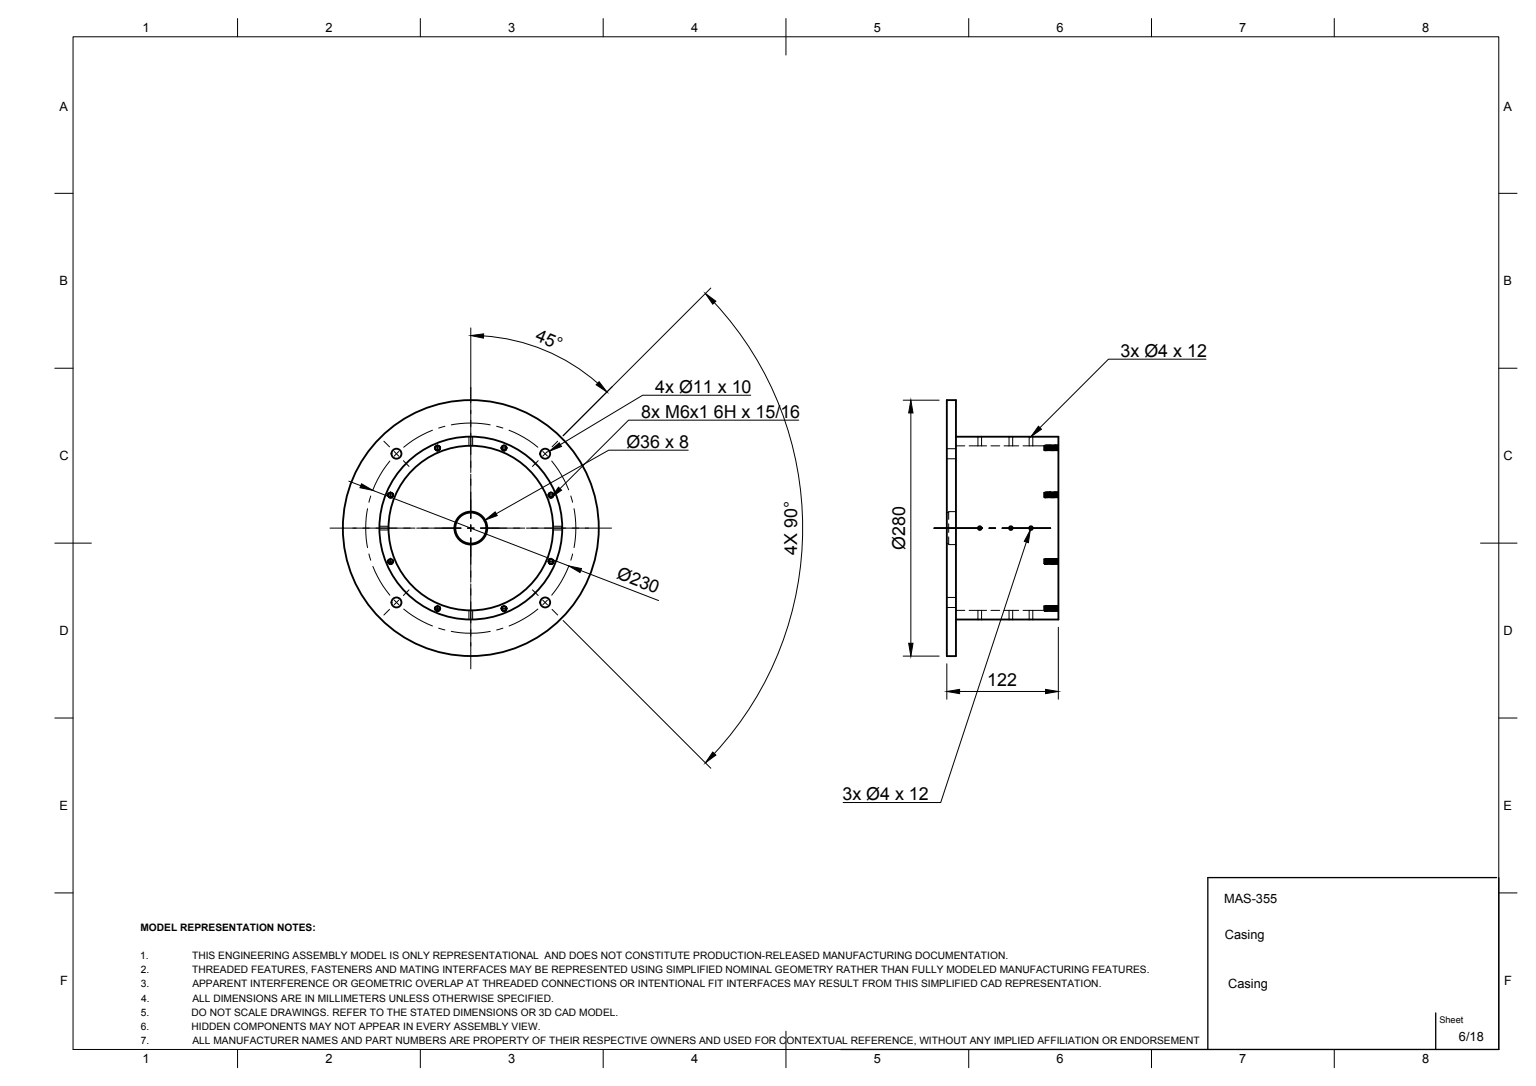
ISO-10303-21;
HEADER;
/* Generated by software containing ST-Developer
 * from STEP Tools, Inc. (www.steptools.com) 
 */

FILE_DESCRIPTION(
/* description */ ('Independent two-stage fixed-ring planetary gearbox,24/24/72 teeth,mod
ule2,20deg involutes,three planets per stage,4:1 x4:1=16:1. Native cut
-space/fillet/pattern tooth profiles derived from reusable gear blanks
; shared sun/planet/ring/carrier parts across both stages. Captured br
onze-journal input/carriers, headed retained planet pins, keyed inters
tage drive and modular keyed output interface. Native ideal gear links
; no torque, precision grade, production backlash/fits, lubrication, s
peed or life rating.'),
/* implementation_level */ '2;1');

FILE_NAME(
/* name */ 'Casing.step',
/* time_stamp */ '2026-11-08T19:10:00-08:00',
/* author */ (''),
/* organization */ (''),
/* preprocessor_version */ 'ST-DEVELOPER v20.2',
/* originating_system */ 'Autodesk Translation Framework v15.17.0.0',
/* authorisation */ '');

FILE_SCHEMA (('AUTOMOTIVE_DESIGN { 1 0 10303 214 3 1 1 }'));
ENDSEC;

DATA;
#10=MECHANICAL_DESIGN_GEOMETRIC_PRESENTATION_REPRESENTATION('',(#1163),#259224);
#1123=SHAPE_REPRESENTATION_RELATIONSHIP('SRR','None',#259370,#1143);
#1143=ADVANCED_BREP_SHAPE_REPRESENTATION('',(#1183),#259204);
#1163=STYLED_ITEM('',(#259479),#1183);
#1183=MANIFOLD_SOLID_BREP('Body1',#25150);
#1203=FACE_BOUND('',#3350,.T.);
#1204=FACE_BOUND('',#3352,.T.);
#1205=FACE_BOUND('',#3353,.T.);
#1206=FACE_BOUND('',#3354,.T.);
#1207=FACE_BOUND('',#3355,.T.);
#1208=FACE_BOUND('',#3356,.T.);
#1209=FACE_BOUND('',#3357,.T.);
#1210=FACE_BOUND('',#3358,.T.);
#1211=FACE_BOUND('',#3359,.T.);
#1212=FACE_BOUND('',#3360,.T.);
#1213=FACE_BOUND('',#3362,.T.);
#1214=FACE_BOUND('',#3363,.T.);
#1215=FACE_BOUND('',#3364,.T.);
#1216=FACE_BOUND('',#3365,.T.);
#1217=FACE_BOUND('',#3366,.T.);
#1218=FACE_BOUND('',#3367,.T.);
#1219=FACE_BOUND('',#3368,.T.);
#1220=FACE_BOUND('',#3369,.T.);
#1221=FACE_BOUND('',#3370,.T.);
#1222=FACE_BOUND('',#3372,.T.);
#1223=FACE_BOUND('',#3373,.T.);
#1224=FACE_BOUND('',#3374,.T.);
#1225=FACE_BOUND('',#3375,.T.);
#1226=FACE_BOUND('',#3376,.T.);
#1227=FACE_BOUND('',#3377,.T.);
#1228=FACE_BOUND('',#3378,.T.);
#1229=FACE_BOUND('',#3379,.T.);
#1230=FACE_BOUND('',#3380,.T.);
#1231=FACE_BOUND('',#3382,.T.);
#1232=FACE_BOUND('',#3383,.T.);
#1233=FACE_BOUND('',#3384,.T.);
#1234=FACE_BOUND('',#3385,.T.);
#1235=FACE_BOUND('',#3386,.T.);
#1236=FACE_BOUND('',#3390,.T.);
#1237=FACE_BOUND('',#3392,.T.);
#1238=FACE_BOUND('',#3393,.T.);
#1239=FACE_BOUND('',#3394,.T.);
#1240=FACE_BOUND('',#3395,.T.);
#1241=FACE_BOUND('',#3396,.T.);
#1318=B_SPLINE_SURFACE_WITH_KNOTS('',3,3,((#42197,#42198,#42199,#42200,
#42201,#42202,#42203,#42204,#42205,#42206,#42207,#42208,#42209,#42210,#42211,
#42212,#42213,#42214,#42215,#42216,#42217,#42218,#42219,#42220,#42221,#42222,
#42223,#42224,#42225,#42226,#42227,#42228,#42229,#42230,#42231,#42232,#42233,
#42234,#42235,#42236,#42237,#42238,#42239,#42240,#42241,#42242,#42243,#42244,
#42245,#42246,#42247,#42248,#42249,#42250,#42251,#42252,#42253,#42254,#42255,
#42256,#42257,#42258,#42259,#42260,#42261,#42262,#42263,#42264,#42265,#42266,
#42267,#42268,#42269,#42270,#42271,#42272,#42273,#42274,#42275,#42276,#42277,
#42278,#42279,#42280,#42281,#42282,#42283,#42284,#42285,#42286,#42287,#42288,
#42289,#42290,#42291,#42292,#42293,#42294,#42295,#42296),(#42297,#42298,
#42299,#42300,#42301,#42302,#42303,#42304,#42305,#42306,#42307,#42308,#42309,
#42310,#42311,#42312,#42313,#42314,#42315,#42316,#42317,#42318,#42319,#42320,
#42321,#42322,#42323,#42324,#42325,#42326,#42327,#42328,#42329,#42330,#42331,
#42332,#42333,#42334,#42335,#42336,#42337,#42338,#42339,#42340,#42341,#42342,
#42343,#42344,#42345,#42346,#42347,#42348,#42349,#42350,#42351,#42352,#42353,
#42354,#42355,#42356,#42357,#42358,#42359,#42360,#42361,#42362,#42363,#42364,
#42365,#42366,#42367,#42368,#42369,#42370,#42371,#42372,#42373,#42374,#42375,
#42376,#42377,#42378,#42379,#42380,#42381,#42382,#42383,#42384,#42385,#42386,
#42387,#42388,#42389,#42390,#42391,#42392,#42393,#42394,#42395,#42396),
(#42397,#42398,#42399,#42400,#42401,#42402,#42403,#42404,#42405,#42406,
#42407,#42408,#42409,#42410,#42411,#42412,#42413,#42414,#42415,#42416,#42417,
#42418,#42419,#42420,#42421,#42422,#42423,#42424,#42425,#42426,#42427,#42428,
#42429,#42430,#42431,#42432,#42433,#42434,#42435,#42436,#42437,#42438,#42439,
#42440,#42441,#42442,#42443,#42444,#42445,#42446,#42447,#42448,#42449,#42450,
#42451,#42452,#42453,#42454,#42455,#42456,#42457,#42458,#42459,#42460,#42461,
#42462,#42463,#42464,#42465,#42466,#42467,#42468,#42469,#42470,#42471,#42472,
#42473,#42474,#42475,#42476,#42477,#42478,#42479,#42480,#42481,#42482,#42483,
#42484,#42485,#42486,#42487,#42488,#42489,#42490,#42491,#42492,#42493,#42494,
#42495,#42496),(#42497,#42498,#42499,#42500,#42501,#42502,#42503,#42504,
#42505,#42506,#42507,#42508,#42509,#42510,#42511,#42512,#42513,#42514,#42515,
#42516,#42517,#42518,#42519,#42520,#42521,#42522,#42523,#42524,#42525,#42526,
#42527,#42528,#42529,#42530,#42531,#42532,#42533,#42534,#42535,#42536,#42537,
#42538,#42539,#42540,#42541,#42542,#42543,#42544,#42545,#42546,#42547,#42548,
#42549,#42550,#42551,#42552,#42553,#42554,#42555,#42556,#42557,#42558,#42559,
#42560,#42561,#42562,#42563,#42564,#42565,#42566,#42567,#42568,#42569,#42570,
#42571,#42572,#42573,#42574,#42575,#42576,#42577,#42578,#42579,#42580,#42581,
#42582,#42583,#42584,#42585,#42586,#42587,#42588,#42589,#42590,#42591,#42592,
#42593,#42594,#42595,#42596)),.UNSPECIFIED.,.F.,.F.,.F.,(4,4),(4,1,1,1,
1,1,1,1,1,1,1,1,1,1,1,1,1,1,1,1,1,1,1,1,1,1,1,1,1,1,1,1,1,1,1,1,1,1,1,1,
1,1,1,1,1,1,1,1,1,1,1,1,1,1,1,1,1,1,1,1,1,1,1,1,1,1,1,1,1,1,1,1,1,1,1,1,
1,1,1,1,1,1,1,1,1,1,1,1,1,1,1,1,1,1,1,1,1,4),(0.,0.064201349933887),(11.8589888623077,
12.8514087025213,13.843828542735,14.8362483829486,15.8286682231622,16.8210880633759,
17.8135079035895,18.8059277438031,19.7983475840168,20.7907674242304,21.783187264444,
22.7756071046577,23.7680269448713,24.7604467850849,25.7528666252985,26.7452864655122,
27.7377063057258,28.7301261459394,29.7225459861531,30.7149658263667,31.7073856665803,
32.699805506794,33.6922253470076,34.6846451872212,35.6770650274349,36.6694848676485,
37.6619047078621,38.6543245480758,39.6467443882894,40.639164228503,41.6315840687166,
42.6240039089303,43.6164237491439,44.6088435893575,45.6012634295712,46.5936832697848,
47.5861031099984,48.5785229502121,49.5709427904257,50.5633626306393,51.555782470853,
52.5482023110666,53.5406221512802,54.5330419914939,55.5254618317075,56.5178816719211,
57.5103015121348,58.5027213523484,59.495141192562,60.4875610327756,61.4799808729893,
62.4724007132029,63.4648205534165,64.4572403936302,65.4496602338438,66.4420800740574,
67.4344999142711,68.4269197544847,69.4193395946983,70.411759434912,71.4041792751256,
72.3965991153392,73.3890189555529,74.3814387957665,75.3738586359801,76.3662784761938,
77.3586983164074,78.351118156621,79.3435379968347,80.3359578370483,81.3283776772619,
82.3207975174756,83.3132173576892,84.3056371979028,85.2980570381164,86.2904768783301,
87.2828967185437,88.2753165587573,89.267736398971,90.2601562391846,91.2525760793982,
92.2449959196119,93.2374157598255,94.2298356000391,95.2222554402528,96.2146752804664,
97.20709512068,98.1995149608937,99.1919348011073,100.184354641321,101.176774481535,
102.169194321748,103.161614161962,104.154034002175,105.146453842389,106.138873682603,
107.131293522816,108.12371336303),.UNSPECIFIED.);
#1319=B_SPLINE_SURFACE_WITH_KNOTS('',3,3,((#42716,#42717,#42718,#42719,
#42720,#42721,#42722,#42723,#42724,#42725,#42726,#42727,#42728,#42729,#42730,
#42731,#42732,#42733,#42734,#42735,#42736,#42737,#42738,#42739,#42740,#42741,
#42742,#42743,#42744,#42745,#42746,#42747,#42748,#42749,#42750,#42751,#42752,
#42753,#42754,#42755,#42756,#42757,#42758,#42759,#42760,#42761,#42762,#42763,
#42764,#42765,#42766,#42767,#42768,#42769,#42770,#42771,#42772,#42773,#42774,
#42775,#42776,#42777,#42778,#42779,#42780,#42781,#42782,#42783,#42784,#42785,
#42786,#42787,#42788,#42789,#42790,#42791,#42792,#42793,#42794,#42795,#42796,
#42797,#42798,#42799,#42800,#42801,#42802,#42803,#42804,#42805,#42806,#42807,
#42808,#42809,#42810,#42811,#42812,#42813,#42814,#42815),(#42816,#42817,
#42818,#42819,#42820,#42821,#42822,#42823,#42824,#42825,#42826,#42827,#42828,
#42829,#42830,#42831,#42832,#42833,#42834,#42835,#42836,#42837,#42838,#42839,
#42840,#42841,#42842,#42843,#42844,#42845,#42846,#42847,#42848,#42849,#42850,
#42851,#42852,#42853,#42854,#42855,#42856,#42857,#42858,#42859,#42860,#42861,
#42862,#42863,#42864,#42865,#42866,#42867,#42868,#42869,#42870,#42871,#42872,
#42873,#42874,#42875,#42876,#42877,#42878,#42879,#42880,#42881,#42882,#42883,
#42884,#42885,#42886,#42887,#42888,#42889,#42890,#42891,#42892,#42893,#42894,
#42895,#42896,#42897,#42898,#42899,#42900,#42901,#42902,#42903,#42904,#42905,
#42906,#42907,#42908,#42909,#42910,#42911,#42912,#42913,#42914,#42915),
(#42916,#42917,#42918,#42919,#42920,#42921,#42922,#42923,#42924,#42925,
#42926,#42927,#42928,#42929,#42930,#42931,#42932,#42933,#42934,#42935,#42936,
#42937,#42938,#42939,#42940,#42941,#42942,#42943,#42944,#42945,#42946,#42947,
#42948,#42949,#42950,#42951,#42952,#42953,#42954,#42955,#42956,#42957,#42958,
#42959,#42960,#42961,#42962,#42963,#42964,#42965,#42966,#42967,#42968,#42969,
#42970,#42971,#42972,#42973,#42974,#42975,#42976,#42977,#42978,#42979,#42980,
#42981,#42982,#42983,#42984,#42985,#42986,#42987,#42988,#42989,#42990,#42991,
#42992,#42993,#42994,#42995,#42996,#42997,#42998,#42999,#43000,#43001,#43002,
#43003,#43004,#43005,#43006,#43007,#43008,#43009,#43010,#43011,#43012,#43013,
#43014,#43015),(#43016,#43017,#43018,#43019,#43020,#43021,#43022,#43023,
#43024,#43025,#43026,#43027,#43028,#43029,#43030,#43031,#43032,#43033,#43034,
#43035,#43036,#43037,#43038,#43039,#43040,#43041,#43042,#43043,#43044,#43045,
#43046,#43047,#43048,#43049,#43050,#43051,#43052,#43053,#43054,#43055,#43056,
#43057,#43058,#43059,#43060,#43061,#43062,#43063,#43064,#43065,#43066,#43067,
#43068,#43069,#43070,#43071,#43072,#43073,#43074,#43075,#43076,#43077,#43078,
#43079,#43080,#43081,#43082,#43083,#43084,#43085,#43086,#43087,#43088,#43089,
#43090,#43091,#43092,#43093,#43094,#43095,#43096,#43097,#43098,#43099,#43100,
#43101,#43102,#43103,#43104,#43105,#43106,#43107,#43108,#43109,#43110,#43111,
#43112,#43113,#43114,#43115)),.UNSPECIFIED.,.F.,.F.,.F.,(4,4),(4,1,1,1,
1,1,1,1,1,1,1,1,1,1,1,1,1,1,1,1,1,1,1,1,1,1,1,1,1,1,1,1,1,1,1,1,1,1,1,1,
1,1,1,1,1,1,1,1,1,1,1,1,1,1,1,1,1,1,1,1,1,1,1,1,1,1,1,1,1,1,1,1,1,1,1,1,
1,1,1,1,1,1,1,1,1,1,1,1,1,1,1,1,1,1,1,1,1,4),(0.,0.064201349933887),(14.3984001269718,
15.3908199671854,16.3832398073991,17.3756596476127,18.3680794878263,19.36049932804,
20.3529191682536,21.3453390084672,22.3377588486809,23.3301786888945,24.3225985291081,
25.3150183693218,26.3074382095354,27.299858049749,28.2922778899627,29.2846977301763,
30.2771175703899,31.2695374106036,32.2619572508172,33.2543770910308,34.2467969312444,
35.2392167714581,36.2316366116717,37.2240564518853,38.216476292099,39.2088961323126,
40.2013159725262,41.1937358127399,42.1861556529535,43.1785754931671,44.1709953333808,
45.1634151735944,46.155835013808,47.1482548540217,48.1406746942353,49.1330945344489,
50.1255143746626,51.1179342148762,52.1103540550898,53.1027738953035,54.0951937355171,
55.0876135757307,56.0800334159443,57.072453256158,58.0648730963716,59.0572929365852,
60.0497127767989,61.0421326170125,62.0345524572261,63.0269722974398,64.0193921376534,
65.011811977867,66.0042318180807,66.9966516582943,67.9890714985079,68.9814913387216,
69.9739111789352,70.9663310191488,71.9587508593625,72.9511706995761,73.9435905397897,
74.9360103800034,75.928430220217,76.9208500604306,77.9132699006443,78.9056897408579,
79.8981095810715,80.8905294212852,81.8829492614988,82.8753691017124,83.867788941926,
84.8602087821397,85.8526286223533,86.8450484625669,87.8374683027806,88.8298881429942,
89.8223079832078,90.8147278234215,91.8071476636351,92.7995675038487,93.7919873440624,
94.784407184276,95.7768270244896,96.7692468647032,97.7616667049169,98.7540865451305,
99.7465063853441,100.738926225558,101.731346065771,102.723765905985,103.716185746199,
104.708605586412,105.701025426626,106.69344526684,107.685865107053,108.678284947267,
109.67070478748,110.663124627694),.UNSPECIFIED.);
#1320=B_SPLINE_SURFACE_WITH_KNOTS('',3,3,((#43444,#43445,#43446,#43447,
#43448,#43449,#43450,#43451,#43452,#43453,#43454,#43455,#43456,#43457,#43458,
#43459,#43460,#43461,#43462,#43463,#43464,#43465,#43466,#43467,#43468,#43469,
#43470,#43471,#43472,#43473,#43474,#43475,#43476,#43477,#43478,#43479,#43480,
#43481,#43482,#43483,#43484,#43485,#43486,#43487,#43488,#43489,#43490,#43491,
#43492,#43493,#43494,#43495,#43496,#43497,#43498,#43499,#43500,#43501,#43502,
#43503,#43504,#43505,#43506,#43507,#43508,#43509,#43510,#43511,#43512,#43513,
#43514,#43515,#43516,#43517,#43518,#43519,#43520,#43521,#43522,#43523,#43524,
#43525,#43526,#43527,#43528,#43529,#43530,#43531,#43532,#43533,#43534,#43535,
#43536,#43537,#43538,#43539,#43540,#43541,#43542,#43543),(#43544,#43545,
#43546,#43547,#43548,#43549,#43550,#43551,#43552,#43553,#43554,#43555,#43556,
#43557,#43558,#43559,#43560,#43561,#43562,#43563,#43564,#43565,#43566,#43567,
#43568,#43569,#43570,#43571,#43572,#43573,#43574,#43575,#43576,#43577,#43578,
#43579,#43580,#43581,#43582,#43583,#43584,#43585,#43586,#43587,#43588,#43589,
#43590,#43591,#43592,#43593,#43594,#43595,#43596,#43597,#43598,#43599,#43600,
#43601,#43602,#43603,#43604,#43605,#43606,#43607,#43608,#43609,#43610,#43611,
#43612,#43613,#43614,#43615,#43616,#43617,#43618,#43619,#43620,#43621,#43622,
#43623,#43624,#43625,#43626,#43627,#43628,#43629,#43630,#43631,#43632,#43633,
#43634,#43635,#43636,#43637,#43638,#43639,#43640,#43641,#43642,#43643),
(#43644,#43645,#43646,#43647,#43648,#43649,#43650,#43651,#43652,#43653,
#43654,#43655,#43656,#43657,#43658,#43659,#43660,#43661,#43662,#43663,#43664,
#43665,#43666,#43667,#43668,#43669,#43670,#43671,#43672,#43673,#43674,#43675,
#43676,#43677,#43678,#43679,#43680,#43681,#43682,#43683,#43684,#43685,#43686,
#43687,#43688,#43689,#43690,#43691,#43692,#43693,#43694,#43695,#43696,#43697,
#43698,#43699,#43700,#43701,#43702,#43703,#43704,#43705,#43706,#43707,#43708,
#43709,#43710,#43711,#43712,#43713,#43714,#43715,#43716,#43717,#43718,#43719,
#43720,#43721,#43722,#43723,#43724,#43725,#43726,#43727,#43728,#43729,#43730,
#43731,#43732,#43733,#43734,#43735,#43736,#43737,#43738,#43739,#43740,#43741,
#43742,#43743),(#43744,#43745,#43746,#43747,#43748,#43749,#43750,#43751,
#43752,#43753,#43754,#43755,#43756,#43757,#43758,#43759,#43760,#43761,#43762,
#43763,#43764,#43765,#43766,#43767,#43768,#43769,#43770,#43771,#43772,#43773,
#43774,#43775,#43776,#43777,#43778,#43779,#43780,#43781,#43782,#43783,#43784,
#43785,#43786,#43787,#43788,#43789,#43790,#43791,#43792,#43793,#43794,#43795,
#43796,#43797,#43798,#43799,#43800,#43801,#43802,#43803,#43804,#43805,#43806,
#43807,#43808,#43809,#43810,#43811,#43812,#43813,#43814,#43815,#43816,#43817,
#43818,#43819,#43820,#43821,#43822,#43823,#43824,#43825,#43826,#43827,#43828,
#43829,#43830,#43831,#43832,#43833,#43834,#43835,#43836,#43837,#43838,#43839,
#43840,#43841,#43842,#43843)),.UNSPECIFIED.,.F.,.F.,.F.,(4,4),(4,1,1,1,
1,1,1,1,1,1,1,1,1,1,1,1,1,1,1,1,1,1,1,1,1,1,1,1,1,1,1,1,1,1,1,1,1,1,1,1,
1,1,1,1,1,1,1,1,1,1,1,1,1,1,1,1,1,1,1,1,1,1,1,1,1,1,1,1,1,1,1,1,1,1,1,1,
1,1,1,1,1,1,1,1,1,1,1,1,1,1,1,1,1,1,1,1,1,4),(0.,0.064201349933887),(11.8589888623077,
12.8514087025213,13.843828542735,14.8362483829486,15.8286682231622,16.8210880633759,
17.8135079035895,18.8059277438031,19.7983475840168,20.7907674242304,21.783187264444,
22.7756071046577,23.7680269448713,24.7604467850849,25.7528666252986,26.7452864655122,
27.7377063057259,28.7301261459395,29.7225459861531,30.7149658263668,31.7073856665804,
32.699805506794,33.6922253470076,34.6846451872213,35.6770650274349,36.6694848676485,
37.6619047078622,38.6543245480758,39.6467443882895,40.6391642285031,41.6315840687167,
42.6240039089304,43.616423749144,44.6088435893576,45.6012634295713,46.5936832697849,
47.5861031099985,48.5785229502122,49.5709427904258,50.5633626306394,51.5557824708531,
52.5482023110667,53.5406221512803,54.533041991494,55.5254618317076,56.5178816719212,
57.5103015121349,58.5027213523485,59.4951411925621,60.4875610327758,61.4799808729894,
62.472400713203,63.4648205534167,64.4572403936303,65.4496602338439,66.4420800740576,
67.4344999142712,68.4269197544848,69.4193395946985,70.4117594349121,71.4041792751257,
72.3965991153394,73.389018955553,74.3814387957666,75.3738586359803,76.3662784761939,
77.3586983164075,78.3511181566212,79.3435379968348,80.3359578370484,81.3283776772621,
82.3207975174757,83.3132173576894,84.305637197903,85.2980570381166,86.2904768783303,
87.2828967185439,88.2753165587575,89.2677363989712,90.2601562391848,91.2525760793984,
92.2449959196121,93.2374157598257,94.2298356000393,95.222255440253,96.2146752804666,
97.2070951206802,98.1995149608939,99.1919348011075,100.184354641321,101.176774481535,
102.169194321748,103.161614161962,104.154034002176,105.146453842389,106.138873682603,
107.131293522817,108.12371336303),.UNSPECIFIED.);
#1321=B_SPLINE_SURFACE_WITH_KNOTS('',3,3,((#43963,#43964,#43965,#43966,
#43967,#43968,#43969,#43970,#43971,#43972,#43973,#43974,#43975,#43976,#43977,
#43978,#43979,#43980,#43981,#43982,#43983,#43984,#43985,#43986,#43987,#43988,
#43989,#43990,#43991,#43992,#43993,#43994,#43995,#43996,#43997,#43998,#43999,
#44000,#44001,#44002,#44003,#44004,#44005,#44006,#44007,#44008,#44009,#44010,
#44011,#44012,#44013,#44014,#44015,#44016,#44017,#44018,#44019,#44020,#44021,
#44022,#44023,#44024,#44025,#44026,#44027,#44028,#44029,#44030,#44031,#44032,
#44033,#44034,#44035,#44036,#44037,#44038,#44039,#44040,#44041,#44042,#44043,
#44044,#44045,#44046,#44047,#44048,#44049,#44050,#44051,#44052,#44053,#44054,
#44055,#44056,#44057,#44058,#44059,#44060,#44061,#44062),(#44063,#44064,
#44065,#44066,#44067,#44068,#44069,#44070,#44071,#44072,#44073,#44074,#44075,
#44076,#44077,#44078,#44079,#44080,#44081,#44082,#44083,#44084,#44085,#44086,
#44087,#44088,#44089,#44090,#44091,#44092,#44093,#44094,#44095,#44096,#44097,
#44098,#44099,#44100,#44101,#44102,#44103,#44104,#44105,#44106,#44107,#44108,
#44109,#44110,#44111,#44112,#44113,#44114,#44115,#44116,#44117,#44118,#44119,
#44120,#44121,#44122,#44123,#44124,#44125,#44126,#44127,#44128,#44129,#44130,
#44131,#44132,#44133,#44134,#44135,#44136,#44137,#44138,#44139,#44140,#44141,
#44142,#44143,#44144,#44145,#44146,#44147,#44148,#44149,#44150,#44151,#44152,
#44153,#44154,#44155,#44156,#44157,#44158,#44159,#44160,#44161,#44162),
(#44163,#44164,#44165,#44166,#44167,#44168,#44169,#44170,#44171,#44172,
#44173,#44174,#44175,#44176,#44177,#44178,#44179,#44180,#44181,#44182,#44183,
#44184,#44185,#44186,#44187,#44188,#44189,#44190,#44191,#44192,#44193,#44194,
#44195,#44196,#44197,#44198,#44199,#44200,#44201,#44202,#44203,#44204,#44205,
#44206,#44207,#44208,#44209,#44210,#44211,#44212,#44213,#44214,#44215,#44216,
#44217,#44218,#44219,#44220,#44221,#44222,#44223,#44224,#44225,#44226,#44227,
#44228,#44229,#44230,#44231,#44232,#44233,#44234,#44235,#44236,#44237,#44238,
#44239,#44240,#44241,#44242,#44243,#44244,#44245,#44246,#44247,#44248,#44249,
#44250,#44251,#44252,#44253,#44254,#44255,#44256,#44257,#44258,#44259,#44260,
#44261,#44262),(#44263,#44264,#44265,#44266,#44267,#44268,#44269,#44270,
#44271,#44272,#44273,#44274,#44275,#44276,#44277,#44278,#44279,#44280,#44281,
#44282,#44283,#44284,#44285,#44286,#44287,#44288,#44289,#44290,#44291,#44292,
#44293,#44294,#44295,#44296,#44297,#44298,#44299,#44300,#44301,#44302,#44303,
#44304,#44305,#44306,#44307,#44308,#44309,#44310,#44311,#44312,#44313,#44314,
#44315,#44316,#44317,#44318,#44319,#44320,#44321,#44322,#44323,#44324,#44325,
#44326,#44327,#44328,#44329,#44330,#44331,#44332,#44333,#44334,#44335,#44336,
#44337,#44338,#44339,#44340,#44341,#44342,#44343,#44344,#44345,#44346,#44347,
#44348,#44349,#44350,#44351,#44352,#44353,#44354,#44355,#44356,#44357,#44358,
#44359,#44360,#44361,#44362)),.UNSPECIFIED.,.F.,.F.,.F.,(4,4),(4,1,1,1,
1,1,1,1,1,1,1,1,1,1,1,1,1,1,1,1,1,1,1,1,1,1,1,1,1,1,1,1,1,1,1,1,1,1,1,1,
1,1,1,1,1,1,1,1,1,1,1,1,1,1,1,1,1,1,1,1,1,1,1,1,1,1,1,1,1,1,1,1,1,1,1,1,
1,1,1,1,1,1,1,1,1,1,1,1,1,1,1,1,1,1,1,1,1,4),(0.,0.064201349933887),(14.3984001269718,
15.3908199671854,16.3832398073991,17.3756596476127,18.3680794878263,19.36049932804,
20.3529191682536,21.3453390084673,22.3377588486809,23.3301786888945,24.3225985291082,
25.3150183693218,26.3074382095354,27.2998580497491,28.2922778899627,29.2846977301763,
30.27711757039,31.2695374106036,32.2619572508172,33.2543770910309,34.2467969312445,
35.2392167714581,36.2316366116718,37.2240564518854,38.216476292099,39.2088961323127,
40.2013159725263,41.1937358127399,42.1861556529536,43.1785754931672,44.1709953333808,
45.1634151735945,46.1558350138081,47.1482548540217,48.1406746942354,49.133094534449,
50.1255143746626,51.1179342148763,52.1103540550899,53.1027738953035,54.0951937355172,
55.0876135757308,56.0800334159444,57.0724532561581,58.0648730963717,59.0572929365853,
60.049712776799,61.0421326170126,62.0345524572262,63.0269722974399,64.0193921376535,
65.0118119778672,66.0042318180808,66.9966516582944,67.9890714985081,68.9814913387217,
69.9739111789353,70.966331019149,71.9587508593626,72.9511706995762,73.9435905397899,
74.9360103800035,75.9284302202171,76.9208500604308,77.9132699006444,78.905689740858,
79.8981095810717,80.8905294212853,81.8829492614989,82.8753691017126,83.8677889419262,
84.8602087821398,85.8526286223535,86.8450484625671,87.8374683027807,88.8298881429944,
89.822307983208,90.8147278234216,91.8071476636353,92.7995675038489,93.7919873440625,
94.7844071842762,95.7768270244898,96.7692468647034,97.7616667049171,98.7540865451307,
99.7465063853443,100.738926225558,101.731346065772,102.723765905985,103.716185746199,
104.708605586413,105.701025426626,106.69344526684,107.685865107053,108.678284947267,
109.670704787481,110.663124627694),.UNSPECIFIED.);
#1322=B_SPLINE_SURFACE_WITH_KNOTS('',3,3,((#44691,#44692,#44693,#44694,
#44695,#44696,#44697,#44698,#44699,#44700,#44701,#44702,#44703,#44704,#44705,
#44706,#44707,#44708,#44709,#44710,#44711,#44712,#44713,#44714,#44715,#44716,
#44717,#44718,#44719,#44720,#44721,#44722,#44723,#44724,#44725,#44726,#44727,
#44728,#44729,#44730,#44731,#44732,#44733,#44734,#44735,#44736,#44737,#44738,
#44739,#44740,#44741,#44742,#44743,#44744,#44745,#44746,#44747,#44748,#44749,
#44750,#44751,#44752,#44753,#44754,#44755,#44756,#44757,#44758,#44759,#44760,
#44761,#44762,#44763,#44764,#44765,#44766,#44767,#44768,#44769,#44770,#44771,
#44772,#44773,#44774,#44775,#44776,#44777,#44778,#44779,#44780,#44781,#44782,
#44783,#44784,#44785,#44786,#44787,#44788,#44789,#44790),(#44791,#44792,
#44793,#44794,#44795,#44796,#44797,#44798,#44799,#44800,#44801,#44802,#44803,
#44804,#44805,#44806,#44807,#44808,#44809,#44810,#44811,#44812,#44813,#44814,
#44815,#44816,#44817,#44818,#44819,#44820,#44821,#44822,#44823,#44824,#44825,
#44826,#44827,#44828,#44829,#44830,#44831,#44832,#44833,#44834,#44835,#44836,
#44837,#44838,#44839,#44840,#44841,#44842,#44843,#44844,#44845,#44846,#44847,
#44848,#44849,#44850,#44851,#44852,#44853,#44854,#44855,#44856,#44857,#44858,
#44859,#44860,#44861,#44862,#44863,#44864,#44865,#44866,#44867,#44868,#44869,
#44870,#44871,#44872,#44873,#44874,#44875,#44876,#44877,#44878,#44879,#44880,
#44881,#44882,#44883,#44884,#44885,#44886,#44887,#44888,#44889,#44890),
(#44891,#44892,#44893,#44894,#44895,#44896,#44897,#44898,#44899,#44900,
#44901,#44902,#44903,#44904,#44905,#44906,#44907,#44908,#44909,#44910,#44911,
#44912,#44913,#44914,#44915,#44916,#44917,#44918,#44919,#44920,#44921,#44922,
#44923,#44924,#44925,#44926,#44927,#44928,#44929,#44930,#44931,#44932,#44933,
#44934,#44935,#44936,#44937,#44938,#44939,#44940,#44941,#44942,#44943,#44944,
#44945,#44946,#44947,#44948,#44949,#44950,#44951,#44952,#44953,#44954,#44955,
#44956,#44957,#44958,#44959,#44960,#44961,#44962,#44963,#44964,#44965,#44966,
#44967,#44968,#44969,#44970,#44971,#44972,#44973,#44974,#44975,#44976,#44977,
#44978,#44979,#44980,#44981,#44982,#44983,#44984,#44985,#44986,#44987,#44988,
#44989,#44990),(#44991,#44992,#44993,#44994,#44995,#44996,#44997,#44998,
#44999,#45000,#45001,#45002,#45003,#45004,#45005,#45006,#45007,#45008,#45009,
#45010,#45011,#45012,#45013,#45014,#45015,#45016,#45017,#45018,#45019,#45020,
#45021,#45022,#45023,#45024,#45025,#45026,#45027,#45028,#45029,#45030,#45031,
#45032,#45033,#45034,#45035,#45036,#45037,#45038,#45039,#45040,#45041,#45042,
#45043,#45044,#45045,#45046,#45047,#45048,#45049,#45050,#45051,#45052,#45053,
#45054,#45055,#45056,#45057,#45058,#45059,#45060,#45061,#45062,#45063,#45064,
#45065,#45066,#45067,#45068,#45069,#45070,#45071,#45072,#45073,#45074,#45075,
#45076,#45077,#45078,#45079,#45080,#45081,#45082,#45083,#45084,#45085,#45086,
#45087,#45088,#45089,#45090)),.UNSPECIFIED.,.F.,.F.,.F.,(4,4),(4,1,1,1,
1,1,1,1,1,1,1,1,1,1,1,1,1,1,1,1,1,1,1,1,1,1,1,1,1,1,1,1,1,1,1,1,1,1,1,1,
1,1,1,1,1,1,1,1,1,1,1,1,1,1,1,1,1,1,1,1,1,1,1,1,1,1,1,1,1,1,1,1,1,1,1,1,
1,1,1,1,1,1,1,1,1,1,1,1,1,1,1,1,1,1,1,1,1,4),(0.,0.064201349933887),(11.8589888623078,
12.8514087025215,13.8438285427351,14.8362483829487,15.8286682231624,16.821088063376,
17.8135079035896,18.8059277438032,19.7983475840169,20.7907674242305,21.7831872644441,
22.7756071046578,23.7680269448714,24.760446785085,25.7528666252987,26.7452864655123,
27.7377063057259,28.7301261459396,29.7225459861532,30.7149658263668,31.7073856665805,
32.6998055067941,33.6922253470077,34.6846451872214,35.677065027435,36.6694848676486,
37.6619047078623,38.6543245480759,39.6467443882895,40.6391642285032,41.6315840687168,
42.6240039089304,43.6164237491441,44.6088435893577,45.6012634295713,46.593683269785,
47.5861031099986,48.5785229502122,49.5709427904259,50.5633626306395,51.5557824708531,
52.5482023110668,53.5406221512804,54.533041991494,55.5254618317077,56.5178816719213,
57.5103015121349,58.5027213523486,59.4951411925622,60.4875610327758,61.4799808729895,
62.4724007132031,63.4648205534167,64.4572403936303,65.449660233844,66.4420800740576,
67.4344999142712,68.4269197544849,69.4193395946985,70.4117594349121,71.4041792751258,
72.3965991153394,73.389018955553,74.3814387957667,75.3738586359803,76.3662784761939,
77.3586983164076,78.3511181566212,79.3435379968348,80.3359578370485,81.3283776772621,
82.3207975174757,83.3132173576894,84.305637197903,85.2980570381166,86.2904768783303,
87.2828967185439,88.2753165587575,89.2677363989712,90.2601562391848,91.2525760793984,
92.2449959196121,93.2374157598257,94.2298356000393,95.222255440253,96.2146752804666,
97.2070951206802,98.1995149608939,99.1919348011075,100.184354641321,101.176774481535,
102.169194321748,103.161614161962,104.154034002176,105.146453842389,106.138873682603,
107.131293522817,108.12371336303),.UNSPECIFIED.);
#1323=B_SPLINE_SURFACE_WITH_KNOTS('',3,3,((#45210,#45211,#45212,#45213,
#45214,#45215,#45216,#45217,#45218,#45219,#45220,#45221,#45222,#45223,#45224,
#45225,#45226,#45227,#45228,#45229,#45230,#45231,#45232,#45233,#45234,#45235,
#45236,#45237,#45238,#45239,#45240,#45241,#45242,#45243,#45244,#45245,#45246,
#45247,#45248,#45249,#45250,#45251,#45252,#45253,#45254,#45255,#45256,#45257,
#45258,#45259,#45260,#45261,#45262,#45263,#45264,#45265,#45266,#45267,#45268,
#45269,#45270,#45271,#45272,#45273,#45274,#45275,#45276,#45277,#45278,#45279,
#45280,#45281,#45282,#45283,#45284,#45285,#45286,#45287,#45288,#45289,#45290,
#45291,#45292,#45293,#45294,#45295,#45296,#45297,#45298,#45299,#45300,#45301,
#45302,#45303,#45304,#45305,#45306,#45307,#45308,#45309),(#45310,#45311,
#45312,#45313,#45314,#45315,#45316,#45317,#45318,#45319,#45320,#45321,#45322,
#45323,#45324,#45325,#45326,#45327,#45328,#45329,#45330,#45331,#45332,#45333,
#45334,#45335,#45336,#45337,#45338,#45339,#45340,#45341,#45342,#45343,#45344,
#45345,#45346,#45347,#45348,#45349,#45350,#45351,#45352,#45353,#45354,#45355,
#45356,#45357,#45358,#45359,#45360,#45361,#45362,#45363,#45364,#45365,#45366,
#45367,#45368,#45369,#45370,#45371,#45372,#45373,#45374,#45375,#45376,#45377,
#45378,#45379,#45380,#45381,#45382,#45383,#45384,#45385,#45386,#45387,#45388,
#45389,#45390,#45391,#45392,#45393,#45394,#45395,#45396,#45397,#45398,#45399,
#45400,#45401,#45402,#45403,#45404,#45405,#45406,#45407,#45408,#45409),
(#45410,#45411,#45412,#45413,#45414,#45415,#45416,#45417,#45418,#45419,
#45420,#45421,#45422,#45423,#45424,#45425,#45426,#45427,#45428,#45429,#45430,
#45431,#45432,#45433,#45434,#45435,#45436,#45437,#45438,#45439,#45440,#45441,
#45442,#45443,#45444,#45445,#45446,#45447,#45448,#45449,#45450,#45451,#45452,
#45453,#45454,#45455,#45456,#45457,#45458,#45459,#45460,#45461,#45462,#45463,
#45464,#45465,#45466,#45467,#45468,#45469,#45470,#45471,#45472,#45473,#45474,
#45475,#45476,#45477,#45478,#45479,#45480,#45481,#45482,#45483,#45484,#45485,
#45486,#45487,#45488,#45489,#45490,#45491,#45492,#45493,#45494,#45495,#45496,
#45497,#45498,#45499,#45500,#45501,#45502,#45503,#45504,#45505,#45506,#45507,
#45508,#45509),(#45510,#45511,#45512,#45513,#45514,#45515,#45516,#45517,
#45518,#45519,#45520,#45521,#45522,#45523,#45524,#45525,#45526,#45527,#45528,
#45529,#45530,#45531,#45532,#45533,#45534,#45535,#45536,#45537,#45538,#45539,
#45540,#45541,#45542,#45543,#45544,#45545,#45546,#45547,#45548,#45549,#45550,
#45551,#45552,#45553,#45554,#45555,#45556,#45557,#45558,#45559,#45560,#45561,
#45562,#45563,#45564,#45565,#45566,#45567,#45568,#45569,#45570,#45571,#45572,
#45573,#45574,#45575,#45576,#45577,#45578,#45579,#45580,#45581,#45582,#45583,
#45584,#45585,#45586,#45587,#45588,#45589,#45590,#45591,#45592,#45593,#45594,
#45595,#45596,#45597,#45598,#45599,#45600,#45601,#45602,#45603,#45604,#45605,
#45606,#45607,#45608,#45609)),.UNSPECIFIED.,.F.,.F.,.F.,(4,4),(4,1,1,1,
1,1,1,1,1,1,1,1,1,1,1,1,1,1,1,1,1,1,1,1,1,1,1,1,1,1,1,1,1,1,1,1,1,1,1,1,
1,1,1,1,1,1,1,1,1,1,1,1,1,1,1,1,1,1,1,1,1,1,1,1,1,1,1,1,1,1,1,1,1,1,1,1,
1,1,1,1,1,1,1,1,1,1,1,1,1,1,1,1,1,1,1,1,1,4),(0.,0.064201349933887),(14.3984001269719,
15.3908199671856,16.3832398073992,17.3756596476128,18.3680794878265,19.3604993280401,
20.3529191682537,21.3453390084674,22.337758848681,23.3301786888946,24.3225985291083,
25.3150183693219,26.3074382095355,27.2998580497492,28.2922778899628,29.2846977301764,
30.2771175703901,31.2695374106037,32.2619572508173,33.2543770910309,34.2467969312446,
35.2392167714582,36.2316366116718,37.2240564518855,38.2164762920991,39.2088961323127,
40.2013159725264,41.19373581274,42.1861556529536,43.1785754931673,44.1709953333809,
45.1634151735945,46.1558350138082,47.1482548540218,48.1406746942354,49.1330945344491,
50.1255143746627,51.1179342148763,52.11035405509,53.1027738953036,54.0951937355172,
55.0876135757309,56.0800334159445,57.0724532561581,58.0648730963718,59.0572929365854,
60.049712776799,61.0421326170127,62.0345524572263,63.0269722974399,64.0193921376536,
65.0118119778672,66.0042318180808,66.9966516582945,67.9890714985081,68.9814913387217,
69.9739111789354,70.966331019149,71.9587508593626,72.9511706995763,73.9435905397899,
74.9360103800035,75.9284302202172,76.9208500604308,77.9132699006444,78.9056897408581,
79.8981095810717,80.8905294212853,81.882949261499,82.8753691017126,83.8677889419262,
84.8602087821399,85.8526286223535,86.8450484625671,87.8374683027808,88.8298881429944,
89.822307983208,90.8147278234217,91.8071476636353,92.7995675038489,93.7919873440626,
94.7844071842762,95.7768270244898,96.7692468647035,97.7616667049171,98.7540865451307,
99.7465063853444,100.738926225558,101.731346065772,102.723765905985,103.716185746199,
104.708605586413,105.701025426626,106.69344526684,107.685865107053,108.678284947267,
109.670704787481,110.663124627694),.UNSPECIFIED.);
#1324=B_SPLINE_SURFACE_WITH_KNOTS('',3,3,((#45938,#45939,#45940,#45941,
#45942,#45943,#45944,#45945,#45946,#45947,#45948,#45949,#45950,#45951,#45952,
#45953,#45954,#45955,#45956,#45957,#45958,#45959,#45960,#45961,#45962,#45963,
#45964,#45965,#45966,#45967,#45968,#45969,#45970,#45971,#45972,#45973,#45974,
#45975,#45976,#45977,#45978,#45979,#45980,#45981,#45982,#45983,#45984,#45985,
#45986,#45987,#45988,#45989,#45990,#45991,#45992,#45993,#45994,#45995,#45996,
#45997,#45998,#45999,#46000,#46001,#46002,#46003,#46004,#46005,#46006,#46007,
#46008,#46009,#46010,#46011,#46012,#46013,#46014,#46015,#46016,#46017,#46018,
#46019,#46020,#46021,#46022,#46023,#46024,#46025,#46026,#46027,#46028,#46029,
#46030,#46031,#46032,#46033,#46034,#46035,#46036,#46037),(#46038,#46039,
#46040,#46041,#46042,#46043,#46044,#46045,#46046,#46047,#46048,#46049,#46050,
#46051,#46052,#46053,#46054,#46055,#46056,#46057,#46058,#46059,#46060,#46061,
#46062,#46063,#46064,#46065,#46066,#46067,#46068,#46069,#46070,#46071,#46072,
#46073,#46074,#46075,#46076,#46077,#46078,#46079,#46080,#46081,#46082,#46083,
#46084,#46085,#46086,#46087,#46088,#46089,#46090,#46091,#46092,#46093,#46094,
#46095,#46096,#46097,#46098,#46099,#46100,#46101,#46102,#46103,#46104,#46105,
#46106,#46107,#46108,#46109,#46110,#46111,#46112,#46113,#46114,#46115,#46116,
#46117,#46118,#46119,#46120,#46121,#46122,#46123,#46124,#46125,#46126,#46127,
#46128,#46129,#46130,#46131,#46132,#46133,#46134,#46135,#46136,#46137),
(#46138,#46139,#46140,#46141,#46142,#46143,#46144,#46145,#46146,#46147,
#46148,#46149,#46150,#46151,#46152,#46153,#46154,#46155,#46156,#46157,#46158,
#46159,#46160,#46161,#46162,#46163,#46164,#46165,#46166,#46167,#46168,#46169,
#46170,#46171,#46172,#46173,#46174,#46175,#46176,#46177,#46178,#46179,#46180,
#46181,#46182,#46183,#46184,#46185,#46186,#46187,#46188,#46189,#46190,#46191,
#46192,#46193,#46194,#46195,#46196,#46197,#46198,#46199,#46200,#46201,#46202,
#46203,#46204,#46205,#46206,#46207,#46208,#46209,#46210,#46211,#46212,#46213,
#46214,#46215,#46216,#46217,#46218,#46219,#46220,#46221,#46222,#46223,#46224,
#46225,#46226,#46227,#46228,#46229,#46230,#46231,#46232,#46233,#46234,#46235,
#46236,#46237),(#46238,#46239,#46240,#46241,#46242,#46243,#46244,#46245,
#46246,#46247,#46248,#46249,#46250,#46251,#46252,#46253,#46254,#46255,#46256,
#46257,#46258,#46259,#46260,#46261,#46262,#46263,#46264,#46265,#46266,#46267,
#46268,#46269,#46270,#46271,#46272,#46273,#46274,#46275,#46276,#46277,#46278,
#46279,#46280,#46281,#46282,#46283,#46284,#46285,#46286,#46287,#46288,#46289,
#46290,#46291,#46292,#46293,#46294,#46295,#46296,#46297,#46298,#46299,#46300,
#46301,#46302,#46303,#46304,#46305,#46306,#46307,#46308,#46309,#46310,#46311,
#46312,#46313,#46314,#46315,#46316,#46317,#46318,#46319,#46320,#46321,#46322,
#46323,#46324,#46325,#46326,#46327,#46328,#46329,#46330,#46331,#46332,#46333,
#46334,#46335,#46336,#46337)),.UNSPECIFIED.,.F.,.F.,.F.,(4,4),(4,1,1,1,
1,1,1,1,1,1,1,1,1,1,1,1,1,1,1,1,1,1,1,1,1,1,1,1,1,1,1,1,1,1,1,1,1,1,1,1,
1,1,1,1,1,1,1,1,1,1,1,1,1,1,1,1,1,1,1,1,1,1,1,1,1,1,1,1,1,1,1,1,1,1,1,1,
1,1,1,1,1,1,1,1,1,1,1,1,1,1,1,1,1,1,1,1,1,4),(0.,0.064201349933887),(11.8589888623077,
12.8514087025213,13.843828542735,14.8362483829486,15.8286682231622,16.8210880633759,
17.8135079035895,18.8059277438031,19.7983475840168,20.7907674242304,21.783187264444,
22.7756071046577,23.7680269448713,24.7604467850849,25.7528666252986,26.7452864655122,
27.7377063057258,28.7301261459395,29.7225459861531,30.7149658263667,31.7073856665804,
32.699805506794,33.6922253470076,34.6846451872213,35.6770650274349,36.6694848676485,
37.6619047078622,38.6543245480758,39.6467443882894,40.6391642285031,41.6315840687167,
42.6240039089303,43.616423749144,44.6088435893576,45.6012634295713,46.5936832697849,
47.5861031099985,48.5785229502122,49.5709427904258,50.5633626306394,51.5557824708531,
52.5482023110667,53.5406221512803,54.533041991494,55.5254618317076,56.5178816719212,
57.5103015121349,58.5027213523485,59.4951411925621,60.4875610327758,61.4799808729894,
62.472400713203,63.4648205534167,64.4572403936303,65.4496602338439,66.4420800740576,
67.4344999142712,68.4269197544848,69.4193395946985,70.4117594349121,71.4041792751257,
72.3965991153394,73.389018955553,74.3814387957666,75.3738586359803,76.3662784761939,
77.3586983164075,78.3511181566212,79.3435379968348,80.3359578370484,81.3283776772621,
82.3207975174757,83.3132173576893,84.305637197903,85.2980570381166,86.2904768783302,
87.2828967185439,88.2753165587575,89.2677363989711,90.2601562391848,91.2525760793984,
92.2449959196121,93.2374157598257,94.2298356000393,95.222255440253,96.2146752804666,
97.2070951206802,98.1995149608939,99.1919348011075,100.184354641321,101.176774481535,
102.169194321748,103.161614161962,104.154034002176,105.146453842389,106.138873682603,
107.131293522817,108.12371336303),.UNSPECIFIED.);
#1325=B_SPLINE_SURFACE_WITH_KNOTS('',3,3,((#46457,#46458,#46459,#46460,
#46461,#46462,#46463,#46464,#46465,#46466,#46467,#46468,#46469,#46470,#46471,
#46472,#46473,#46474,#46475,#46476,#46477,#46478,#46479,#46480,#46481,#46482,
#46483,#46484,#46485,#46486,#46487,#46488,#46489,#46490,#46491,#46492,#46493,
#46494,#46495,#46496,#46497,#46498,#46499,#46500,#46501,#46502,#46503,#46504,
#46505,#46506,#46507,#46508,#46509,#46510,#46511,#46512,#46513,#46514,#46515,
#46516,#46517,#46518,#46519,#46520,#46521,#46522,#46523,#46524,#46525,#46526,
#46527,#46528,#46529,#46530,#46531,#46532,#46533,#46534,#46535,#46536,#46537,
#46538,#46539,#46540,#46541,#46542,#46543,#46544,#46545,#46546,#46547,#46548,
#46549,#46550,#46551,#46552,#46553,#46554,#46555,#46556),(#46557,#46558,
#46559,#46560,#46561,#46562,#46563,#46564,#46565,#46566,#46567,#46568,#46569,
#46570,#46571,#46572,#46573,#46574,#46575,#46576,#46577,#46578,#46579,#46580,
#46581,#46582,#46583,#46584,#46585,#46586,#46587,#46588,#46589,#46590,#46591,
#46592,#46593,#46594,#46595,#46596,#46597,#46598,#46599,#46600,#46601,#46602,
#46603,#46604,#46605,#46606,#46607,#46608,#46609,#46610,#46611,#46612,#46613,
#46614,#46615,#46616,#46617,#46618,#46619,#46620,#46621,#46622,#46623,#46624,
#46625,#46626,#46627,#46628,#46629,#46630,#46631,#46632,#46633,#46634,#46635,
#46636,#46637,#46638,#46639,#46640,#46641,#46642,#46643,#46644,#46645,#46646,
#46647,#46648,#46649,#46650,#46651,#46652,#46653,#46654,#46655,#46656),
(#46657,#46658,#46659,#46660,#46661,#46662,#46663,#46664,#46665,#46666,
#46667,#46668,#46669,#46670,#46671,#46672,#46673,#46674,#46675,#46676,#46677,
#46678,#46679,#46680,#46681,#46682,#46683,#46684,#46685,#46686,#46687,#46688,
#46689,#46690,#46691,#46692,#46693,#46694,#46695,#46696,#46697,#46698,#46699,
#46700,#46701,#46702,#46703,#46704,#46705,#46706,#46707,#46708,#46709,#46710,
#46711,#46712,#46713,#46714,#46715,#46716,#46717,#46718,#46719,#46720,#46721,
#46722,#46723,#46724,#46725,#46726,#46727,#46728,#46729,#46730,#46731,#46732,
#46733,#46734,#46735,#46736,#46737,#46738,#46739,#46740,#46741,#46742,#46743,
#46744,#46745,#46746,#46747,#46748,#46749,#46750,#46751,#46752,#46753,#46754,
#46755,#46756),(#46757,#46758,#46759,#46760,#46761,#46762,#46763,#46764,
#46765,#46766,#46767,#46768,#46769,#46770,#46771,#46772,#46773,#46774,#46775,
#46776,#46777,#46778,#46779,#46780,#46781,#46782,#46783,#46784,#46785,#46786,
#46787,#46788,#46789,#46790,#46791,#46792,#46793,#46794,#46795,#46796,#46797,
#46798,#46799,#46800,#46801,#46802,#46803,#46804,#46805,#46806,#46807,#46808,
#46809,#46810,#46811,#46812,#46813,#46814,#46815,#46816,#46817,#46818,#46819,
#46820,#46821,#46822,#46823,#46824,#46825,#46826,#46827,#46828,#46829,#46830,
#46831,#46832,#46833,#46834,#46835,#46836,#46837,#46838,#46839,#46840,#46841,
#46842,#46843,#46844,#46845,#46846,#46847,#46848,#46849,#46850,#46851,#46852,
#46853,#46854,#46855,#46856)),.UNSPECIFIED.,.F.,.F.,.F.,(4,4),(4,1,1,1,
1,1,1,1,1,1,1,1,1,1,1,1,1,1,1,1,1,1,1,1,1,1,1,1,1,1,1,1,1,1,1,1,1,1,1,1,
1,1,1,1,1,1,1,1,1,1,1,1,1,1,1,1,1,1,1,1,1,1,1,1,1,1,1,1,1,1,1,1,1,1,1,1,
1,1,1,1,1,1,1,1,1,1,1,1,1,1,1,1,1,1,1,1,1,4),(0.,0.064201349933887),(14.3984001269718,
15.3908199671854,16.3832398073991,17.3756596476127,18.3680794878263,19.36049932804,
20.3529191682536,21.3453390084673,22.3377588486809,23.3301786888945,24.3225985291082,
25.3150183693218,26.3074382095354,27.2998580497491,28.2922778899627,29.2846977301763,
30.27711757039,31.2695374106036,32.2619572508172,33.2543770910309,34.2467969312445,
35.2392167714581,36.2316366116718,37.2240564518854,38.216476292099,39.2088961323127,
40.2013159725263,41.1937358127399,42.1861556529536,43.1785754931672,44.1709953333808,
45.1634151735945,46.1558350138081,47.1482548540217,48.1406746942354,49.133094534449,
50.1255143746626,51.1179342148763,52.1103540550899,53.1027738953035,54.0951937355172,
55.0876135757308,56.0800334159444,57.0724532561581,58.0648730963717,59.0572929365853,
60.049712776799,61.0421326170126,62.0345524572262,63.0269722974399,64.0193921376535,
65.0118119778672,66.0042318180808,66.9966516582944,67.9890714985081,68.9814913387217,
69.9739111789353,70.966331019149,71.9587508593626,72.9511706995762,73.9435905397899,
74.9360103800035,75.9284302202171,76.9208500604308,77.9132699006444,78.905689740858,
79.8981095810717,80.8905294212853,81.8829492614989,82.8753691017126,83.8677889419262,
84.8602087821398,85.8526286223535,86.8450484625671,87.8374683027807,88.8298881429944,
89.822307983208,90.8147278234216,91.8071476636353,92.7995675038489,93.7919873440625,
94.7844071842762,95.7768270244898,96.7692468647034,97.7616667049171,98.7540865451307,
99.7465063853443,100.738926225558,101.731346065772,102.723765905985,103.716185746199,
104.708605586413,105.701025426626,106.69344526684,107.685865107053,108.678284947267,
109.670704787481,110.663124627694),.UNSPECIFIED.);
#1326=B_SPLINE_SURFACE_WITH_KNOTS('',3,3,((#47185,#47186,#47187,#47188,
#47189,#47190,#47191,#47192,#47193,#47194,#47195,#47196,#47197,#47198,#47199,
#47200,#47201,#47202,#47203,#47204,#47205,#47206,#47207,#47208,#47209,#47210,
#47211,#47212,#47213,#47214,#47215,#47216,#47217,#47218,#47219,#47220,#47221,
#47222,#47223,#47224,#47225,#47226,#47227,#47228,#47229,#47230,#47231,#47232,
#47233,#47234,#47235,#47236,#47237,#47238,#47239,#47240,#47241,#47242,#47243,
#47244,#47245,#47246,#47247,#47248,#47249,#47250,#47251,#47252,#47253,#47254,
#47255,#47256,#47257,#47258,#47259,#47260,#47261,#47262,#47263,#47264,#47265,
#47266,#47267,#47268,#47269,#47270,#47271,#47272,#47273,#47274,#47275,#47276,
#47277,#47278,#47279,#47280,#47281,#47282,#47283,#47284),(#47285,#47286,
#47287,#47288,#47289,#47290,#47291,#47292,#47293,#47294,#47295,#47296,#47297,
#47298,#47299,#47300,#47301,#47302,#47303,#47304,#47305,#47306,#47307,#47308,
#47309,#47310,#47311,#47312,#47313,#47314,#47315,#47316,#47317,#47318,#47319,
#47320,#47321,#47322,#47323,#47324,#47325,#47326,#47327,#47328,#47329,#47330,
#47331,#47332,#47333,#47334,#47335,#47336,#47337,#47338,#47339,#47340,#47341,
#47342,#47343,#47344,#47345,#47346,#47347,#47348,#47349,#47350,#47351,#47352,
#47353,#47354,#47355,#47356,#47357,#47358,#47359,#47360,#47361,#47362,#47363,
#47364,#47365,#47366,#47367,#47368,#47369,#47370,#47371,#47372,#47373,#47374,
#47375,#47376,#47377,#47378,#47379,#47380,#47381,#47382,#47383,#47384),
(#47385,#47386,#47387,#47388,#47389,#47390,#47391,#47392,#47393,#47394,
#47395,#47396,#47397,#47398,#47399,#47400,#47401,#47402,#47403,#47404,#47405,
#47406,#47407,#47408,#47409,#47410,#47411,#47412,#47413,#47414,#47415,#47416,
#47417,#47418,#47419,#47420,#47421,#47422,#47423,#47424,#47425,#47426,#47427,
#47428,#47429,#47430,#47431,#47432,#47433,#47434,#47435,#47436,#47437,#47438,
#47439,#47440,#47441,#47442,#47443,#47444,#47445,#47446,#47447,#47448,#47449,
#47450,#47451,#47452,#47453,#47454,#47455,#47456,#47457,#47458,#47459,#47460,
#47461,#47462,#47463,#47464,#47465,#47466,#47467,#47468,#47469,#47470,#47471,
#47472,#47473,#47474,#47475,#47476,#47477,#47478,#47479,#47480,#47481,#47482,
#47483,#47484),(#47485,#47486,#47487,#47488,#47489,#47490,#47491,#47492,
#47493,#47494,#47495,#47496,#47497,#47498,#47499,#47500,#47501,#47502,#47503,
#47504,#47505,#47506,#47507,#47508,#47509,#47510,#47511,#47512,#47513,#47514,
#47515,#47516,#47517,#47518,#47519,#47520,#47521,#47522,#47523,#47524,#47525,
#47526,#47527,#47528,#47529,#47530,#47531,#47532,#47533,#47534,#47535,#47536,
#47537,#47538,#47539,#47540,#47541,#47542,#47543,#47544,#47545,#47546,#47547,
#47548,#47549,#47550,#47551,#47552,#47553,#47554,#47555,#47556,#47557,#47558,
#47559,#47560,#47561,#47562,#47563,#47564,#47565,#47566,#47567,#47568,#47569,
#47570,#47571,#47572,#47573,#47574,#47575,#47576,#47577,#47578,#47579,#47580,
#47581,#47582,#47583,#47584)),.UNSPECIFIED.,.F.,.F.,.F.,(4,4),(4,1,1,1,
1,1,1,1,1,1,1,1,1,1,1,1,1,1,1,1,1,1,1,1,1,1,1,1,1,1,1,1,1,1,1,1,1,1,1,1,
1,1,1,1,1,1,1,1,1,1,1,1,1,1,1,1,1,1,1,1,1,1,1,1,1,1,1,1,1,1,1,1,1,1,1,1,
1,1,1,1,1,1,1,1,1,1,1,1,1,1,1,1,1,1,1,1,1,4),(0.,0.064201349933887),(11.8589888623078,
12.8514087025215,13.8438285427351,14.8362483829487,15.8286682231624,16.821088063376,
17.8135079035896,18.8059277438032,19.7983475840169,20.7907674242305,21.7831872644441,
22.7756071046578,23.7680269448714,24.760446785085,25.7528666252987,26.7452864655123,
27.7377063057259,28.7301261459396,29.7225459861532,30.7149658263668,31.7073856665805,
32.6998055067941,33.6922253470077,34.6846451872214,35.677065027435,36.6694848676486,
37.6619047078623,38.6543245480759,39.6467443882895,40.6391642285032,41.6315840687168,
42.6240039089304,43.6164237491441,44.6088435893577,45.6012634295713,46.593683269785,
47.5861031099986,48.5785229502122,49.5709427904259,50.5633626306395,51.5557824708531,
52.5482023110668,53.5406221512804,54.533041991494,55.5254618317077,56.5178816719213,
57.5103015121349,58.5027213523486,59.4951411925622,60.4875610327758,61.4799808729895,
62.4724007132031,63.4648205534167,64.4572403936303,65.449660233844,66.4420800740576,
67.4344999142712,68.4269197544849,69.4193395946985,70.4117594349121,71.4041792751258,
72.3965991153394,73.389018955553,74.3814387957667,75.3738586359803,76.3662784761939,
77.3586983164076,78.3511181566212,79.3435379968348,80.3359578370485,81.3283776772621,
82.3207975174757,83.3132173576894,84.305637197903,85.2980570381166,86.2904768783303,
87.2828967185439,88.2753165587575,89.2677363989712,90.2601562391848,91.2525760793984,
92.2449959196121,93.2374157598257,94.2298356000393,95.222255440253,96.2146752804666,
97.2070951206802,98.1995149608939,99.1919348011075,100.184354641321,101.176774481535,
102.169194321748,103.161614161962,104.154034002176,105.146453842389,106.138873682603,
107.131293522817,108.12371336303),.UNSPECIFIED.);
#1327=B_SPLINE_SURFACE_WITH_KNOTS('',3,3,((#47704,#47705,#47706,#47707,
#47708,#47709,#47710,#47711,#47712,#47713,#47714,#47715,#47716,#47717,#47718,
#47719,#47720,#47721,#47722,#47723,#47724,#47725,#47726,#47727,#47728,#47729,
#47730,#47731,#47732,#47733,#47734,#47735,#47736,#47737,#47738,#47739,#47740,
#47741,#47742,#47743,#47744,#47745,#47746,#47747,#47748,#47749,#47750,#47751,
#47752,#47753,#47754,#47755,#47756,#47757,#47758,#47759,#47760,#47761,#47762,
#47763,#47764,#47765,#47766,#47767,#47768,#47769,#47770,#47771,#47772,#47773,
#47774,#47775,#47776,#47777,#47778,#47779,#47780,#47781,#47782,#47783,#47784,
#47785,#47786,#47787,#47788,#47789,#47790,#47791,#47792,#47793,#47794,#47795,
#47796,#47797,#47798,#47799,#47800,#47801,#47802,#47803),(#47804,#47805,
#47806,#47807,#47808,#47809,#47810,#47811,#47812,#47813,#47814,#47815,#47816,
#47817,#47818,#47819,#47820,#47821,#47822,#47823,#47824,#47825,#47826,#47827,
#47828,#47829,#47830,#47831,#47832,#47833,#47834,#47835,#47836,#47837,#47838,
#47839,#47840,#47841,#47842,#47843,#47844,#47845,#47846,#47847,#47848,#47849,
#47850,#47851,#47852,#47853,#47854,#47855,#47856,#47857,#47858,#47859,#47860,
#47861,#47862,#47863,#47864,#47865,#47866,#47867,#47868,#47869,#47870,#47871,
#47872,#47873,#47874,#47875,#47876,#47877,#47878,#47879,#47880,#47881,#47882,
#47883,#47884,#47885,#47886,#47887,#47888,#47889,#47890,#47891,#47892,#47893,
#47894,#47895,#47896,#47897,#47898,#47899,#47900,#47901,#47902,#47903),
(#47904,#47905,#47906,#47907,#47908,#47909,#47910,#47911,#47912,#47913,
#47914,#47915,#47916,#47917,#47918,#47919,#47920,#47921,#47922,#47923,#47924,
#47925,#47926,#47927,#47928,#47929,#47930,#47931,#47932,#47933,#47934,#47935,
#47936,#47937,#47938,#47939,#47940,#47941,#47942,#47943,#47944,#47945,#47946,
#47947,#47948,#47949,#47950,#47951,#47952,#47953,#47954,#47955,#47956,#47957,
#47958,#47959,#47960,#47961,#47962,#47963,#47964,#47965,#47966,#47967,#47968,
#47969,#47970,#47971,#47972,#47973,#47974,#47975,#47976,#47977,#47978,#47979,
#47980,#47981,#47982,#47983,#47984,#47985,#47986,#47987,#47988,#47989,#47990,
#47991,#47992,#47993,#47994,#47995,#47996,#47997,#47998,#47999,#48000,#48001,
#48002,#48003),(#48004,#48005,#48006,#48007,#48008,#48009,#48010,#48011,
#48012,#48013,#48014,#48015,#48016,#48017,#48018,#48019,#48020,#48021,#48022,
#48023,#48024,#48025,#48026,#48027,#48028,#48029,#48030,#48031,#48032,#48033,
#48034,#48035,#48036,#48037,#48038,#48039,#48040,#48041,#48042,#48043,#48044,
#48045,#48046,#48047,#48048,#48049,#48050,#48051,#48052,#48053,#48054,#48055,
#48056,#48057,#48058,#48059,#48060,#48061,#48062,#48063,#48064,#48065,#48066,
#48067,#48068,#48069,#48070,#48071,#48072,#48073,#48074,#48075,#48076,#48077,
#48078,#48079,#48080,#48081,#48082,#48083,#48084,#48085,#48086,#48087,#48088,
#48089,#48090,#48091,#48092,#48093,#48094,#48095,#48096,#48097,#48098,#48099,
#48100,#48101,#48102,#48103)),.UNSPECIFIED.,.F.,.F.,.F.,(4,4),(4,1,1,1,
1,1,1,1,1,1,1,1,1,1,1,1,1,1,1,1,1,1,1,1,1,1,1,1,1,1,1,1,1,1,1,1,1,1,1,1,
1,1,1,1,1,1,1,1,1,1,1,1,1,1,1,1,1,1,1,1,1,1,1,1,1,1,1,1,1,1,1,1,1,1,1,1,
1,1,1,1,1,1,1,1,1,1,1,1,1,1,1,1,1,1,1,1,1,4),(0.,0.064201349933887),(14.3984001269719,
15.3908199671856,16.3832398073992,17.3756596476128,18.3680794878265,19.3604993280401,
20.3529191682537,21.3453390084674,22.337758848681,23.3301786888946,24.3225985291083,
25.3150183693219,26.3074382095355,27.2998580497492,28.2922778899628,29.2846977301764,
30.2771175703901,31.2695374106037,32.2619572508173,33.2543770910309,34.2467969312446,
35.2392167714582,36.2316366116718,37.2240564518855,38.2164762920991,39.2088961323127,
40.2013159725264,41.19373581274,42.1861556529536,43.1785754931673,44.1709953333809,
45.1634151735945,46.1558350138082,47.1482548540218,48.1406746942354,49.1330945344491,
50.1255143746627,51.1179342148763,52.11035405509,53.1027738953036,54.0951937355172,
55.0876135757309,56.0800334159445,57.0724532561581,58.0648730963718,59.0572929365854,
60.049712776799,61.0421326170127,62.0345524572263,63.0269722974399,64.0193921376536,
65.0118119778672,66.0042318180808,66.9966516582945,67.9890714985081,68.9814913387217,
69.9739111789354,70.966331019149,71.9587508593626,72.9511706995763,73.9435905397899,
74.9360103800035,75.9284302202172,76.9208500604308,77.9132699006444,78.9056897408581,
79.8981095810717,80.8905294212853,81.882949261499,82.8753691017126,83.8677889419262,
84.8602087821399,85.8526286223535,86.8450484625671,87.8374683027808,88.8298881429944,
89.822307983208,90.8147278234217,91.8071476636353,92.7995675038489,93.7919873440626,
94.7844071842762,95.7768270244898,96.7692468647035,97.7616667049171,98.7540865451307,
99.7465063853444,100.738926225558,101.731346065772,102.723765905985,103.716185746199,
104.708605586413,105.701025426626,106.69344526684,107.685865107053,108.678284947267,
109.670704787481,110.663124627694),.UNSPECIFIED.);
#1328=B_SPLINE_SURFACE_WITH_KNOTS('',3,3,((#48432,#48433,#48434,#48435,
#48436,#48437,#48438,#48439,#48440,#48441,#48442,#48443,#48444,#48445,#48446,
#48447,#48448,#48449,#48450,#48451,#48452,#48453,#48454,#48455,#48456,#48457,
#48458,#48459,#48460,#48461,#48462,#48463,#48464,#48465,#48466,#48467,#48468,
#48469,#48470,#48471,#48472,#48473,#48474,#48475,#48476,#48477,#48478,#48479,
#48480,#48481,#48482,#48483,#48484,#48485,#48486,#48487,#48488,#48489,#48490,
#48491,#48492,#48493,#48494,#48495,#48496,#48497,#48498,#48499,#48500,#48501,
#48502,#48503,#48504,#48505,#48506,#48507,#48508,#48509,#48510,#48511,#48512,
#48513,#48514,#48515,#48516,#48517,#48518,#48519,#48520,#48521,#48522,#48523,
#48524,#48525,#48526,#48527,#48528,#48529,#48530,#48531),(#48532,#48533,
#48534,#48535,#48536,#48537,#48538,#48539,#48540,#48541,#48542,#48543,#48544,
#48545,#48546,#48547,#48548,#48549,#48550,#48551,#48552,#48553,#48554,#48555,
#48556,#48557,#48558,#48559,#48560,#48561,#48562,#48563,#48564,#48565,#48566,
#48567,#48568,#48569,#48570,#48571,#48572,#48573,#48574,#48575,#48576,#48577,
#48578,#48579,#48580,#48581,#48582,#48583,#48584,#48585,#48586,#48587,#48588,
#48589,#48590,#48591,#48592,#48593,#48594,#48595,#48596,#48597,#48598,#48599,
#48600,#48601,#48602,#48603,#48604,#48605,#48606,#48607,#48608,#48609,#48610,
#48611,#48612,#48613,#48614,#48615,#48616,#48617,#48618,#48619,#48620,#48621,
#48622,#48623,#48624,#48625,#48626,#48627,#48628,#48629,#48630,#48631),
(#48632,#48633,#48634,#48635,#48636,#48637,#48638,#48639,#48640,#48641,
#48642,#48643,#48644,#48645,#48646,#48647,#48648,#48649,#48650,#48651,#48652,
#48653,#48654,#48655,#48656,#48657,#48658,#48659,#48660,#48661,#48662,#48663,
#48664,#48665,#48666,#48667,#48668,#48669,#48670,#48671,#48672,#48673,#48674,
#48675,#48676,#48677,#48678,#48679,#48680,#48681,#48682,#48683,#48684,#48685,
#48686,#48687,#48688,#48689,#48690,#48691,#48692,#48693,#48694,#48695,#48696,
#48697,#48698,#48699,#48700,#48701,#48702,#48703,#48704,#48705,#48706,#48707,
#48708,#48709,#48710,#48711,#48712,#48713,#48714,#48715,#48716,#48717,#48718,
#48719,#48720,#48721,#48722,#48723,#48724,#48725,#48726,#48727,#48728,#48729,
#48730,#48731),(#48732,#48733,#48734,#48735,#48736,#48737,#48738,#48739,
#48740,#48741,#48742,#48743,#48744,#48745,#48746,#48747,#48748,#48749,#48750,
#48751,#48752,#48753,#48754,#48755,#48756,#48757,#48758,#48759,#48760,#48761,
#48762,#48763,#48764,#48765,#48766,#48767,#48768,#48769,#48770,#48771,#48772,
#48773,#48774,#48775,#48776,#48777,#48778,#48779,#48780,#48781,#48782,#48783,
#48784,#48785,#48786,#48787,#48788,#48789,#48790,#48791,#48792,#48793,#48794,
#48795,#48796,#48797,#48798,#48799,#48800,#48801,#48802,#48803,#48804,#48805,
#48806,#48807,#48808,#48809,#48810,#48811,#48812,#48813,#48814,#48815,#48816,
#48817,#48818,#48819,#48820,#48821,#48822,#48823,#48824,#48825,#48826,#48827,
#48828,#48829,#48830,#48831)),.UNSPECIFIED.,.F.,.F.,.F.,(4,4),(4,1,1,1,
1,1,1,1,1,1,1,1,1,1,1,1,1,1,1,1,1,1,1,1,1,1,1,1,1,1,1,1,1,1,1,1,1,1,1,1,
1,1,1,1,1,1,1,1,1,1,1,1,1,1,1,1,1,1,1,1,1,1,1,1,1,1,1,1,1,1,1,1,1,1,1,1,
1,1,1,1,1,1,1,1,1,1,1,1,1,1,1,1,1,1,1,1,1,4),(0.,0.064201349933887),(11.8589888623077,
12.8514087025213,13.843828542735,14.8362483829486,15.8286682231622,16.8210880633759,
17.8135079035895,18.8059277438031,19.7983475840168,20.7907674242304,21.783187264444,
22.7756071046577,23.7680269448713,24.7604467850849,25.7528666252986,26.7452864655122,
27.7377063057258,28.7301261459395,29.7225459861531,30.7149658263668,31.7073856665804,
32.699805506794,33.6922253470076,34.6846451872213,35.6770650274349,36.6694848676485,
37.6619047078622,38.6543245480758,39.6467443882895,40.6391642285031,41.6315840687167,
42.6240039089304,43.616423749144,44.6088435893576,45.6012634295713,46.5936832697849,
47.5861031099985,48.5785229502122,49.5709427904258,50.5633626306394,51.5557824708531,
52.5482023110667,53.5406221512803,54.533041991494,55.5254618317076,56.5178816719212,
57.5103015121349,58.5027213523485,59.4951411925621,60.4875610327758,61.4799808729894,
62.472400713203,63.4648205534167,64.4572403936303,65.4496602338439,66.4420800740576,
67.4344999142712,68.4269197544848,69.4193395946985,70.4117594349121,71.4041792751257,
72.3965991153394,73.389018955553,74.3814387957666,75.3738586359803,76.3662784761939,
77.3586983164075,78.3511181566212,79.3435379968348,80.3359578370484,81.3283776772621,
82.3207975174757,83.3132173576894,84.305637197903,85.2980570381166,86.2904768783303,
87.2828967185439,88.2753165587575,89.2677363989712,90.2601562391848,91.2525760793984,
92.2449959196121,93.2374157598257,94.2298356000393,95.222255440253,96.2146752804666,
97.2070951206802,98.1995149608939,99.1919348011075,100.184354641321,101.176774481535,
102.169194321748,103.161614161962,104.154034002176,105.146453842389,106.138873682603,
107.131293522817,108.12371336303),.UNSPECIFIED.);
#1329=B_SPLINE_SURFACE_WITH_KNOTS('',3,3,((#48951,#48952,#48953,#48954,
#48955,#48956,#48957,#48958,#48959,#48960,#48961,#48962,#48963,#48964,#48965,
#48966,#48967,#48968,#48969,#48970,#48971,#48972,#48973,#48974,#48975,#48976,
#48977,#48978,#48979,#48980,#48981,#48982,#48983,#48984,#48985,#48986,#48987,
#48988,#48989,#48990,#48991,#48992,#48993,#48994,#48995,#48996,#48997,#48998,
#48999,#49000,#49001,#49002,#49003,#49004,#49005,#49006,#49007,#49008,#49009,
#49010,#49011,#49012,#49013,#49014,#49015,#49016,#49017,#49018,#49019,#49020,
#49021,#49022,#49023,#49024,#49025,#49026,#49027,#49028,#49029,#49030,#49031,
#49032,#49033,#49034,#49035,#49036,#49037,#49038,#49039,#49040,#49041,#49042,
#49043,#49044,#49045,#49046,#49047,#49048,#49049,#49050),(#49051,#49052,
#49053,#49054,#49055,#49056,#49057,#49058,#49059,#49060,#49061,#49062,#49063,
#49064,#49065,#49066,#49067,#49068,#49069,#49070,#49071,#49072,#49073,#49074,
#49075,#49076,#49077,#49078,#49079,#49080,#49081,#49082,#49083,#49084,#49085,
#49086,#49087,#49088,#49089,#49090,#49091,#49092,#49093,#49094,#49095,#49096,
#49097,#49098,#49099,#49100,#49101,#49102,#49103,#49104,#49105,#49106,#49107,
#49108,#49109,#49110,#49111,#49112,#49113,#49114,#49115,#49116,#49117,#49118,
#49119,#49120,#49121,#49122,#49123,#49124,#49125,#49126,#49127,#49128,#49129,
#49130,#49131,#49132,#49133,#49134,#49135,#49136,#49137,#49138,#49139,#49140,
#49141,#49142,#49143,#49144,#49145,#49146,#49147,#49148,#49149,#49150),
(#49151,#49152,#49153,#49154,#49155,#49156,#49157,#49158,#49159,#49160,
#49161,#49162,#49163,#49164,#49165,#49166,#49167,#49168,#49169,#49170,#49171,
#49172,#49173,#49174,#49175,#49176,#49177,#49178,#49179,#49180,#49181,#49182,
#49183,#49184,#49185,#49186,#49187,#49188,#49189,#49190,#49191,#49192,#49193,
#49194,#49195,#49196,#49197,#49198,#49199,#49200,#49201,#49202,#49203,#49204,
#49205,#49206,#49207,#49208,#49209,#49210,#49211,#49212,#49213,#49214,#49215,
#49216,#49217,#49218,#49219,#49220,#49221,#49222,#49223,#49224,#49225,#49226,
#49227,#49228,#49229,#49230,#49231,#49232,#49233,#49234,#49235,#49236,#49237,
#49238,#49239,#49240,#49241,#49242,#49243,#49244,#49245,#49246,#49247,#49248,
#49249,#49250),(#49251,#49252,#49253,#49254,#49255,#49256,#49257,#49258,
#49259,#49260,#49261,#49262,#49263,#49264,#49265,#49266,#49267,#49268,#49269,
#49270,#49271,#49272,#49273,#49274,#49275,#49276,#49277,#49278,#49279,#49280,
#49281,#49282,#49283,#49284,#49285,#49286,#49287,#49288,#49289,#49290,#49291,
#49292,#49293,#49294,#49295,#49296,#49297,#49298,#49299,#49300,#49301,#49302,
#49303,#49304,#49305,#49306,#49307,#49308,#49309,#49310,#49311,#49312,#49313,
#49314,#49315,#49316,#49317,#49318,#49319,#49320,#49321,#49322,#49323,#49324,
#49325,#49326,#49327,#49328,#49329,#49330,#49331,#49332,#49333,#49334,#49335,
#49336,#49337,#49338,#49339,#49340,#49341,#49342,#49343,#49344,#49345,#49346,
#49347,#49348,#49349,#49350)),.UNSPECIFIED.,.F.,.F.,.F.,(4,4),(4,1,1,1,
1,1,1,1,1,1,1,1,1,1,1,1,1,1,1,1,1,1,1,1,1,1,1,1,1,1,1,1,1,1,1,1,1,1,1,1,
1,1,1,1,1,1,1,1,1,1,1,1,1,1,1,1,1,1,1,1,1,1,1,1,1,1,1,1,1,1,1,1,1,1,1,1,
1,1,1,1,1,1,1,1,1,1,1,1,1,1,1,1,1,1,1,1,1,4),(0.,0.064201349933887),(14.3984001269718,
15.3908199671854,16.3832398073991,17.3756596476127,18.3680794878263,19.36049932804,
20.3529191682536,21.3453390084673,22.3377588486809,23.3301786888945,24.3225985291082,
25.3150183693218,26.3074382095354,27.2998580497491,28.2922778899627,29.2846977301763,
30.27711757039,31.2695374106036,32.2619572508172,33.2543770910309,34.2467969312445,
35.2392167714581,36.2316366116718,37.2240564518854,38.216476292099,39.2088961323127,
40.2013159725263,41.1937358127399,42.1861556529536,43.1785754931672,44.1709953333808,
45.1634151735945,46.1558350138081,47.1482548540217,48.1406746942354,49.133094534449,
50.1255143746626,51.1179342148763,52.1103540550899,53.1027738953035,54.0951937355172,
55.0876135757308,56.0800334159444,57.0724532561581,58.0648730963717,59.0572929365853,
60.049712776799,61.0421326170126,62.0345524572262,63.0269722974399,64.0193921376535,
65.0118119778672,66.0042318180808,66.9966516582944,67.9890714985081,68.9814913387217,
69.9739111789353,70.966331019149,71.9587508593626,72.9511706995762,73.9435905397899,
74.9360103800035,75.9284302202171,76.9208500604308,77.9132699006444,78.905689740858,
79.8981095810717,80.8905294212853,81.8829492614989,82.8753691017126,83.8677889419262,
84.8602087821398,85.8526286223535,86.8450484625671,87.8374683027807,88.8298881429944,
89.822307983208,90.8147278234216,91.8071476636353,92.7995675038489,93.7919873440625,
94.7844071842762,95.7768270244898,96.7692468647034,97.7616667049171,98.7540865451307,
99.7465063853443,100.738926225558,101.731346065772,102.723765905985,103.716185746199,
104.708605586413,105.701025426626,106.69344526684,107.685865107053,108.678284947267,
109.670704787481,110.663124627694),.UNSPECIFIED.);
#1330=B_SPLINE_SURFACE_WITH_KNOTS('',3,3,((#49679,#49680,#49681,#49682,
#49683,#49684,#49685,#49686,#49687,#49688,#49689,#49690,#49691,#49692,#49693,
#49694,#49695,#49696,#49697,#49698,#49699,#49700,#49701,#49702,#49703,#49704,
#49705,#49706,#49707,#49708,#49709,#49710,#49711,#49712,#49713,#49714,#49715,
#49716,#49717,#49718,#49719,#49720,#49721,#49722,#49723,#49724,#49725,#49726,
#49727,#49728,#49729,#49730,#49731,#49732,#49733,#49734,#49735,#49736,#49737,
#49738,#49739,#49740,#49741,#49742,#49743,#49744,#49745,#49746,#49747,#49748,
#49749,#49750,#49751,#49752,#49753,#49754,#49755,#49756,#49757,#49758,#49759,
#49760,#49761,#49762,#49763,#49764,#49765,#49766,#49767,#49768,#49769,#49770,
#49771,#49772,#49773,#49774,#49775,#49776,#49777,#49778),(#49779,#49780,
#49781,#49782,#49783,#49784,#49785,#49786,#49787,#49788,#49789,#49790,#49791,
#49792,#49793,#49794,#49795,#49796,#49797,#49798,#49799,#49800,#49801,#49802,
#49803,#49804,#49805,#49806,#49807,#49808,#49809,#49810,#49811,#49812,#49813,
#49814,#49815,#49816,#49817,#49818,#49819,#49820,#49821,#49822,#49823,#49824,
#49825,#49826,#49827,#49828,#49829,#49830,#49831,#49832,#49833,#49834,#49835,
#49836,#49837,#49838,#49839,#49840,#49841,#49842,#49843,#49844,#49845,#49846,
#49847,#49848,#49849,#49850,#49851,#49852,#49853,#49854,#49855,#49856,#49857,
#49858,#49859,#49860,#49861,#49862,#49863,#49864,#49865,#49866,#49867,#49868,
#49869,#49870,#49871,#49872,#49873,#49874,#49875,#49876,#49877,#49878),
(#49879,#49880,#49881,#49882,#49883,#49884,#49885,#49886,#49887,#49888,
#49889,#49890,#49891,#49892,#49893,#49894,#49895,#49896,#49897,#49898,#49899,
#49900,#49901,#49902,#49903,#49904,#49905,#49906,#49907,#49908,#49909,#49910,
#49911,#49912,#49913,#49914,#49915,#49916,#49917,#49918,#49919,#49920,#49921,
#49922,#49923,#49924,#49925,#49926,#49927,#49928,#49929,#49930,#49931,#49932,
#49933,#49934,#49935,#49936,#49937,#49938,#49939,#49940,#49941,#49942,#49943,
#49944,#49945,#49946,#49947,#49948,#49949,#49950,#49951,#49952,#49953,#49954,
#49955,#49956,#49957,#49958,#49959,#49960,#49961,#49962,#49963,#49964,#49965,
#49966,#49967,#49968,#49969,#49970,#49971,#49972,#49973,#49974,#49975,#49976,
#49977,#49978),(#49979,#49980,#49981,#49982,#49983,#49984,#49985,#49986,
#49987,#49988,#49989,#49990,#49991,#49992,#49993,#49994,#49995,#49996,#49997,
#49998,#49999,#50000,#50001,#50002,#50003,#50004,#50005,#50006,#50007,#50008,
#50009,#50010,#50011,#50012,#50013,#50014,#50015,#50016,#50017,#50018,#50019,
#50020,#50021,#50022,#50023,#50024,#50025,#50026,#50027,#50028,#50029,#50030,
#50031,#50032,#50033,#50034,#50035,#50036,#50037,#50038,#50039,#50040,#50041,
#50042,#50043,#50044,#50045,#50046,#50047,#50048,#50049,#50050,#50051,#50052,
#50053,#50054,#50055,#50056,#50057,#50058,#50059,#50060,#50061,#50062,#50063,
#50064,#50065,#50066,#50067,#50068,#50069,#50070,#50071,#50072,#50073,#50074,
#50075,#50076,#50077,#50078)),.UNSPECIFIED.,.F.,.F.,.F.,(4,4),(4,1,1,1,
1,1,1,1,1,1,1,1,1,1,1,1,1,1,1,1,1,1,1,1,1,1,1,1,1,1,1,1,1,1,1,1,1,1,1,1,
1,1,1,1,1,1,1,1,1,1,1,1,1,1,1,1,1,1,1,1,1,1,1,1,1,1,1,1,1,1,1,1,1,1,1,1,
1,1,1,1,1,1,1,1,1,1,1,1,1,1,1,1,1,1,1,1,1,4),(0.,0.064201349933887),(11.8589888623078,
12.8514087025215,13.8438285427351,14.8362483829487,15.8286682231624,16.821088063376,
17.8135079035896,18.8059277438032,19.7983475840169,20.7907674242305,21.7831872644441,
22.7756071046578,23.7680269448714,24.760446785085,25.7528666252987,26.7452864655123,
27.7377063057259,28.7301261459396,29.7225459861532,30.7149658263668,31.7073856665805,
32.6998055067941,33.6922253470077,34.6846451872214,35.677065027435,36.6694848676486,
37.6619047078623,38.6543245480759,39.6467443882895,40.6391642285032,41.6315840687168,
42.6240039089304,43.6164237491441,44.6088435893577,45.6012634295713,46.593683269785,
47.5861031099986,48.5785229502122,49.5709427904259,50.5633626306395,51.5557824708531,
52.5482023110668,53.5406221512804,54.533041991494,55.5254618317077,56.5178816719213,
57.5103015121349,58.5027213523486,59.4951411925622,60.4875610327758,61.4799808729895,
62.4724007132031,63.4648205534167,64.4572403936303,65.449660233844,66.4420800740576,
67.4344999142712,68.4269197544849,69.4193395946985,70.4117594349121,71.4041792751258,
72.3965991153394,73.389018955553,74.3814387957667,75.3738586359803,76.3662784761939,
77.3586983164076,78.3511181566212,79.3435379968348,80.3359578370485,81.3283776772621,
82.3207975174757,83.3132173576894,84.305637197903,85.2980570381166,86.2904768783303,
87.2828967185439,88.2753165587575,89.2677363989712,90.2601562391848,91.2525760793984,
92.2449959196121,93.2374157598257,94.2298356000393,95.222255440253,96.2146752804666,
97.2070951206802,98.1995149608939,99.1919348011075,100.184354641321,101.176774481535,
102.169194321748,103.161614161962,104.154034002176,105.146453842389,106.138873682603,
107.131293522817,108.12371336303),.UNSPECIFIED.);
#1331=B_SPLINE_SURFACE_WITH_KNOTS('',3,3,((#50198,#50199,#50200,#50201,
#50202,#50203,#50204,#50205,#50206,#50207,#50208,#50209,#50210,#50211,#50212,
#50213,#50214,#50215,#50216,#50217,#50218,#50219,#50220,#50221,#50222,#50223,
#50224,#50225,#50226,#50227,#50228,#50229,#50230,#50231,#50232,#50233,#50234,
#50235,#50236,#50237,#50238,#50239,#50240,#50241,#50242,#50243,#50244,#50245,
#50246,#50247,#50248,#50249,#50250,#50251,#50252,#50253,#50254,#50255,#50256,
#50257,#50258,#50259,#50260,#50261,#50262,#50263,#50264,#50265,#50266,#50267,
#50268,#50269,#50270,#50271,#50272,#50273,#50274,#50275,#50276,#50277,#50278,
#50279,#50280,#50281,#50282,#50283,#50284,#50285,#50286,#50287,#50288,#50289,
#50290,#50291,#50292,#50293,#50294,#50295,#50296,#50297),(#50298,#50299,
#50300,#50301,#50302,#50303,#50304,#50305,#50306,#50307,#50308,#50309,#50310,
#50311,#50312,#50313,#50314,#50315,#50316,#50317,#50318,#50319,#50320,#50321,
#50322,#50323,#50324,#50325,#50326,#50327,#50328,#50329,#50330,#50331,#50332,
#50333,#50334,#50335,#50336,#50337,#50338,#50339,#50340,#50341,#50342,#50343,
#50344,#50345,#50346,#50347,#50348,#50349,#50350,#50351,#50352,#50353,#50354,
#50355,#50356,#50357,#50358,#50359,#50360,#50361,#50362,#50363,#50364,#50365,
#50366,#50367,#50368,#50369,#50370,#50371,#50372,#50373,#50374,#50375,#50376,
#50377,#50378,#50379,#50380,#50381,#50382,#50383,#50384,#50385,#50386,#50387,
#50388,#50389,#50390,#50391,#50392,#50393,#50394,#50395,#50396,#50397),
(#50398,#50399,#50400,#50401,#50402,#50403,#50404,#50405,#50406,#50407,
#50408,#50409,#50410,#50411,#50412,#50413,#50414,#50415,#50416,#50417,#50418,
#50419,#50420,#50421,#50422,#50423,#50424,#50425,#50426,#50427,#50428,#50429,
#50430,#50431,#50432,#50433,#50434,#50435,#50436,#50437,#50438,#50439,#50440,
#50441,#50442,#50443,#50444,#50445,#50446,#50447,#50448,#50449,#50450,#50451,
#50452,#50453,#50454,#50455,#50456,#50457,#50458,#50459,#50460,#50461,#50462,
#50463,#50464,#50465,#50466,#50467,#50468,#50469,#50470,#50471,#50472,#50473,
#50474,#50475,#50476,#50477,#50478,#50479,#50480,#50481,#50482,#50483,#50484,
#50485,#50486,#50487,#50488,#50489,#50490,#50491,#50492,#50493,#50494,#50495,
#50496,#50497),(#50498,#50499,#50500,#50501,#50502,#50503,#50504,#50505,
#50506,#50507,#50508,#50509,#50510,#50511,#50512,#50513,#50514,#50515,#50516,
#50517,#50518,#50519,#50520,#50521,#50522,#50523,#50524,#50525,#50526,#50527,
#50528,#50529,#50530,#50531,#50532,#50533,#50534,#50535,#50536,#50537,#50538,
#50539,#50540,#50541,#50542,#50543,#50544,#50545,#50546,#50547,#50548,#50549,
#50550,#50551,#50552,#50553,#50554,#50555,#50556,#50557,#50558,#50559,#50560,
#50561,#50562,#50563,#50564,#50565,#50566,#50567,#50568,#50569,#50570,#50571,
#50572,#50573,#50574,#50575,#50576,#50577,#50578,#50579,#50580,#50581,#50582,
#50583,#50584,#50585,#50586,#50587,#50588,#50589,#50590,#50591,#50592,#50593,
#50594,#50595,#50596,#50597)),.UNSPECIFIED.,.F.,.F.,.F.,(4,4),(4,1,1,1,
1,1,1,1,1,1,1,1,1,1,1,1,1,1,1,1,1,1,1,1,1,1,1,1,1,1,1,1,1,1,1,1,1,1,1,1,
1,1,1,1,1,1,1,1,1,1,1,1,1,1,1,1,1,1,1,1,1,1,1,1,1,1,1,1,1,1,1,1,1,1,1,1,
1,1,1,1,1,1,1,1,1,1,1,1,1,1,1,1,1,1,1,1,1,4),(0.,0.064201349933887),(14.3984001269719,
15.3908199671856,16.3832398073992,17.3756596476128,18.3680794878265,19.3604993280401,
20.3529191682537,21.3453390084674,22.337758848681,23.3301786888946,24.3225985291083,
25.3150183693219,26.3074382095355,27.2998580497492,28.2922778899628,29.2846977301764,
30.2771175703901,31.2695374106037,32.2619572508173,33.2543770910309,34.2467969312446,
35.2392167714582,36.2316366116718,37.2240564518855,38.2164762920991,39.2088961323127,
40.2013159725264,41.19373581274,42.1861556529536,43.1785754931673,44.1709953333809,
45.1634151735945,46.1558350138082,47.1482548540218,48.1406746942354,49.1330945344491,
50.1255143746627,51.1179342148763,52.11035405509,53.1027738953036,54.0951937355172,
55.0876135757309,56.0800334159445,57.0724532561581,58.0648730963718,59.0572929365854,
60.049712776799,61.0421326170127,62.0345524572263,63.0269722974399,64.0193921376536,
65.0118119778672,66.0042318180808,66.9966516582945,67.9890714985081,68.9814913387217,
69.9739111789354,70.966331019149,71.9587508593626,72.9511706995763,73.9435905397899,
74.9360103800035,75.9284302202172,76.9208500604308,77.9132699006444,78.9056897408581,
79.8981095810717,80.8905294212853,81.882949261499,82.8753691017126,83.8677889419262,
84.8602087821399,85.8526286223535,86.8450484625671,87.8374683027808,88.8298881429944,
89.822307983208,90.8147278234217,91.8071476636353,92.7995675038489,93.7919873440626,
94.7844071842762,95.7768270244898,96.7692468647035,97.7616667049171,98.7540865451307,
99.7465063853444,100.738926225558,101.731346065772,102.723765905985,103.716185746199,
104.708605586413,105.701025426626,106.69344526684,107.685865107053,108.678284947267,
109.670704787481,110.663124627694),.UNSPECIFIED.);
#1332=B_SPLINE_SURFACE_WITH_KNOTS('',3,3,((#50926,#50927,#50928,#50929,
#50930,#50931,#50932,#50933,#50934,#50935,#50936,#50937,#50938,#50939,#50940,
#50941,#50942,#50943,#50944,#50945,#50946,#50947,#50948,#50949,#50950,#50951,
#50952,#50953,#50954,#50955,#50956,#50957,#50958,#50959,#50960,#50961,#50962,
#50963,#50964,#50965,#50966,#50967,#50968,#50969,#50970,#50971,#50972,#50973,
#50974,#50975,#50976,#50977,#50978,#50979,#50980,#50981,#50982,#50983,#50984,
#50985,#50986,#50987,#50988,#50989,#50990,#50991,#50992,#50993,#50994,#50995,
#50996,#50997,#50998,#50999,#51000,#51001,#51002,#51003,#51004,#51005,#51006,
#51007,#51008,#51009,#51010,#51011,#51012,#51013,#51014,#51015,#51016,#51017,
#51018,#51019,#51020,#51021,#51022,#51023,#51024,#51025),(#51026,#51027,
#51028,#51029,#51030,#51031,#51032,#51033,#51034,#51035,#51036,#51037,#51038,
#51039,#51040,#51041,#51042,#51043,#51044,#51045,#51046,#51047,#51048,#51049,
#51050,#51051,#51052,#51053,#51054,#51055,#51056,#51057,#51058,#51059,#51060,
#51061,#51062,#51063,#51064,#51065,#51066,#51067,#51068,#51069,#51070,#51071,
#51072,#51073,#51074,#51075,#51076,#51077,#51078,#51079,#51080,#51081,#51082,
#51083,#51084,#51085,#51086,#51087,#51088,#51089,#51090,#51091,#51092,#51093,
#51094,#51095,#51096,#51097,#51098,#51099,#51100,#51101,#51102,#51103,#51104,
#51105,#51106,#51107,#51108,#51109,#51110,#51111,#51112,#51113,#51114,#51115,
#51116,#51117,#51118,#51119,#51120,#51121,#51122,#51123,#51124,#51125),
(#51126,#51127,#51128,#51129,#51130,#51131,#51132,#51133,#51134,#51135,
#51136,#51137,#51138,#51139,#51140,#51141,#51142,#51143,#51144,#51145,#51146,
#51147,#51148,#51149,#51150,#51151,#51152,#51153,#51154,#51155,#51156,#51157,
#51158,#51159,#51160,#51161,#51162,#51163,#51164,#51165,#51166,#51167,#51168,
#51169,#51170,#51171,#51172,#51173,#51174,#51175,#51176,#51177,#51178,#51179,
#51180,#51181,#51182,#51183,#51184,#51185,#51186,#51187,#51188,#51189,#51190,
#51191,#51192,#51193,#51194,#51195,#51196,#51197,#51198,#51199,#51200,#51201,
#51202,#51203,#51204,#51205,#51206,#51207,#51208,#51209,#51210,#51211,#51212,
#51213,#51214,#51215,#51216,#51217,#51218,#51219,#51220,#51221,#51222,#51223,
#51224,#51225),(#51226,#51227,#51228,#51229,#51230,#51231,#51232,#51233,
#51234,#51235,#51236,#51237,#51238,#51239,#51240,#51241,#51242,#51243,#51244,
#51245,#51246,#51247,#51248,#51249,#51250,#51251,#51252,#51253,#51254,#51255,
#51256,#51257,#51258,#51259,#51260,#51261,#51262,#51263,#51264,#51265,#51266,
#51267,#51268,#51269,#51270,#51271,#51272,#51273,#51274,#51275,#51276,#51277,
#51278,#51279,#51280,#51281,#51282,#51283,#51284,#51285,#51286,#51287,#51288,
#51289,#51290,#51291,#51292,#51293,#51294,#51295,#51296,#51297,#51298,#51299,
#51300,#51301,#51302,#51303,#51304,#51305,#51306,#51307,#51308,#51309,#51310,
#51311,#51312,#51313,#51314,#51315,#51316,#51317,#51318,#51319,#51320,#51321,
#51322,#51323,#51324,#51325)),.UNSPECIFIED.,.F.,.F.,.F.,(4,4),(4,1,1,1,
1,1,1,1,1,1,1,1,1,1,1,1,1,1,1,1,1,1,1,1,1,1,1,1,1,1,1,1,1,1,1,1,1,1,1,1,
1,1,1,1,1,1,1,1,1,1,1,1,1,1,1,1,1,1,1,1,1,1,1,1,1,1,1,1,1,1,1,1,1,1,1,1,
1,1,1,1,1,1,1,1,1,1,1,1,1,1,1,1,1,1,1,1,1,4),(0.,0.064201349933887),(11.8589888623078,
12.8514087025215,13.8438285427351,14.8362483829487,15.8286682231624,16.821088063376,
17.8135079035896,18.8059277438032,19.7983475840169,20.7907674242305,21.7831872644441,
22.7756071046578,23.7680269448714,24.760446785085,25.7528666252987,26.7452864655123,
27.7377063057259,28.7301261459396,29.7225459861532,30.7149658263668,31.7073856665805,
32.6998055067941,33.6922253470077,34.6846451872214,35.677065027435,36.6694848676486,
37.6619047078623,38.6543245480759,39.6467443882895,40.6391642285032,41.6315840687168,
42.6240039089304,43.6164237491441,44.6088435893577,45.6012634295713,46.593683269785,
47.5861031099986,48.5785229502122,49.5709427904259,50.5633626306395,51.5557824708531,
52.5482023110668,53.5406221512804,54.533041991494,55.5254618317077,56.5178816719213,
57.5103015121349,58.5027213523486,59.4951411925622,60.4875610327758,61.4799808729895,
62.4724007132031,63.4648205534167,64.4572403936303,65.449660233844,66.4420800740576,
67.4344999142712,68.4269197544849,69.4193395946985,70.4117594349121,71.4041792751258,
72.3965991153394,73.389018955553,74.3814387957667,75.3738586359803,76.3662784761939,
77.3586983164076,78.3511181566212,79.3435379968348,80.3359578370485,81.3283776772621,
82.3207975174757,83.3132173576894,84.305637197903,85.2980570381166,86.2904768783303,
87.2828967185439,88.2753165587575,89.2677363989712,90.2601562391848,91.2525760793984,
92.2449959196121,93.2374157598257,94.2298356000393,95.222255440253,96.2146752804666,
97.2070951206802,98.1995149608939,99.1919348011075,100.184354641321,101.176774481535,
102.169194321748,103.161614161962,104.154034002176,105.146453842389,106.138873682603,
107.131293522817,108.12371336303),.UNSPECIFIED.);
#1333=B_SPLINE_SURFACE_WITH_KNOTS('',3,3,((#51445,#51446,#51447,#51448,
#51449,#51450,#51451,#51452,#51453,#51454,#51455,#51456,#51457,#51458,#51459,
#51460,#51461,#51462,#51463,#51464,#51465,#51466,#51467,#51468,#51469,#51470,
#51471,#51472,#51473,#51474,#51475,#51476,#51477,#51478,#51479,#51480,#51481,
#51482,#51483,#51484,#51485,#51486,#51487,#51488,#51489,#51490,#51491,#51492,
#51493,#51494,#51495,#51496,#51497,#51498,#51499,#51500,#51501,#51502,#51503,
#51504,#51505,#51506,#51507,#51508,#51509,#51510,#51511,#51512,#51513,#51514,
#51515,#51516,#51517,#51518,#51519,#51520,#51521,#51522,#51523,#51524,#51525,
#51526,#51527,#51528,#51529,#51530,#51531,#51532,#51533,#51534,#51535,#51536,
#51537,#51538,#51539,#51540,#51541,#51542,#51543,#51544),(#51545,#51546,
#51547,#51548,#51549,#51550,#51551,#51552,#51553,#51554,#51555,#51556,#51557,
#51558,#51559,#51560,#51561,#51562,#51563,#51564,#51565,#51566,#51567,#51568,
#51569,#51570,#51571,#51572,#51573,#51574,#51575,#51576,#51577,#51578,#51579,
#51580,#51581,#51582,#51583,#51584,#51585,#51586,#51587,#51588,#51589,#51590,
#51591,#51592,#51593,#51594,#51595,#51596,#51597,#51598,#51599,#51600,#51601,
#51602,#51603,#51604,#51605,#51606,#51607,#51608,#51609,#51610,#51611,#51612,
#51613,#51614,#51615,#51616,#51617,#51618,#51619,#51620,#51621,#51622,#51623,
#51624,#51625,#51626,#51627,#51628,#51629,#51630,#51631,#51632,#51633,#51634,
#51635,#51636,#51637,#51638,#51639,#51640,#51641,#51642,#51643,#51644),
(#51645,#51646,#51647,#51648,#51649,#51650,#51651,#51652,#51653,#51654,
#51655,#51656,#51657,#51658,#51659,#51660,#51661,#51662,#51663,#51664,#51665,
#51666,#51667,#51668,#51669,#51670,#51671,#51672,#51673,#51674,#51675,#51676,
#51677,#51678,#51679,#51680,#51681,#51682,#51683,#51684,#51685,#51686,#51687,
#51688,#51689,#51690,#51691,#51692,#51693,#51694,#51695,#51696,#51697,#51698,
#51699,#51700,#51701,#51702,#51703,#51704,#51705,#51706,#51707,#51708,#51709,
#51710,#51711,#51712,#51713,#51714,#51715,#51716,#51717,#51718,#51719,#51720,
#51721,#51722,#51723,#51724,#51725,#51726,#51727,#51728,#51729,#51730,#51731,
#51732,#51733,#51734,#51735,#51736,#51737,#51738,#51739,#51740,#51741,#51742,
#51743,#51744),(#51745,#51746,#51747,#51748,#51749,#51750,#51751,#51752,
#51753,#51754,#51755,#51756,#51757,#51758,#51759,#51760,#51761,#51762,#51763,
#51764,#51765,#51766,#51767,#51768,#51769,#51770,#51771,#51772,#51773,#51774,
#51775,#51776,#51777,#51778,#51779,#51780,#51781,#51782,#51783,#51784,#51785,
#51786,#51787,#51788,#51789,#51790,#51791,#51792,#51793,#51794,#51795,#51796,
#51797,#51798,#51799,#51800,#51801,#51802,#51803,#51804,#51805,#51806,#51807,
#51808,#51809,#51810,#51811,#51812,#51813,#51814,#51815,#51816,#51817,#51818,
#51819,#51820,#51821,#51822,#51823,#51824,#51825,#51826,#51827,#51828,#51829,
#51830,#51831,#51832,#51833,#51834,#51835,#51836,#51837,#51838,#51839,#51840,
#51841,#51842,#51843,#51844)),.UNSPECIFIED.,.F.,.F.,.F.,(4,4),(4,1,1,1,
1,1,1,1,1,1,1,1,1,1,1,1,1,1,1,1,1,1,1,1,1,1,1,1,1,1,1,1,1,1,1,1,1,1,1,1,
1,1,1,1,1,1,1,1,1,1,1,1,1,1,1,1,1,1,1,1,1,1,1,1,1,1,1,1,1,1,1,1,1,1,1,1,
1,1,1,1,1,1,1,1,1,1,1,1,1,1,1,1,1,1,1,1,1,4),(0.,0.064201349933887),(14.3984001269719,
15.3908199671856,16.3832398073992,17.3756596476128,18.3680794878265,19.3604993280401,
20.3529191682537,21.3453390084674,22.337758848681,23.3301786888946,24.3225985291083,
25.3150183693219,26.3074382095355,27.2998580497492,28.2922778899628,29.2846977301764,
30.2771175703901,31.2695374106037,32.2619572508173,33.2543770910309,34.2467969312446,
35.2392167714582,36.2316366116718,37.2240564518855,38.2164762920991,39.2088961323127,
40.2013159725264,41.19373581274,42.1861556529536,43.1785754931673,44.1709953333809,
45.1634151735945,46.1558350138082,47.1482548540218,48.1406746942354,49.1330945344491,
50.1255143746627,51.1179342148763,52.11035405509,53.1027738953036,54.0951937355172,
55.0876135757309,56.0800334159445,57.0724532561581,58.0648730963718,59.0572929365854,
60.049712776799,61.0421326170127,62.0345524572263,63.0269722974399,64.0193921376536,
65.0118119778672,66.0042318180808,66.9966516582945,67.9890714985081,68.9814913387217,
69.9739111789354,70.966331019149,71.9587508593626,72.9511706995763,73.9435905397899,
74.9360103800035,75.9284302202172,76.9208500604308,77.9132699006444,78.9056897408581,
79.8981095810717,80.8905294212853,81.882949261499,82.8753691017126,83.8677889419262,
84.8602087821399,85.8526286223535,86.8450484625671,87.8374683027808,88.8298881429944,
89.822307983208,90.8147278234217,91.8071476636353,92.7995675038489,93.7919873440626,
94.7844071842762,95.7768270244898,96.7692468647035,97.7616667049171,98.7540865451307,
99.7465063853444,100.738926225558,101.731346065772,102.723765905985,103.716185746199,
104.708605586413,105.701025426626,106.69344526684,107.685865107053,108.678284947267,
109.670704787481,110.663124627694),.UNSPECIFIED.);
#1480=PLANE('',#25693);
#1481=PLANE('',#25696);
#1482=PLANE('',#25699);
#1483=PLANE('',#25702);
#1484=PLANE('',#25705);
#1485=PLANE('',#25708);
#1486=PLANE('',#25711);
#1487=PLANE('',#25714);
#1488=PLANE('',#25717);
#1489=PLANE('',#25718);
#1490=PLANE('',#25719);
#1491=PLANE('',#25720);
#1492=PLANE('',#25721);
#1493=PLANE('',#25722);
#1494=PLANE('',#25723);
#1495=PLANE('',#25724);
#1496=PLANE('',#25740);
#1497=PLANE('',#25748);
#1498=PLANE('',#25749);
#1499=PLANE('',#25755);
#1500=PLANE('',#25756);
#1698=FACE_OUTER_BOUND('',#3044,.T.);
#1699=FACE_OUTER_BOUND('',#3045,.T.);
#1700=FACE_OUTER_BOUND('',#3046,.T.);
#1701=FACE_OUTER_BOUND('',#3047,.T.);
#1702=FACE_OUTER_BOUND('',#3048,.T.);
#1703=FACE_OUTER_BOUND('',#3049,.T.);
#1704=FACE_OUTER_BOUND('',#3050,.T.);
#1705=FACE_OUTER_BOUND('',#3051,.T.);
#1706=FACE_OUTER_BOUND('',#3052,.T.);
#1707=FACE_OUTER_BOUND('',#3053,.T.);
#1708=FACE_OUTER_BOUND('',#3054,.T.);
#1709=FACE_OUTER_BOUND('',#3055,.T.);
#1710=FACE_OUTER_BOUND('',#3056,.T.);
#1711=FACE_OUTER_BOUND('',#3057,.T.);
#1712=FACE_OUTER_BOUND('',#3058,.T.);
#1713=FACE_OUTER_BOUND('',#3059,.T.);
#1714=FACE_OUTER_BOUND('',#3060,.T.);
#1715=FACE_OUTER_BOUND('',#3061,.T.);
#1716=FACE_OUTER_BOUND('',#3062,.T.);
#1717=FACE_OUTER_BOUND('',#3063,.T.);
#1718=FACE_OUTER_BOUND('',#3064,.T.);
#1719=FACE_OUTER_BOUND('',#3065,.T.);
#1720=FACE_OUTER_BOUND('',#3066,.T.);
#1721=FACE_OUTER_BOUND('',#3067,.T.);
#1722=FACE_OUTER_BOUND('',#3068,.T.);
#1723=FACE_OUTER_BOUND('',#3069,.T.);
#1724=FACE_OUTER_BOUND('',#3070,.T.);
#1725=FACE_OUTER_BOUND('',#3071,.T.);
#1726=FACE_OUTER_BOUND('',#3072,.T.);
#1727=FACE_OUTER_BOUND('',#3073,.T.);
#1728=FACE_OUTER_BOUND('',#3074,.T.);
#1729=FACE_OUTER_BOUND('',#3075,.T.);
#1730=FACE_OUTER_BOUND('',#3076,.T.);
#1731=FACE_OUTER_BOUND('',#3077,.T.);
#1732=FACE_OUTER_BOUND('',#3078,.T.);
#1733=FACE_OUTER_BOUND('',#3079,.T.);
#1734=FACE_OUTER_BOUND('',#3080,.T.);
#1735=FACE_OUTER_BOUND('',#3081,.T.);
#1736=FACE_OUTER_BOUND('',#3082,.T.);
#1737=FACE_OUTER_BOUND('',#3083,.T.);
#1738=FACE_OUTER_BOUND('',#3084,.T.);
#1739=FACE_OUTER_BOUND('',#3085,.T.);
#1740=FACE_OUTER_BOUND('',#3086,.T.);
#1741=FACE_OUTER_BOUND('',#3087,.T.);
#1742=FACE_OUTER_BOUND('',#3088,.T.);
#1743=FACE_OUTER_BOUND('',#3089,.T.);
#1744=FACE_OUTER_BOUND('',#3090,.T.);
#1745=FACE_OUTER_BOUND('',#3091,.T.);
#1746=FACE_OUTER_BOUND('',#3092,.T.);
#1747=FACE_OUTER_BOUND('',#3093,.T.);
#1748=FACE_OUTER_BOUND('',#3094,.T.);
#1749=FACE_OUTER_BOUND('',#3095,.T.);
#1750=FACE_OUTER_BOUND('',#3096,.T.);
#1751=FACE_OUTER_BOUND('',#3097,.T.);
#1752=FACE_OUTER_BOUND('',#3098,.T.);
#1753=FACE_OUTER_BOUND('',#3099,.T.);
#1754=FACE_OUTER_BOUND('',#3100,.T.);
#1755=FACE_OUTER_BOUND('',#3101,.T.);
#1756=FACE_OUTER_BOUND('',#3102,.T.);
#1757=FACE_OUTER_BOUND('',#3103,.T.);
#1758=FACE_OUTER_BOUND('',#3104,.T.);
#1759=FACE_OUTER_BOUND('',#3105,.T.);
#1760=FACE_OUTER_BOUND('',#3106,.T.);
#1761=FACE_OUTER_BOUND('',#3107,.T.);
#1762=FACE_OUTER_BOUND('',#3108,.T.);
#1763=FACE_OUTER_BOUND('',#3109,.T.);
#1764=FACE_OUTER_BOUND('',#3110,.T.);
#1765=FACE_OUTER_BOUND('',#3111,.T.);
#1766=FACE_OUTER_BOUND('',#3112,.T.);
#1767=FACE_OUTER_BOUND('',#3113,.T.);
#1768=FACE_OUTER_BOUND('',#3114,.T.);
#1769=FACE_OUTER_BOUND('',#3115,.T.);
#1770=FACE_OUTER_BOUND('',#3116,.T.);
#1771=FACE_OUTER_BOUND('',#3117,.T.);
#1772=FACE_OUTER_BOUND('',#3118,.T.);
#1773=FACE_OUTER_BOUND('',#3119,.T.);
#1774=FACE_OUTER_BOUND('',#3120,.T.);
#1775=FACE_OUTER_BOUND('',#3121,.T.);
#1776=FACE_OUTER_BOUND('',#3122,.T.);
#1777=FACE_OUTER_BOUND('',#3123,.T.);
#1778=FACE_OUTER_BOUND('',#3124,.T.);
#1779=FACE_OUTER_BOUND('',#3125,.T.);
#1780=FACE_OUTER_BOUND('',#3126,.T.);
#1781=FACE_OUTER_BOUND('',#3127,.T.);
#1782=FACE_OUTER_BOUND('',#3128,.T.);
#1783=FACE_OUTER_BOUND('',#3129,.T.);
#1784=FACE_OUTER_BOUND('',#3130,.T.);
#1785=FACE_OUTER_BOUND('',#3131,.T.);
#1786=FACE_OUTER_BOUND('',#3132,.T.);
#1787=FACE_OUTER_BOUND('',#3133,.T.);
#1788=FACE_OUTER_BOUND('',#3134,.T.);
#1789=FACE_OUTER_BOUND('',#3135,.T.);
#1790=FACE_OUTER_BOUND('',#3136,.T.);
#1791=FACE_OUTER_BOUND('',#3137,.T.);
#1792=FACE_OUTER_BOUND('',#3138,.T.);
#1793=FACE_OUTER_BOUND('',#3139,.T.);
#1794=FACE_OUTER_BOUND('',#3140,.T.);
#1795=FACE_OUTER_BOUND('',#3141,.T.);
#1796=FACE_OUTER_BOUND('',#3142,.T.);
#1797=FACE_OUTER_BOUND('',#3143,.T.);
#1798=FACE_OUTER_BOUND('',#3144,.T.);
#1799=FACE_OUTER_BOUND('',#3145,.T.);
#1800=FACE_OUTER_BOUND('',#3146,.T.);
#1801=FACE_OUTER_BOUND('',#3147,.T.);
#1802=FACE_OUTER_BOUND('',#3148,.T.);
#1803=FACE_OUTER_BOUND('',#3149,.T.);
#1804=FACE_OUTER_BOUND('',#3150,.T.);
#1805=FACE_OUTER_BOUND('',#3151,.T.);
#1806=FACE_OUTER_BOUND('',#3152,.T.);
#1807=FACE_OUTER_BOUND('',#3153,.T.);
#1808=FACE_OUTER_BOUND('',#3154,.T.);
#1809=FACE_OUTER_BOUND('',#3155,.T.);
#1810=FACE_OUTER_BOUND('',#3156,.T.);
#1811=FACE_OUTER_BOUND('',#3157,.T.);
#1812=FACE_OUTER_BOUND('',#3158,.T.);
#1813=FACE_OUTER_BOUND('',#3159,.T.);
#1814=FACE_OUTER_BOUND('',#3160,.T.);
#1815=FACE_OUTER_BOUND('',#3161,.T.);
#1816=FACE_OUTER_BOUND('',#3162,.T.);
#1817=FACE_OUTER_BOUND('',#3163,.T.);
#1818=FACE_OUTER_BOUND('',#3164,.T.);
#1819=FACE_OUTER_BOUND('',#3165,.T.);
#1820=FACE_OUTER_BOUND('',#3166,.T.);
#1821=FACE_OUTER_BOUND('',#3167,.T.);
#1822=FACE_OUTER_BOUND('',#3168,.T.);
#1823=FACE_OUTER_BOUND('',#3169,.T.);
#1824=FACE_OUTER_BOUND('',#3170,.T.);
#1825=FACE_OUTER_BOUND('',#3171,.T.);
#1826=FACE_OUTER_BOUND('',#3172,.T.);
#1827=FACE_OUTER_BOUND('',#3173,.T.);
#1828=FACE_OUTER_BOUND('',#3174,.T.);
#1829=FACE_OUTER_BOUND('',#3175,.T.);
#1830=FACE_OUTER_BOUND('',#3176,.T.);
#1831=FACE_OUTER_BOUND('',#3177,.T.);
#1832=FACE_OUTER_BOUND('',#3178,.T.);
#1833=FACE_OUTER_BOUND('',#3179,.T.);
#1834=FACE_OUTER_BOUND('',#3180,.T.);
#1835=FACE_OUTER_BOUND('',#3181,.T.);
#1836=FACE_OUTER_BOUND('',#3182,.T.);
#1837=FACE_OUTER_BOUND('',#3183,.T.);
#1838=FACE_OUTER_BOUND('',#3184,.T.);
#1839=FACE_OUTER_BOUND('',#3185,.T.);
#1840=FACE_OUTER_BOUND('',#3186,.T.);
#1841=FACE_OUTER_BOUND('',#3187,.T.);
#1842=FACE_OUTER_BOUND('',#3188,.T.);
#1843=FACE_OUTER_BOUND('',#3189,.T.);
#1844=FACE_OUTER_BOUND('',#3190,.T.);
#1845=FACE_OUTER_BOUND('',#3191,.T.);
#1846=FACE_OUTER_BOUND('',#3192,.T.);
#1847=FACE_OUTER_BOUND('',#3193,.T.);
#1848=FACE_OUTER_BOUND('',#3194,.T.);
#1849=FACE_OUTER_BOUND('',#3195,.T.);
#1850=FACE_OUTER_BOUND('',#3196,.T.);
#1851=FACE_OUTER_BOUND('',#3197,.T.);
#1852=FACE_OUTER_BOUND('',#3198,.T.);
#1853=FACE_OUTER_BOUND('',#3199,.T.);
#1854=FACE_OUTER_BOUND('',#3200,.T.);
#1855=FACE_OUTER_BOUND('',#3201,.T.);
#1856=FACE_OUTER_BOUND('',#3202,.T.);
#1857=FACE_OUTER_BOUND('',#3203,.T.);
#1858=FACE_OUTER_BOUND('',#3204,.T.);
#1859=FACE_OUTER_BOUND('',#3205,.T.);
#1860=FACE_OUTER_BOUND('',#3206,.T.);
#1861=FACE_OUTER_BOUND('',#3207,.T.);
#1862=FACE_OUTER_BOUND('',#3208,.T.);
#1863=FACE_OUTER_BOUND('',#3209,.T.);
#1864=FACE_OUTER_BOUND('',#3210,.T.);
#1865=FACE_OUTER_BOUND('',#3211,.T.);
#1866=FACE_OUTER_BOUND('',#3212,.T.);
#1867=FACE_OUTER_BOUND('',#3213,.T.);
#1868=FACE_OUTER_BOUND('',#3214,.T.);
#1869=FACE_OUTER_BOUND('',#3215,.T.);
#1870=FACE_OUTER_BOUND('',#3216,.T.);
#1871=FACE_OUTER_BOUND('',#3217,.T.);
#1872=FACE_OUTER_BOUND('',#3218,.T.);
#1873=FACE_OUTER_BOUND('',#3219,.T.);
#1874=FACE_OUTER_BOUND('',#3220,.T.);
#1875=FACE_OUTER_BOUND('',#3221,.T.);
#1876=FACE_OUTER_BOUND('',#3222,.T.);
#1877=FACE_OUTER_BOUND('',#3223,.T.);
#1878=FACE_OUTER_BOUND('',#3224,.T.);
#1879=FACE_OUTER_BOUND('',#3225,.T.);
#1880=FACE_OUTER_BOUND('',#3226,.T.);
#1881=FACE_OUTER_BOUND('',#3227,.T.);
#1882=FACE_OUTER_BOUND('',#3228,.T.);
#1883=FACE_OUTER_BOUND('',#3229,.T.);
#1884=FACE_OUTER_BOUND('',#3230,.T.);
#1885=FACE_OUTER_BOUND('',#3231,.T.);
#1886=FACE_OUTER_BOUND('',#3232,.T.);
#1887=FACE_OUTER_BOUND('',#3233,.T.);
#1888=FACE_OUTER_BOUND('',#3234,.T.);
#1889=FACE_OUTER_BOUND('',#3235,.T.);
#1890=FACE_OUTER_BOUND('',#3236,.T.);
#1891=FACE_OUTER_BOUND('',#3237,.T.);
#1892=FACE_OUTER_BOUND('',#3238,.T.);
#1893=FACE_OUTER_BOUND('',#3239,.T.);
#1894=FACE_OUTER_BOUND('',#3240,.T.);
#1895=FACE_OUTER_BOUND('',#3241,.T.);
#1896=FACE_OUTER_BOUND('',#3242,.T.);
#1897=FACE_OUTER_BOUND('',#3243,.T.);
#1898=FACE_OUTER_BOUND('',#3244,.T.);
#1899=FACE_OUTER_BOUND('',#3245,.T.);
#1900=FACE_OUTER_BOUND('',#3246,.T.);
#1901=FACE_OUTER_BOUND('',#3247,.T.);
#1902=FACE_OUTER_BOUND('',#3248,.T.);
#1903=FACE_OUTER_BOUND('',#3249,.T.);
#1904=FACE_OUTER_BOUND('',#3250,.T.);
#1905=FACE_OUTER_BOUND('',#3251,.T.);
#1906=FACE_OUTER_BOUND('',#3252,.T.);
#1907=FACE_OUTER_BOUND('',#3253,.T.);
#1908=FACE_OUTER_BOUND('',#3254,.T.);
#1909=FACE_OUTER_BOUND('',#3255,.T.);
#1910=FACE_OUTER_BOUND('',#3256,.T.);
#1911=FACE_OUTER_BOUND('',#3257,.T.);
#1912=FACE_OUTER_BOUND('',#3258,.T.);
#1913=FACE_OUTER_BOUND('',#3259,.T.);
#1914=FACE_OUTER_BOUND('',#3260,.T.);
#1915=FACE_OUTER_BOUND('',#3261,.T.);
#1916=FACE_OUTER_BOUND('',#3262,.T.);
#1917=FACE_OUTER_BOUND('',#3263,.T.);
#1918=FACE_OUTER_BOUND('',#3264,.T.);
#1919=FACE_OUTER_BOUND('',#3265,.T.);
#1920=FACE_OUTER_BOUND('',#3266,.T.);
#1921=FACE_OUTER_BOUND('',#3267,.T.);
#1922=FACE_OUTER_BOUND('',#3268,.T.);
#1923=FACE_OUTER_BOUND('',#3269,.T.);
#1924=FACE_OUTER_BOUND('',#3270,.T.);
#1925=FACE_OUTER_BOUND('',#3271,.T.);
#1926=FACE_OUTER_BOUND('',#3272,.T.);
#1927=FACE_OUTER_BOUND('',#3273,.T.);
#1928=FACE_OUTER_BOUND('',#3274,.T.);
#1929=FACE_OUTER_BOUND('',#3275,.T.);
#1930=FACE_OUTER_BOUND('',#3276,.T.);
#1931=FACE_OUTER_BOUND('',#3277,.T.);
#1932=FACE_OUTER_BOUND('',#3278,.T.);
#1933=FACE_OUTER_BOUND('',#3279,.T.);
#1934=FACE_OUTER_BOUND('',#3280,.T.);
#1935=FACE_OUTER_BOUND('',#3281,.T.);
#1936=FACE_OUTER_BOUND('',#3282,.T.);
#1937=FACE_OUTER_BOUND('',#3283,.T.);
#1938=FACE_OUTER_BOUND('',#3284,.T.);
#1939=FACE_OUTER_BOUND('',#3285,.T.);
#1940=FACE_OUTER_BOUND('',#3286,.T.);
#1941=FACE_OUTER_BOUND('',#3287,.T.);
#1942=FACE_OUTER_BOUND('',#3288,.T.);
#1943=FACE_OUTER_BOUND('',#3289,.T.);
#1944=FACE_OUTER_BOUND('',#3290,.T.);
#1945=FACE_OUTER_BOUND('',#3291,.T.);
#1946=FACE_OUTER_BOUND('',#3292,.T.);
#1947=FACE_OUTER_BOUND('',#3293,.T.);
#1948=FACE_OUTER_BOUND('',#3294,.T.);
#1949=FACE_OUTER_BOUND('',#3295,.T.);
#1950=FACE_OUTER_BOUND('',#3296,.T.);
#1951=FACE_OUTER_BOUND('',#3297,.T.);
#1952=FACE_OUTER_BOUND('',#3298,.T.);
#1953=FACE_OUTER_BOUND('',#3299,.T.);
#1954=FACE_OUTER_BOUND('',#3300,.T.);
#1955=FACE_OUTER_BOUND('',#3301,.T.);
#1956=FACE_OUTER_BOUND('',#3302,.T.);
#1957=FACE_OUTER_BOUND('',#3303,.T.);
#1958=FACE_OUTER_BOUND('',#3304,.T.);
#1959=FACE_OUTER_BOUND('',#3305,.T.);
#1960=FACE_OUTER_BOUND('',#3306,.T.);
#1961=FACE_OUTER_BOUND('',#3307,.T.);
#1962=FACE_OUTER_BOUND('',#3308,.T.);
#1963=FACE_OUTER_BOUND('',#3309,.T.);
#1964=FACE_OUTER_BOUND('',#3310,.T.);
#1965=FACE_OUTER_BOUND('',#3311,.T.);
#1966=FACE_OUTER_BOUND('',#3312,.T.);
#1967=FACE_OUTER_BOUND('',#3313,.T.);
#1968=FACE_OUTER_BOUND('',#3314,.T.);
#1969=FACE_OUTER_BOUND('',#3315,.T.);
#1970=FACE_OUTER_BOUND('',#3316,.T.);
#1971=FACE_OUTER_BOUND('',#3317,.T.);
#1972=FACE_OUTER_BOUND('',#3318,.T.);
#1973=FACE_OUTER_BOUND('',#3319,.T.);
#1974=FACE_OUTER_BOUND('',#3320,.T.);
#1975=FACE_OUTER_BOUND('',#3321,.T.);
#1976=FACE_OUTER_BOUND('',#3322,.T.);
#1977=FACE_OUTER_BOUND('',#3323,.T.);
#1978=FACE_OUTER_BOUND('',#3324,.T.);
#1979=FACE_OUTER_BOUND('',#3325,.T.);
#1980=FACE_OUTER_BOUND('',#3326,.T.);
#1981=FACE_OUTER_BOUND('',#3327,.T.);
#1982=FACE_OUTER_BOUND('',#3328,.T.);
#1983=FACE_OUTER_BOUND('',#3329,.T.);
#1984=FACE_OUTER_BOUND('',#3330,.T.);
#1985=FACE_OUTER_BOUND('',#3331,.T.);
#1986=FACE_OUTER_BOUND('',#3332,.T.);
#1987=FACE_OUTER_BOUND('',#3333,.T.);
#1988=FACE_OUTER_BOUND('',#3334,.T.);
#1989=FACE_OUTER_BOUND('',#3335,.T.);
#1990=FACE_OUTER_BOUND('',#3336,.T.);
#1991=FACE_OUTER_BOUND('',#3337,.T.);
#1992=FACE_OUTER_BOUND('',#3338,.T.);
#1993=FACE_OUTER_BOUND('',#3339,.T.);
#1994=FACE_OUTER_BOUND('',#3340,.T.);
#1995=FACE_OUTER_BOUND('',#3341,.T.);
#1996=FACE_OUTER_BOUND('',#3342,.T.);
#1997=FACE_OUTER_BOUND('',#3343,.T.);
#1998=FACE_OUTER_BOUND('',#3344,.T.);
#1999=FACE_OUTER_BOUND('',#3345,.T.);
#2000=FACE_OUTER_BOUND('',#3346,.T.);
#2001=FACE_OUTER_BOUND('',#3347,.T.);
#2002=FACE_OUTER_BOUND('',#3348,.T.);
#2003=FACE_OUTER_BOUND('',#3349,.T.);
#2004=FACE_OUTER_BOUND('',#3351,.T.);
#2005=FACE_OUTER_BOUND('',#3361,.T.);
#2006=FACE_OUTER_BOUND('',#3371,.T.);
#2007=FACE_OUTER_BOUND('',#3381,.T.);
#2008=FACE_OUTER_BOUND('',#3387,.T.);
#2009=FACE_OUTER_BOUND('',#3388,.T.);
#2010=FACE_OUTER_BOUND('',#3389,.T.);
#2011=FACE_OUTER_BOUND('',#3391,.T.);
#3044=EDGE_LOOP('',(#15424,#15425,#15426,#15427,#15428,#15429,#15430,#15431));
#3045=EDGE_LOOP('',(#15432,#15433,#15434,#15435));
#3046=EDGE_LOOP('',(#15436,#15437,#15438,#15439));
#3047=EDGE_LOOP('',(#15440,#15441,#15442,#15443));
#3048=EDGE_LOOP('',(#15444,#15445,#15446,#15447));
#3049=EDGE_LOOP('',(#15448,#15449,#15450,#15451));
#3050=EDGE_LOOP('',(#15452,#15453,#15454,#15455));
#3051=EDGE_LOOP('',(#15456,#15457,#15458,#15459));
#3052=EDGE_LOOP('',(#15460,#15461,#15462,#15463));
#3053=EDGE_LOOP('',(#15464,#15465,#15466,#15467));
#3054=EDGE_LOOP('',(#15468,#15469,#15470,#15471));
#3055=EDGE_LOOP('',(#15472,#15473,#15474,#15475));
#3056=EDGE_LOOP('',(#15476,#15477,#15478,#15479));
#3057=EDGE_LOOP('',(#15480,#15481,#15482,#15483));
#3058=EDGE_LOOP('',(#15484,#15485,#15486,#15487));
#3059=EDGE_LOOP('',(#15488,#15489,#15490,#15491));
#3060=EDGE_LOOP('',(#15492,#15493,#15494,#15495));
#3061=EDGE_LOOP('',(#15496,#15497,#15498,#15499));
#3062=EDGE_LOOP('',(#15500,#15501,#15502,#15503));
#3063=EDGE_LOOP('',(#15504,#15505,#15506,#15507));
#3064=EDGE_LOOP('',(#15508,#15509,#15510,#15511));
#3065=EDGE_LOOP('',(#15512,#15513,#15514,#15515));
#3066=EDGE_LOOP('',(#15516,#15517,#15518,#15519));
#3067=EDGE_LOOP('',(#15520,#15521,#15522,#15523));
#3068=EDGE_LOOP('',(#15524,#15525,#15526,#15527));
#3069=EDGE_LOOP('',(#15528,#15529,#15530,#15531));
#3070=EDGE_LOOP('',(#15532,#15533,#15534,#15535));
#3071=EDGE_LOOP('',(#15536,#15537,#15538,#15539));
#3072=EDGE_LOOP('',(#15540,#15541,#15542,#15543));
#3073=EDGE_LOOP('',(#15544,#15545,#15546,#15547));
#3074=EDGE_LOOP('',(#15548,#15549,#15550,#15551,#15552,#15553,#15554,#15555));
#3075=EDGE_LOOP('',(#15556,#15557,#15558,#15559));
#3076=EDGE_LOOP('',(#15560,#15561,#15562,#15563));
#3077=EDGE_LOOP('',(#15564,#15565,#15566,#15567));
#3078=EDGE_LOOP('',(#15568,#15569,#15570,#15571));
#3079=EDGE_LOOP('',(#15572,#15573,#15574,#15575));
#3080=EDGE_LOOP('',(#15576,#15577,#15578,#15579));
#3081=EDGE_LOOP('',(#15580,#15581,#15582,#15583));
#3082=EDGE_LOOP('',(#15584,#15585,#15586,#15587));
#3083=EDGE_LOOP('',(#15588,#15589,#15590,#15591));
#3084=EDGE_LOOP('',(#15592,#15593,#15594,#15595));
#3085=EDGE_LOOP('',(#15596,#15597,#15598,#15599));
#3086=EDGE_LOOP('',(#15600,#15601,#15602,#15603));
#3087=EDGE_LOOP('',(#15604,#15605,#15606,#15607));
#3088=EDGE_LOOP('',(#15608,#15609,#15610,#15611));
#3089=EDGE_LOOP('',(#15612,#15613,#15614,#15615));
#3090=EDGE_LOOP('',(#15616,#15617,#15618,#15619));
#3091=EDGE_LOOP('',(#15620,#15621,#15622,#15623));
#3092=EDGE_LOOP('',(#15624,#15625,#15626,#15627));
#3093=EDGE_LOOP('',(#15628,#15629,#15630,#15631));
#3094=EDGE_LOOP('',(#15632,#15633,#15634,#15635));
#3095=EDGE_LOOP('',(#15636,#15637,#15638,#15639));
#3096=EDGE_LOOP('',(#15640,#15641,#15642,#15643));
#3097=EDGE_LOOP('',(#15644,#15645,#15646,#15647));
#3098=EDGE_LOOP('',(#15648,#15649,#15650,#15651));
#3099=EDGE_LOOP('',(#15652,#15653,#15654,#15655));
#3100=EDGE_LOOP('',(#15656,#15657,#15658,#15659));
#3101=EDGE_LOOP('',(#15660,#15661,#15662,#15663));
#3102=EDGE_LOOP('',(#15664,#15665,#15666,#15667));
#3103=EDGE_LOOP('',(#15668,#15669,#15670,#15671));
#3104=EDGE_LOOP('',(#15672,#15673,#15674,#15675,#15676,#15677,#15678,#15679));
#3105=EDGE_LOOP('',(#15680,#15681,#15682,#15683));
#3106=EDGE_LOOP('',(#15684,#15685,#15686,#15687));
#3107=EDGE_LOOP('',(#15688,#15689,#15690,#15691));
#3108=EDGE_LOOP('',(#15692,#15693,#15694,#15695));
#3109=EDGE_LOOP('',(#15696,#15697,#15698,#15699));
#3110=EDGE_LOOP('',(#15700,#15701,#15702,#15703));
#3111=EDGE_LOOP('',(#15704,#15705,#15706,#15707));
#3112=EDGE_LOOP('',(#15708,#15709,#15710,#15711));
#3113=EDGE_LOOP('',(#15712,#15713,#15714,#15715));
#3114=EDGE_LOOP('',(#15716,#15717,#15718,#15719));
#3115=EDGE_LOOP('',(#15720,#15721,#15722,#15723));
#3116=EDGE_LOOP('',(#15724,#15725,#15726,#15727));
#3117=EDGE_LOOP('',(#15728,#15729,#15730,#15731));
#3118=EDGE_LOOP('',(#15732,#15733,#15734,#15735));
#3119=EDGE_LOOP('',(#15736,#15737,#15738,#15739));
#3120=EDGE_LOOP('',(#15740,#15741,#15742,#15743));
#3121=EDGE_LOOP('',(#15744,#15745,#15746,#15747));
#3122=EDGE_LOOP('',(#15748,#15749,#15750,#15751));
#3123=EDGE_LOOP('',(#15752,#15753,#15754,#15755));
#3124=EDGE_LOOP('',(#15756,#15757,#15758,#15759));
#3125=EDGE_LOOP('',(#15760,#15761,#15762,#15763));
#3126=EDGE_LOOP('',(#15764,#15765,#15766,#15767));
#3127=EDGE_LOOP('',(#15768,#15769,#15770,#15771));
#3128=EDGE_LOOP('',(#15772,#15773,#15774,#15775));
#3129=EDGE_LOOP('',(#15776,#15777,#15778,#15779));
#3130=EDGE_LOOP('',(#15780,#15781,#15782,#15783));
#3131=EDGE_LOOP('',(#15784,#15785,#15786,#15787));
#3132=EDGE_LOOP('',(#15788,#15789,#15790,#15791));
#3133=EDGE_LOOP('',(#15792,#15793,#15794,#15795));
#3134=EDGE_LOOP('',(#15796,#15797,#15798,#15799,#15800,#15801,#15802,#15803));
#3135=EDGE_LOOP('',(#15804,#15805,#15806,#15807));
#3136=EDGE_LOOP('',(#15808,#15809,#15810,#15811));
#3137=EDGE_LOOP('',(#15812,#15813,#15814,#15815));
#3138=EDGE_LOOP('',(#15816,#15817,#15818,#15819));
#3139=EDGE_LOOP('',(#15820,#15821,#15822,#15823));
#3140=EDGE_LOOP('',(#15824,#15825,#15826,#15827));
#3141=EDGE_LOOP('',(#15828,#15829,#15830,#15831));
#3142=EDGE_LOOP('',(#15832,#15833,#15834,#15835));
#3143=EDGE_LOOP('',(#15836,#15837,#15838,#15839));
#3144=EDGE_LOOP('',(#15840,#15841,#15842,#15843));
#3145=EDGE_LOOP('',(#15844,#15845,#15846,#15847));
#3146=EDGE_LOOP('',(#15848,#15849,#15850,#15851));
#3147=EDGE_LOOP('',(#15852,#15853,#15854,#15855));
#3148=EDGE_LOOP('',(#15856,#15857,#15858,#15859));
#3149=EDGE_LOOP('',(#15860,#15861,#15862,#15863));
#3150=EDGE_LOOP('',(#15864,#15865,#15866,#15867));
#3151=EDGE_LOOP('',(#15868,#15869,#15870,#15871));
#3152=EDGE_LOOP('',(#15872,#15873,#15874,#15875));
#3153=EDGE_LOOP('',(#15876,#15877,#15878,#15879));
#3154=EDGE_LOOP('',(#15880,#15881,#15882,#15883));
#3155=EDGE_LOOP('',(#15884,#15885,#15886,#15887));
#3156=EDGE_LOOP('',(#15888,#15889,#15890,#15891));
#3157=EDGE_LOOP('',(#15892,#15893,#15894,#15895));
#3158=EDGE_LOOP('',(#15896,#15897,#15898,#15899));
#3159=EDGE_LOOP('',(#15900,#15901,#15902,#15903));
#3160=EDGE_LOOP('',(#15904,#15905,#15906,#15907));
#3161=EDGE_LOOP('',(#15908,#15909,#15910,#15911));
#3162=EDGE_LOOP('',(#15912,#15913,#15914,#15915));
#3163=EDGE_LOOP('',(#15916,#15917,#15918,#15919));
#3164=EDGE_LOOP('',(#15920,#15921,#15922,#15923,#15924,#15925,#15926,#15927));
#3165=EDGE_LOOP('',(#15928,#15929,#15930,#15931));
#3166=EDGE_LOOP('',(#15932,#15933,#15934,#15935));
#3167=EDGE_LOOP('',(#15936,#15937,#15938,#15939));
#3168=EDGE_LOOP('',(#15940,#15941,#15942,#15943));
#3169=EDGE_LOOP('',(#15944,#15945,#15946,#15947));
#3170=EDGE_LOOP('',(#15948,#15949,#15950,#15951));
#3171=EDGE_LOOP('',(#15952,#15953,#15954,#15955));
#3172=EDGE_LOOP('',(#15956,#15957,#15958,#15959));
#3173=EDGE_LOOP('',(#15960,#15961,#15962,#15963));
#3174=EDGE_LOOP('',(#15964,#15965,#15966,#15967));
#3175=EDGE_LOOP('',(#15968,#15969,#15970,#15971));
#3176=EDGE_LOOP('',(#15972,#15973,#15974,#15975));
#3177=EDGE_LOOP('',(#15976,#15977,#15978,#15979));
#3178=EDGE_LOOP('',(#15980,#15981,#15982,#15983));
#3179=EDGE_LOOP('',(#15984,#15985,#15986,#15987));
#3180=EDGE_LOOP('',(#15988,#15989,#15990,#15991));
#3181=EDGE_LOOP('',(#15992,#15993,#15994,#15995));
#3182=EDGE_LOOP('',(#15996,#15997,#15998,#15999));
#3183=EDGE_LOOP('',(#16000,#16001,#16002,#16003));
#3184=EDGE_LOOP('',(#16004,#16005,#16006,#16007));
#3185=EDGE_LOOP('',(#16008,#16009,#16010,#16011));
#3186=EDGE_LOOP('',(#16012,#16013,#16014,#16015));
#3187=EDGE_LOOP('',(#16016,#16017,#16018,#16019));
#3188=EDGE_LOOP('',(#16020,#16021,#16022,#16023));
#3189=EDGE_LOOP('',(#16024,#16025,#16026,#16027));
#3190=EDGE_LOOP('',(#16028,#16029,#16030,#16031));
#3191=EDGE_LOOP('',(#16032,#16033,#16034,#16035));
#3192=EDGE_LOOP('',(#16036,#16037,#16038,#16039));
#3193=EDGE_LOOP('',(#16040,#16041,#16042,#16043));
#3194=EDGE_LOOP('',(#16044,#16045,#16046,#16047,#16048,#16049,#16050,#16051));
#3195=EDGE_LOOP('',(#16052,#16053,#16054,#16055));
#3196=EDGE_LOOP('',(#16056,#16057,#16058,#16059));
#3197=EDGE_LOOP('',(#16060,#16061,#16062,#16063));
#3198=EDGE_LOOP('',(#16064,#16065,#16066,#16067));
#3199=EDGE_LOOP('',(#16068,#16069,#16070,#16071));
#3200=EDGE_LOOP('',(#16072,#16073,#16074,#16075));
#3201=EDGE_LOOP('',(#16076,#16077,#16078,#16079));
#3202=EDGE_LOOP('',(#16080,#16081,#16082,#16083));
#3203=EDGE_LOOP('',(#16084,#16085,#16086,#16087));
#3204=EDGE_LOOP('',(#16088,#16089,#16090,#16091));
#3205=EDGE_LOOP('',(#16092,#16093,#16094,#16095));
#3206=EDGE_LOOP('',(#16096,#16097,#16098,#16099));
#3207=EDGE_LOOP('',(#16100,#16101,#16102,#16103));
#3208=EDGE_LOOP('',(#16104,#16105,#16106,#16107));
#3209=EDGE_LOOP('',(#16108,#16109,#16110,#16111));
#3210=EDGE_LOOP('',(#16112,#16113,#16114,#16115));
#3211=EDGE_LOOP('',(#16116,#16117,#16118,#16119));
#3212=EDGE_LOOP('',(#16120,#16121,#16122,#16123));
#3213=EDGE_LOOP('',(#16124,#16125,#16126,#16127));
#3214=EDGE_LOOP('',(#16128,#16129,#16130,#16131));
#3215=EDGE_LOOP('',(#16132,#16133,#16134,#16135));
#3216=EDGE_LOOP('',(#16136,#16137,#16138,#16139));
#3217=EDGE_LOOP('',(#16140,#16141,#16142,#16143));
#3218=EDGE_LOOP('',(#16144,#16145,#16146,#16147));
#3219=EDGE_LOOP('',(#16148,#16149,#16150,#16151));
#3220=EDGE_LOOP('',(#16152,#16153,#16154,#16155));
#3221=EDGE_LOOP('',(#16156,#16157,#16158,#16159));
#3222=EDGE_LOOP('',(#16160,#16161,#16162,#16163));
#3223=EDGE_LOOP('',(#16164,#16165,#16166,#16167));
#3224=EDGE_LOOP('',(#16168,#16169,#16170,#16171,#16172,#16173,#16174,#16175));
#3225=EDGE_LOOP('',(#16176,#16177,#16178,#16179));
#3226=EDGE_LOOP('',(#16180,#16181,#16182,#16183));
#3227=EDGE_LOOP('',(#16184,#16185,#16186,#16187));
#3228=EDGE_LOOP('',(#16188,#16189,#16190,#16191));
#3229=EDGE_LOOP('',(#16192,#16193,#16194,#16195));
#3230=EDGE_LOOP('',(#16196,#16197,#16198,#16199));
#3231=EDGE_LOOP('',(#16200,#16201,#16202,#16203));
#3232=EDGE_LOOP('',(#16204,#16205,#16206,#16207));
#3233=EDGE_LOOP('',(#16208,#16209,#16210,#16211));
#3234=EDGE_LOOP('',(#16212,#16213,#16214,#16215));
#3235=EDGE_LOOP('',(#16216,#16217,#16218,#16219));
#3236=EDGE_LOOP('',(#16220,#16221,#16222,#16223));
#3237=EDGE_LOOP('',(#16224,#16225,#16226,#16227));
#3238=EDGE_LOOP('',(#16228,#16229,#16230,#16231));
#3239=EDGE_LOOP('',(#16232,#16233,#16234,#16235));
#3240=EDGE_LOOP('',(#16236,#16237,#16238,#16239));
#3241=EDGE_LOOP('',(#16240,#16241,#16242,#16243));
#3242=EDGE_LOOP('',(#16244,#16245,#16246,#16247));
#3243=EDGE_LOOP('',(#16248,#16249,#16250,#16251));
#3244=EDGE_LOOP('',(#16252,#16253,#16254,#16255));
#3245=EDGE_LOOP('',(#16256,#16257,#16258,#16259));
#3246=EDGE_LOOP('',(#16260,#16261,#16262,#16263));
#3247=EDGE_LOOP('',(#16264,#16265,#16266,#16267));
#3248=EDGE_LOOP('',(#16268,#16269,#16270,#16271));
#3249=EDGE_LOOP('',(#16272,#16273,#16274,#16275));
#3250=EDGE_LOOP('',(#16276,#16277,#16278,#16279));
#3251=EDGE_LOOP('',(#16280,#16281,#16282,#16283));
#3252=EDGE_LOOP('',(#16284,#16285,#16286,#16287));
#3253=EDGE_LOOP('',(#16288,#16289,#16290,#16291));
#3254=EDGE_LOOP('',(#16292,#16293,#16294,#16295,#16296,#16297,#16298,#16299));
#3255=EDGE_LOOP('',(#16300,#16301,#16302,#16303));
#3256=EDGE_LOOP('',(#16304,#16305,#16306,#16307));
#3257=EDGE_LOOP('',(#16308,#16309,#16310,#16311));
#3258=EDGE_LOOP('',(#16312,#16313,#16314,#16315));
#3259=EDGE_LOOP('',(#16316,#16317,#16318,#16319));
#3260=EDGE_LOOP('',(#16320,#16321,#16322,#16323));
#3261=EDGE_LOOP('',(#16324,#16325,#16326,#16327));
#3262=EDGE_LOOP('',(#16328,#16329,#16330,#16331));
#3263=EDGE_LOOP('',(#16332,#16333,#16334,#16335));
#3264=EDGE_LOOP('',(#16336,#16337,#16338,#16339));
#3265=EDGE_LOOP('',(#16340,#16341,#16342,#16343));
#3266=EDGE_LOOP('',(#16344,#16345,#16346,#16347));
#3267=EDGE_LOOP('',(#16348,#16349,#16350,#16351));
#3268=EDGE_LOOP('',(#16352,#16353,#16354,#16355));
#3269=EDGE_LOOP('',(#16356,#16357,#16358,#16359));
#3270=EDGE_LOOP('',(#16360,#16361,#16362,#16363));
#3271=EDGE_LOOP('',(#16364,#16365,#16366,#16367));
#3272=EDGE_LOOP('',(#16368,#16369,#16370,#16371));
#3273=EDGE_LOOP('',(#16372,#16373,#16374,#16375));
#3274=EDGE_LOOP('',(#16376,#16377,#16378,#16379));
#3275=EDGE_LOOP('',(#16380,#16381,#16382,#16383));
#3276=EDGE_LOOP('',(#16384,#16385,#16386,#16387));
#3277=EDGE_LOOP('',(#16388,#16389,#16390,#16391));
#3278=EDGE_LOOP('',(#16392,#16393,#16394,#16395));
#3279=EDGE_LOOP('',(#16396,#16397,#16398,#16399));
#3280=EDGE_LOOP('',(#16400,#16401,#16402,#16403));
#3281=EDGE_LOOP('',(#16404,#16405,#16406,#16407));
#3282=EDGE_LOOP('',(#16408,#16409,#16410,#16411));
#3283=EDGE_LOOP('',(#16412,#16413,#16414,#16415));
#3284=EDGE_LOOP('',(#16416,#16417,#16418,#16419,#16420,#16421));
#3285=EDGE_LOOP('',(#16422,#16423,#16424,#16425,#16426,#16427));
#3286=EDGE_LOOP('',(#16428,#16429,#16430,#16431,#16432,#16433,#16434,#16435));
#3287=EDGE_LOOP('',(#16436,#16437,#16438,#16439,#16440,#16441));
#3288=EDGE_LOOP('',(#16442,#16443,#16444,#16445,#16446,#16447));
#3289=EDGE_LOOP('',(#16448,#16449,#16450,#16451,#16452,#16453));
#3290=EDGE_LOOP('',(#16454,#16455,#16456,#16457,#16458,#16459,#16460,#16461));
#3291=EDGE_LOOP('',(#16462,#16463,#16464,#16465,#16466,#16467));
#3292=EDGE_LOOP('',(#16468,#16469,#16470,#16471,#16472,#16473));
#3293=EDGE_LOOP('',(#16474,#16475,#16476,#16477,#16478,#16479));
#3294=EDGE_LOOP('',(#16480,#16481,#16482,#16483,#16484,#16485,#16486,#16487));
#3295=EDGE_LOOP('',(#16488,#16489,#16490,#16491,#16492,#16493));
#3296=EDGE_LOOP('',(#16494,#16495,#16496,#16497,#16498));
#3297=EDGE_LOOP('',(#16499,#16500,#16501,#16502));
#3298=EDGE_LOOP('',(#16503,#16504,#16505,#16506,#16507,#16508,#16509,#16510,
#16511,#16512,#16513,#16514,#16515,#16516,#16517,#16518,#16519,#16520,#16521,
#16522,#16523,#16524,#16525,#16526,#16527,#16528,#16529,#16530,#16531,#16532,
#16533,#16534,#16535,#16536));
#3299=EDGE_LOOP('',(#16537,#16538,#16539,#16540,#16541,#16542,#16543,#16544,
#16545,#16546,#16547,#16548,#16549,#16550,#16551,#16552,#16553,#16554,#16555,
#16556,#16557,#16558,#16559,#16560,#16561,#16562,#16563,#16564,#16565,#16566,
#16567,#16568,#16569,#16570));
#3300=EDGE_LOOP('',(#16571,#16572,#16573,#16574));
#3301=EDGE_LOOP('',(#16575,#16576,#16577,#16578,#16579));
#3302=EDGE_LOOP('',(#16580,#16581,#16582,#16583));
#3303=EDGE_LOOP('',(#16584,#16585,#16586,#16587,#16588,#16589,#16590,#16591,
#16592,#16593,#16594,#16595,#16596,#16597,#16598,#16599,#16600,#16601,#16602,
#16603,#16604,#16605,#16606,#16607,#16608,#16609,#16610,#16611,#16612,#16613,
#16614,#16615,#16616,#16617));
#3304=EDGE_LOOP('',(#16618,#16619,#16620,#16621,#16622,#16623,#16624,#16625,
#16626,#16627,#16628,#16629,#16630,#16631,#16632,#16633,#16634,#16635,#16636,
#16637,#16638,#16639,#16640,#16641,#16642,#16643,#16644,#16645,#16646,#16647,
#16648,#16649,#16650,#16651));
#3305=EDGE_LOOP('',(#16652,#16653,#16654,#16655));
#3306=EDGE_LOOP('',(#16656,#16657,#16658,#16659,#16660));
#3307=EDGE_LOOP('',(#16661,#16662,#16663,#16664));
#3308=EDGE_LOOP('',(#16665,#16666,#16667,#16668,#16669,#16670,#16671,#16672,
#16673,#16674,#16675,#16676,#16677,#16678,#16679,#16680,#16681,#16682,#16683,
#16684,#16685,#16686,#16687,#16688,#16689,#16690,#16691,#16692,#16693,#16694,
#16695,#16696,#16697,#16698));
#3309=EDGE_LOOP('',(#16699,#16700,#16701,#16702,#16703,#16704,#16705,#16706,
#16707,#16708,#16709,#16710,#16711,#16712,#16713,#16714,#16715,#16716,#16717,
#16718,#16719,#16720,#16721,#16722,#16723,#16724,#16725,#16726,#16727,#16728,
#16729,#16730,#16731,#16732));
#3310=EDGE_LOOP('',(#16733,#16734,#16735,#16736));
#3311=EDGE_LOOP('',(#16737,#16738,#16739,#16740,#16741));
#3312=EDGE_LOOP('',(#16742,#16743,#16744,#16745));
#3313=EDGE_LOOP('',(#16746,#16747,#16748,#16749,#16750,#16751,#16752,#16753,
#16754,#16755,#16756,#16757,#16758,#16759,#16760,#16761,#16762,#16763,#16764,
#16765,#16766,#16767,#16768,#16769,#16770,#16771,#16772,#16773,#16774,#16775,
#16776,#16777,#16778,#16779));
#3314=EDGE_LOOP('',(#16780,#16781,#16782,#16783,#16784,#16785,#16786,#16787,
#16788,#16789,#16790,#16791,#16792,#16793,#16794,#16795,#16796,#16797,#16798,
#16799,#16800,#16801,#16802,#16803,#16804,#16805,#16806,#16807,#16808,#16809,
#16810,#16811,#16812,#16813));
#3315=EDGE_LOOP('',(#16814,#16815,#16816,#16817));
#3316=EDGE_LOOP('',(#16818,#16819,#16820,#16821,#16822));
#3317=EDGE_LOOP('',(#16823,#16824,#16825,#16826));
#3318=EDGE_LOOP('',(#16827,#16828,#16829,#16830,#16831,#16832,#16833,#16834,
#16835,#16836,#16837,#16838,#16839,#16840,#16841,#16842,#16843,#16844,#16845,
#16846,#16847,#16848,#16849,#16850,#16851,#16852,#16853,#16854,#16855,#16856,
#16857,#16858,#16859,#16860));
#3319=EDGE_LOOP('',(#16861,#16862,#16863,#16864,#16865,#16866,#16867,#16868,
#16869,#16870,#16871,#16872,#16873,#16874,#16875,#16876,#16877,#16878,#16879,
#16880,#16881,#16882,#16883,#16884,#16885,#16886,#16887,#16888,#16889,#16890,
#16891,#16892,#16893,#16894));
#3320=EDGE_LOOP('',(#16895,#16896,#16897,#16898));
#3321=EDGE_LOOP('',(#16899,#16900,#16901,#16902,#16903));
#3322=EDGE_LOOP('',(#16904,#16905,#16906,#16907));
#3323=EDGE_LOOP('',(#16908,#16909,#16910,#16911,#16912,#16913,#16914,#16915,
#16916,#16917,#16918,#16919,#16920,#16921,#16922,#16923,#16924,#16925,#16926,
#16927,#16928,#16929,#16930,#16931,#16932,#16933,#16934,#16935,#16936,#16937,
#16938,#16939,#16940,#16941));
#3324=EDGE_LOOP('',(#16942,#16943,#16944,#16945,#16946,#16947,#16948,#16949,
#16950,#16951,#16952,#16953,#16954,#16955,#16956,#16957,#16958,#16959,#16960,
#16961,#16962,#16963,#16964,#16965,#16966,#16967,#16968,#16969,#16970,#16971,
#16972,#16973,#16974,#16975));
#3325=EDGE_LOOP('',(#16976,#16977,#16978,#16979));
#3326=EDGE_LOOP('',(#16980,#16981,#16982,#16983,#16984));
#3327=EDGE_LOOP('',(#16985,#16986,#16987,#16988));
#3328=EDGE_LOOP('',(#16989,#16990,#16991,#16992,#16993,#16994,#16995,#16996,
#16997,#16998,#16999,#17000,#17001,#17002,#17003,#17004,#17005,#17006,#17007,
#17008,#17009,#17010,#17011,#17012,#17013,#17014,#17015,#17016,#17017,#17018,
#17019,#17020,#17021,#17022));
#3329=EDGE_LOOP('',(#17023,#17024,#17025,#17026,#17027,#17028,#17029,#17030,
#17031,#17032,#17033,#17034,#17035,#17036,#17037,#17038,#17039,#17040,#17041,
#17042,#17043,#17044,#17045,#17046,#17047,#17048,#17049,#17050,#17051,#17052,
#17053,#17054,#17055,#17056));
#3330=EDGE_LOOP('',(#17057,#17058,#17059,#17060));
#3331=EDGE_LOOP('',(#17061,#17062,#17063,#17064,#17065));
#3332=EDGE_LOOP('',(#17066,#17067,#17068,#17069));
#3333=EDGE_LOOP('',(#17070,#17071,#17072,#17073,#17074,#17075,#17076,#17077,
#17078,#17079,#17080,#17081,#17082,#17083,#17084,#17085,#17086,#17087,#17088,
#17089,#17090,#17091,#17092,#17093,#17094,#17095,#17096,#17097,#17098,#17099,
#17100,#17101,#17102,#17103));
#3334=EDGE_LOOP('',(#17104,#17105,#17106,#17107,#17108,#17109,#17110,#17111,
#17112,#17113,#17114,#17115,#17116,#17117,#17118,#17119,#17120,#17121,#17122,
#17123,#17124,#17125,#17126,#17127,#17128,#17129,#17130,#17131,#17132,#17133,
#17134,#17135,#17136,#17137));
#3335=EDGE_LOOP('',(#17138,#17139,#17140,#17141));
#3336=EDGE_LOOP('',(#17142));
#3337=EDGE_LOOP('',(#17143));
#3338=EDGE_LOOP('',(#17144));
#3339=EDGE_LOOP('',(#17145));
#3340=EDGE_LOOP('',(#17146));
#3341=EDGE_LOOP('',(#17147));
#3342=EDGE_LOOP('',(#17148));
#3343=EDGE_LOOP('',(#17149));
#3344=EDGE_LOOP('',(#17150,#17151,#17152,#17153));
#3345=EDGE_LOOP('',(#17154,#17155,#17156,#17157));
#3346=EDGE_LOOP('',(#17158,#17159,#17160,#17161));
#3347=EDGE_LOOP('',(#17162,#17163,#17164,#17165));
#3348=EDGE_LOOP('',(#17166,#17167,#17168,#17169));
#3349=EDGE_LOOP('',(#17170));
#3350=EDGE_LOOP('',(#17171));
#3351=EDGE_LOOP('',(#17172,#17173,#17174,#17175,#17176,#17177,#17178,#17179,
#17180,#17181,#17182,#17183,#17184,#17185,#17186,#17187,#17188,#17189,#17190));
#3352=EDGE_LOOP('',(#17191,#17192));
#3353=EDGE_LOOP('',(#17193,#17194));
#3354=EDGE_LOOP('',(#17195));
#3355=EDGE_LOOP('',(#17196,#17197));
#3356=EDGE_LOOP('',(#17198,#17199));
#3357=EDGE_LOOP('',(#17200));
#3358=EDGE_LOOP('',(#17201,#17202));
#3359=EDGE_LOOP('',(#17203,#17204));
#3360=EDGE_LOOP('',(#17205));
#3361=EDGE_LOOP('',(#17206,#17207,#17208,#17209,#17210,#17211,#17212,#17213,
#17214,#17215,#17216,#17217,#17218,#17219,#17220,#17221,#17222,#17223,#17224));
#3362=EDGE_LOOP('',(#17225,#17226));
#3363=EDGE_LOOP('',(#17227,#17228));
#3364=EDGE_LOOP('',(#17229,#17230,#17231));
#3365=EDGE_LOOP('',(#17232,#17233));
#3366=EDGE_LOOP('',(#17234,#17235));
#3367=EDGE_LOOP('',(#17236,#17237,#17238));
#3368=EDGE_LOOP('',(#17239,#17240));
#3369=EDGE_LOOP('',(#17241,#17242));
#3370=EDGE_LOOP('',(#17243,#17244,#17245));
#3371=EDGE_LOOP('',(#17246));
#3372=EDGE_LOOP('',(#17247,#17248,#17249,#17250));
#3373=EDGE_LOOP('',(#17251,#17252,#17253,#17254));
#3374=EDGE_LOOP('',(#17255,#17256,#17257,#17258));
#3375=EDGE_LOOP('',(#17259,#17260,#17261,#17262));
#3376=EDGE_LOOP('',(#17263));
#3377=EDGE_LOOP('',(#17264,#17265,#17266,#17267));
#3378=EDGE_LOOP('',(#17268,#17269,#17270,#17271));
#3379=EDGE_LOOP('',(#17272,#17273,#17274,#17275));
#3380=EDGE_LOOP('',(#17276,#17277,#17278,#17279));
#3381=EDGE_LOOP('',(#17280));
#3382=EDGE_LOOP('',(#17281));
#3383=EDGE_LOOP('',(#17282));
#3384=EDGE_LOOP('',(#17283));
#3385=EDGE_LOOP('',(#17284));
#3386=EDGE_LOOP('',(#17285));
#3387=EDGE_LOOP('',(#17286,#17287,#17288,#17289));
#3388=EDGE_LOOP('',(#17290,#17291,#17292,#17293));
#3389=EDGE_LOOP('',(#17294));
#3390=EDGE_LOOP('',(#17295));
#3391=EDGE_LOOP('',(#17296));
#3392=EDGE_LOOP('',(#17297));
#3393=EDGE_LOOP('',(#17298));
#3394=EDGE_LOOP('',(#17299));
#3395=EDGE_LOOP('',(#17300));
#3396=EDGE_LOOP('',(#17301));
#4505=CIRCLE('',#25394,2.5175);
#4506=CIRCLE('',#25395,2.5175);
#4507=CIRCLE('',#25396,2.5175);
#4508=CIRCLE('',#25411,2.5175);
#4509=CIRCLE('',#25413,3.07349999999999);
#4510=CIRCLE('',#25428,3.0735);
#4511=CIRCLE('',#25430,2.5175);
#4512=CIRCLE('',#25431,2.5175);
#4513=CIRCLE('',#25432,2.5175);
#4514=CIRCLE('',#25447,2.5175);
#4515=CIRCLE('',#25449,3.07349999999999);
#4516=CIRCLE('',#25464,3.0735);
#4517=CIRCLE('',#25466,2.5175);
#4518=CIRCLE('',#25467,2.5175);
#4519=CIRCLE('',#25468,2.5175);
#4520=CIRCLE('',#25483,2.5175);
#4521=CIRCLE('',#25485,3.0735);
#4522=CIRCLE('',#25500,3.0735);
#4523=CIRCLE('',#25502,2.5175);
#4524=CIRCLE('',#25503,2.5175);
#4525=CIRCLE('',#25504,2.5175);
#4526=CIRCLE('',#25519,2.5175);
#4527=CIRCLE('',#25521,3.07349999999999);
#4528=CIRCLE('',#25536,3.0735);
#4529=CIRCLE('',#25538,2.5175);
#4530=CIRCLE('',#25539,2.5175);
#4531=CIRCLE('',#25540,2.5175);
#4532=CIRCLE('',#25555,2.5175);
#4533=CIRCLE('',#25557,3.0735);
#4534=CIRCLE('',#25572,3.0735);
#4535=CIRCLE('',#25574,2.5175);
#4536=CIRCLE('',#25575,2.5175);
#4537=CIRCLE('',#25576,2.5175);
#4538=CIRCLE('',#25591,2.5175);
#4539=CIRCLE('',#25593,3.07349999999999);
#4540=CIRCLE('',#25608,3.0735);
#4541=CIRCLE('',#25610,2.5175);
#4542=CIRCLE('',#25611,2.5175);
#4543=CIRCLE('',#25612,2.5175);
#4544=CIRCLE('',#25627,2.5175);
#4545=CIRCLE('',#25629,3.0735);
#4546=CIRCLE('',#25644,3.0735);
#4547=CIRCLE('',#25646,2.5175);
#4548=CIRCLE('',#25647,2.5175);
#4549=CIRCLE('',#25648,2.5175);
#4550=CIRCLE('',#25663,2.5175);
#4551=CIRCLE('',#25665,3.0735);
#4552=CIRCLE('',#25680,3.0735);
#4553=CIRCLE('',#25726,5.5);
#4554=CIRCLE('',#25727,5.5);
#4555=CIRCLE('',#25729,5.5);
#4556=CIRCLE('',#25730,5.5);
#4557=CIRCLE('',#25732,5.5);
#4558=CIRCLE('',#25733,5.5);
#4559=CIRCLE('',#25735,5.5);
#4560=CIRCLE('',#25736,5.5);
#4561=CIRCLE('',#25738,18.);
#4562=CIRCLE('',#25739,18.);
#4563=CIRCLE('',#25741,17.);
#4564=CIRCLE('',#25743,90.);
#4565=CIRCLE('',#25744,90.);
#4566=CIRCLE('',#25746,100.);
#4567=CIRCLE('',#25747,100.);
#4568=CIRCLE('',#25750,140.);
#4569=CIRCLE('',#25752,17.);
#4570=CIRCLE('',#25754,140.);
#5385=B_SPLINE_CURVE_WITH_KNOTS('',3,(#32412,#32413,#32414,#32415),
 .UNSPECIFIED.,.F.,.F.,(4,4),(95.5573427486707,96.2647245007224),
 .UNSPECIFIED.);
#5386=B_SPLINE_CURVE_WITH_KNOTS('',3,(#32423,#32424,#32425,#32426,#32427,
#32428,#32429,#32430,#32431,#32432),.UNSPECIFIED.,.F.,.F.,(4,3,3,4),(-94.2477796076938,
-93.2874649800815,-92.2950451398679,-91.8135687061554),.UNSPECIFIED.);
#5387=B_SPLINE_CURVE_WITH_KNOTS('',3,(#32437,#32438,#32439,#32440,#32441,
#32442,#32443,#32444,#32445,#32446,#32447,#32448,#32449,#32450,#32451,#32452,
#32453,#32454,#32455,#32456,#32457,#32458,#32459,#32460,#32461),
 .UNSPECIFIED.,.F.,.F.,(4,3,3,3,3,3,3,3,4),(89.2741574414911,89.317785619227,
90.3102054594406,91.3026252996542,92.2950451398679,93.2874649800815,94.2798848202951,
95.2723046605088,95.5573427486707),.UNSPECIFIED.);
#5388=B_SPLINE_CURVE_WITH_KNOTS('',3,(#32462,#32463,#32464,#32465,#32466,
#32467,#32468,#32469,#32470,#32471,#32472,#32473,#32474,#32475,#32476,#32477,
#32478,#32479,#32480,#32481,#32482,#32483),.UNSPECIFIED.,.F.,.F.,(4,3,3,
3,3,3,3,4),(-91.8135687061554,-91.3026252996542,-90.3102054594406,-89.317785619227,
-88.3253657790133,-87.3329459387997,-86.3405260985861,-85.5303833989757),
 .UNSPECIFIED.);
#5389=B_SPLINE_CURVE_WITH_KNOTS('',3,(#32488,#32489,#32490,#32491,#32492,
#32493,#32494,#32495,#32496,#32497,#32498,#32499,#32500,#32501,#32502,#32503,
#32504,#32505,#32506,#32507,#32508,#32509),.UNSPECIFIED.,.F.,.F.,(4,3,3,
3,3,3,3,4),(82.9909721343116,83.3632665779452,84.3556864181588,85.3481062583724,
86.3405260985861,87.3329459387997,88.3253657790133,89.2741574414911),
 .UNSPECIFIED.);
#5390=B_SPLINE_CURVE_WITH_KNOTS('',3,(#32510,#32511,#32512,#32513,#32514,
#32515,#32516,#32517,#32518,#32519,#32520,#32521,#32522,#32523,#32524,#32525,
#32526,#32527,#32528,#32529,#32530,#32531,#32532,#32533,#32534),
 .UNSPECIFIED.,.F.,.F.,(4,3,3,3,3,3,3,3,4),(-85.5303833989757,-85.3481062583724,
-84.3556864181588,-83.3632665779452,-82.3708467377315,-81.3784268975179,
-80.3860070573043,-79.3935872170906,-79.2471980917961),.UNSPECIFIED.);
#5391=B_SPLINE_CURVE_WITH_KNOTS('',3,(#32539,#32540,#32541,#32542,#32543,
#32544,#32545,#32546,#32547,#32548,#32549,#32550,#32551,#32552,#32553,#32554,
#32555,#32556,#32557,#32558,#32559,#32560),.UNSPECIFIED.,.F.,.F.,(4,3,3,
3,3,3,3,4),(76.7077868271319,77.4087475366634,78.401167376877,79.3935872170906,
80.3860070573043,81.3784268975179,82.3708467377315,82.9909721343116),
 .UNSPECIFIED.);
#5392=B_SPLINE_CURVE_WITH_KNOTS('',3,(#32561,#32562,#32563,#32564,#32565,
#32566,#32567,#32568,#32569,#32570,#32571,#32572,#32573,#32574,#32575,#32576,
#32577,#32578,#32579,#32580,#32581,#32582),.UNSPECIFIED.,.F.,.F.,(4,3,3,
3,3,3,3,4),(-79.2471980917961,-78.401167376877,-77.4087475366633,-76.4163276964497,
-75.4239078562361,-74.4314880160224,-73.4390681758088,-72.9640127846165),
 .UNSPECIFIED.);
#5393=B_SPLINE_CURVE_WITH_KNOTS('',3,(#32587,#32588,#32589,#32590,#32591,
#32592,#32593,#32594,#32595,#32596,#32597,#32598,#32599,#32600,#32601,#32602,
#32603,#32604,#32605,#32606,#32607,#32608,#32609,#32610,#32611),
 .UNSPECIFIED.,.F.,.F.,(4,3,3,3,3,3,3,3,4),(70.4246015199523,70.4618086551679,
71.4542284953816,72.4466483355952,73.4390681758088,74.4314880160225,75.4239078562361,
76.4163276964497,76.7077868271319),.UNSPECIFIED.);
#5394=B_SPLINE_CURVE_WITH_KNOTS('',3,(#32612,#32613,#32614,#32615,#32616,
#32617,#32618,#32619,#32620,#32621,#32622,#32623,#32624,#32625,#32626,#32627,
#32628,#32629,#32630,#32631,#32632,#32633),.UNSPECIFIED.,.F.,.F.,(4,3,3,
3,3,3,3,4),(-72.9640127846165,-72.4466483355952,-71.4542284953815,-70.4618086551679,
-69.4693888149543,-68.4769689747406,-67.484549134527,-66.680827477437),
 .UNSPECIFIED.);
#5395=B_SPLINE_CURVE_WITH_KNOTS('',3,(#32638,#32639,#32640,#32641,#32642,
#32643,#32644,#32645,#32646,#32647,#32648,#32649,#32650,#32651,#32652,#32653,
#32654,#32655,#32656,#32657,#32658,#32659),.UNSPECIFIED.,.F.,.F.,(4,3,3,
3,3,3,3,4),(64.1414162127728,64.5072896138861,65.4997094540998,66.4921292943134,
67.484549134527,68.4769689747407,69.4693888149543,70.4246015199523),
 .UNSPECIFIED.);
#5396=B_SPLINE_CURVE_WITH_KNOTS('',3,(#32660,#32661,#32662,#32663,#32664,
#32665,#32666,#32667,#32668,#32669,#32670,#32671,#32672,#32673,#32674,#32675,
#32676,#32677,#32678,#32679,#32680,#32681,#32682,#32683,#32684),
 .UNSPECIFIED.,.F.,.F.,(4,3,3,3,3,3,3,3,4),(-66.680827477437,-66.4921292943134,
-65.4997094540998,-64.5072896138861,-63.5148697736725,-62.5224499334589,
-61.5300300932452,-60.5376102530316,-60.3976421702573),.UNSPECIFIED.);
#5397=B_SPLINE_CURVE_WITH_KNOTS('',3,(#32689,#32690,#32691,#32692,#32693,
#32694,#32695,#32696,#32697,#32698,#32699,#32700,#32701,#32702,#32703,#32704,
#32705,#32706,#32707,#32708,#32709,#32710),.UNSPECIFIED.,.F.,.F.,(4,3,3,
3,3,3,3,4),(57.8582309055932,58.5527705726043,59.545190412818,60.5376102530316,
61.5300300932452,62.5224499334589,63.5148697736725,64.1414162127728),
 .UNSPECIFIED.);
#5398=B_SPLINE_CURVE_WITH_KNOTS('',3,(#32711,#32712,#32713,#32714,#32715,
#32716,#32717,#32718,#32719,#32720,#32721,#32722,#32723,#32724,#32725,#32726,
#32727,#32728,#32729,#32730,#32731,#32732),.UNSPECIFIED.,.F.,.F.,(4,3,3,
3,3,3,3,4),(-60.3976421702573,-59.545190412818,-58.5527705726043,-57.5603507323907,
-56.5679308921771,-55.5755110519634,-54.5830912117498,-54.1144568630777),
 .UNSPECIFIED.);
#5399=B_SPLINE_CURVE_WITH_KNOTS('',3,(#32737,#32738,#32739,#32740,#32741,
#32742,#32743,#32744,#32745,#32746,#32747,#32748,#32749,#32750,#32751,#32752,
#32753,#32754,#32755,#32756,#32757,#32758,#32759,#32760,#32761),
 .UNSPECIFIED.,.F.,.F.,(4,3,3,3,3,3,3,3,4),(51.5750455984135,51.6058316911089,
52.5982515313225,53.5906713715362,54.5830912117498,55.5755110519634,56.5679308921771,
57.5603507323907,57.8582309055932),.UNSPECIFIED.);
#5400=B_SPLINE_CURVE_WITH_KNOTS('',3,(#32762,#32763,#32764,#32765,#32766,
#32767,#32768,#32769,#32770,#32771,#32772,#32773,#32774,#32775,#32776,#32777,
#32778,#32779,#32780,#32781,#32782,#32783),.UNSPECIFIED.,.F.,.F.,(4,3,3,
3,3,3,3,4),(-54.1144568630777,-53.5906713715362,-52.5982515313225,-51.6058316911089,
-50.6134118508953,-49.6209920106816,-48.628572170468,-47.8312715558982),
 .UNSPECIFIED.);
#5401=B_SPLINE_CURVE_WITH_KNOTS('',3,(#32788,#32789,#32790,#32791,#32792,
#32793,#32794,#32795,#32796,#32797,#32798,#32799,#32800,#32801,#32802,#32803,
#32804,#32805,#32806,#32807,#32808,#32809),.UNSPECIFIED.,.F.,.F.,(4,3,3,
3,3,3,3,4),(45.291860291234,45.6513126498271,46.6437324900407,47.6361523302544,
48.628572170468,49.6209920106816,50.6134118508953,51.5750455984135),
 .UNSPECIFIED.);
#5402=B_SPLINE_CURVE_WITH_KNOTS('',3,(#32810,#32811,#32812,#32813,#32814,
#32815,#32816,#32817,#32818,#32819,#32820,#32821,#32822,#32823,#32824,#32825,
#32826,#32827,#32828,#32829,#32830,#32831,#32832,#32833,#32834),
 .UNSPECIFIED.,.F.,.F.,(4,3,3,3,3,3,3,3,4),(-47.8312715558982,-47.6361523302544,
-46.6437324900407,-45.6513126498271,-44.6588928096135,-43.6664729693998,
-42.6740531291862,-41.6816332889726,-41.5480862487186),.UNSPECIFIED.);
#5403=B_SPLINE_CURVE_WITH_KNOTS('',3,(#32839,#32840,#32841,#32842,#32843,
#32844,#32845,#32846,#32847,#32848,#32849,#32850,#32851,#32852,#32853,#32854,
#32855,#32856,#32857,#32858,#32859,#32860),.UNSPECIFIED.,.F.,.F.,(4,3,3,
3,3,3,3,4),(39.0086749840544,39.6967936085453,40.6892134487589,41.6816332889726,
42.6740531291862,43.6664729693998,44.6588928096135,45.291860291234),
 .UNSPECIFIED.);
#5404=B_SPLINE_CURVE_WITH_KNOTS('',3,(#32861,#32862,#32863,#32864,#32865,
#32866,#32867,#32868,#32869,#32870,#32871,#32872,#32873,#32874,#32875,#32876,
#32877,#32878,#32879,#32880,#32881,#32882),.UNSPECIFIED.,.F.,.F.,(4,3,3,
3,3,3,3,4),(-41.5480862487186,-40.6892134487589,-39.6967936085453,-38.7043737683317,
-37.711953928118,-36.7195340879044,-35.7271142476908,-35.2649009415389),
 .UNSPECIFIED.);
#5405=B_SPLINE_CURVE_WITH_KNOTS('',3,(#32887,#32888,#32889,#32890,#32891,
#32892,#32893,#32894,#32895,#32896,#32897,#32898,#32899,#32900,#32901,#32902,
#32903,#32904,#32905,#32906,#32907,#32908,#32909,#32910,#32911),
 .UNSPECIFIED.,.F.,.F.,(4,3,3,3,3,3,3,3,4),(32.7254896768748,32.7498547270499,
33.7422745672635,34.7346944074771,35.7271142476908,36.7195340879044,37.711953928118,
38.7043737683317,39.0086749840544),.UNSPECIFIED.);
#5406=B_SPLINE_CURVE_WITH_KNOTS('',3,(#32912,#32913,#32914,#32915,#32916,
#32917,#32918,#32919,#32920,#32921,#32922,#32923,#32924,#32925,#32926,#32927,
#32928,#32929,#32930,#32931,#32932,#32933),.UNSPECIFIED.,.F.,.F.,(4,3,3,
3,3,3,3,4),(-35.2649009415389,-34.7346944074771,-33.7422745672635,-32.7498547270499,
-31.7574348868362,-30.7650150466226,-29.772595206409,-28.9817156343594),
 .UNSPECIFIED.);
#5407=B_SPLINE_CURVE_WITH_KNOTS('',3,(#32938,#32939,#32940,#32941,#32942,
#32943,#32944,#32945,#32946,#32947,#32948,#32949,#32950,#32951,#32952,#32953,
#32954,#32955,#32956,#32957,#32958,#32959),.UNSPECIFIED.,.F.,.F.,(4,3,3,
3,3,3,3,4),(26.4423043696952,26.7953356857681,27.7877555259817,28.7801753661954,
29.772595206409,30.7650150466226,31.7574348868363,32.7254896768748),
 .UNSPECIFIED.);
#5408=B_SPLINE_CURVE_WITH_KNOTS('',3,(#32960,#32961,#32962,#32963,#32964,
#32965,#32966,#32967,#32968,#32969,#32970,#32971,#32972,#32973,#32974,#32975,
#32976,#32977,#32978,#32979,#32980,#32981,#32982,#32983,#32984),
 .UNSPECIFIED.,.F.,.F.,(4,3,3,3,3,3,3,3,4),(-28.9817156343594,-28.7801753661953,
-27.7877555259817,-26.7953356857681,-25.8029158455544,-24.8104960053408,
-23.8180761651272,-22.8256563249135,-22.6985303271798),.UNSPECIFIED.);
#5409=B_SPLINE_CURVE_WITH_KNOTS('',3,(#32989,#32990,#32991,#32992,#32993,
#32994,#32995,#32996,#32997,#32998,#32999,#33000,#33001,#33002,#33003,#33004,
#33005,#33006,#33007,#33008,#33009,#33010),.UNSPECIFIED.,.F.,.F.,(4,3,3,
3,3,3,3,4),(20.1591190625156,20.8408166444863,21.8332364846999,22.8256563249136,
23.8180761651272,24.8104960053408,25.8029158455545,26.4423043696952),
 .UNSPECIFIED.);
#5410=B_SPLINE_CURVE_WITH_KNOTS('',3,(#33011,#33012,#33013,#33014,#33015,
#33016,#33017,#33018,#33019,#33020,#33021,#33022,#33023,#33024,#33025,#33026,
#33027,#33028,#33029,#33030,#33031,#33032),.UNSPECIFIED.,.F.,.F.,(4,3,3,
3,3,3,3,4),(-22.6985303271798,-21.8332364846999,-20.8408166444863,-19.8483968042727,
-18.855976964059,-17.8635571238454,-16.8711372836318,-16.4153450200002),
 .UNSPECIFIED.);
#5411=B_SPLINE_CURVE_WITH_KNOTS('',3,(#33037,#33038,#33039,#33040,#33041,
#33042,#33043,#33044,#33045,#33046,#33047,#33048,#33049,#33050,#33051,#33052,
#33053,#33054,#33055,#33056,#33057,#33058,#33059,#33060,#33061),
 .UNSPECIFIED.,.F.,.F.,(4,3,3,3,3,3,3,3,4),(13.875933755336,13.8938777629909,
14.8862976032045,15.8787174434181,16.8711372836318,17.8635571238454,18.855976964059,
19.8483968042727,20.1591190625156),.UNSPECIFIED.);
#5412=B_SPLINE_CURVE_WITH_KNOTS('',3,(#33062,#33063,#33064,#33065,#33066,
#33067,#33068,#33069,#33070,#33071,#33072,#33073,#33074,#33075,#33076,#33077,
#33078,#33079,#33080,#33081,#33082,#33083),.UNSPECIFIED.,.F.,.F.,(4,3,3,
3,3,3,3,4),(-16.4153450200002,-15.8787174434181,-14.8862976032045,-13.8938777629909,
-12.9014579227772,-11.9090380825636,-10.91661824235,-10.1321597128207),
 .UNSPECIFIED.);
#5413=B_SPLINE_CURVE_WITH_KNOTS('',3,(#33089,#33090,#33091,#33092,#33093,
#33094,#33095,#33096,#33097,#33098,#33099,#33100,#33101),.UNSPECIFIED.,
 .F.,.F.,(4,3,3,3,4),(-3.848974405641,-2.9772595206409,-1.98483968042726,
-0.992419840213632,0.),.UNSPECIFIED.);
#5414=B_SPLINE_CURVE_WITH_KNOTS('',3,(#33104,#33105,#33106,#33107,#33108,
#33109,#33110,#33111,#33112,#33113,#33114,#33115,#33116,#33117,#33118,#33119,
#33120,#33121,#33122),.UNSPECIFIED.,.F.,.F.,(4,3,3,3,3,3,4),(2.01694489302852,
2.9772595206409,3.96967936085453,4.96209920106817,5.9545190412818,6.94693888149543,
7.59274844815647),.UNSPECIFIED.);
#5415=B_SPLINE_CURVE_WITH_KNOTS('',3,(#33128,#33129,#33130,#33131,#33132,
#33133,#33134,#33135),.UNSPECIFIED.,.F.,.F.,(4,1,1,1,1,4),(103.672557568463,
104.154034002176,105.146453842389,106.138873682603,107.131293522817,108.12371336303),
 .UNSPECIFIED.);
#5416=B_SPLINE_CURVE_WITH_KNOTS('',3,(#33138,#33139,#33140,#33141,#33142,
#33143,#33144,#33145,#33146),.UNSPECIFIED.,.F.,.F.,(4,1,1,1,1,1,4),(103.672557568463,
103.716185746199,104.708605586413,105.701025426626,106.69344526684,107.685865107053,
108.646179734666),.UNSPECIFIED.);
#5417=B_SPLINE_CURVE_WITH_KNOTS('',3,(#33151,#33152,#33153,#33154,#33155,
#33156,#33157,#33158,#33159,#33160),.UNSPECIFIED.,.F.,.F.,(4,1,1,1,1,1,
1,4),(97.3893722612835,98.1995149608939,99.1919348011075,100.184354641321,
101.176774481535,102.169194321748,103.161614161962,103.672557568463),
 .UNSPECIFIED.);
#5418=B_SPLINE_CURVE_WITH_KNOTS('',3,(#33161,#33162,#33163,#33164,#33165,
#33166,#33167,#33168,#33169,#33170),.UNSPECIFIED.,.F.,.F.,(4,1,1,1,1,1,
1,4),(97.3893722612835,97.7616667049171,98.7540865451307,99.7465063853444,
100.738926225558,101.731346065772,102.723765905985,103.672557568463),
 .UNSPECIFIED.);
#5419=B_SPLINE_CURVE_WITH_KNOTS('',3,(#33175,#33176,#33177,#33178,#33179,
#33180,#33181,#33182,#33183,#33184,#33185),.UNSPECIFIED.,.F.,.F.,(4,1,1,
1,1,1,1,1,4),(91.106186954104,91.2525760793984,92.2449959196121,93.2374157598257,
94.2298356000393,95.222255440253,96.2146752804666,97.2070951206802,97.3893722612835),
 .UNSPECIFIED.);
#5420=B_SPLINE_CURVE_WITH_KNOTS('',3,(#33186,#33187,#33188,#33189,#33190,
#33191,#33192,#33193,#33194,#33195),.UNSPECIFIED.,.F.,.F.,(4,1,1,1,1,1,
1,4),(91.106186954104,91.8071476636353,92.7995675038489,93.7919873440626,
94.7844071842762,95.7768270244898,96.7692468647035,97.3893722612835),
 .UNSPECIFIED.);
#5421=B_SPLINE_CURVE_WITH_KNOTS('',3,(#33200,#33201,#33202,#33203,#33204,
#33205,#33206,#33207,#33208,#33209),.UNSPECIFIED.,.F.,.F.,(4,1,1,1,1,1,
1,4),(84.8230016469244,85.2980570381166,86.2904768783303,87.2828967185439,
88.2753165587575,89.2677363989712,90.2601562391848,91.106186954104),
 .UNSPECIFIED.);
#5422=B_SPLINE_CURVE_WITH_KNOTS('',3,(#33210,#33211,#33212,#33213,#33214,
#33215,#33216,#33217,#33218,#33219,#33220),.UNSPECIFIED.,.F.,.F.,(4,1,1,
1,1,1,1,1,4),(84.8230016469244,84.8602087821399,85.8526286223535,86.8450484625671,
87.8374683027808,88.8298881429944,89.822307983208,90.8147278234217,91.106186954104),
 .UNSPECIFIED.);
#5423=B_SPLINE_CURVE_WITH_KNOTS('',3,(#33225,#33226,#33227,#33228,#33229,
#33230,#33231,#33232,#33233,#33234),.UNSPECIFIED.,.F.,.F.,(4,1,1,1,1,1,
1,4),(78.5398163397448,79.3435379968348,80.3359578370485,81.3283776772621,
82.3207975174757,83.3132173576894,84.305637197903,84.8230016469244),
 .UNSPECIFIED.);
#5424=B_SPLINE_CURVE_WITH_KNOTS('',3,(#33235,#33236,#33237,#33238,#33239,
#33240,#33241,#33242,#33243,#33244),.UNSPECIFIED.,.F.,.F.,(4,1,1,1,1,1,
1,4),(78.5398163397448,78.9056897408581,79.8981095810717,80.8905294212853,
81.882949261499,82.8753691017126,83.8677889419262,84.8230016469244),
 .UNSPECIFIED.);
#5425=B_SPLINE_CURVE_WITH_KNOTS('',3,(#33249,#33250,#33251,#33252,#33253,
#33254,#33255,#33256,#33257,#33258,#33259),.UNSPECIFIED.,.F.,.F.,(4,1,1,
1,1,1,1,1,4),(72.2566310325653,72.3965991153394,73.389018955553,74.3814387957667,
75.3738586359803,76.3662784761939,77.3586983164076,78.3511181566212,78.5398163397448),
 .UNSPECIFIED.);
#5426=B_SPLINE_CURVE_WITH_KNOTS('',3,(#33260,#33261,#33262,#33263,#33264,
#33265,#33266,#33267,#33268,#33269),.UNSPECIFIED.,.F.,.F.,(4,1,1,1,1,1,
1,4),(72.2566310325651,72.9511706995763,73.9435905397899,74.9360103800035,
75.9284302202172,76.9208500604308,77.9132699006444,78.5398163397448),
 .UNSPECIFIED.);
#5427=B_SPLINE_CURVE_WITH_KNOTS('',3,(#33274,#33275,#33276,#33277,#33278,
#33279,#33280,#33281,#33282,#33283),.UNSPECIFIED.,.F.,.F.,(4,1,1,1,1,1,
1,4),(65.9734457253856,66.4420800740576,67.4344999142712,68.4269197544849,
69.4193395946985,70.4117594349121,71.4041792751258,72.2566310325653),
 .UNSPECIFIED.);
#5428=B_SPLINE_CURVE_WITH_KNOTS('',3,(#33284,#33285,#33286,#33287,#33288,
#33289,#33290,#33291,#33292,#33293,#33294),.UNSPECIFIED.,.F.,.F.,(4,1,1,
1,1,1,1,1,4),(65.9734457253856,66.0042318180808,66.9966516582945,67.9890714985081,
68.9814913387217,69.9739111789354,70.966331019149,71.9587508593626,72.2566310325651),
 .UNSPECIFIED.);
#5429=B_SPLINE_CURVE_WITH_KNOTS('',3,(#33299,#33300,#33301,#33302,#33303,
#33304,#33305,#33306,#33307,#33308),.UNSPECIFIED.,.F.,.F.,(4,1,1,1,1,1,
1,4),(59.690260418206,60.4875610327758,61.4799808729895,62.4724007132031,
63.4648205534167,64.4572403936303,65.449660233844,65.9734457253856),
 .UNSPECIFIED.);
#5430=B_SPLINE_CURVE_WITH_KNOTS('',3,(#33309,#33310,#33311,#33312,#33313,
#33314,#33315,#33316,#33317,#33318),.UNSPECIFIED.,.F.,.F.,(4,1,1,1,1,1,
1,4),(59.690260418206,60.049712776799,61.0421326170127,62.0345524572263,
63.0269722974399,64.0193921376536,65.0118119778672,65.9734457253856),
 .UNSPECIFIED.);
#5431=B_SPLINE_CURVE_WITH_KNOTS('',3,(#33323,#33324,#33325,#33326,#33327,
#33328,#33329,#33330,#33331,#33332,#33333),.UNSPECIFIED.,.F.,.F.,(4,1,1,
1,1,1,1,1,4),(53.4070751110265,53.5406221512804,54.533041991494,55.5254618317077,
56.5178816719213,57.5103015121349,58.5027213523486,59.4951411925622,59.690260418206),
 .UNSPECIFIED.);
#5432=B_SPLINE_CURVE_WITH_KNOTS('',3,(#33334,#33335,#33336,#33337,#33338,
#33339,#33340,#33341,#33342,#33343),.UNSPECIFIED.,.F.,.F.,(4,1,1,1,1,1,
1,4),(53.4070751110265,54.0951937355172,55.0876135757309,56.0800334159445,
57.0724532561581,58.0648730963718,59.0572929365854,59.690260418206),
 .UNSPECIFIED.);
#5433=B_SPLINE_CURVE_WITH_KNOTS('',3,(#33348,#33349,#33350,#33351,#33352,
#33353,#33354,#33355,#33356,#33357),.UNSPECIFIED.,.F.,.F.,(4,1,1,1,1,1,
1,4),(47.1238898038468,47.5861031099986,48.5785229502122,49.5709427904259,
50.5633626306395,51.5557824708531,52.5482023110668,53.4070751110265),
 .UNSPECIFIED.);
#5434=B_SPLINE_CURVE_WITH_KNOTS('',3,(#33358,#33359,#33360,#33361,#33362,
#33363,#33364,#33365,#33366,#33367,#33368),.UNSPECIFIED.,.F.,.F.,(4,1,1,
1,1,1,1,1,4),(47.1238898038468,47.1482548540218,48.1406746942354,49.1330945344491,
50.1255143746627,51.1179342148763,52.11035405509,53.1027738953036,53.4070751110265),
 .UNSPECIFIED.);
#5435=B_SPLINE_CURVE_WITH_KNOTS('',3,(#33373,#33374,#33375,#33376,#33377,
#33378,#33379,#33380,#33381,#33382),.UNSPECIFIED.,.F.,.F.,(4,1,1,1,1,1,
1,4),(40.8407044966672,41.6315840687168,42.6240039089304,43.6164237491441,
44.6088435893577,45.6012634295713,46.593683269785,47.1238898038468),
 .UNSPECIFIED.);
#5436=B_SPLINE_CURVE_WITH_KNOTS('',3,(#33383,#33384,#33385,#33386,#33387,
#33388,#33389,#33390,#33391,#33392),.UNSPECIFIED.,.F.,.F.,(4,1,1,1,1,1,
1,4),(40.8407044966672,41.19373581274,42.1861556529536,43.1785754931673,
44.1709953333809,45.1634151735945,46.1558350138082,47.1238898038468),
 .UNSPECIFIED.);
#5437=B_SPLINE_CURVE_WITH_KNOTS('',3,(#33397,#33398,#33399,#33400,#33401,
#33402,#33403,#33404,#33405,#33406,#33407),.UNSPECIFIED.,.F.,.F.,(4,1,1,
1,1,1,1,1,4),(34.5575191894877,34.6846451872214,35.677065027435,36.6694848676486,
37.6619047078623,38.6543245480759,39.6467443882895,40.6391642285032,40.8407044966672),
 .UNSPECIFIED.);
#5438=B_SPLINE_CURVE_WITH_KNOTS('',3,(#33408,#33409,#33410,#33411,#33412,
#33413,#33414,#33415,#33416,#33417),.UNSPECIFIED.,.F.,.F.,(4,1,1,1,1,1,
1,4),(34.5575191894877,35.2392167714582,36.2316366116718,37.2240564518855,
38.2164762920991,39.2088961323127,40.2013159725264,40.8407044966672),
 .UNSPECIFIED.);
#5439=B_SPLINE_CURVE_WITH_KNOTS('',3,(#33422,#33423,#33424,#33425,#33426,
#33427,#33428,#33429,#33430,#33431),.UNSPECIFIED.,.F.,.F.,(4,1,1,1,1,1,
1,4),(28.2743338823081,28.7301261459396,29.7225459861532,30.7149658263668,
31.7073856665805,32.6998055067941,33.6922253470077,34.5575191894877),
 .UNSPECIFIED.);
#5440=B_SPLINE_CURVE_WITH_KNOTS('',3,(#33432,#33433,#33434,#33435,#33436,
#33437,#33438,#33439,#33440,#33441,#33442),.UNSPECIFIED.,.F.,.F.,(4,1,1,
1,1,1,1,1,4),(28.2743338823081,28.2922778899628,29.2846977301764,30.2771175703901,
31.2695374106037,32.2619572508173,33.2543770910309,34.2467969312446,34.5575191894877),
 .UNSPECIFIED.);
#5441=B_SPLINE_CURVE_WITH_KNOTS('',3,(#33447,#33448,#33449,#33450,#33451,
#33452,#33453,#33454,#33455,#33456),.UNSPECIFIED.,.F.,.F.,(4,1,1,1,1,1,
1,4),(21.9911485751285,22.7756071046578,23.7680269448714,24.760446785085,
25.7528666252987,26.7452864655123,27.7377063057259,28.2743338823081),
 .UNSPECIFIED.);
#5442=B_SPLINE_CURVE_WITH_KNOTS('',3,(#33457,#33458,#33459,#33460,#33461,
#33462,#33463,#33464,#33465,#33466),.UNSPECIFIED.,.F.,.F.,(4,1,1,1,1,1,
1,4),(21.9911485751284,22.337758848681,23.3301786888946,24.3225985291083,
25.3150183693219,26.3074382095355,27.2998580497492,28.2743338823081),
 .UNSPECIFIED.);
#5443=B_SPLINE_CURVE_WITH_KNOTS('',3,(#33472,#33473,#33474,#33475,#33476),
 .UNSPECIFIED.,.F.,.F.,(4,1,4),(14.3984001269719,15.3908199671856,15.7079632679489),
 .UNSPECIFIED.);
#5444=B_SPLINE_CURVE_WITH_KNOTS('',3,(#33479,#33480,#33481,#33482,#33483),
 .UNSPECIFIED.,.F.,.F.,(4,1,4),(13.8759337553364,14.8362483829487,15.7079632679489),
 .UNSPECIFIED.);
#5445=B_SPLINE_CURVE_WITH_KNOTS('',3,(#33489,#33490,#33491,#33492),
 .UNSPECIFIED.,.F.,.F.,(4,4),(95.5573427486707,96.2647245007224),
 .UNSPECIFIED.);
#5446=B_SPLINE_CURVE_WITH_KNOTS('',3,(#33500,#33501,#33502,#33503,#33504,
#33505,#33506,#33507,#33508,#33509),.UNSPECIFIED.,.F.,.F.,(4,3,3,4),(-94.2477796076938,
-93.2874649800815,-92.2950451398678,-91.8135687061554),.UNSPECIFIED.);
#5447=B_SPLINE_CURVE_WITH_KNOTS('',3,(#33514,#33515,#33516,#33517,#33518,
#33519,#33520,#33521,#33522,#33523,#33524,#33525,#33526,#33527,#33528,#33529,
#33530,#33531,#33532,#33533,#33534,#33535,#33536,#33537,#33538),
 .UNSPECIFIED.,.F.,.F.,(4,3,3,3,3,3,3,3,4),(89.2741574414911,89.317785619227,
90.3102054594406,91.3026252996542,92.2950451398679,93.2874649800815,94.2798848202951,
95.2723046605088,95.5573427486707),.UNSPECIFIED.);
#5448=B_SPLINE_CURVE_WITH_KNOTS('',3,(#33539,#33540,#33541,#33542,#33543,
#33544,#33545,#33546,#33547,#33548,#33549,#33550,#33551,#33552,#33553,#33554,
#33555,#33556,#33557,#33558,#33559,#33560),.UNSPECIFIED.,.F.,.F.,(4,3,3,
3,3,3,3,4),(-91.8135687061554,-91.3026252996542,-90.3102054594406,-89.3177856192269,
-88.3253657790133,-87.3329459387997,-86.3405260985861,-85.5303833989757),
 .UNSPECIFIED.);
#5449=B_SPLINE_CURVE_WITH_KNOTS('',3,(#33565,#33566,#33567,#33568,#33569,
#33570,#33571,#33572,#33573,#33574,#33575,#33576,#33577,#33578,#33579,#33580,
#33581,#33582,#33583,#33584,#33585,#33586),.UNSPECIFIED.,.F.,.F.,(4,3,3,
3,3,3,3,4),(82.9909721343116,83.3632665779452,84.3556864181588,85.3481062583724,
86.3405260985861,87.3329459387997,88.3253657790133,89.2741574414911),
 .UNSPECIFIED.);
#5450=B_SPLINE_CURVE_WITH_KNOTS('',3,(#33587,#33588,#33589,#33590,#33591,
#33592,#33593,#33594,#33595,#33596,#33597,#33598,#33599,#33600,#33601,#33602,
#33603,#33604,#33605,#33606,#33607,#33608,#33609,#33610,#33611),
 .UNSPECIFIED.,.F.,.F.,(4,3,3,3,3,3,3,3,4),(-85.5303833989757,-85.3481062583724,
-84.3556864181588,-83.3632665779452,-82.3708467377315,-81.3784268975179,
-80.3860070573042,-79.3935872170906,-79.2471980917961),.UNSPECIFIED.);
#5451=B_SPLINE_CURVE_WITH_KNOTS('',3,(#33616,#33617,#33618,#33619,#33620,
#33621,#33622,#33623,#33624,#33625,#33626,#33627,#33628,#33629,#33630,#33631,
#33632,#33633,#33634,#33635,#33636,#33637),.UNSPECIFIED.,.F.,.F.,(4,3,3,
3,3,3,3,4),(76.7077868271319,77.4087475366634,78.401167376877,79.3935872170907,
80.3860070573043,81.3784268975179,82.3708467377316,82.9909721343116),
 .UNSPECIFIED.);
#5452=B_SPLINE_CURVE_WITH_KNOTS('',3,(#33638,#33639,#33640,#33641,#33642,
#33643,#33644,#33645,#33646,#33647,#33648,#33649,#33650,#33651,#33652,#33653,
#33654,#33655,#33656,#33657,#33658,#33659),.UNSPECIFIED.,.F.,.F.,(4,3,3,
3,3,3,3,4),(-79.2471980917961,-78.401167376877,-77.4087475366634,-76.4163276964497,
-75.4239078562361,-74.4314880160224,-73.4390681758088,-72.9640127846165),
 .UNSPECIFIED.);
#5453=B_SPLINE_CURVE_WITH_KNOTS('',3,(#33664,#33665,#33666,#33667,#33668,
#33669,#33670,#33671,#33672,#33673,#33674,#33675,#33676,#33677,#33678,#33679,
#33680,#33681,#33682,#33683,#33684,#33685,#33686,#33687,#33688),
 .UNSPECIFIED.,.F.,.F.,(4,3,3,3,3,3,3,3,4),(70.4246015199523,70.4618086551679,
71.4542284953816,72.4466483355952,73.4390681758088,74.4314880160225,75.4239078562361,
76.4163276964497,76.7077868271319),.UNSPECIFIED.);
#5454=B_SPLINE_CURVE_WITH_KNOTS('',3,(#33689,#33690,#33691,#33692,#33693,
#33694,#33695,#33696,#33697,#33698,#33699,#33700,#33701,#33702,#33703,#33704,
#33705,#33706,#33707,#33708,#33709,#33710),.UNSPECIFIED.,.F.,.F.,(4,3,3,
3,3,3,3,4),(-72.9640127846165,-72.4466483355952,-71.4542284953815,-70.4618086551679,
-69.4693888149543,-68.4769689747406,-67.484549134527,-66.680827477437),
 .UNSPECIFIED.);
#5455=B_SPLINE_CURVE_WITH_KNOTS('',3,(#33715,#33716,#33717,#33718,#33719,
#33720,#33721,#33722,#33723,#33724,#33725,#33726,#33727,#33728,#33729,#33730,
#33731,#33732,#33733,#33734,#33735,#33736),.UNSPECIFIED.,.F.,.F.,(4,3,3,
3,3,3,3,4),(64.1414162127728,64.5072896138861,65.4997094540998,66.4921292943134,
67.484549134527,68.4769689747407,69.4693888149543,70.4246015199523),
 .UNSPECIFIED.);
#5456=B_SPLINE_CURVE_WITH_KNOTS('',3,(#33737,#33738,#33739,#33740,#33741,
#33742,#33743,#33744,#33745,#33746,#33747,#33748,#33749,#33750,#33751,#33752,
#33753,#33754,#33755,#33756,#33757,#33758,#33759,#33760,#33761),
 .UNSPECIFIED.,.F.,.F.,(4,3,3,3,3,3,3,3,4),(-66.680827477437,-66.4921292943134,
-65.4997094540998,-64.5072896138861,-63.5148697736725,-62.5224499334589,
-61.5300300932452,-60.5376102530316,-60.3976421702573),.UNSPECIFIED.);
#5457=B_SPLINE_CURVE_WITH_KNOTS('',3,(#33766,#33767,#33768,#33769,#33770,
#33771,#33772,#33773,#33774,#33775,#33776,#33777,#33778,#33779,#33780,#33781,
#33782,#33783,#33784,#33785,#33786,#33787),.UNSPECIFIED.,.F.,.F.,(4,3,3,
3,3,3,3,4),(57.8582309055932,58.5527705726044,59.545190412818,60.5376102530316,
61.5300300932453,62.5224499334589,63.5148697736725,64.1414162127728),
 .UNSPECIFIED.);
#5458=B_SPLINE_CURVE_WITH_KNOTS('',3,(#33788,#33789,#33790,#33791,#33792,
#33793,#33794,#33795,#33796,#33797,#33798,#33799,#33800,#33801,#33802,#33803,
#33804,#33805,#33806,#33807,#33808,#33809),.UNSPECIFIED.,.F.,.F.,(4,3,3,
3,3,3,3,4),(-60.3976421702573,-59.545190412818,-58.5527705726043,-57.5603507323907,
-56.5679308921771,-55.5755110519634,-54.5830912117498,-54.1144568630777),
 .UNSPECIFIED.);
#5459=B_SPLINE_CURVE_WITH_KNOTS('',3,(#33814,#33815,#33816,#33817,#33818,
#33819,#33820,#33821,#33822,#33823,#33824,#33825,#33826,#33827,#33828,#33829,
#33830,#33831,#33832,#33833,#33834,#33835,#33836,#33837,#33838),
 .UNSPECIFIED.,.F.,.F.,(4,3,3,3,3,3,3,3,4),(51.5750455984135,51.6058316911089,
52.5982515313226,53.5906713715362,54.5830912117498,55.5755110519634,56.5679308921771,
57.5603507323907,57.8582309055932),.UNSPECIFIED.);
#5460=B_SPLINE_CURVE_WITH_KNOTS('',3,(#33839,#33840,#33841,#33842,#33843,
#33844,#33845,#33846,#33847,#33848,#33849,#33850,#33851,#33852,#33853,#33854,
#33855,#33856,#33857,#33858,#33859,#33860),.UNSPECIFIED.,.F.,.F.,(4,3,3,
3,3,3,3,4),(-54.1144568630777,-53.5906713715362,-52.5982515313225,-51.6058316911089,
-50.6134118508953,-49.6209920106816,-48.628572170468,-47.8312715558982),
 .UNSPECIFIED.);
#5461=B_SPLINE_CURVE_WITH_KNOTS('',3,(#33865,#33866,#33867,#33868,#33869,
#33870,#33871,#33872,#33873,#33874,#33875,#33876,#33877,#33878,#33879,#33880,
#33881,#33882,#33883,#33884,#33885,#33886),.UNSPECIFIED.,.F.,.F.,(4,3,3,
3,3,3,3,4),(45.291860291234,45.6513126498271,46.6437324900408,47.6361523302544,
48.628572170468,49.6209920106817,50.6134118508953,51.5750455984135),
 .UNSPECIFIED.);
#5462=B_SPLINE_CURVE_WITH_KNOTS('',3,(#33887,#33888,#33889,#33890,#33891,
#33892,#33893,#33894,#33895,#33896,#33897,#33898,#33899,#33900,#33901,#33902,
#33903,#33904,#33905,#33906,#33907,#33908,#33909,#33910,#33911),
 .UNSPECIFIED.,.F.,.F.,(4,3,3,3,3,3,3,3,4),(-47.8312715558982,-47.6361523302544,
-46.6437324900407,-45.6513126498271,-44.6588928096135,-43.6664729693998,
-42.6740531291862,-41.6816332889726,-41.5480862487186),.UNSPECIFIED.);
#5463=B_SPLINE_CURVE_WITH_KNOTS('',3,(#33916,#33917,#33918,#33919,#33920,
#33921,#33922,#33923,#33924,#33925,#33926,#33927,#33928,#33929,#33930,#33931,
#33932,#33933,#33934,#33935,#33936,#33937),.UNSPECIFIED.,.F.,.F.,(4,3,3,
3,3,3,3,4),(39.0086749840544,39.6967936085453,40.6892134487589,41.6816332889726,
42.6740531291862,43.6664729693998,44.6588928096135,45.291860291234),
 .UNSPECIFIED.);
#5464=B_SPLINE_CURVE_WITH_KNOTS('',3,(#33938,#33939,#33940,#33941,#33942,
#33943,#33944,#33945,#33946,#33947,#33948,#33949,#33950,#33951,#33952,#33953,
#33954,#33955,#33956,#33957,#33958,#33959),.UNSPECIFIED.,.F.,.F.,(4,3,3,
3,3,3,3,4),(-41.5480862487186,-40.6892134487589,-39.6967936085453,-38.7043737683317,
-37.711953928118,-36.7195340879044,-35.7271142476908,-35.2649009415389),
 .UNSPECIFIED.);
#5465=B_SPLINE_CURVE_WITH_KNOTS('',3,(#33964,#33965,#33966,#33967,#33968,
#33969,#33970,#33971,#33972,#33973,#33974,#33975,#33976,#33977,#33978,#33979,
#33980,#33981,#33982,#33983,#33984,#33985,#33986,#33987,#33988),
 .UNSPECIFIED.,.F.,.F.,(4,3,3,3,3,3,3,3,4),(32.7254896768748,32.7498547270499,
33.7422745672635,34.7346944074771,35.7271142476908,36.7195340879044,37.711953928118,
38.7043737683317,39.0086749840544),.UNSPECIFIED.);
#5466=B_SPLINE_CURVE_WITH_KNOTS('',3,(#33989,#33990,#33991,#33992,#33993,
#33994,#33995,#33996,#33997,#33998,#33999,#34000,#34001,#34002,#34003,#34004,
#34005,#34006,#34007,#34008,#34009,#34010),.UNSPECIFIED.,.F.,.F.,(4,3,3,
3,3,3,3,4),(-35.2649009415389,-34.7346944074771,-33.7422745672635,-32.7498547270499,
-31.7574348868362,-30.7650150466226,-29.772595206409,-28.9817156343594),
 .UNSPECIFIED.);
#5467=B_SPLINE_CURVE_WITH_KNOTS('',3,(#34015,#34016,#34017,#34018,#34019,
#34020,#34021,#34022,#34023,#34024,#34025,#34026,#34027,#34028,#34029,#34030,
#34031,#34032,#34033,#34034,#34035,#34036),.UNSPECIFIED.,.F.,.F.,(4,3,3,
3,3,3,3,4),(26.4423043696952,26.7953356857681,27.7877555259817,28.7801753661954,
29.772595206409,30.7650150466226,31.7574348868363,32.7254896768748),
 .UNSPECIFIED.);
#5468=B_SPLINE_CURVE_WITH_KNOTS('',3,(#34037,#34038,#34039,#34040,#34041,
#34042,#34043,#34044,#34045,#34046,#34047,#34048,#34049,#34050,#34051,#34052,
#34053,#34054,#34055,#34056,#34057,#34058,#34059,#34060,#34061),
 .UNSPECIFIED.,.F.,.F.,(4,3,3,3,3,3,3,3,4),(-28.9817156343594,-28.7801753661953,
-27.7877555259817,-26.7953356857681,-25.8029158455544,-24.8104960053408,
-23.8180761651272,-22.8256563249135,-22.6985303271798),.UNSPECIFIED.);
#5469=B_SPLINE_CURVE_WITH_KNOTS('',3,(#34066,#34067,#34068,#34069,#34070,
#34071,#34072,#34073,#34074,#34075,#34076,#34077,#34078,#34079,#34080,#34081,
#34082,#34083,#34084,#34085,#34086,#34087),.UNSPECIFIED.,.F.,.F.,(4,3,3,
3,3,3,3,4),(20.1591190625156,20.8408166444863,21.8332364846999,22.8256563249136,
23.8180761651272,24.8104960053408,25.8029158455545,26.4423043696952),
 .UNSPECIFIED.);
#5470=B_SPLINE_CURVE_WITH_KNOTS('',3,(#34088,#34089,#34090,#34091,#34092,
#34093,#34094,#34095,#34096,#34097,#34098,#34099,#34100,#34101,#34102,#34103,
#34104,#34105,#34106,#34107,#34108,#34109),.UNSPECIFIED.,.F.,.F.,(4,3,3,
3,3,3,3,4),(-22.6985303271798,-21.8332364846999,-20.8408166444863,-19.8483968042727,
-18.855976964059,-17.8635571238454,-16.8711372836318,-16.4153450200002),
 .UNSPECIFIED.);
#5471=B_SPLINE_CURVE_WITH_KNOTS('',3,(#34114,#34115,#34116,#34117,#34118,
#34119,#34120,#34121,#34122,#34123,#34124,#34125,#34126,#34127,#34128,#34129,
#34130,#34131,#34132,#34133,#34134,#34135,#34136,#34137,#34138),
 .UNSPECIFIED.,.F.,.F.,(4,3,3,3,3,3,3,3,4),(13.875933755336,13.8938777629909,
14.8862976032045,15.8787174434181,16.8711372836318,17.8635571238454,18.855976964059,
19.8483968042727,20.1591190625156),.UNSPECIFIED.);
#5472=B_SPLINE_CURVE_WITH_KNOTS('',3,(#34139,#34140,#34141,#34142,#34143,
#34144,#34145,#34146,#34147,#34148,#34149,#34150,#34151,#34152,#34153,#34154,
#34155,#34156,#34157,#34158,#34159,#34160),.UNSPECIFIED.,.F.,.F.,(4,3,3,
3,3,3,3,4),(-16.4153450200002,-15.8787174434181,-14.8862976032045,-13.8938777629909,
-12.9014579227772,-11.9090380825636,-10.91661824235,-10.1321597128207),
 .UNSPECIFIED.);
#5473=B_SPLINE_CURVE_WITH_KNOTS('',3,(#34166,#34167,#34168,#34169,#34170,
#34171,#34172,#34173,#34174,#34175,#34176,#34177,#34178),.UNSPECIFIED.,
 .F.,.F.,(4,3,3,3,4),(-3.848974405641,-2.9772595206409,-1.98483968042726,
-0.99241984021363,0.),.UNSPECIFIED.);
#5474=B_SPLINE_CURVE_WITH_KNOTS('',3,(#34181,#34182,#34183,#34184,#34185,
#34186,#34187,#34188,#34189,#34190,#34191,#34192,#34193,#34194,#34195,#34196,
#34197,#34198,#34199),.UNSPECIFIED.,.F.,.F.,(4,3,3,3,3,3,4),(2.01694489302852,
2.9772595206409,3.96967936085454,4.96209920106817,5.9545190412818,6.94693888149544,
7.59274844815647),.UNSPECIFIED.);
#5475=B_SPLINE_CURVE_WITH_KNOTS('',3,(#34205,#34206,#34207,#34208,#34209,
#34210,#34211,#34212),.UNSPECIFIED.,.F.,.F.,(4,1,1,1,1,4),(103.672557568463,
104.154034002176,105.146453842389,106.138873682603,107.131293522817,108.12371336303),
 .UNSPECIFIED.);
#5476=B_SPLINE_CURVE_WITH_KNOTS('',3,(#34215,#34216,#34217,#34218,#34219,
#34220,#34221,#34222,#34223),.UNSPECIFIED.,.F.,.F.,(4,1,1,1,1,1,4),(103.672557568463,
103.716185746199,104.708605586413,105.701025426626,106.69344526684,107.685865107053,
108.646179734666),.UNSPECIFIED.);
#5477=B_SPLINE_CURVE_WITH_KNOTS('',3,(#34228,#34229,#34230,#34231,#34232,
#34233,#34234,#34235,#34236,#34237),.UNSPECIFIED.,.F.,.F.,(4,1,1,1,1,1,
1,4),(97.3893722612835,98.1995149608939,99.1919348011075,100.184354641321,
101.176774481535,102.169194321748,103.161614161962,103.672557568463),
 .UNSPECIFIED.);
#5478=B_SPLINE_CURVE_WITH_KNOTS('',3,(#34238,#34239,#34240,#34241,#34242,
#34243,#34244,#34245,#34246,#34247),.UNSPECIFIED.,.F.,.F.,(4,1,1,1,1,1,
1,4),(97.3893722612835,97.7616667049171,98.7540865451307,99.7465063853444,
100.738926225558,101.731346065772,102.723765905985,103.672557568463),
 .UNSPECIFIED.);
#5479=B_SPLINE_CURVE_WITH_KNOTS('',3,(#34252,#34253,#34254,#34255,#34256,
#34257,#34258,#34259,#34260,#34261,#34262),.UNSPECIFIED.,.F.,.F.,(4,1,1,
1,1,1,1,1,4),(91.106186954104,91.2525760793984,92.2449959196121,93.2374157598257,
94.2298356000393,95.222255440253,96.2146752804666,97.2070951206802,97.3893722612835),
 .UNSPECIFIED.);
#5480=B_SPLINE_CURVE_WITH_KNOTS('',3,(#34263,#34264,#34265,#34266,#34267,
#34268,#34269,#34270,#34271,#34272),.UNSPECIFIED.,.F.,.F.,(4,1,1,1,1,1,
1,4),(91.106186954104,91.8071476636353,92.7995675038489,93.7919873440626,
94.7844071842762,95.7768270244898,96.7692468647035,97.3893722612835),
 .UNSPECIFIED.);
#5481=B_SPLINE_CURVE_WITH_KNOTS('',3,(#34277,#34278,#34279,#34280,#34281,
#34282,#34283,#34284,#34285,#34286),.UNSPECIFIED.,.F.,.F.,(4,1,1,1,1,1,
1,4),(84.8230016469244,85.2980570381166,86.2904768783303,87.2828967185439,
88.2753165587575,89.2677363989712,90.2601562391848,91.106186954104),
 .UNSPECIFIED.);
#5482=B_SPLINE_CURVE_WITH_KNOTS('',3,(#34287,#34288,#34289,#34290,#34291,
#34292,#34293,#34294,#34295,#34296,#34297),.UNSPECIFIED.,.F.,.F.,(4,1,1,
1,1,1,1,1,4),(84.8230016469244,84.8602087821399,85.8526286223535,86.8450484625671,
87.8374683027808,88.8298881429944,89.822307983208,90.8147278234217,91.106186954104),
 .UNSPECIFIED.);
#5483=B_SPLINE_CURVE_WITH_KNOTS('',3,(#34302,#34303,#34304,#34305,#34306,
#34307,#34308,#34309,#34310,#34311),.UNSPECIFIED.,.F.,.F.,(4,1,1,1,1,1,
1,4),(78.5398163397448,79.3435379968348,80.3359578370485,81.3283776772621,
82.3207975174757,83.3132173576894,84.305637197903,84.8230016469244),
 .UNSPECIFIED.);
#5484=B_SPLINE_CURVE_WITH_KNOTS('',3,(#34312,#34313,#34314,#34315,#34316,
#34317,#34318,#34319,#34320,#34321),.UNSPECIFIED.,.F.,.F.,(4,1,1,1,1,1,
1,4),(78.5398163397448,78.9056897408581,79.8981095810717,80.8905294212853,
81.882949261499,82.8753691017126,83.8677889419262,84.8230016469244),
 .UNSPECIFIED.);
#5485=B_SPLINE_CURVE_WITH_KNOTS('',3,(#34326,#34327,#34328,#34329,#34330,
#34331,#34332,#34333,#34334,#34335,#34336),.UNSPECIFIED.,.F.,.F.,(4,1,1,
1,1,1,1,1,4),(72.2566310325653,72.3965991153394,73.389018955553,74.3814387957667,
75.3738586359803,76.3662784761939,77.3586983164076,78.3511181566212,78.5398163397448),
 .UNSPECIFIED.);
#5486=B_SPLINE_CURVE_WITH_KNOTS('',3,(#34337,#34338,#34339,#34340,#34341,
#34342,#34343,#34344,#34345,#34346),.UNSPECIFIED.,.F.,.F.,(4,1,1,1,1,1,
1,4),(72.2566310325651,72.9511706995763,73.9435905397899,74.9360103800035,
75.9284302202172,76.9208500604308,77.9132699006444,78.5398163397448),
 .UNSPECIFIED.);
#5487=B_SPLINE_CURVE_WITH_KNOTS('',3,(#34351,#34352,#34353,#34354,#34355,
#34356,#34357,#34358,#34359,#34360),.UNSPECIFIED.,.F.,.F.,(4,1,1,1,1,1,
1,4),(65.9734457253856,66.4420800740576,67.4344999142712,68.4269197544849,
69.4193395946985,70.4117594349121,71.4041792751258,72.2566310325653),
 .UNSPECIFIED.);
#5488=B_SPLINE_CURVE_WITH_KNOTS('',3,(#34361,#34362,#34363,#34364,#34365,
#34366,#34367,#34368,#34369,#34370,#34371),.UNSPECIFIED.,.F.,.F.,(4,1,1,
1,1,1,1,1,4),(65.9734457253856,66.0042318180808,66.9966516582945,67.9890714985081,
68.9814913387217,69.9739111789354,70.966331019149,71.9587508593626,72.2566310325651),
 .UNSPECIFIED.);
#5489=B_SPLINE_CURVE_WITH_KNOTS('',3,(#34376,#34377,#34378,#34379,#34380,
#34381,#34382,#34383,#34384,#34385),.UNSPECIFIED.,.F.,.F.,(4,1,1,1,1,1,
1,4),(59.690260418206,60.4875610327758,61.4799808729895,62.4724007132031,
63.4648205534167,64.4572403936303,65.449660233844,65.9734457253856),
 .UNSPECIFIED.);
#5490=B_SPLINE_CURVE_WITH_KNOTS('',3,(#34386,#34387,#34388,#34389,#34390,
#34391,#34392,#34393,#34394,#34395),.UNSPECIFIED.,.F.,.F.,(4,1,1,1,1,1,
1,4),(59.690260418206,60.049712776799,61.0421326170127,62.0345524572263,
63.0269722974399,64.0193921376536,65.0118119778672,65.9734457253856),
 .UNSPECIFIED.);
#5491=B_SPLINE_CURVE_WITH_KNOTS('',3,(#34400,#34401,#34402,#34403,#34404,
#34405,#34406,#34407,#34408,#34409,#34410),.UNSPECIFIED.,.F.,.F.,(4,1,1,
1,1,1,1,1,4),(53.4070751110265,53.5406221512804,54.533041991494,55.5254618317077,
56.5178816719213,57.5103015121349,58.5027213523486,59.4951411925622,59.690260418206),
 .UNSPECIFIED.);
#5492=B_SPLINE_CURVE_WITH_KNOTS('',3,(#34411,#34412,#34413,#34414,#34415,
#34416,#34417,#34418,#34419,#34420),.UNSPECIFIED.,.F.,.F.,(4,1,1,1,1,1,
1,4),(53.4070751110265,54.0951937355172,55.0876135757309,56.0800334159445,
57.0724532561581,58.0648730963718,59.0572929365854,59.690260418206),
 .UNSPECIFIED.);
#5493=B_SPLINE_CURVE_WITH_KNOTS('',3,(#34425,#34426,#34427,#34428,#34429,
#34430,#34431,#34432,#34433,#34434),.UNSPECIFIED.,.F.,.F.,(4,1,1,1,1,1,
1,4),(47.1238898038468,47.5861031099986,48.5785229502122,49.5709427904259,
50.5633626306395,51.5557824708531,52.5482023110668,53.4070751110265),
 .UNSPECIFIED.);
#5494=B_SPLINE_CURVE_WITH_KNOTS('',3,(#34435,#34436,#34437,#34438,#34439,
#34440,#34441,#34442,#34443,#34444,#34445),.UNSPECIFIED.,.F.,.F.,(4,1,1,
1,1,1,1,1,4),(47.1238898038468,47.1482548540218,48.1406746942354,49.1330945344491,
50.1255143746627,51.1179342148763,52.11035405509,53.1027738953036,53.4070751110265),
 .UNSPECIFIED.);
#5495=B_SPLINE_CURVE_WITH_KNOTS('',3,(#34450,#34451,#34452,#34453,#34454,
#34455,#34456,#34457,#34458,#34459),.UNSPECIFIED.,.F.,.F.,(4,1,1,1,1,1,
1,4),(40.8407044966672,41.6315840687168,42.6240039089304,43.6164237491441,
44.6088435893577,45.6012634295713,46.593683269785,47.1238898038468),
 .UNSPECIFIED.);
#5496=B_SPLINE_CURVE_WITH_KNOTS('',3,(#34460,#34461,#34462,#34463,#34464,
#34465,#34466,#34467,#34468,#34469),.UNSPECIFIED.,.F.,.F.,(4,1,1,1,1,1,
1,4),(40.8407044966672,41.19373581274,42.1861556529536,43.1785754931673,
44.1709953333809,45.1634151735945,46.1558350138082,47.1238898038468),
 .UNSPECIFIED.);
#5497=B_SPLINE_CURVE_WITH_KNOTS('',3,(#34474,#34475,#34476,#34477,#34478,
#34479,#34480,#34481,#34482,#34483,#34484),.UNSPECIFIED.,.F.,.F.,(4,1,1,
1,1,1,1,1,4),(34.5575191894877,34.6846451872214,35.677065027435,36.6694848676486,
37.6619047078623,38.6543245480759,39.6467443882895,40.6391642285032,40.8407044966672),
 .UNSPECIFIED.);
#5498=B_SPLINE_CURVE_WITH_KNOTS('',3,(#34485,#34486,#34487,#34488,#34489,
#34490,#34491,#34492,#34493,#34494),.UNSPECIFIED.,.F.,.F.,(4,1,1,1,1,1,
1,4),(34.5575191894877,35.2392167714582,36.2316366116718,37.2240564518855,
38.2164762920991,39.2088961323127,40.2013159725264,40.8407044966672),
 .UNSPECIFIED.);
#5499=B_SPLINE_CURVE_WITH_KNOTS('',3,(#34499,#34500,#34501,#34502,#34503,
#34504,#34505,#34506,#34507,#34508),.UNSPECIFIED.,.F.,.F.,(4,1,1,1,1,1,
1,4),(28.2743338823081,28.7301261459396,29.7225459861532,30.7149658263668,
31.7073856665805,32.6998055067941,33.6922253470077,34.5575191894877),
 .UNSPECIFIED.);
#5500=B_SPLINE_CURVE_WITH_KNOTS('',3,(#34509,#34510,#34511,#34512,#34513,
#34514,#34515,#34516,#34517,#34518,#34519),.UNSPECIFIED.,.F.,.F.,(4,1,1,
1,1,1,1,1,4),(28.2743338823081,28.2922778899628,29.2846977301764,30.2771175703901,
31.2695374106037,32.2619572508173,33.2543770910309,34.2467969312446,34.5575191894877),
 .UNSPECIFIED.);
#5501=B_SPLINE_CURVE_WITH_KNOTS('',3,(#34524,#34525,#34526,#34527,#34528,
#34529,#34530,#34531,#34532,#34533),.UNSPECIFIED.,.F.,.F.,(4,1,1,1,1,1,
1,4),(21.9911485751285,22.7756071046578,23.7680269448714,24.760446785085,
25.7528666252987,26.7452864655123,27.7377063057259,28.2743338823081),
 .UNSPECIFIED.);
#5502=B_SPLINE_CURVE_WITH_KNOTS('',3,(#34534,#34535,#34536,#34537,#34538,
#34539,#34540,#34541,#34542,#34543),.UNSPECIFIED.,.F.,.F.,(4,1,1,1,1,1,
1,4),(21.9911485751284,22.337758848681,23.3301786888946,24.3225985291083,
25.3150183693219,26.3074382095355,27.2998580497492,28.2743338823081),
 .UNSPECIFIED.);
#5503=B_SPLINE_CURVE_WITH_KNOTS('',3,(#34549,#34550,#34551,#34552,#34553),
 .UNSPECIFIED.,.F.,.F.,(4,1,4),(14.3984001269719,15.3908199671856,15.7079632679489),
 .UNSPECIFIED.);
#5504=B_SPLINE_CURVE_WITH_KNOTS('',3,(#34556,#34557,#34558,#34559,#34560),
 .UNSPECIFIED.,.F.,.F.,(4,1,4),(13.8759337553364,14.8362483829487,15.7079632679489),
 .UNSPECIFIED.);
#5505=B_SPLINE_CURVE_WITH_KNOTS('',3,(#34566,#34567,#34568,#34569),
 .UNSPECIFIED.,.F.,.F.,(4,4),(95.5573427486708,96.2647245007226),
 .UNSPECIFIED.);
#5506=B_SPLINE_CURVE_WITH_KNOTS('',3,(#34577,#34578,#34579,#34580,#34581,
#34582,#34583,#34584,#34585,#34586),.UNSPECIFIED.,.F.,.F.,(4,3,3,4),(-94.2477796076939,
-93.2874649800816,-92.295045139868,-91.8135687061555),.UNSPECIFIED.);
#5507=B_SPLINE_CURVE_WITH_KNOTS('',3,(#34591,#34592,#34593,#34594,#34595,
#34596,#34597,#34598,#34599,#34600,#34601,#34602,#34603,#34604,#34605,#34606,
#34607,#34608,#34609,#34610,#34611,#34612,#34613,#34614,#34615),
 .UNSPECIFIED.,.F.,.F.,(4,3,3,3,3,3,3,3,4),(89.2741574414912,89.3177856192271,
90.3102054594407,91.3026252996544,92.295045139868,93.2874649800816,94.2798848202952,
95.2723046605089,95.5573427486708),.UNSPECIFIED.);
#5508=B_SPLINE_CURVE_WITH_KNOTS('',3,(#34616,#34617,#34618,#34619,#34620,
#34621,#34622,#34623,#34624,#34625,#34626,#34627,#34628,#34629,#34630,#34631,
#34632,#34633,#34634,#34635,#34636,#34637),.UNSPECIFIED.,.F.,.F.,(4,3,3,
3,3,3,3,4),(-91.8135687061555,-91.3026252996543,-90.3102054594407,-89.3177856192271,
-88.3253657790134,-87.3329459387998,-86.3405260985862,-85.5303833989758),
 .UNSPECIFIED.);
#5509=B_SPLINE_CURVE_WITH_KNOTS('',3,(#34642,#34643,#34644,#34645,#34646,
#34647,#34648,#34649,#34650,#34651,#34652,#34653,#34654,#34655,#34656,#34657,
#34658,#34659,#34660,#34661,#34662,#34663),.UNSPECIFIED.,.F.,.F.,(4,3,3,
3,3,3,3,4),(82.9909721343117,83.3632665779453,84.3556864181589,85.3481062583725,
86.3405260985862,87.3329459387998,88.3253657790134,89.2741574414912),
 .UNSPECIFIED.);
#5510=B_SPLINE_CURVE_WITH_KNOTS('',3,(#34664,#34665,#34666,#34667,#34668,
#34669,#34670,#34671,#34672,#34673,#34674,#34675,#34676,#34677,#34678,#34679,
#34680,#34681,#34682,#34683,#34684,#34685,#34686,#34687,#34688),
 .UNSPECIFIED.,.F.,.F.,(4,3,3,3,3,3,3,3,4),(-85.5303833989758,-85.3481062583725,
-84.3556864181589,-83.3632665779453,-82.3708467377316,-81.378426897518,
-80.3860070573044,-79.3935872170907,-79.2471980917962),.UNSPECIFIED.);
#5511=B_SPLINE_CURVE_WITH_KNOTS('',3,(#34693,#34694,#34695,#34696,#34697,
#34698,#34699,#34700,#34701,#34702,#34703,#34704,#34705,#34706,#34707,#34708,
#34709,#34710,#34711,#34712,#34713,#34714),.UNSPECIFIED.,.F.,.F.,(4,3,3,
3,3,3,3,4),(76.707786827132,77.4087475366635,78.4011673768771,79.3935872170907,
80.3860070573044,81.378426897518,82.3708467377316,82.9909721343117),
 .UNSPECIFIED.);
#5512=B_SPLINE_CURVE_WITH_KNOTS('',3,(#34715,#34716,#34717,#34718,#34719,
#34720,#34721,#34722,#34723,#34724,#34725,#34726,#34727,#34728,#34729,#34730,
#34731,#34732,#34733,#34734,#34735,#34736),.UNSPECIFIED.,.F.,.F.,(4,3,3,
3,3,3,3,4),(-79.2471980917962,-78.4011673768771,-77.4087475366635,-76.4163276964498,
-75.4239078562362,-74.4314880160225,-73.4390681758089,-72.9640127846167),
 .UNSPECIFIED.);
#5513=B_SPLINE_CURVE_WITH_KNOTS('',3,(#34741,#34742,#34743,#34744,#34745,
#34746,#34747,#34748,#34749,#34750,#34751,#34752,#34753,#34754,#34755,#34756,
#34757,#34758,#34759,#34760,#34761,#34762,#34763,#34764,#34765),
 .UNSPECIFIED.,.F.,.F.,(4,3,3,3,3,3,3,3,4),(70.4246015199524,70.461808655168,
71.4542284953817,72.4466483355953,73.4390681758089,74.4314880160226,75.4239078562362,
76.4163276964498,76.707786827132),.UNSPECIFIED.);
#5514=B_SPLINE_CURVE_WITH_KNOTS('',3,(#34766,#34767,#34768,#34769,#34770,
#34771,#34772,#34773,#34774,#34775,#34776,#34777,#34778,#34779,#34780,#34781,
#34782,#34783,#34784,#34785,#34786,#34787),.UNSPECIFIED.,.F.,.F.,(4,3,3,
3,3,3,3,4),(-72.9640127846167,-72.4466483355953,-71.4542284953816,-70.461808655168,
-69.4693888149544,-68.4769689747407,-67.4845491345271,-66.6808274774371),
 .UNSPECIFIED.);
#5515=B_SPLINE_CURVE_WITH_KNOTS('',3,(#34792,#34793,#34794,#34795,#34796,
#34797,#34798,#34799,#34800,#34801,#34802,#34803,#34804,#34805,#34806,#34807,
#34808,#34809,#34810,#34811,#34812,#34813),.UNSPECIFIED.,.F.,.F.,(4,3,3,
3,3,3,3,4),(64.1414162127729,64.5072896138862,65.4997094540998,66.4921292943135,
67.4845491345271,68.4769689747407,69.4693888149544,70.4246015199524),
 .UNSPECIFIED.);
#5516=B_SPLINE_CURVE_WITH_KNOTS('',3,(#34814,#34815,#34816,#34817,#34818,
#34819,#34820,#34821,#34822,#34823,#34824,#34825,#34826,#34827,#34828,#34829,
#34830,#34831,#34832,#34833,#34834,#34835,#34836,#34837,#34838),
 .UNSPECIFIED.,.F.,.F.,(4,3,3,3,3,3,3,3,4),(-66.6808274774371,-66.4921292943135,
-65.4997094540998,-64.5072896138862,-63.5148697736726,-62.5224499334589,
-61.5300300932453,-60.5376102530317,-60.3976421702574),.UNSPECIFIED.);
#5517=B_SPLINE_CURVE_WITH_KNOTS('',3,(#34843,#34844,#34845,#34846,#34847,
#34848,#34849,#34850,#34851,#34852,#34853,#34854,#34855,#34856,#34857,#34858,
#34859,#34860,#34861,#34862,#34863,#34864),.UNSPECIFIED.,.F.,.F.,(4,3,3,
3,3,3,3,4),(57.8582309055933,58.5527705726044,59.545190412818,60.5376102530317,
61.5300300932453,62.5224499334589,63.5148697736726,64.1414162127729),
 .UNSPECIFIED.);
#5518=B_SPLINE_CURVE_WITH_KNOTS('',3,(#34865,#34866,#34867,#34868,#34869,
#34870,#34871,#34872,#34873,#34874,#34875,#34876,#34877,#34878,#34879,#34880,
#34881,#34882,#34883,#34884,#34885,#34886),.UNSPECIFIED.,.F.,.F.,(4,3,3,
3,3,3,3,4),(-60.3976421702574,-59.545190412818,-58.5527705726044,-57.5603507323908,
-56.5679308921771,-55.5755110519635,-54.5830912117499,-54.1144568630778),
 .UNSPECIFIED.);
#5519=B_SPLINE_CURVE_WITH_KNOTS('',3,(#34891,#34892,#34893,#34894,#34895,
#34896,#34897,#34898,#34899,#34900,#34901,#34902,#34903,#34904,#34905,#34906,
#34907,#34908,#34909,#34910,#34911,#34912,#34913,#34914,#34915),
 .UNSPECIFIED.,.F.,.F.,(4,3,3,3,3,3,3,3,4),(51.5750455984136,51.605831691109,
52.5982515313226,53.5906713715362,54.5830912117499,55.5755110519635,56.5679308921771,
57.5603507323908,57.8582309055933),.UNSPECIFIED.);
#5520=B_SPLINE_CURVE_WITH_KNOTS('',3,(#34916,#34917,#34918,#34919,#34920,
#34921,#34922,#34923,#34924,#34925,#34926,#34927,#34928,#34929,#34930,#34931,
#34932,#34933,#34934,#34935,#34936,#34937),.UNSPECIFIED.,.F.,.F.,(4,3,3,
3,3,3,3,4),(-54.1144568630778,-53.5906713715362,-52.5982515313226,-51.605831691109,
-50.6134118508953,-49.6209920106817,-48.6285721704681,-47.8312715558983),
 .UNSPECIFIED.);
#5521=B_SPLINE_CURVE_WITH_KNOTS('',3,(#34942,#34943,#34944,#34945,#34946,
#34947,#34948,#34949,#34950,#34951,#34952,#34953,#34954,#34955,#34956,#34957,
#34958,#34959,#34960,#34961,#34962,#34963),.UNSPECIFIED.,.F.,.F.,(4,3,3,
3,3,3,3,4),(45.2918602912341,45.6513126498272,46.6437324900408,47.6361523302544,
48.6285721704681,49.6209920106817,50.6134118508953,51.5750455984136),
 .UNSPECIFIED.);
#5522=B_SPLINE_CURVE_WITH_KNOTS('',3,(#34964,#34965,#34966,#34967,#34968,
#34969,#34970,#34971,#34972,#34973,#34974,#34975,#34976,#34977,#34978,#34979,
#34980,#34981,#34982,#34983,#34984,#34985,#34986,#34987,#34988),
 .UNSPECIFIED.,.F.,.F.,(4,3,3,3,3,3,3,3,4),(-47.8312715558983,-47.6361523302544,
-46.6437324900408,-45.6513126498272,-44.6588928096135,-43.6664729693999,
-42.6740531291863,-41.6816332889726,-41.5480862487187),.UNSPECIFIED.);
#5523=B_SPLINE_CURVE_WITH_KNOTS('',3,(#34993,#34994,#34995,#34996,#34997,
#34998,#34999,#35000,#35001,#35002,#35003,#35004,#35005,#35006,#35007,#35008,
#35009,#35010,#35011,#35012,#35013,#35014),.UNSPECIFIED.,.F.,.F.,(4,3,3,
3,3,3,3,4),(39.0086749840545,39.6967936085454,40.689213448759,41.6816332889726,
42.6740531291863,43.6664729693999,44.6588928096135,45.2918602912341),
 .UNSPECIFIED.);
#5524=B_SPLINE_CURVE_WITH_KNOTS('',3,(#35015,#35016,#35017,#35018,#35019,
#35020,#35021,#35022,#35023,#35024,#35025,#35026,#35027,#35028,#35029,#35030,
#35031,#35032,#35033,#35034,#35035,#35036),.UNSPECIFIED.,.F.,.F.,(4,3,3,
3,3,3,3,4),(-41.5480862487187,-40.689213448759,-39.6967936085454,-38.7043737683317,
-37.7119539281181,-36.7195340879044,-35.7271142476908,-35.264900941539),
 .UNSPECIFIED.);
#5525=B_SPLINE_CURVE_WITH_KNOTS('',3,(#35041,#35042,#35043,#35044,#35045,
#35046,#35047,#35048,#35049,#35050,#35051,#35052,#35053,#35054,#35055,#35056,
#35057,#35058,#35059,#35060,#35061,#35062,#35063,#35064,#35065),
 .UNSPECIFIED.,.F.,.F.,(4,3,3,3,3,3,3,3,4),(32.725489676875,32.7498547270499,
33.7422745672636,34.7346944074772,35.7271142476908,36.7195340879045,37.7119539281181,
38.7043737683317,39.0086749840545),.UNSPECIFIED.);
#5526=B_SPLINE_CURVE_WITH_KNOTS('',3,(#35066,#35067,#35068,#35069,#35070,
#35071,#35072,#35073,#35074,#35075,#35076,#35077,#35078,#35079,#35080,#35081,
#35082,#35083,#35084,#35085,#35086,#35087),.UNSPECIFIED.,.F.,.F.,(4,3,3,
3,3,3,3,4),(-35.264900941539,-34.7346944074772,-33.7422745672636,-32.7498547270499,
-31.7574348868363,-30.7650150466227,-29.772595206409,-28.9817156343595),
 .UNSPECIFIED.);
#5527=B_SPLINE_CURVE_WITH_KNOTS('',3,(#35092,#35093,#35094,#35095,#35096,
#35097,#35098,#35099,#35100,#35101,#35102,#35103,#35104,#35105,#35106,#35107,
#35108,#35109,#35110,#35111,#35112,#35113),.UNSPECIFIED.,.F.,.F.,(4,3,3,
3,3,3,3,4),(26.4423043696953,26.7953356857681,27.7877555259818,28.7801753661954,
29.772595206409,30.7650150466227,31.7574348868363,32.725489676875),
 .UNSPECIFIED.);
#5528=B_SPLINE_CURVE_WITH_KNOTS('',3,(#35114,#35115,#35116,#35117,#35118,
#35119,#35120,#35121,#35122,#35123,#35124,#35125,#35126,#35127,#35128,#35129,
#35130,#35131,#35132,#35133,#35134,#35135,#35136,#35137,#35138),
 .UNSPECIFIED.,.F.,.F.,(4,3,3,3,3,3,3,3,4),(-28.9817156343595,-28.7801753661954,
-27.7877555259818,-26.7953356857681,-25.8029158455545,-24.8104960053408,
-23.8180761651272,-22.8256563249136,-22.6985303271799),.UNSPECIFIED.);
#5529=B_SPLINE_CURVE_WITH_KNOTS('',3,(#35143,#35144,#35145,#35146,#35147,
#35148,#35149,#35150,#35151,#35152,#35153,#35154,#35155,#35156,#35157,#35158,
#35159,#35160,#35161,#35162,#35163,#35164),.UNSPECIFIED.,.F.,.F.,(4,3,3,
3,3,3,3,4),(20.1591190625157,20.8408166444863,21.8332364846999,22.8256563249136,
23.8180761651272,24.8104960053408,25.8029158455545,26.4423043696953),
 .UNSPECIFIED.);
#5530=B_SPLINE_CURVE_WITH_KNOTS('',3,(#35165,#35166,#35167,#35168,#35169,
#35170,#35171,#35172,#35173,#35174,#35175,#35176,#35177,#35178,#35179,#35180,
#35181,#35182,#35183,#35184,#35185,#35186),.UNSPECIFIED.,.F.,.F.,(4,3,3,
3,3,3,3,4),(-22.6985303271799,-21.8332364846999,-20.8408166444863,-19.8483968042727,
-18.855976964059,-17.8635571238454,-16.8711372836318,-16.4153450200004),
 .UNSPECIFIED.);
#5531=B_SPLINE_CURVE_WITH_KNOTS('',3,(#35191,#35192,#35193,#35194,#35195,
#35196,#35197,#35198,#35199,#35200,#35201,#35202,#35203,#35204,#35205,#35206,
#35207,#35208,#35209,#35210,#35211,#35212,#35213,#35214,#35215),
 .UNSPECIFIED.,.F.,.F.,(4,3,3,3,3,3,3,3,4),(13.8759337553361,13.8938777629909,
14.8862976032045,15.8787174434181,16.8711372836318,17.8635571238454,18.855976964059,
19.8483968042727,20.1591190625157),.UNSPECIFIED.);
#5532=B_SPLINE_CURVE_WITH_KNOTS('',3,(#35216,#35217,#35218,#35219,#35220,
#35221,#35222,#35223,#35224,#35225,#35226,#35227,#35228,#35229,#35230,#35231,
#35232,#35233,#35234,#35235,#35236,#35237),.UNSPECIFIED.,.F.,.F.,(4,3,3,
3,3,3,3,4),(-16.4153450200004,-15.8787174434181,-14.8862976032045,-13.8938777629909,
-12.9014579227772,-11.9090380825636,-10.91661824235,-10.1321597128207),
 .UNSPECIFIED.);
#5533=B_SPLINE_CURVE_WITH_KNOTS('',3,(#35243,#35244,#35245,#35246,#35247,
#35248,#35249,#35250,#35251,#35252,#35253,#35254,#35255),.UNSPECIFIED.,
 .F.,.F.,(4,3,3,3,4),(-3.84897440564112,-2.9772595206409,-1.98483968042727,
-0.992419840213633,0.),.UNSPECIFIED.);
#5534=B_SPLINE_CURVE_WITH_KNOTS('',3,(#35258,#35259,#35260,#35261,#35262,
#35263,#35264,#35265,#35266,#35267,#35268,#35269,#35270,#35271,#35272,#35273,
#35274,#35275,#35276),.UNSPECIFIED.,.F.,.F.,(4,3,3,3,3,3,4),(2.01694489302852,
2.97725952064091,3.96967936085454,4.96209920106817,5.95451904128181,6.94693888149544,
7.59274844815659),.UNSPECIFIED.);
#5535=B_SPLINE_CURVE_WITH_KNOTS('',3,(#35282,#35283,#35284,#35285,#35286,
#35287,#35288,#35289),.UNSPECIFIED.,.F.,.F.,(4,1,1,1,1,4),(103.672557568463,
104.154034002176,105.146453842389,106.138873682603,107.131293522817,108.12371336303),
 .UNSPECIFIED.);
#5536=B_SPLINE_CURVE_WITH_KNOTS('',3,(#35292,#35293,#35294,#35295,#35296,
#35297,#35298,#35299,#35300),.UNSPECIFIED.,.F.,.F.,(4,1,1,1,1,1,4),(103.672557568463,
103.716185746199,104.708605586413,105.701025426626,106.69344526684,107.685865107053,
108.646179734666),.UNSPECIFIED.);
#5537=B_SPLINE_CURVE_WITH_KNOTS('',3,(#35305,#35306,#35307,#35308,#35309,
#35310,#35311,#35312,#35313,#35314),.UNSPECIFIED.,.F.,.F.,(4,1,1,1,1,1,
1,4),(97.3893722612835,98.1995149608939,99.1919348011075,100.184354641321,
101.176774481535,102.169194321748,103.161614161962,103.672557568463),
 .UNSPECIFIED.);
#5538=B_SPLINE_CURVE_WITH_KNOTS('',3,(#35315,#35316,#35317,#35318,#35319,
#35320,#35321,#35322,#35323,#35324),.UNSPECIFIED.,.F.,.F.,(4,1,1,1,1,1,
1,4),(97.3893722612835,97.7616667049171,98.7540865451307,99.7465063853443,
100.738926225558,101.731346065772,102.723765905985,103.672557568463),
 .UNSPECIFIED.);
#5539=B_SPLINE_CURVE_WITH_KNOTS('',3,(#35329,#35330,#35331,#35332,#35333,
#35334,#35335,#35336,#35337,#35338,#35339),.UNSPECIFIED.,.F.,.F.,(4,1,1,
1,1,1,1,1,4),(91.106186954104,91.2525760793984,92.2449959196121,93.2374157598257,
94.2298356000393,95.222255440253,96.2146752804666,97.2070951206802,97.3893722612835),
 .UNSPECIFIED.);
#5540=B_SPLINE_CURVE_WITH_KNOTS('',3,(#35340,#35341,#35342,#35343,#35344,
#35345,#35346,#35347,#35348,#35349),.UNSPECIFIED.,.F.,.F.,(4,1,1,1,1,1,
1,4),(91.106186954104,91.8071476636353,92.7995675038489,93.7919873440625,
94.7844071842762,95.7768270244898,96.7692468647034,97.3893722612835),
 .UNSPECIFIED.);
#5541=B_SPLINE_CURVE_WITH_KNOTS('',3,(#35354,#35355,#35356,#35357,#35358,
#35359,#35360,#35361,#35362,#35363),.UNSPECIFIED.,.F.,.F.,(4,1,1,1,1,1,
1,4),(84.8230016469244,85.2980570381166,86.2904768783303,87.2828967185439,
88.2753165587575,89.2677363989712,90.2601562391848,91.106186954104),
 .UNSPECIFIED.);
#5542=B_SPLINE_CURVE_WITH_KNOTS('',3,(#35364,#35365,#35366,#35367,#35368,
#35369,#35370,#35371,#35372,#35373,#35374),.UNSPECIFIED.,.F.,.F.,(4,1,1,
1,1,1,1,1,4),(84.8230016469244,84.8602087821398,85.8526286223535,86.8450484625671,
87.8374683027807,88.8298881429944,89.822307983208,90.8147278234216,91.106186954104),
 .UNSPECIFIED.);
#5543=B_SPLINE_CURVE_WITH_KNOTS('',3,(#35379,#35380,#35381,#35382,#35383,
#35384,#35385,#35386,#35387,#35388),.UNSPECIFIED.,.F.,.F.,(4,1,1,1,1,1,
1,4),(78.5398163397448,79.3435379968348,80.3359578370484,81.3283776772621,
82.3207975174757,83.3132173576894,84.305637197903,84.8230016469244),
 .UNSPECIFIED.);
#5544=B_SPLINE_CURVE_WITH_KNOTS('',3,(#35389,#35390,#35391,#35392,#35393,
#35394,#35395,#35396,#35397,#35398),.UNSPECIFIED.,.F.,.F.,(4,1,1,1,1,1,
1,4),(78.5398163397448,78.905689740858,79.8981095810717,80.8905294212853,
81.8829492614989,82.8753691017126,83.8677889419262,84.8230016469244),
 .UNSPECIFIED.);
#5545=B_SPLINE_CURVE_WITH_KNOTS('',3,(#35403,#35404,#35405,#35406,#35407,
#35408,#35409,#35410,#35411,#35412,#35413),.UNSPECIFIED.,.F.,.F.,(4,1,1,
1,1,1,1,1,4),(72.2566310325653,72.3965991153394,73.389018955553,74.3814387957666,
75.3738586359803,76.3662784761939,77.3586983164075,78.3511181566212,78.5398163397448),
 .UNSPECIFIED.);
#5546=B_SPLINE_CURVE_WITH_KNOTS('',3,(#35414,#35415,#35416,#35417,#35418,
#35419,#35420,#35421,#35422,#35423),.UNSPECIFIED.,.F.,.F.,(4,1,1,1,1,1,
1,4),(72.2566310325651,72.9511706995762,73.9435905397899,74.9360103800035,
75.9284302202171,76.9208500604308,77.9132699006444,78.5398163397448),
 .UNSPECIFIED.);
#5547=B_SPLINE_CURVE_WITH_KNOTS('',3,(#35428,#35429,#35430,#35431,#35432,
#35433,#35434,#35435,#35436,#35437),.UNSPECIFIED.,.F.,.F.,(4,1,1,1,1,1,
1,4),(65.9734457253856,66.4420800740576,67.4344999142712,68.4269197544848,
69.4193395946985,70.4117594349121,71.4041792751257,72.2566310325653),
 .UNSPECIFIED.);
#5548=B_SPLINE_CURVE_WITH_KNOTS('',3,(#35438,#35439,#35440,#35441,#35442,
#35443,#35444,#35445,#35446,#35447,#35448),.UNSPECIFIED.,.F.,.F.,(4,1,1,
1,1,1,1,1,4),(65.9734457253856,66.0042318180808,66.9966516582944,67.9890714985081,
68.9814913387217,69.9739111789353,70.966331019149,71.9587508593626,72.2566310325651),
 .UNSPECIFIED.);
#5549=B_SPLINE_CURVE_WITH_KNOTS('',3,(#35453,#35454,#35455,#35456,#35457,
#35458,#35459,#35460,#35461,#35462),.UNSPECIFIED.,.F.,.F.,(4,1,1,1,1,1,
1,4),(59.690260418206,60.4875610327758,61.4799808729894,62.472400713203,
63.4648205534167,64.4572403936303,65.4496602338439,65.9734457253856),
 .UNSPECIFIED.);
#5550=B_SPLINE_CURVE_WITH_KNOTS('',3,(#35463,#35464,#35465,#35466,#35467,
#35468,#35469,#35470,#35471,#35472),.UNSPECIFIED.,.F.,.F.,(4,1,1,1,1,1,
1,4),(59.690260418206,60.049712776799,61.0421326170126,62.0345524572262,
63.0269722974399,64.0193921376535,65.0118119778672,65.9734457253856),
 .UNSPECIFIED.);
#5551=B_SPLINE_CURVE_WITH_KNOTS('',3,(#35477,#35478,#35479,#35480,#35481,
#35482,#35483,#35484,#35485,#35486,#35487),.UNSPECIFIED.,.F.,.F.,(4,1,1,
1,1,1,1,1,4),(53.4070751110265,53.5406221512803,54.533041991494,55.5254618317076,
56.5178816719212,57.5103015121349,58.5027213523485,59.4951411925621,59.690260418206),
 .UNSPECIFIED.);
#5552=B_SPLINE_CURVE_WITH_KNOTS('',3,(#35488,#35489,#35490,#35491,#35492,
#35493,#35494,#35495,#35496,#35497),.UNSPECIFIED.,.F.,.F.,(4,1,1,1,1,1,
1,4),(53.4070751110265,54.0951937355172,55.0876135757308,56.0800334159444,
57.0724532561581,58.0648730963717,59.0572929365853,59.690260418206),
 .UNSPECIFIED.);
#5553=B_SPLINE_CURVE_WITH_KNOTS('',3,(#35502,#35503,#35504,#35505,#35506,
#35507,#35508,#35509,#35510,#35511),.UNSPECIFIED.,.F.,.F.,(4,1,1,1,1,1,
1,4),(47.1238898038468,47.5861031099985,48.5785229502122,49.5709427904258,
50.5633626306394,51.5557824708531,52.5482023110667,53.4070751110265),
 .UNSPECIFIED.);
#5554=B_SPLINE_CURVE_WITH_KNOTS('',3,(#35512,#35513,#35514,#35515,#35516,
#35517,#35518,#35519,#35520,#35521,#35522),.UNSPECIFIED.,.F.,.F.,(4,1,1,
1,1,1,1,1,4),(47.1238898038468,47.1482548540217,48.1406746942354,49.133094534449,
50.1255143746626,51.1179342148763,52.1103540550899,53.1027738953035,53.4070751110265),
 .UNSPECIFIED.);
#5555=B_SPLINE_CURVE_WITH_KNOTS('',3,(#35527,#35528,#35529,#35530,#35531,
#35532,#35533,#35534,#35535,#35536),.UNSPECIFIED.,.F.,.F.,(4,1,1,1,1,1,
1,4),(40.8407044966672,41.6315840687167,42.6240039089304,43.616423749144,
44.6088435893576,45.6012634295713,46.5936832697849,47.1238898038468),
 .UNSPECIFIED.);
#5556=B_SPLINE_CURVE_WITH_KNOTS('',3,(#35537,#35538,#35539,#35540,#35541,
#35542,#35543,#35544,#35545,#35546),.UNSPECIFIED.,.F.,.F.,(4,1,1,1,1,1,
1,4),(40.8407044966672,41.1937358127399,42.1861556529536,43.1785754931672,
44.1709953333808,45.1634151735945,46.1558350138081,47.1238898038468),
 .UNSPECIFIED.);
#5557=B_SPLINE_CURVE_WITH_KNOTS('',3,(#35551,#35552,#35553,#35554,#35555,
#35556,#35557,#35558,#35559,#35560,#35561),.UNSPECIFIED.,.F.,.F.,(4,1,1,
1,1,1,1,1,4),(34.5575191894877,34.6846451872213,35.6770650274349,36.6694848676485,
37.6619047078622,38.6543245480758,39.6467443882895,40.6391642285031,40.8407044966672),
 .UNSPECIFIED.);
#5558=B_SPLINE_CURVE_WITH_KNOTS('',3,(#35562,#35563,#35564,#35565,#35566,
#35567,#35568,#35569,#35570,#35571),.UNSPECIFIED.,.F.,.F.,(4,1,1,1,1,1,
1,4),(34.5575191894877,35.2392167714581,36.2316366116718,37.2240564518854,
38.216476292099,39.2088961323127,40.2013159725263,40.8407044966672),
 .UNSPECIFIED.);
#5559=B_SPLINE_CURVE_WITH_KNOTS('',3,(#35576,#35577,#35578,#35579,#35580,
#35581,#35582,#35583,#35584,#35585),.UNSPECIFIED.,.F.,.F.,(4,1,1,1,1,1,
1,4),(28.2743338823081,28.7301261459395,29.7225459861531,30.7149658263668,
31.7073856665804,32.699805506794,33.6922253470076,34.5575191894877),
 .UNSPECIFIED.);
#5560=B_SPLINE_CURVE_WITH_KNOTS('',3,(#35586,#35587,#35588,#35589,#35590,
#35591,#35592,#35593,#35594,#35595,#35596),.UNSPECIFIED.,.F.,.F.,(4,1,1,
1,1,1,1,1,4),(28.2743338823081,28.2922778899627,29.2846977301763,30.27711757039,
31.2695374106036,32.2619572508172,33.2543770910309,34.2467969312445,34.5575191894877),
 .UNSPECIFIED.);
#5561=B_SPLINE_CURVE_WITH_KNOTS('',3,(#35601,#35602,#35603,#35604,#35605,
#35606,#35607,#35608,#35609,#35610),.UNSPECIFIED.,.F.,.F.,(4,1,1,1,1,1,
1,4),(21.9911485751285,22.7756071046577,23.7680269448713,24.7604467850849,
25.7528666252986,26.7452864655122,27.7377063057258,28.2743338823081),
 .UNSPECIFIED.);
#5562=B_SPLINE_CURVE_WITH_KNOTS('',3,(#35611,#35612,#35613,#35614,#35615,
#35616,#35617,#35618,#35619,#35620),.UNSPECIFIED.,.F.,.F.,(4,1,1,1,1,1,
1,4),(21.9911485751284,22.3377588486809,23.3301786888945,24.3225985291082,
25.3150183693218,26.3074382095354,27.2998580497491,28.2743338823081),
 .UNSPECIFIED.);
#5563=B_SPLINE_CURVE_WITH_KNOTS('',3,(#35626,#35627,#35628,#35629,#35630),
 .UNSPECIFIED.,.F.,.F.,(4,1,4),(14.3984001269718,15.3908199671854,15.7079632679489),
 .UNSPECIFIED.);
#5564=B_SPLINE_CURVE_WITH_KNOTS('',3,(#35633,#35634,#35635,#35636,#35637),
 .UNSPECIFIED.,.F.,.F.,(4,1,4),(13.8759337553363,14.8362483829486,15.7079632679489),
 .UNSPECIFIED.);
#5565=B_SPLINE_CURVE_WITH_KNOTS('',3,(#35643,#35644,#35645,#35646),
 .UNSPECIFIED.,.F.,.F.,(4,4),(95.5573427486707,96.2647245007224),
 .UNSPECIFIED.);
#5566=B_SPLINE_CURVE_WITH_KNOTS('',3,(#35654,#35655,#35656,#35657,#35658,
#35659,#35660,#35661,#35662,#35663),.UNSPECIFIED.,.F.,.F.,(4,3,3,4),(-94.2477796076938,
-93.2874649800815,-92.2950451398679,-91.8135687061554),.UNSPECIFIED.);
#5567=B_SPLINE_CURVE_WITH_KNOTS('',3,(#35668,#35669,#35670,#35671,#35672,
#35673,#35674,#35675,#35676,#35677,#35678,#35679,#35680,#35681,#35682,#35683,
#35684,#35685,#35686,#35687,#35688,#35689,#35690,#35691,#35692),
 .UNSPECIFIED.,.F.,.F.,(4,3,3,3,3,3,3,3,4),(89.2741574414911,89.317785619227,
90.3102054594406,91.3026252996542,92.2950451398679,93.2874649800815,94.2798848202951,
95.2723046605088,95.5573427486707),.UNSPECIFIED.);
#5568=B_SPLINE_CURVE_WITH_KNOTS('',3,(#35693,#35694,#35695,#35696,#35697,
#35698,#35699,#35700,#35701,#35702,#35703,#35704,#35705,#35706,#35707,#35708,
#35709,#35710,#35711,#35712,#35713,#35714),.UNSPECIFIED.,.F.,.F.,(4,3,3,
3,3,3,3,4),(-91.8135687061554,-91.3026252996542,-90.3102054594406,-89.317785619227,
-88.3253657790133,-87.3329459387997,-86.3405260985861,-85.5303833989757),
 .UNSPECIFIED.);
#5569=B_SPLINE_CURVE_WITH_KNOTS('',3,(#35719,#35720,#35721,#35722,#35723,
#35724,#35725,#35726,#35727,#35728,#35729,#35730,#35731,#35732,#35733,#35734,
#35735,#35736,#35737,#35738,#35739,#35740),.UNSPECIFIED.,.F.,.F.,(4,3,3,
3,3,3,3,4),(82.9909721343116,83.3632665779452,84.3556864181588,85.3481062583724,
86.3405260985861,87.3329459387997,88.3253657790133,89.2741574414911),
 .UNSPECIFIED.);
#5570=B_SPLINE_CURVE_WITH_KNOTS('',3,(#35741,#35742,#35743,#35744,#35745,
#35746,#35747,#35748,#35749,#35750,#35751,#35752,#35753,#35754,#35755,#35756,
#35757,#35758,#35759,#35760,#35761,#35762,#35763,#35764,#35765),
 .UNSPECIFIED.,.F.,.F.,(4,3,3,3,3,3,3,3,4),(-85.5303833989757,-85.3481062583724,
-84.3556864181588,-83.3632665779452,-82.3708467377315,-81.3784268975179,
-80.3860070573043,-79.3935872170906,-79.2471980917961),.UNSPECIFIED.);
#5571=B_SPLINE_CURVE_WITH_KNOTS('',3,(#35770,#35771,#35772,#35773,#35774,
#35775,#35776,#35777,#35778,#35779,#35780,#35781,#35782,#35783,#35784,#35785,
#35786,#35787,#35788,#35789,#35790,#35791),.UNSPECIFIED.,.F.,.F.,(4,3,3,
3,3,3,3,4),(76.7077868271319,77.4087475366634,78.401167376877,79.3935872170906,
80.3860070573043,81.3784268975179,82.3708467377315,82.9909721343116),
 .UNSPECIFIED.);
#5572=B_SPLINE_CURVE_WITH_KNOTS('',3,(#35792,#35793,#35794,#35795,#35796,
#35797,#35798,#35799,#35800,#35801,#35802,#35803,#35804,#35805,#35806,#35807,
#35808,#35809,#35810,#35811,#35812,#35813),.UNSPECIFIED.,.F.,.F.,(4,3,3,
3,3,3,3,4),(-79.2471980917961,-78.401167376877,-77.4087475366633,-76.4163276964497,
-75.4239078562361,-74.4314880160224,-73.4390681758088,-72.9640127846165),
 .UNSPECIFIED.);
#5573=B_SPLINE_CURVE_WITH_KNOTS('',3,(#35818,#35819,#35820,#35821,#35822,
#35823,#35824,#35825,#35826,#35827,#35828,#35829,#35830,#35831,#35832,#35833,
#35834,#35835,#35836,#35837,#35838,#35839,#35840,#35841,#35842),
 .UNSPECIFIED.,.F.,.F.,(4,3,3,3,3,3,3,3,4),(70.4246015199523,70.4618086551679,
71.4542284953816,72.4466483355952,73.4390681758088,74.4314880160225,75.4239078562361,
76.4163276964497,76.7077868271319),.UNSPECIFIED.);
#5574=B_SPLINE_CURVE_WITH_KNOTS('',3,(#35843,#35844,#35845,#35846,#35847,
#35848,#35849,#35850,#35851,#35852,#35853,#35854,#35855,#35856,#35857,#35858,
#35859,#35860,#35861,#35862,#35863,#35864),.UNSPECIFIED.,.F.,.F.,(4,3,3,
3,3,3,3,4),(-72.9640127846165,-72.4466483355952,-71.4542284953815,-70.4618086551679,
-69.4693888149543,-68.4769689747406,-67.484549134527,-66.680827477437),
 .UNSPECIFIED.);
#5575=B_SPLINE_CURVE_WITH_KNOTS('',3,(#35869,#35870,#35871,#35872,#35873,
#35874,#35875,#35876,#35877,#35878,#35879,#35880,#35881,#35882,#35883,#35884,
#35885,#35886,#35887,#35888,#35889,#35890),.UNSPECIFIED.,.F.,.F.,(4,3,3,
3,3,3,3,4),(64.1414162127728,64.5072896138861,65.4997094540998,66.4921292943134,
67.484549134527,68.4769689747407,69.4693888149543,70.4246015199523),
 .UNSPECIFIED.);
#5576=B_SPLINE_CURVE_WITH_KNOTS('',3,(#35891,#35892,#35893,#35894,#35895,
#35896,#35897,#35898,#35899,#35900,#35901,#35902,#35903,#35904,#35905,#35906,
#35907,#35908,#35909,#35910,#35911,#35912,#35913,#35914,#35915),
 .UNSPECIFIED.,.F.,.F.,(4,3,3,3,3,3,3,3,4),(-66.680827477437,-66.4921292943134,
-65.4997094540998,-64.5072896138861,-63.5148697736725,-62.5224499334589,
-61.5300300932452,-60.5376102530316,-60.3976421702573),.UNSPECIFIED.);
#5577=B_SPLINE_CURVE_WITH_KNOTS('',3,(#35920,#35921,#35922,#35923,#35924,
#35925,#35926,#35927,#35928,#35929,#35930,#35931,#35932,#35933,#35934,#35935,
#35936,#35937,#35938,#35939,#35940,#35941),.UNSPECIFIED.,.F.,.F.,(4,3,3,
3,3,3,3,4),(57.8582309055932,58.5527705726043,59.545190412818,60.5376102530316,
61.5300300932452,62.5224499334589,63.5148697736725,64.1414162127728),
 .UNSPECIFIED.);
#5578=B_SPLINE_CURVE_WITH_KNOTS('',3,(#35942,#35943,#35944,#35945,#35946,
#35947,#35948,#35949,#35950,#35951,#35952,#35953,#35954,#35955,#35956,#35957,
#35958,#35959,#35960,#35961,#35962,#35963),.UNSPECIFIED.,.F.,.F.,(4,3,3,
3,3,3,3,4),(-60.3976421702573,-59.545190412818,-58.5527705726043,-57.5603507323907,
-56.5679308921771,-55.5755110519634,-54.5830912117498,-54.1144568630777),
 .UNSPECIFIED.);
#5579=B_SPLINE_CURVE_WITH_KNOTS('',3,(#35968,#35969,#35970,#35971,#35972,
#35973,#35974,#35975,#35976,#35977,#35978,#35979,#35980,#35981,#35982,#35983,
#35984,#35985,#35986,#35987,#35988,#35989,#35990,#35991,#35992),
 .UNSPECIFIED.,.F.,.F.,(4,3,3,3,3,3,3,3,4),(51.5750455984135,51.6058316911089,
52.5982515313225,53.5906713715362,54.5830912117498,55.5755110519634,56.5679308921771,
57.5603507323907,57.8582309055932),.UNSPECIFIED.);
#5580=B_SPLINE_CURVE_WITH_KNOTS('',3,(#35993,#35994,#35995,#35996,#35997,
#35998,#35999,#36000,#36001,#36002,#36003,#36004,#36005,#36006,#36007,#36008,
#36009,#36010,#36011,#36012,#36013,#36014),.UNSPECIFIED.,.F.,.F.,(4,3,3,
3,3,3,3,4),(-54.1144568630777,-53.5906713715362,-52.5982515313225,-51.6058316911089,
-50.6134118508953,-49.6209920106816,-48.628572170468,-47.8312715558982),
 .UNSPECIFIED.);
#5581=B_SPLINE_CURVE_WITH_KNOTS('',3,(#36019,#36020,#36021,#36022,#36023,
#36024,#36025,#36026,#36027,#36028,#36029,#36030,#36031,#36032,#36033,#36034,
#36035,#36036,#36037,#36038,#36039,#36040),.UNSPECIFIED.,.F.,.F.,(4,3,3,
3,3,3,3,4),(45.291860291234,45.6513126498271,46.6437324900408,47.6361523302544,
48.628572170468,49.6209920106816,50.6134118508953,51.5750455984135),
 .UNSPECIFIED.);
#5582=B_SPLINE_CURVE_WITH_KNOTS('',3,(#36041,#36042,#36043,#36044,#36045,
#36046,#36047,#36048,#36049,#36050,#36051,#36052,#36053,#36054,#36055,#36056,
#36057,#36058,#36059,#36060,#36061,#36062,#36063,#36064,#36065),
 .UNSPECIFIED.,.F.,.F.,(4,3,3,3,3,3,3,3,4),(-47.8312715558982,-47.6361523302544,
-46.6437324900407,-45.6513126498271,-44.6588928096135,-43.6664729693998,
-42.6740531291862,-41.6816332889726,-41.5480862487186),.UNSPECIFIED.);
#5583=B_SPLINE_CURVE_WITH_KNOTS('',3,(#36070,#36071,#36072,#36073,#36074,
#36075,#36076,#36077,#36078,#36079,#36080,#36081,#36082,#36083,#36084,#36085,
#36086,#36087,#36088,#36089,#36090,#36091),.UNSPECIFIED.,.F.,.F.,(4,3,3,
3,3,3,3,4),(39.0086749840544,39.6967936085453,40.6892134487589,41.6816332889726,
42.6740531291862,43.6664729693998,44.6588928096135,45.291860291234),
 .UNSPECIFIED.);
#5584=B_SPLINE_CURVE_WITH_KNOTS('',3,(#36092,#36093,#36094,#36095,#36096,
#36097,#36098,#36099,#36100,#36101,#36102,#36103,#36104,#36105,#36106,#36107,
#36108,#36109,#36110,#36111,#36112,#36113),.UNSPECIFIED.,.F.,.F.,(4,3,3,
3,3,3,3,4),(-41.5480862487186,-40.6892134487589,-39.6967936085453,-38.7043737683317,
-37.711953928118,-36.7195340879044,-35.7271142476908,-35.2649009415389),
 .UNSPECIFIED.);
#5585=B_SPLINE_CURVE_WITH_KNOTS('',3,(#36118,#36119,#36120,#36121,#36122,
#36123,#36124,#36125,#36126,#36127,#36128,#36129,#36130,#36131,#36132,#36133,
#36134,#36135,#36136,#36137,#36138,#36139,#36140,#36141,#36142),
 .UNSPECIFIED.,.F.,.F.,(4,3,3,3,3,3,3,3,4),(32.7254896768748,32.7498547270499,
33.7422745672635,34.7346944074771,35.7271142476908,36.7195340879044,37.711953928118,
38.7043737683317,39.0086749840544),.UNSPECIFIED.);
#5586=B_SPLINE_CURVE_WITH_KNOTS('',3,(#36143,#36144,#36145,#36146,#36147,
#36148,#36149,#36150,#36151,#36152,#36153,#36154,#36155,#36156,#36157,#36158,
#36159,#36160,#36161,#36162,#36163,#36164),.UNSPECIFIED.,.F.,.F.,(4,3,3,
3,3,3,3,4),(-35.2649009415389,-34.7346944074771,-33.7422745672635,-32.7498547270499,
-31.7574348868362,-30.7650150466226,-29.772595206409,-28.9817156343594),
 .UNSPECIFIED.);
#5587=B_SPLINE_CURVE_WITH_KNOTS('',3,(#36169,#36170,#36171,#36172,#36173,
#36174,#36175,#36176,#36177,#36178,#36179,#36180,#36181,#36182,#36183,#36184,
#36185,#36186,#36187,#36188,#36189,#36190),.UNSPECIFIED.,.F.,.F.,(4,3,3,
3,3,3,3,4),(26.4423043696952,26.7953356857681,27.7877555259817,28.7801753661954,
29.772595206409,30.7650150466226,31.7574348868363,32.7254896768748),
 .UNSPECIFIED.);
#5588=B_SPLINE_CURVE_WITH_KNOTS('',3,(#36191,#36192,#36193,#36194,#36195,
#36196,#36197,#36198,#36199,#36200,#36201,#36202,#36203,#36204,#36205,#36206,
#36207,#36208,#36209,#36210,#36211,#36212,#36213,#36214,#36215),
 .UNSPECIFIED.,.F.,.F.,(4,3,3,3,3,3,3,3,4),(-28.9817156343594,-28.7801753661953,
-27.7877555259817,-26.7953356857681,-25.8029158455544,-24.8104960053408,
-23.8180761651272,-22.8256563249135,-22.6985303271798),.UNSPECIFIED.);
#5589=B_SPLINE_CURVE_WITH_KNOTS('',3,(#36220,#36221,#36222,#36223,#36224,
#36225,#36226,#36227,#36228,#36229,#36230,#36231,#36232,#36233,#36234,#36235,
#36236,#36237,#36238,#36239,#36240,#36241),.UNSPECIFIED.,.F.,.F.,(4,3,3,
3,3,3,3,4),(20.1591190625156,20.8408166444863,21.8332364846999,22.8256563249136,
23.8180761651272,24.8104960053408,25.8029158455545,26.4423043696952),
 .UNSPECIFIED.);
#5590=B_SPLINE_CURVE_WITH_KNOTS('',3,(#36242,#36243,#36244,#36245,#36246,
#36247,#36248,#36249,#36250,#36251,#36252,#36253,#36254,#36255,#36256,#36257,
#36258,#36259,#36260,#36261,#36262,#36263),.UNSPECIFIED.,.F.,.F.,(4,3,3,
3,3,3,3,4),(-22.6985303271798,-21.8332364846999,-20.8408166444863,-19.8483968042727,
-18.855976964059,-17.8635571238454,-16.8711372836318,-16.4153450200002),
 .UNSPECIFIED.);
#5591=B_SPLINE_CURVE_WITH_KNOTS('',3,(#36268,#36269,#36270,#36271,#36272,
#36273,#36274,#36275,#36276,#36277,#36278,#36279,#36280,#36281,#36282,#36283,
#36284,#36285,#36286,#36287,#36288,#36289,#36290,#36291,#36292),
 .UNSPECIFIED.,.F.,.F.,(4,3,3,3,3,3,3,3,4),(13.875933755336,13.8938777629909,
14.8862976032045,15.8787174434181,16.8711372836318,17.8635571238454,18.855976964059,
19.8483968042727,20.1591190625156),.UNSPECIFIED.);
#5592=B_SPLINE_CURVE_WITH_KNOTS('',3,(#36293,#36294,#36295,#36296,#36297,
#36298,#36299,#36300,#36301,#36302,#36303,#36304,#36305,#36306,#36307,#36308,
#36309,#36310,#36311,#36312,#36313,#36314),.UNSPECIFIED.,.F.,.F.,(4,3,3,
3,3,3,3,4),(-16.4153450200002,-15.8787174434181,-14.8862976032045,-13.8938777629909,
-12.9014579227772,-11.9090380825636,-10.91661824235,-10.1321597128207),
 .UNSPECIFIED.);
#5593=B_SPLINE_CURVE_WITH_KNOTS('',3,(#36320,#36321,#36322,#36323,#36324,
#36325,#36326,#36327,#36328,#36329,#36330,#36331,#36332),.UNSPECIFIED.,
 .F.,.F.,(4,3,3,3,4),(-3.848974405641,-2.9772595206409,-1.98483968042726,
-0.992419840213632,0.),.UNSPECIFIED.);
#5594=B_SPLINE_CURVE_WITH_KNOTS('',3,(#36335,#36336,#36337,#36338,#36339,
#36340,#36341,#36342,#36343,#36344,#36345,#36346,#36347,#36348,#36349,#36350,
#36351,#36352,#36353),.UNSPECIFIED.,.F.,.F.,(4,3,3,3,3,3,4),(2.01694489302852,
2.9772595206409,3.96967936085453,4.96209920106817,5.9545190412818,6.94693888149543,
7.59274844815647),.UNSPECIFIED.);
#5595=B_SPLINE_CURVE_WITH_KNOTS('',3,(#36359,#36360,#36361,#36362,#36363,
#36364,#36365,#36366),.UNSPECIFIED.,.F.,.F.,(4,1,1,1,1,4),(103.672557568463,
104.154034002176,105.146453842389,106.138873682603,107.131293522817,108.12371336303),
 .UNSPECIFIED.);
#5596=B_SPLINE_CURVE_WITH_KNOTS('',3,(#36369,#36370,#36371,#36372,#36373,
#36374,#36375,#36376,#36377),.UNSPECIFIED.,.F.,.F.,(4,1,1,1,1,1,4),(103.672557568463,
103.716185746199,104.708605586413,105.701025426626,106.69344526684,107.685865107053,
108.646179734666),.UNSPECIFIED.);
#5597=B_SPLINE_CURVE_WITH_KNOTS('',3,(#36382,#36383,#36384,#36385,#36386,
#36387,#36388,#36389,#36390,#36391),.UNSPECIFIED.,.F.,.F.,(4,1,1,1,1,1,
1,4),(97.3893722612835,98.1995149608939,99.1919348011075,100.184354641321,
101.176774481535,102.169194321748,103.161614161962,103.672557568463),
 .UNSPECIFIED.);
#5598=B_SPLINE_CURVE_WITH_KNOTS('',3,(#36392,#36393,#36394,#36395,#36396,
#36397,#36398,#36399,#36400,#36401),.UNSPECIFIED.,.F.,.F.,(4,1,1,1,1,1,
1,4),(97.3893722612835,97.7616667049171,98.7540865451307,99.7465063853444,
100.738926225558,101.731346065772,102.723765905985,103.672557568463),
 .UNSPECIFIED.);
#5599=B_SPLINE_CURVE_WITH_KNOTS('',3,(#36406,#36407,#36408,#36409,#36410,
#36411,#36412,#36413,#36414,#36415,#36416),.UNSPECIFIED.,.F.,.F.,(4,1,1,
1,1,1,1,1,4),(91.106186954104,91.2525760793984,92.2449959196121,93.2374157598257,
94.2298356000393,95.222255440253,96.2146752804666,97.2070951206802,97.3893722612835),
 .UNSPECIFIED.);
#5600=B_SPLINE_CURVE_WITH_KNOTS('',3,(#36417,#36418,#36419,#36420,#36421,
#36422,#36423,#36424,#36425,#36426),.UNSPECIFIED.,.F.,.F.,(4,1,1,1,1,1,
1,4),(91.106186954104,91.8071476636353,92.7995675038489,93.7919873440626,
94.7844071842762,95.7768270244898,96.7692468647035,97.3893722612835),
 .UNSPECIFIED.);
#5601=B_SPLINE_CURVE_WITH_KNOTS('',3,(#36431,#36432,#36433,#36434,#36435,
#36436,#36437,#36438,#36439,#36440),.UNSPECIFIED.,.F.,.F.,(4,1,1,1,1,1,
1,4),(84.8230016469244,85.2980570381166,86.2904768783303,87.2828967185439,
88.2753165587575,89.2677363989712,90.2601562391848,91.106186954104),
 .UNSPECIFIED.);
#5602=B_SPLINE_CURVE_WITH_KNOTS('',3,(#36441,#36442,#36443,#36444,#36445,
#36446,#36447,#36448,#36449,#36450,#36451),.UNSPECIFIED.,.F.,.F.,(4,1,1,
1,1,1,1,1,4),(84.8230016469244,84.8602087821399,85.8526286223535,86.8450484625671,
87.8374683027808,88.8298881429944,89.822307983208,90.8147278234217,91.106186954104),
 .UNSPECIFIED.);
#5603=B_SPLINE_CURVE_WITH_KNOTS('',3,(#36456,#36457,#36458,#36459,#36460,
#36461,#36462,#36463,#36464,#36465),.UNSPECIFIED.,.F.,.F.,(4,1,1,1,1,1,
1,4),(78.5398163397448,79.3435379968348,80.3359578370485,81.3283776772621,
82.3207975174757,83.3132173576894,84.305637197903,84.8230016469244),
 .UNSPECIFIED.);
#5604=B_SPLINE_CURVE_WITH_KNOTS('',3,(#36466,#36467,#36468,#36469,#36470,
#36471,#36472,#36473,#36474,#36475),.UNSPECIFIED.,.F.,.F.,(4,1,1,1,1,1,
1,4),(78.5398163397448,78.9056897408581,79.8981095810717,80.8905294212853,
81.882949261499,82.8753691017126,83.8677889419262,84.8230016469244),
 .UNSPECIFIED.);
#5605=B_SPLINE_CURVE_WITH_KNOTS('',3,(#36480,#36481,#36482,#36483,#36484,
#36485,#36486,#36487,#36488,#36489,#36490),.UNSPECIFIED.,.F.,.F.,(4,1,1,
1,1,1,1,1,4),(72.2566310325653,72.3965991153394,73.389018955553,74.3814387957667,
75.3738586359803,76.3662784761939,77.3586983164076,78.3511181566212,78.5398163397448),
 .UNSPECIFIED.);
#5606=B_SPLINE_CURVE_WITH_KNOTS('',3,(#36491,#36492,#36493,#36494,#36495,
#36496,#36497,#36498,#36499,#36500),.UNSPECIFIED.,.F.,.F.,(4,1,1,1,1,1,
1,4),(72.2566310325651,72.9511706995763,73.9435905397899,74.9360103800035,
75.9284302202172,76.9208500604308,77.9132699006444,78.5398163397448),
 .UNSPECIFIED.);
#5607=B_SPLINE_CURVE_WITH_KNOTS('',3,(#36505,#36506,#36507,#36508,#36509,
#36510,#36511,#36512,#36513,#36514),.UNSPECIFIED.,.F.,.F.,(4,1,1,1,1,1,
1,4),(65.9734457253856,66.4420800740576,67.4344999142712,68.4269197544849,
69.4193395946985,70.4117594349121,71.4041792751258,72.2566310325653),
 .UNSPECIFIED.);
#5608=B_SPLINE_CURVE_WITH_KNOTS('',3,(#36515,#36516,#36517,#36518,#36519,
#36520,#36521,#36522,#36523,#36524,#36525),.UNSPECIFIED.,.F.,.F.,(4,1,1,
1,1,1,1,1,4),(65.9734457253856,66.0042318180808,66.9966516582945,67.9890714985081,
68.9814913387217,69.9739111789354,70.966331019149,71.9587508593626,72.2566310325651),
 .UNSPECIFIED.);
#5609=B_SPLINE_CURVE_WITH_KNOTS('',3,(#36530,#36531,#36532,#36533,#36534,
#36535,#36536,#36537,#36538,#36539),.UNSPECIFIED.,.F.,.F.,(4,1,1,1,1,1,
1,4),(59.690260418206,60.4875610327758,61.4799808729895,62.4724007132031,
63.4648205534167,64.4572403936303,65.449660233844,65.9734457253856),
 .UNSPECIFIED.);
#5610=B_SPLINE_CURVE_WITH_KNOTS('',3,(#36540,#36541,#36542,#36543,#36544,
#36545,#36546,#36547,#36548,#36549),.UNSPECIFIED.,.F.,.F.,(4,1,1,1,1,1,
1,4),(59.690260418206,60.049712776799,61.0421326170127,62.0345524572263,
63.0269722974399,64.0193921376536,65.0118119778672,65.9734457253856),
 .UNSPECIFIED.);
#5611=B_SPLINE_CURVE_WITH_KNOTS('',3,(#36554,#36555,#36556,#36557,#36558,
#36559,#36560,#36561,#36562,#36563,#36564),.UNSPECIFIED.,.F.,.F.,(4,1,1,
1,1,1,1,1,4),(53.4070751110265,53.5406221512804,54.533041991494,55.5254618317077,
56.5178816719213,57.5103015121349,58.5027213523486,59.4951411925622,59.690260418206),
 .UNSPECIFIED.);
#5612=B_SPLINE_CURVE_WITH_KNOTS('',3,(#36565,#36566,#36567,#36568,#36569,
#36570,#36571,#36572,#36573,#36574),.UNSPECIFIED.,.F.,.F.,(4,1,1,1,1,1,
1,4),(53.4070751110265,54.0951937355172,55.0876135757309,56.0800334159445,
57.0724532561581,58.0648730963718,59.0572929365854,59.690260418206),
 .UNSPECIFIED.);
#5613=B_SPLINE_CURVE_WITH_KNOTS('',3,(#36579,#36580,#36581,#36582,#36583,
#36584,#36585,#36586,#36587,#36588),.UNSPECIFIED.,.F.,.F.,(4,1,1,1,1,1,
1,4),(47.1238898038468,47.5861031099986,48.5785229502122,49.5709427904259,
50.5633626306395,51.5557824708531,52.5482023110668,53.4070751110265),
 .UNSPECIFIED.);
#5614=B_SPLINE_CURVE_WITH_KNOTS('',3,(#36589,#36590,#36591,#36592,#36593,
#36594,#36595,#36596,#36597,#36598,#36599),.UNSPECIFIED.,.F.,.F.,(4,1,1,
1,1,1,1,1,4),(47.1238898038468,47.1482548540218,48.1406746942354,49.1330945344491,
50.1255143746627,51.1179342148763,52.11035405509,53.1027738953036,53.4070751110265),
 .UNSPECIFIED.);
#5615=B_SPLINE_CURVE_WITH_KNOTS('',3,(#36604,#36605,#36606,#36607,#36608,
#36609,#36610,#36611,#36612,#36613),.UNSPECIFIED.,.F.,.F.,(4,1,1,1,1,1,
1,4),(40.8407044966672,41.6315840687168,42.6240039089304,43.6164237491441,
44.6088435893577,45.6012634295713,46.593683269785,47.1238898038468),
 .UNSPECIFIED.);
#5616=B_SPLINE_CURVE_WITH_KNOTS('',3,(#36614,#36615,#36616,#36617,#36618,
#36619,#36620,#36621,#36622,#36623),.UNSPECIFIED.,.F.,.F.,(4,1,1,1,1,1,
1,4),(40.8407044966672,41.19373581274,42.1861556529536,43.1785754931673,
44.1709953333809,45.1634151735945,46.1558350138082,47.1238898038468),
 .UNSPECIFIED.);
#5617=B_SPLINE_CURVE_WITH_KNOTS('',3,(#36628,#36629,#36630,#36631,#36632,
#36633,#36634,#36635,#36636,#36637,#36638),.UNSPECIFIED.,.F.,.F.,(4,1,1,
1,1,1,1,1,4),(34.5575191894877,34.6846451872214,35.677065027435,36.6694848676486,
37.6619047078623,38.6543245480759,39.6467443882895,40.6391642285032,40.8407044966672),
 .UNSPECIFIED.);
#5618=B_SPLINE_CURVE_WITH_KNOTS('',3,(#36639,#36640,#36641,#36642,#36643,
#36644,#36645,#36646,#36647,#36648),.UNSPECIFIED.,.F.,.F.,(4,1,1,1,1,1,
1,4),(34.5575191894877,35.2392167714582,36.2316366116718,37.2240564518855,
38.2164762920991,39.2088961323127,40.2013159725264,40.8407044966672),
 .UNSPECIFIED.);
#5619=B_SPLINE_CURVE_WITH_KNOTS('',3,(#36653,#36654,#36655,#36656,#36657,
#36658,#36659,#36660,#36661,#36662),.UNSPECIFIED.,.F.,.F.,(4,1,1,1,1,1,
1,4),(28.2743338823081,28.7301261459396,29.7225459861532,30.7149658263668,
31.7073856665805,32.6998055067941,33.6922253470077,34.5575191894877),
 .UNSPECIFIED.);
#5620=B_SPLINE_CURVE_WITH_KNOTS('',3,(#36663,#36664,#36665,#36666,#36667,
#36668,#36669,#36670,#36671,#36672,#36673),.UNSPECIFIED.,.F.,.F.,(4,1,1,
1,1,1,1,1,4),(28.2743338823081,28.2922778899628,29.2846977301764,30.2771175703901,
31.2695374106037,32.2619572508173,33.2543770910309,34.2467969312446,34.5575191894877),
 .UNSPECIFIED.);
#5621=B_SPLINE_CURVE_WITH_KNOTS('',3,(#36678,#36679,#36680,#36681,#36682,
#36683,#36684,#36685,#36686,#36687),.UNSPECIFIED.,.F.,.F.,(4,1,1,1,1,1,
1,4),(21.9911485751285,22.7756071046578,23.7680269448714,24.760446785085,
25.7528666252987,26.7452864655123,27.7377063057259,28.2743338823081),
 .UNSPECIFIED.);
#5622=B_SPLINE_CURVE_WITH_KNOTS('',3,(#36688,#36689,#36690,#36691,#36692,
#36693,#36694,#36695,#36696,#36697),.UNSPECIFIED.,.F.,.F.,(4,1,1,1,1,1,
1,4),(21.9911485751284,22.337758848681,23.3301786888946,24.3225985291083,
25.3150183693219,26.3074382095355,27.2998580497492,28.2743338823081),
 .UNSPECIFIED.);
#5623=B_SPLINE_CURVE_WITH_KNOTS('',3,(#36703,#36704,#36705,#36706,#36707),
 .UNSPECIFIED.,.F.,.F.,(4,1,4),(14.3984001269719,15.3908199671856,15.7079632679489),
 .UNSPECIFIED.);
#5624=B_SPLINE_CURVE_WITH_KNOTS('',3,(#36710,#36711,#36712,#36713,#36714),
 .UNSPECIFIED.,.F.,.F.,(4,1,4),(13.8759337553364,14.8362483829487,15.7079632679489),
 .UNSPECIFIED.);
#5625=B_SPLINE_CURVE_WITH_KNOTS('',3,(#36720,#36721,#36722,#36723),
 .UNSPECIFIED.,.F.,.F.,(4,4),(95.5573427486708,96.2647245007224),
 .UNSPECIFIED.);
#5626=B_SPLINE_CURVE_WITH_KNOTS('',3,(#36731,#36732,#36733,#36734,#36735,
#36736,#36737,#36738,#36739,#36740),.UNSPECIFIED.,.F.,.F.,(4,3,3,4),(-94.2477796076939,
-93.2874649800816,-92.295045139868,-91.8135687061555),.UNSPECIFIED.);
#5627=B_SPLINE_CURVE_WITH_KNOTS('',3,(#36745,#36746,#36747,#36748,#36749,
#36750,#36751,#36752,#36753,#36754,#36755,#36756,#36757,#36758,#36759,#36760,
#36761,#36762,#36763,#36764,#36765,#36766,#36767,#36768,#36769),
 .UNSPECIFIED.,.F.,.F.,(4,3,3,3,3,3,3,3,4),(89.2741574414912,89.3177856192271,
90.3102054594407,91.3026252996544,92.295045139868,93.2874649800816,94.2798848202953,
95.2723046605089,95.5573427486708),.UNSPECIFIED.);
#5628=B_SPLINE_CURVE_WITH_KNOTS('',3,(#36770,#36771,#36772,#36773,#36774,
#36775,#36776,#36777,#36778,#36779,#36780,#36781,#36782,#36783,#36784,#36785,
#36786,#36787,#36788,#36789,#36790,#36791),.UNSPECIFIED.,.F.,.F.,(4,3,3,
3,3,3,3,4),(-91.8135687061555,-91.3026252996543,-90.3102054594407,-89.3177856192271,
-88.3253657790134,-87.3329459387998,-86.3405260985862,-85.5303833989759),
 .UNSPECIFIED.);
#5629=B_SPLINE_CURVE_WITH_KNOTS('',3,(#36796,#36797,#36798,#36799,#36800,
#36801,#36802,#36803,#36804,#36805,#36806,#36807,#36808,#36809,#36810,#36811,
#36812,#36813,#36814,#36815,#36816,#36817),.UNSPECIFIED.,.F.,.F.,(4,3,3,
3,3,3,3,4),(82.9909721343117,83.3632665779453,84.3556864181589,85.3481062583725,
86.3405260985862,87.3329459387998,88.3253657790134,89.2741574414912),
 .UNSPECIFIED.);
#5630=B_SPLINE_CURVE_WITH_KNOTS('',3,(#36818,#36819,#36820,#36821,#36822,
#36823,#36824,#36825,#36826,#36827,#36828,#36829,#36830,#36831,#36832,#36833,
#36834,#36835,#36836,#36837,#36838,#36839,#36840,#36841,#36842),
 .UNSPECIFIED.,.F.,.F.,(4,3,3,3,3,3,3,3,4),(-85.5303833989759,-85.3481062583725,
-84.3556864181589,-83.3632665779453,-82.3708467377316,-81.378426897518,
-80.3860070573044,-79.3935872170907,-79.2471980917963),.UNSPECIFIED.);
#5631=B_SPLINE_CURVE_WITH_KNOTS('',3,(#36847,#36848,#36849,#36850,#36851,
#36852,#36853,#36854,#36855,#36856,#36857,#36858,#36859,#36860,#36861,#36862,
#36863,#36864,#36865,#36866,#36867,#36868),.UNSPECIFIED.,.F.,.F.,(4,3,3,
3,3,3,3,4),(76.7077868271321,77.4087475366635,78.4011673768771,79.3935872170907,
80.3860070573044,81.378426897518,82.3708467377316,82.9909721343117),
 .UNSPECIFIED.);
#5632=B_SPLINE_CURVE_WITH_KNOTS('',3,(#36869,#36870,#36871,#36872,#36873,
#36874,#36875,#36876,#36877,#36878,#36879,#36880,#36881,#36882,#36883,#36884,
#36885,#36886,#36887,#36888,#36889,#36890),.UNSPECIFIED.,.F.,.F.,(4,3,3,
3,3,3,3,4),(-79.2471980917963,-78.4011673768771,-77.4087475366634,-76.4163276964498,
-75.4239078562362,-74.4314880160225,-73.4390681758089,-72.9640127846167),
 .UNSPECIFIED.);
#5633=B_SPLINE_CURVE_WITH_KNOTS('',3,(#36895,#36896,#36897,#36898,#36899,
#36900,#36901,#36902,#36903,#36904,#36905,#36906,#36907,#36908,#36909,#36910,
#36911,#36912,#36913,#36914,#36915,#36916,#36917,#36918,#36919),
 .UNSPECIFIED.,.F.,.F.,(4,3,3,3,3,3,3,3,4),(70.4246015199524,70.461808655168,
71.4542284953817,72.4466483355953,73.4390681758089,74.4314880160226,75.4239078562362,
76.4163276964498,76.7077868271321),.UNSPECIFIED.);
#5634=B_SPLINE_CURVE_WITH_KNOTS('',3,(#36920,#36921,#36922,#36923,#36924,
#36925,#36926,#36927,#36928,#36929,#36930,#36931,#36932,#36933,#36934,#36935,
#36936,#36937,#36938,#36939,#36940,#36941),.UNSPECIFIED.,.F.,.F.,(4,3,3,
3,3,3,3,4),(-72.9640127846167,-72.4466483355953,-71.4542284953816,-70.461808655168,
-69.4693888149544,-68.4769689747407,-67.4845491345271,-66.6808274774371),
 .UNSPECIFIED.);
#5635=B_SPLINE_CURVE_WITH_KNOTS('',3,(#36946,#36947,#36948,#36949,#36950,
#36951,#36952,#36953,#36954,#36955,#36956,#36957,#36958,#36959,#36960,#36961,
#36962,#36963,#36964,#36965,#36966,#36967),.UNSPECIFIED.,.F.,.F.,(4,3,3,
3,3,3,3,4),(64.1414162127729,64.5072896138862,65.4997094540998,66.4921292943135,
67.4845491345271,68.4769689747407,69.4693888149544,70.4246015199524),
 .UNSPECIFIED.);
#5636=B_SPLINE_CURVE_WITH_KNOTS('',3,(#36968,#36969,#36970,#36971,#36972,
#36973,#36974,#36975,#36976,#36977,#36978,#36979,#36980,#36981,#36982,#36983,
#36984,#36985,#36986,#36987,#36988,#36989,#36990,#36991,#36992),
 .UNSPECIFIED.,.F.,.F.,(4,3,3,3,3,3,3,3,4),(-66.6808274774371,-66.4921292943135,
-65.4997094540998,-64.5072896138862,-63.5148697736726,-62.5224499334589,
-61.5300300932453,-60.5376102530317,-60.3976421702575),.UNSPECIFIED.);
#5637=B_SPLINE_CURVE_WITH_KNOTS('',3,(#36997,#36998,#36999,#37000,#37001,
#37002,#37003,#37004,#37005,#37006,#37007,#37008,#37009,#37010,#37011,#37012,
#37013,#37014,#37015,#37016,#37017,#37018),.UNSPECIFIED.,.F.,.F.,(4,3,3,
3,3,3,3,4),(57.8582309055933,58.5527705726044,59.545190412818,60.5376102530317,
61.5300300932453,62.5224499334589,63.5148697736726,64.1414162127729),
 .UNSPECIFIED.);
#5638=B_SPLINE_CURVE_WITH_KNOTS('',3,(#37019,#37020,#37021,#37022,#37023,
#37024,#37025,#37026,#37027,#37028,#37029,#37030,#37031,#37032,#37033,#37034,
#37035,#37036,#37037,#37038,#37039,#37040),.UNSPECIFIED.,.F.,.F.,(4,3,3,
3,3,3,3,4),(-60.3976421702575,-59.545190412818,-58.5527705726044,-57.5603507323908,
-56.5679308921771,-55.5755110519635,-54.5830912117499,-54.1144568630778),
 .UNSPECIFIED.);
#5639=B_SPLINE_CURVE_WITH_KNOTS('',3,(#37045,#37046,#37047,#37048,#37049,
#37050,#37051,#37052,#37053,#37054,#37055,#37056,#37057,#37058,#37059,#37060,
#37061,#37062,#37063,#37064,#37065,#37066,#37067,#37068,#37069),
 .UNSPECIFIED.,.F.,.F.,(4,3,3,3,3,3,3,3,4),(51.5750455984138,51.605831691109,
52.5982515313226,53.5906713715362,54.5830912117499,55.5755110519635,56.5679308921771,
57.5603507323908,57.8582309055933),.UNSPECIFIED.);
#5640=B_SPLINE_CURVE_WITH_KNOTS('',3,(#37070,#37071,#37072,#37073,#37074,
#37075,#37076,#37077,#37078,#37079,#37080,#37081,#37082,#37083,#37084,#37085,
#37086,#37087,#37088,#37089,#37090,#37091),.UNSPECIFIED.,.F.,.F.,(4,3,3,
3,3,3,3,4),(-54.1144568630778,-53.5906713715362,-52.5982515313226,-51.605831691109,
-50.6134118508953,-49.6209920106817,-48.6285721704681,-47.8312715558983),
 .UNSPECIFIED.);
#5641=B_SPLINE_CURVE_WITH_KNOTS('',3,(#37096,#37097,#37098,#37099,#37100,
#37101,#37102,#37103,#37104,#37105,#37106,#37107,#37108,#37109,#37110,#37111,
#37112,#37113,#37114,#37115,#37116,#37117),.UNSPECIFIED.,.F.,.F.,(4,3,3,
3,3,3,3,4),(45.2918602912341,45.6513126498272,46.6437324900408,47.6361523302544,
48.6285721704681,49.6209920106817,50.6134118508953,51.5750455984138),
 .UNSPECIFIED.);
#5642=B_SPLINE_CURVE_WITH_KNOTS('',3,(#37118,#37119,#37120,#37121,#37122,
#37123,#37124,#37125,#37126,#37127,#37128,#37129,#37130,#37131,#37132,#37133,
#37134,#37135,#37136,#37137,#37138,#37139,#37140,#37141,#37142),
 .UNSPECIFIED.,.F.,.F.,(4,3,3,3,3,3,3,3,4),(-47.8312715558983,-47.6361523302544,
-46.6437324900408,-45.6513126498272,-44.6588928096135,-43.6664729693999,
-42.6740531291863,-41.6816332889726,-41.5480862487187),.UNSPECIFIED.);
#5643=B_SPLINE_CURVE_WITH_KNOTS('',3,(#37147,#37148,#37149,#37150,#37151,
#37152,#37153,#37154,#37155,#37156,#37157,#37158,#37159,#37160,#37161,#37162,
#37163,#37164,#37165,#37166,#37167,#37168),.UNSPECIFIED.,.F.,.F.,(4,3,3,
3,3,3,3,4),(39.0086749840545,39.6967936085454,40.689213448759,41.6816332889726,
42.6740531291863,43.6664729693999,44.6588928096135,45.2918602912341),
 .UNSPECIFIED.);
#5644=B_SPLINE_CURVE_WITH_KNOTS('',3,(#37169,#37170,#37171,#37172,#37173,
#37174,#37175,#37176,#37177,#37178,#37179,#37180,#37181,#37182,#37183,#37184,
#37185,#37186,#37187,#37188,#37189,#37190),.UNSPECIFIED.,.F.,.F.,(4,3,3,
3,3,3,3,4),(-41.5480862487187,-40.689213448759,-39.6967936085454,-38.7043737683317,
-37.7119539281181,-36.7195340879045,-35.7271142476908,-35.2649009415392),
 .UNSPECIFIED.);
#5645=B_SPLINE_CURVE_WITH_KNOTS('',3,(#37195,#37196,#37197,#37198,#37199,
#37200,#37201,#37202,#37203,#37204,#37205,#37206,#37207,#37208,#37209,#37210,
#37211,#37212,#37213,#37214,#37215,#37216,#37217,#37218,#37219),
 .UNSPECIFIED.,.F.,.F.,(4,3,3,3,3,3,3,3,4),(32.725489676875,32.7498547270499,
33.7422745672636,34.7346944074772,35.7271142476908,36.7195340879045,37.7119539281181,
38.7043737683317,39.0086749840545),.UNSPECIFIED.);
#5646=B_SPLINE_CURVE_WITH_KNOTS('',3,(#37220,#37221,#37222,#37223,#37224,
#37225,#37226,#37227,#37228,#37229,#37230,#37231,#37232,#37233,#37234,#37235,
#37236,#37237,#37238,#37239,#37240,#37241),.UNSPECIFIED.,.F.,.F.,(4,3,3,
3,3,3,3,4),(-35.2649009415392,-34.7346944074772,-33.7422745672636,-32.7498547270499,
-31.7574348868363,-30.7650150466226,-29.772595206409,-28.9817156343596),
 .UNSPECIFIED.);
#5647=B_SPLINE_CURVE_WITH_KNOTS('',3,(#37246,#37247,#37248,#37249,#37250,
#37251,#37252,#37253,#37254,#37255,#37256,#37257,#37258,#37259,#37260,#37261,
#37262,#37263,#37264,#37265,#37266,#37267),.UNSPECIFIED.,.F.,.F.,(4,3,3,
3,3,3,3,4),(26.4423043696954,26.7953356857681,27.7877555259818,28.7801753661954,
29.772595206409,30.7650150466227,31.7574348868363,32.725489676875),
 .UNSPECIFIED.);
#5648=B_SPLINE_CURVE_WITH_KNOTS('',3,(#37268,#37269,#37270,#37271,#37272,
#37273,#37274,#37275,#37276,#37277,#37278,#37279,#37280,#37281,#37282,#37283,
#37284,#37285,#37286,#37287,#37288,#37289,#37290,#37291,#37292),
 .UNSPECIFIED.,.F.,.F.,(4,3,3,3,3,3,3,3,4),(-28.9817156343596,-28.7801753661954,
-27.7877555259817,-26.7953356857681,-25.8029158455545,-24.8104960053408,
-23.8180761651272,-22.8256563249136,-22.6985303271799),.UNSPECIFIED.);
#5649=B_SPLINE_CURVE_WITH_KNOTS('',3,(#37297,#37298,#37299,#37300,#37301,
#37302,#37303,#37304,#37305,#37306,#37307,#37308,#37309,#37310,#37311,#37312,
#37313,#37314,#37315,#37316,#37317,#37318),.UNSPECIFIED.,.F.,.F.,(4,3,3,
3,3,3,3,4),(20.1591190625157,20.8408166444863,21.8332364846999,22.8256563249136,
23.8180761651272,24.8104960053409,25.8029158455545,26.4423043696954),
 .UNSPECIFIED.);
#5650=B_SPLINE_CURVE_WITH_KNOTS('',3,(#37319,#37320,#37321,#37322,#37323,
#37324,#37325,#37326,#37327,#37328,#37329,#37330,#37331,#37332,#37333,#37334,
#37335,#37336,#37337,#37338,#37339,#37340),.UNSPECIFIED.,.F.,.F.,(4,3,3,
3,3,3,3,4),(-22.6985303271799,-21.8332364846999,-20.8408166444863,-19.8483968042727,
-18.855976964059,-17.8635571238454,-16.8711372836318,-16.4153450200004),
 .UNSPECIFIED.);
#5651=B_SPLINE_CURVE_WITH_KNOTS('',3,(#37345,#37346,#37347,#37348,#37349,
#37350,#37351,#37352,#37353,#37354,#37355,#37356,#37357,#37358,#37359,#37360,
#37361,#37362,#37363,#37364,#37365,#37366,#37367,#37368,#37369),
 .UNSPECIFIED.,.F.,.F.,(4,3,3,3,3,3,3,3,4),(13.8759337553361,13.8938777629909,
14.8862976032045,15.8787174434181,16.8711372836318,17.8635571238454,18.855976964059,
19.8483968042727,20.1591190625157),.UNSPECIFIED.);
#5652=B_SPLINE_CURVE_WITH_KNOTS('',3,(#37370,#37371,#37372,#37373,#37374,
#37375,#37376,#37377,#37378,#37379,#37380,#37381,#37382,#37383,#37384,#37385,
#37386,#37387,#37388,#37389,#37390,#37391),.UNSPECIFIED.,.F.,.F.,(4,3,3,
3,3,3,3,4),(-16.4153450200004,-15.8787174434181,-14.8862976032045,-13.8938777629909,
-12.9014579227772,-11.9090380825636,-10.91661824235,-10.1321597128208),
 .UNSPECIFIED.);
#5653=B_SPLINE_CURVE_WITH_KNOTS('',3,(#37397,#37398,#37399,#37400,#37401,
#37402,#37403,#37404,#37405,#37406,#37407,#37408,#37409),.UNSPECIFIED.,
 .F.,.F.,(4,3,3,3,4),(-3.84897440564123,-2.9772595206409,-1.98483968042727,
-0.99241984021363,0.),.UNSPECIFIED.);
#5654=B_SPLINE_CURVE_WITH_KNOTS('',3,(#37412,#37413,#37414,#37415,#37416,
#37417,#37418,#37419,#37420,#37421,#37422,#37423,#37424,#37425,#37426,#37427,
#37428,#37429,#37430),.UNSPECIFIED.,.F.,.F.,(4,3,3,3,3,3,4),(2.01694489302852,
2.9772595206409,3.96967936085453,4.96209920106817,5.9545190412818,6.94693888149544,
7.59274844815659),.UNSPECIFIED.);
#5655=B_SPLINE_CURVE_WITH_KNOTS('',3,(#37436,#37437,#37438,#37439,#37440,
#37441,#37442,#37443),.UNSPECIFIED.,.F.,.F.,(4,1,1,1,1,4),(103.672557568463,
104.154034002176,105.146453842389,106.138873682603,107.131293522817,108.12371336303),
 .UNSPECIFIED.);
#5656=B_SPLINE_CURVE_WITH_KNOTS('',3,(#37446,#37447,#37448,#37449,#37450,
#37451,#37452,#37453,#37454),.UNSPECIFIED.,.F.,.F.,(4,1,1,1,1,1,4),(103.672557568463,
103.716185746199,104.708605586413,105.701025426626,106.69344526684,107.685865107053,
108.646179734666),.UNSPECIFIED.);
#5657=B_SPLINE_CURVE_WITH_KNOTS('',3,(#37459,#37460,#37461,#37462,#37463,
#37464,#37465,#37466,#37467,#37468),.UNSPECIFIED.,.F.,.F.,(4,1,1,1,1,1,
1,4),(97.3893722612835,98.1995149608939,99.1919348011075,100.184354641321,
101.176774481535,102.169194321748,103.161614161962,103.672557568463),
 .UNSPECIFIED.);
#5658=B_SPLINE_CURVE_WITH_KNOTS('',3,(#37469,#37470,#37471,#37472,#37473,
#37474,#37475,#37476,#37477,#37478),.UNSPECIFIED.,.F.,.F.,(4,1,1,1,1,1,
1,4),(97.3893722612835,97.7616667049171,98.7540865451307,99.7465063853443,
100.738926225558,101.731346065772,102.723765905985,103.672557568463),
 .UNSPECIFIED.);
#5659=B_SPLINE_CURVE_WITH_KNOTS('',3,(#37483,#37484,#37485,#37486,#37487,
#37488,#37489,#37490,#37491,#37492,#37493),.UNSPECIFIED.,.F.,.F.,(4,1,1,
1,1,1,1,1,4),(91.106186954104,91.2525760793984,92.2449959196121,93.2374157598257,
94.2298356000393,95.222255440253,96.2146752804666,97.2070951206802,97.3893722612835),
 .UNSPECIFIED.);
#5660=B_SPLINE_CURVE_WITH_KNOTS('',3,(#37494,#37495,#37496,#37497,#37498,
#37499,#37500,#37501,#37502,#37503),.UNSPECIFIED.,.F.,.F.,(4,1,1,1,1,1,
1,4),(91.106186954104,91.8071476636353,92.7995675038489,93.7919873440625,
94.7844071842762,95.7768270244898,96.7692468647034,97.3893722612835),
 .UNSPECIFIED.);
#5661=B_SPLINE_CURVE_WITH_KNOTS('',3,(#37508,#37509,#37510,#37511,#37512,
#37513,#37514,#37515,#37516,#37517),.UNSPECIFIED.,.F.,.F.,(4,1,1,1,1,1,
1,4),(84.8230016469244,85.2980570381166,86.2904768783302,87.2828967185439,
88.2753165587575,89.2677363989711,90.2601562391848,91.106186954104),
 .UNSPECIFIED.);
#5662=B_SPLINE_CURVE_WITH_KNOTS('',3,(#37518,#37519,#37520,#37521,#37522,
#37523,#37524,#37525,#37526,#37527,#37528),.UNSPECIFIED.,.F.,.F.,(4,1,1,
1,1,1,1,1,4),(84.8230016469244,84.8602087821398,85.8526286223535,86.8450484625671,
87.8374683027807,88.8298881429944,89.822307983208,90.8147278234216,91.106186954104),
 .UNSPECIFIED.);
#5663=B_SPLINE_CURVE_WITH_KNOTS('',3,(#37533,#37534,#37535,#37536,#37537,
#37538,#37539,#37540,#37541,#37542),.UNSPECIFIED.,.F.,.F.,(4,1,1,1,1,1,
1,4),(78.5398163397448,79.3435379968348,80.3359578370484,81.3283776772621,
82.3207975174757,83.3132173576893,84.305637197903,84.8230016469244),
 .UNSPECIFIED.);
#5664=B_SPLINE_CURVE_WITH_KNOTS('',3,(#37543,#37544,#37545,#37546,#37547,
#37548,#37549,#37550,#37551,#37552),.UNSPECIFIED.,.F.,.F.,(4,1,1,1,1,1,
1,4),(78.5398163397448,78.905689740858,79.8981095810717,80.8905294212853,
81.8829492614989,82.8753691017126,83.8677889419262,84.8230016469244),
 .UNSPECIFIED.);
#5665=B_SPLINE_CURVE_WITH_KNOTS('',3,(#37557,#37558,#37559,#37560,#37561,
#37562,#37563,#37564,#37565,#37566,#37567),.UNSPECIFIED.,.F.,.F.,(4,1,1,
1,1,1,1,1,4),(72.2566310325653,72.3965991153394,73.389018955553,74.3814387957666,
75.3738586359803,76.3662784761939,77.3586983164075,78.3511181566212,78.5398163397448),
 .UNSPECIFIED.);
#5666=B_SPLINE_CURVE_WITH_KNOTS('',3,(#37568,#37569,#37570,#37571,#37572,
#37573,#37574,#37575,#37576,#37577),.UNSPECIFIED.,.F.,.F.,(4,1,1,1,1,1,
1,4),(72.2566310325651,72.9511706995762,73.9435905397899,74.9360103800035,
75.9284302202171,76.9208500604308,77.9132699006444,78.5398163397448),
 .UNSPECIFIED.);
#5667=B_SPLINE_CURVE_WITH_KNOTS('',3,(#37582,#37583,#37584,#37585,#37586,
#37587,#37588,#37589,#37590,#37591),.UNSPECIFIED.,.F.,.F.,(4,1,1,1,1,1,
1,4),(65.9734457253856,66.4420800740576,67.4344999142712,68.4269197544848,
69.4193395946985,70.4117594349121,71.4041792751257,72.2566310325653),
 .UNSPECIFIED.);
#5668=B_SPLINE_CURVE_WITH_KNOTS('',3,(#37592,#37593,#37594,#37595,#37596,
#37597,#37598,#37599,#37600,#37601,#37602),.UNSPECIFIED.,.F.,.F.,(4,1,1,
1,1,1,1,1,4),(65.9734457253856,66.0042318180808,66.9966516582944,67.9890714985081,
68.9814913387217,69.9739111789353,70.966331019149,71.9587508593626,72.2566310325651),
 .UNSPECIFIED.);
#5669=B_SPLINE_CURVE_WITH_KNOTS('',3,(#37607,#37608,#37609,#37610,#37611,
#37612,#37613,#37614,#37615,#37616),.UNSPECIFIED.,.F.,.F.,(4,1,1,1,1,1,
1,4),(59.690260418206,60.4875610327758,61.4799808729894,62.472400713203,
63.4648205534167,64.4572403936303,65.4496602338439,65.9734457253856),
 .UNSPECIFIED.);
#5670=B_SPLINE_CURVE_WITH_KNOTS('',3,(#37617,#37618,#37619,#37620,#37621,
#37622,#37623,#37624,#37625,#37626),.UNSPECIFIED.,.F.,.F.,(4,1,1,1,1,1,
1,4),(59.690260418206,60.049712776799,61.0421326170126,62.0345524572262,
63.0269722974399,64.0193921376535,65.0118119778672,65.9734457253856),
 .UNSPECIFIED.);
#5671=B_SPLINE_CURVE_WITH_KNOTS('',3,(#37631,#37632,#37633,#37634,#37635,
#37636,#37637,#37638,#37639,#37640,#37641),.UNSPECIFIED.,.F.,.F.,(4,1,1,
1,1,1,1,1,4),(53.4070751110265,53.5406221512803,54.533041991494,55.5254618317076,
56.5178816719212,57.5103015121349,58.5027213523485,59.4951411925621,59.690260418206),
 .UNSPECIFIED.);
#5672=B_SPLINE_CURVE_WITH_KNOTS('',3,(#37642,#37643,#37644,#37645,#37646,
#37647,#37648,#37649,#37650,#37651),.UNSPECIFIED.,.F.,.F.,(4,1,1,1,1,1,
1,4),(53.4070751110265,54.0951937355172,55.0876135757308,56.0800334159444,
57.0724532561581,58.0648730963717,59.0572929365853,59.690260418206),
 .UNSPECIFIED.);
#5673=B_SPLINE_CURVE_WITH_KNOTS('',3,(#37656,#37657,#37658,#37659,#37660,
#37661,#37662,#37663,#37664,#37665),.UNSPECIFIED.,.F.,.F.,(4,1,1,1,1,1,
1,4),(47.1238898038468,47.5861031099985,48.5785229502122,49.5709427904258,
50.5633626306394,51.5557824708531,52.5482023110667,53.4070751110265),
 .UNSPECIFIED.);
#5674=B_SPLINE_CURVE_WITH_KNOTS('',3,(#37666,#37667,#37668,#37669,#37670,
#37671,#37672,#37673,#37674,#37675,#37676),.UNSPECIFIED.,.F.,.F.,(4,1,1,
1,1,1,1,1,4),(47.1238898038468,47.1482548540217,48.1406746942354,49.133094534449,
50.1255143746626,51.1179342148763,52.1103540550899,53.1027738953035,53.4070751110265),
 .UNSPECIFIED.);
#5675=B_SPLINE_CURVE_WITH_KNOTS('',3,(#37681,#37682,#37683,#37684,#37685,
#37686,#37687,#37688,#37689,#37690),.UNSPECIFIED.,.F.,.F.,(4,1,1,1,1,1,
1,4),(40.8407044966672,41.6315840687167,42.6240039089303,43.616423749144,
44.6088435893576,45.6012634295713,46.5936832697849,47.1238898038468),
 .UNSPECIFIED.);
#5676=B_SPLINE_CURVE_WITH_KNOTS('',3,(#37691,#37692,#37693,#37694,#37695,
#37696,#37697,#37698,#37699,#37700),.UNSPECIFIED.,.F.,.F.,(4,1,1,1,1,1,
1,4),(40.8407044966672,41.1937358127399,42.1861556529536,43.1785754931672,
44.1709953333808,45.1634151735945,46.1558350138081,47.1238898038468),
 .UNSPECIFIED.);
#5677=B_SPLINE_CURVE_WITH_KNOTS('',3,(#37705,#37706,#37707,#37708,#37709,
#37710,#37711,#37712,#37713,#37714,#37715),.UNSPECIFIED.,.F.,.F.,(4,1,1,
1,1,1,1,1,4),(34.5575191894877,34.6846451872213,35.6770650274349,36.6694848676485,
37.6619047078622,38.6543245480758,39.6467443882894,40.6391642285031,40.8407044966672),
 .UNSPECIFIED.);
#5678=B_SPLINE_CURVE_WITH_KNOTS('',3,(#37716,#37717,#37718,#37719,#37720,
#37721,#37722,#37723,#37724,#37725),.UNSPECIFIED.,.F.,.F.,(4,1,1,1,1,1,
1,4),(34.5575191894877,35.2392167714581,36.2316366116718,37.2240564518854,
38.216476292099,39.2088961323127,40.2013159725263,40.8407044966672),
 .UNSPECIFIED.);
#5679=B_SPLINE_CURVE_WITH_KNOTS('',3,(#37730,#37731,#37732,#37733,#37734,
#37735,#37736,#37737,#37738,#37739),.UNSPECIFIED.,.F.,.F.,(4,1,1,1,1,1,
1,4),(28.2743338823081,28.7301261459395,29.7225459861531,30.7149658263667,
31.7073856665804,32.699805506794,33.6922253470076,34.5575191894877),
 .UNSPECIFIED.);
#5680=B_SPLINE_CURVE_WITH_KNOTS('',3,(#37740,#37741,#37742,#37743,#37744,
#37745,#37746,#37747,#37748,#37749,#37750),.UNSPECIFIED.,.F.,.F.,(4,1,1,
1,1,1,1,1,4),(28.2743338823081,28.2922778899627,29.2846977301763,30.27711757039,
31.2695374106036,32.2619572508172,33.2543770910309,34.2467969312445,34.5575191894877),
 .UNSPECIFIED.);
#5681=B_SPLINE_CURVE_WITH_KNOTS('',3,(#37755,#37756,#37757,#37758,#37759,
#37760,#37761,#37762,#37763,#37764),.UNSPECIFIED.,.F.,.F.,(4,1,1,1,1,1,
1,4),(21.9911485751285,22.7756071046577,23.7680269448713,24.7604467850849,
25.7528666252986,26.7452864655122,27.7377063057258,28.2743338823081),
 .UNSPECIFIED.);
#5682=B_SPLINE_CURVE_WITH_KNOTS('',3,(#37765,#37766,#37767,#37768,#37769,
#37770,#37771,#37772,#37773,#37774),.UNSPECIFIED.,.F.,.F.,(4,1,1,1,1,1,
1,4),(21.9911485751284,22.3377588486809,23.3301786888945,24.3225985291082,
25.3150183693218,26.3074382095354,27.2998580497491,28.2743338823081),
 .UNSPECIFIED.);
#5683=B_SPLINE_CURVE_WITH_KNOTS('',3,(#37780,#37781,#37782,#37783,#37784),
 .UNSPECIFIED.,.F.,.F.,(4,1,4),(14.3984001269718,15.3908199671854,15.7079632679489),
 .UNSPECIFIED.);
#5684=B_SPLINE_CURVE_WITH_KNOTS('',3,(#37787,#37788,#37789,#37790,#37791),
 .UNSPECIFIED.,.F.,.F.,(4,1,4),(13.8759337553363,14.8362483829486,15.7079632679488),
 .UNSPECIFIED.);
#5685=B_SPLINE_CURVE_WITH_KNOTS('',3,(#37797,#37798,#37799,#37800),
 .UNSPECIFIED.,.F.,.F.,(4,4),(95.5573427486707,96.2647245007224),
 .UNSPECIFIED.);
#5686=B_SPLINE_CURVE_WITH_KNOTS('',3,(#37808,#37809,#37810,#37811,#37812,
#37813,#37814,#37815,#37816,#37817),.UNSPECIFIED.,.F.,.F.,(4,3,3,4),(-94.2477796076938,
-93.2874649800815,-92.2950451398679,-91.8135687061554),.UNSPECIFIED.);
#5687=B_SPLINE_CURVE_WITH_KNOTS('',3,(#37822,#37823,#37824,#37825,#37826,
#37827,#37828,#37829,#37830,#37831,#37832,#37833,#37834,#37835,#37836,#37837,
#37838,#37839,#37840,#37841,#37842,#37843,#37844,#37845,#37846),
 .UNSPECIFIED.,.F.,.F.,(4,3,3,3,3,3,3,3,4),(89.2741574414911,89.317785619227,
90.3102054594406,91.3026252996542,92.2950451398679,93.2874649800815,94.2798848202951,
95.2723046605088,95.5573427486707),.UNSPECIFIED.);
#5688=B_SPLINE_CURVE_WITH_KNOTS('',3,(#37847,#37848,#37849,#37850,#37851,
#37852,#37853,#37854,#37855,#37856,#37857,#37858,#37859,#37860,#37861,#37862,
#37863,#37864,#37865,#37866,#37867,#37868),.UNSPECIFIED.,.F.,.F.,(4,3,3,
3,3,3,3,4),(-91.8135687061554,-91.3026252996542,-90.3102054594406,-89.317785619227,
-88.3253657790133,-87.3329459387997,-86.3405260985861,-85.5303833989757),
 .UNSPECIFIED.);
#5689=B_SPLINE_CURVE_WITH_KNOTS('',3,(#37873,#37874,#37875,#37876,#37877,
#37878,#37879,#37880,#37881,#37882,#37883,#37884,#37885,#37886,#37887,#37888,
#37889,#37890,#37891,#37892,#37893,#37894),.UNSPECIFIED.,.F.,.F.,(4,3,3,
3,3,3,3,4),(82.9909721343116,83.3632665779452,84.3556864181588,85.3481062583724,
86.3405260985861,87.3329459387997,88.3253657790133,89.2741574414911),
 .UNSPECIFIED.);
#5690=B_SPLINE_CURVE_WITH_KNOTS('',3,(#37895,#37896,#37897,#37898,#37899,
#37900,#37901,#37902,#37903,#37904,#37905,#37906,#37907,#37908,#37909,#37910,
#37911,#37912,#37913,#37914,#37915,#37916,#37917,#37918,#37919),
 .UNSPECIFIED.,.F.,.F.,(4,3,3,3,3,3,3,3,4),(-85.5303833989757,-85.3481062583724,
-84.3556864181588,-83.3632665779452,-82.3708467377315,-81.3784268975179,
-80.3860070573043,-79.3935872170906,-79.2471980917961),.UNSPECIFIED.);
#5691=B_SPLINE_CURVE_WITH_KNOTS('',3,(#37924,#37925,#37926,#37927,#37928,
#37929,#37930,#37931,#37932,#37933,#37934,#37935,#37936,#37937,#37938,#37939,
#37940,#37941,#37942,#37943,#37944,#37945),.UNSPECIFIED.,.F.,.F.,(4,3,3,
3,3,3,3,4),(76.7077868271319,77.4087475366634,78.401167376877,79.3935872170906,
80.3860070573043,81.3784268975179,82.3708467377315,82.9909721343116),
 .UNSPECIFIED.);
#5692=B_SPLINE_CURVE_WITH_KNOTS('',3,(#37946,#37947,#37948,#37949,#37950,
#37951,#37952,#37953,#37954,#37955,#37956,#37957,#37958,#37959,#37960,#37961,
#37962,#37963,#37964,#37965,#37966,#37967),.UNSPECIFIED.,.F.,.F.,(4,3,3,
3,3,3,3,4),(-79.2471980917961,-78.401167376877,-77.4087475366633,-76.4163276964497,
-75.4239078562361,-74.4314880160224,-73.4390681758088,-72.9640127846165),
 .UNSPECIFIED.);
#5693=B_SPLINE_CURVE_WITH_KNOTS('',3,(#37972,#37973,#37974,#37975,#37976,
#37977,#37978,#37979,#37980,#37981,#37982,#37983,#37984,#37985,#37986,#37987,
#37988,#37989,#37990,#37991,#37992,#37993,#37994,#37995,#37996),
 .UNSPECIFIED.,.F.,.F.,(4,3,3,3,3,3,3,3,4),(70.4246015199523,70.4618086551679,
71.4542284953816,72.4466483355952,73.4390681758088,74.4314880160225,75.4239078562361,
76.4163276964497,76.7077868271319),.UNSPECIFIED.);
#5694=B_SPLINE_CURVE_WITH_KNOTS('',3,(#37997,#37998,#37999,#38000,#38001,
#38002,#38003,#38004,#38005,#38006,#38007,#38008,#38009,#38010,#38011,#38012,
#38013,#38014,#38015,#38016,#38017,#38018),.UNSPECIFIED.,.F.,.F.,(4,3,3,
3,3,3,3,4),(-72.9640127846165,-72.4466483355952,-71.4542284953815,-70.4618086551679,
-69.4693888149543,-68.4769689747406,-67.484549134527,-66.680827477437),
 .UNSPECIFIED.);
#5695=B_SPLINE_CURVE_WITH_KNOTS('',3,(#38023,#38024,#38025,#38026,#38027,
#38028,#38029,#38030,#38031,#38032,#38033,#38034,#38035,#38036,#38037,#38038,
#38039,#38040,#38041,#38042,#38043,#38044),.UNSPECIFIED.,.F.,.F.,(4,3,3,
3,3,3,3,4),(64.1414162127728,64.5072896138861,65.4997094540998,66.4921292943134,
67.484549134527,68.4769689747407,69.4693888149543,70.4246015199523),
 .UNSPECIFIED.);
#5696=B_SPLINE_CURVE_WITH_KNOTS('',3,(#38045,#38046,#38047,#38048,#38049,
#38050,#38051,#38052,#38053,#38054,#38055,#38056,#38057,#38058,#38059,#38060,
#38061,#38062,#38063,#38064,#38065,#38066,#38067,#38068,#38069),
 .UNSPECIFIED.,.F.,.F.,(4,3,3,3,3,3,3,3,4),(-66.680827477437,-66.4921292943134,
-65.4997094540998,-64.5072896138861,-63.5148697736725,-62.5224499334589,
-61.5300300932452,-60.5376102530316,-60.3976421702573),.UNSPECIFIED.);
#5697=B_SPLINE_CURVE_WITH_KNOTS('',3,(#38074,#38075,#38076,#38077,#38078,
#38079,#38080,#38081,#38082,#38083,#38084,#38085,#38086,#38087,#38088,#38089,
#38090,#38091,#38092,#38093,#38094,#38095),.UNSPECIFIED.,.F.,.F.,(4,3,3,
3,3,3,3,4),(57.8582309055932,58.5527705726043,59.545190412818,60.5376102530316,
61.5300300932452,62.5224499334589,63.5148697736725,64.1414162127728),
 .UNSPECIFIED.);
#5698=B_SPLINE_CURVE_WITH_KNOTS('',3,(#38096,#38097,#38098,#38099,#38100,
#38101,#38102,#38103,#38104,#38105,#38106,#38107,#38108,#38109,#38110,#38111,
#38112,#38113,#38114,#38115,#38116,#38117),.UNSPECIFIED.,.F.,.F.,(4,3,3,
3,3,3,3,4),(-60.3976421702573,-59.545190412818,-58.5527705726043,-57.5603507323907,
-56.5679308921771,-55.5755110519634,-54.5830912117498,-54.1144568630777),
 .UNSPECIFIED.);
#5699=B_SPLINE_CURVE_WITH_KNOTS('',3,(#38122,#38123,#38124,#38125,#38126,
#38127,#38128,#38129,#38130,#38131,#38132,#38133,#38134,#38135,#38136,#38137,
#38138,#38139,#38140,#38141,#38142,#38143,#38144,#38145,#38146),
 .UNSPECIFIED.,.F.,.F.,(4,3,3,3,3,3,3,3,4),(51.5750455984135,51.6058316911089,
52.5982515313225,53.5906713715362,54.5830912117498,55.5755110519634,56.5679308921771,
57.5603507323907,57.8582309055932),.UNSPECIFIED.);
#5700=B_SPLINE_CURVE_WITH_KNOTS('',3,(#38147,#38148,#38149,#38150,#38151,
#38152,#38153,#38154,#38155,#38156,#38157,#38158,#38159,#38160,#38161,#38162,
#38163,#38164,#38165,#38166,#38167,#38168),.UNSPECIFIED.,.F.,.F.,(4,3,3,
3,3,3,3,4),(-54.1144568630777,-53.5906713715362,-52.5982515313225,-51.6058316911089,
-50.6134118508953,-49.6209920106816,-48.628572170468,-47.8312715558982),
 .UNSPECIFIED.);
#5701=B_SPLINE_CURVE_WITH_KNOTS('',3,(#38173,#38174,#38175,#38176,#38177,
#38178,#38179,#38180,#38181,#38182,#38183,#38184,#38185,#38186,#38187,#38188,
#38189,#38190,#38191,#38192,#38193,#38194),.UNSPECIFIED.,.F.,.F.,(4,3,3,
3,3,3,3,4),(45.291860291234,45.6513126498271,46.6437324900407,47.6361523302544,
48.628572170468,49.6209920106816,50.6134118508953,51.5750455984135),
 .UNSPECIFIED.);
#5702=B_SPLINE_CURVE_WITH_KNOTS('',3,(#38195,#38196,#38197,#38198,#38199,
#38200,#38201,#38202,#38203,#38204,#38205,#38206,#38207,#38208,#38209,#38210,
#38211,#38212,#38213,#38214,#38215,#38216,#38217,#38218,#38219),
 .UNSPECIFIED.,.F.,.F.,(4,3,3,3,3,3,3,3,4),(-47.8312715558982,-47.6361523302544,
-46.6437324900407,-45.6513126498271,-44.6588928096135,-43.6664729693998,
-42.6740531291862,-41.6816332889726,-41.5480862487186),.UNSPECIFIED.);
#5703=B_SPLINE_CURVE_WITH_KNOTS('',3,(#38224,#38225,#38226,#38227,#38228,
#38229,#38230,#38231,#38232,#38233,#38234,#38235,#38236,#38237,#38238,#38239,
#38240,#38241,#38242,#38243,#38244,#38245),.UNSPECIFIED.,.F.,.F.,(4,3,3,
3,3,3,3,4),(39.0086749840544,39.6967936085453,40.6892134487589,41.6816332889726,
42.6740531291862,43.6664729693998,44.6588928096135,45.291860291234),
 .UNSPECIFIED.);
#5704=B_SPLINE_CURVE_WITH_KNOTS('',3,(#38246,#38247,#38248,#38249,#38250,
#38251,#38252,#38253,#38254,#38255,#38256,#38257,#38258,#38259,#38260,#38261,
#38262,#38263,#38264,#38265,#38266,#38267),.UNSPECIFIED.,.F.,.F.,(4,3,3,
3,3,3,3,4),(-41.5480862487186,-40.6892134487589,-39.6967936085453,-38.7043737683317,
-37.711953928118,-36.7195340879044,-35.7271142476908,-35.2649009415389),
 .UNSPECIFIED.);
#5705=B_SPLINE_CURVE_WITH_KNOTS('',3,(#38272,#38273,#38274,#38275,#38276,
#38277,#38278,#38279,#38280,#38281,#38282,#38283,#38284,#38285,#38286,#38287,
#38288,#38289,#38290,#38291,#38292,#38293,#38294,#38295,#38296),
 .UNSPECIFIED.,.F.,.F.,(4,3,3,3,3,3,3,3,4),(32.7254896768748,32.7498547270499,
33.7422745672635,34.7346944074771,35.7271142476908,36.7195340879044,37.711953928118,
38.7043737683317,39.0086749840544),.UNSPECIFIED.);
#5706=B_SPLINE_CURVE_WITH_KNOTS('',3,(#38297,#38298,#38299,#38300,#38301,
#38302,#38303,#38304,#38305,#38306,#38307,#38308,#38309,#38310,#38311,#38312,
#38313,#38314,#38315,#38316,#38317,#38318),.UNSPECIFIED.,.F.,.F.,(4,3,3,
3,3,3,3,4),(-35.2649009415389,-34.7346944074771,-33.7422745672635,-32.7498547270499,
-31.7574348868362,-30.7650150466226,-29.772595206409,-28.9817156343594),
 .UNSPECIFIED.);
#5707=B_SPLINE_CURVE_WITH_KNOTS('',3,(#38323,#38324,#38325,#38326,#38327,
#38328,#38329,#38330,#38331,#38332,#38333,#38334,#38335,#38336,#38337,#38338,
#38339,#38340,#38341,#38342,#38343,#38344),.UNSPECIFIED.,.F.,.F.,(4,3,3,
3,3,3,3,4),(26.4423043696952,26.7953356857681,27.7877555259817,28.7801753661954,
29.772595206409,30.7650150466226,31.7574348868363,32.7254896768748),
 .UNSPECIFIED.);
#5708=B_SPLINE_CURVE_WITH_KNOTS('',3,(#38345,#38346,#38347,#38348,#38349,
#38350,#38351,#38352,#38353,#38354,#38355,#38356,#38357,#38358,#38359,#38360,
#38361,#38362,#38363,#38364,#38365,#38366,#38367,#38368,#38369),
 .UNSPECIFIED.,.F.,.F.,(4,3,3,3,3,3,3,3,4),(-28.9817156343594,-28.7801753661953,
-27.7877555259817,-26.7953356857681,-25.8029158455544,-24.8104960053408,
-23.8180761651272,-22.8256563249135,-22.6985303271798),.UNSPECIFIED.);
#5709=B_SPLINE_CURVE_WITH_KNOTS('',3,(#38374,#38375,#38376,#38377,#38378,
#38379,#38380,#38381,#38382,#38383,#38384,#38385,#38386,#38387,#38388,#38389,
#38390,#38391,#38392,#38393,#38394,#38395),.UNSPECIFIED.,.F.,.F.,(4,3,3,
3,3,3,3,4),(20.1591190625156,20.8408166444863,21.8332364846999,22.8256563249136,
23.8180761651272,24.8104960053408,25.8029158455545,26.4423043696952),
 .UNSPECIFIED.);
#5710=B_SPLINE_CURVE_WITH_KNOTS('',3,(#38396,#38397,#38398,#38399,#38400,
#38401,#38402,#38403,#38404,#38405,#38406,#38407,#38408,#38409,#38410,#38411,
#38412,#38413,#38414,#38415,#38416,#38417),.UNSPECIFIED.,.F.,.F.,(4,3,3,
3,3,3,3,4),(-22.6985303271798,-21.8332364846999,-20.8408166444863,-19.8483968042727,
-18.855976964059,-17.8635571238454,-16.8711372836318,-16.4153450200002),
 .UNSPECIFIED.);
#5711=B_SPLINE_CURVE_WITH_KNOTS('',3,(#38422,#38423,#38424,#38425,#38426,
#38427,#38428,#38429,#38430,#38431,#38432,#38433,#38434,#38435,#38436,#38437,
#38438,#38439,#38440,#38441,#38442,#38443,#38444,#38445,#38446),
 .UNSPECIFIED.,.F.,.F.,(4,3,3,3,3,3,3,3,4),(13.875933755336,13.8938777629909,
14.8862976032045,15.8787174434181,16.8711372836318,17.8635571238454,18.855976964059,
19.8483968042727,20.1591190625156),.UNSPECIFIED.);
#5712=B_SPLINE_CURVE_WITH_KNOTS('',3,(#38447,#38448,#38449,#38450,#38451,
#38452,#38453,#38454,#38455,#38456,#38457,#38458,#38459,#38460,#38461,#38462,
#38463,#38464,#38465,#38466,#38467,#38468),.UNSPECIFIED.,.F.,.F.,(4,3,3,
3,3,3,3,4),(-16.4153450200002,-15.8787174434181,-14.8862976032045,-13.8938777629909,
-12.9014579227772,-11.9090380825636,-10.91661824235,-10.1321597128207),
 .UNSPECIFIED.);
#5713=B_SPLINE_CURVE_WITH_KNOTS('',3,(#38474,#38475,#38476,#38477,#38478,
#38479,#38480,#38481,#38482,#38483,#38484,#38485,#38486),.UNSPECIFIED.,
 .F.,.F.,(4,3,3,3,4),(-3.848974405641,-2.9772595206409,-1.98483968042726,
-0.992419840213632,0.),.UNSPECIFIED.);
#5714=B_SPLINE_CURVE_WITH_KNOTS('',3,(#38489,#38490,#38491,#38492,#38493,
#38494,#38495,#38496,#38497,#38498,#38499,#38500,#38501,#38502,#38503,#38504,
#38505,#38506,#38507),.UNSPECIFIED.,.F.,.F.,(4,3,3,3,3,3,4),(2.01694489302852,
2.9772595206409,3.96967936085453,4.96209920106817,5.9545190412818,6.94693888149543,
7.59274844815647),.UNSPECIFIED.);
#5715=B_SPLINE_CURVE_WITH_KNOTS('',3,(#38513,#38514,#38515,#38516,#38517,
#38518,#38519,#38520),.UNSPECIFIED.,.F.,.F.,(4,1,1,1,1,4),(103.672557568463,
104.154034002176,105.146453842389,106.138873682603,107.131293522817,108.12371336303),
 .UNSPECIFIED.);
#5716=B_SPLINE_CURVE_WITH_KNOTS('',3,(#38523,#38524,#38525,#38526,#38527,
#38528,#38529,#38530,#38531),.UNSPECIFIED.,.F.,.F.,(4,1,1,1,1,1,4),(103.672557568463,
103.716185746199,104.708605586413,105.701025426626,106.69344526684,107.685865107053,
108.646179734666),.UNSPECIFIED.);
#5717=B_SPLINE_CURVE_WITH_KNOTS('',3,(#38536,#38537,#38538,#38539,#38540,
#38541,#38542,#38543,#38544,#38545),.UNSPECIFIED.,.F.,.F.,(4,1,1,1,1,1,
1,4),(97.3893722612835,98.1995149608939,99.1919348011075,100.184354641321,
101.176774481535,102.169194321748,103.161614161962,103.672557568463),
 .UNSPECIFIED.);
#5718=B_SPLINE_CURVE_WITH_KNOTS('',3,(#38546,#38547,#38548,#38549,#38550,
#38551,#38552,#38553,#38554,#38555),.UNSPECIFIED.,.F.,.F.,(4,1,1,1,1,1,
1,4),(97.3893722612835,97.7616667049171,98.7540865451307,99.7465063853444,
100.738926225558,101.731346065772,102.723765905985,103.672557568463),
 .UNSPECIFIED.);
#5719=B_SPLINE_CURVE_WITH_KNOTS('',3,(#38560,#38561,#38562,#38563,#38564,
#38565,#38566,#38567,#38568,#38569,#38570),.UNSPECIFIED.,.F.,.F.,(4,1,1,
1,1,1,1,1,4),(91.106186954104,91.2525760793984,92.2449959196121,93.2374157598257,
94.2298356000393,95.222255440253,96.2146752804666,97.2070951206802,97.3893722612835),
 .UNSPECIFIED.);
#5720=B_SPLINE_CURVE_WITH_KNOTS('',3,(#38571,#38572,#38573,#38574,#38575,
#38576,#38577,#38578,#38579,#38580),.UNSPECIFIED.,.F.,.F.,(4,1,1,1,1,1,
1,4),(91.106186954104,91.8071476636353,92.7995675038489,93.7919873440626,
94.7844071842762,95.7768270244898,96.7692468647035,97.3893722612835),
 .UNSPECIFIED.);
#5721=B_SPLINE_CURVE_WITH_KNOTS('',3,(#38585,#38586,#38587,#38588,#38589,
#38590,#38591,#38592,#38593,#38594),.UNSPECIFIED.,.F.,.F.,(4,1,1,1,1,1,
1,4),(84.8230016469244,85.2980570381166,86.2904768783303,87.2828967185439,
88.2753165587575,89.2677363989712,90.2601562391848,91.106186954104),
 .UNSPECIFIED.);
#5722=B_SPLINE_CURVE_WITH_KNOTS('',3,(#38595,#38596,#38597,#38598,#38599,
#38600,#38601,#38602,#38603,#38604,#38605),.UNSPECIFIED.,.F.,.F.,(4,1,1,
1,1,1,1,1,4),(84.8230016469244,84.8602087821399,85.8526286223535,86.8450484625671,
87.8374683027808,88.8298881429944,89.822307983208,90.8147278234217,91.106186954104),
 .UNSPECIFIED.);
#5723=B_SPLINE_CURVE_WITH_KNOTS('',3,(#38610,#38611,#38612,#38613,#38614,
#38615,#38616,#38617,#38618,#38619),.UNSPECIFIED.,.F.,.F.,(4,1,1,1,1,1,
1,4),(78.5398163397448,79.3435379968348,80.3359578370485,81.3283776772621,
82.3207975174757,83.3132173576894,84.305637197903,84.8230016469244),
 .UNSPECIFIED.);
#5724=B_SPLINE_CURVE_WITH_KNOTS('',3,(#38620,#38621,#38622,#38623,#38624,
#38625,#38626,#38627,#38628,#38629),.UNSPECIFIED.,.F.,.F.,(4,1,1,1,1,1,
1,4),(78.5398163397448,78.9056897408581,79.8981095810717,80.8905294212853,
81.882949261499,82.8753691017126,83.8677889419262,84.8230016469244),
 .UNSPECIFIED.);
#5725=B_SPLINE_CURVE_WITH_KNOTS('',3,(#38634,#38635,#38636,#38637,#38638,
#38639,#38640,#38641,#38642,#38643,#38644),.UNSPECIFIED.,.F.,.F.,(4,1,1,
1,1,1,1,1,4),(72.2566310325653,72.3965991153394,73.389018955553,74.3814387957667,
75.3738586359803,76.3662784761939,77.3586983164076,78.3511181566212,78.5398163397448),
 .UNSPECIFIED.);
#5726=B_SPLINE_CURVE_WITH_KNOTS('',3,(#38645,#38646,#38647,#38648,#38649,
#38650,#38651,#38652,#38653,#38654),.UNSPECIFIED.,.F.,.F.,(4,1,1,1,1,1,
1,4),(72.2566310325651,72.9511706995763,73.9435905397899,74.9360103800035,
75.9284302202172,76.9208500604308,77.9132699006444,78.5398163397448),
 .UNSPECIFIED.);
#5727=B_SPLINE_CURVE_WITH_KNOTS('',3,(#38659,#38660,#38661,#38662,#38663,
#38664,#38665,#38666,#38667,#38668),.UNSPECIFIED.,.F.,.F.,(4,1,1,1,1,1,
1,4),(65.9734457253856,66.4420800740576,67.4344999142712,68.4269197544849,
69.4193395946985,70.4117594349121,71.4041792751258,72.2566310325653),
 .UNSPECIFIED.);
#5728=B_SPLINE_CURVE_WITH_KNOTS('',3,(#38669,#38670,#38671,#38672,#38673,
#38674,#38675,#38676,#38677,#38678,#38679),.UNSPECIFIED.,.F.,.F.,(4,1,1,
1,1,1,1,1,4),(65.9734457253856,66.0042318180808,66.9966516582945,67.9890714985081,
68.9814913387217,69.9739111789354,70.966331019149,71.9587508593626,72.2566310325651),
 .UNSPECIFIED.);
#5729=B_SPLINE_CURVE_WITH_KNOTS('',3,(#38684,#38685,#38686,#38687,#38688,
#38689,#38690,#38691,#38692,#38693),.UNSPECIFIED.,.F.,.F.,(4,1,1,1,1,1,
1,4),(59.690260418206,60.4875610327758,61.4799808729895,62.4724007132031,
63.4648205534167,64.4572403936303,65.449660233844,65.9734457253856),
 .UNSPECIFIED.);
#5730=B_SPLINE_CURVE_WITH_KNOTS('',3,(#38694,#38695,#38696,#38697,#38698,
#38699,#38700,#38701,#38702,#38703),.UNSPECIFIED.,.F.,.F.,(4,1,1,1,1,1,
1,4),(59.690260418206,60.049712776799,61.0421326170127,62.0345524572263,
63.0269722974399,64.0193921376536,65.0118119778672,65.9734457253856),
 .UNSPECIFIED.);
#5731=B_SPLINE_CURVE_WITH_KNOTS('',3,(#38708,#38709,#38710,#38711,#38712,
#38713,#38714,#38715,#38716,#38717,#38718),.UNSPECIFIED.,.F.,.F.,(4,1,1,
1,1,1,1,1,4),(53.4070751110265,53.5406221512804,54.533041991494,55.5254618317077,
56.5178816719213,57.5103015121349,58.5027213523486,59.4951411925622,59.690260418206),
 .UNSPECIFIED.);
#5732=B_SPLINE_CURVE_WITH_KNOTS('',3,(#38719,#38720,#38721,#38722,#38723,
#38724,#38725,#38726,#38727,#38728),.UNSPECIFIED.,.F.,.F.,(4,1,1,1,1,1,
1,4),(53.4070751110265,54.0951937355172,55.0876135757309,56.0800334159445,
57.0724532561581,58.0648730963718,59.0572929365854,59.690260418206),
 .UNSPECIFIED.);
#5733=B_SPLINE_CURVE_WITH_KNOTS('',3,(#38733,#38734,#38735,#38736,#38737,
#38738,#38739,#38740,#38741,#38742),.UNSPECIFIED.,.F.,.F.,(4,1,1,1,1,1,
1,4),(47.1238898038468,47.5861031099986,48.5785229502122,49.5709427904259,
50.5633626306395,51.5557824708531,52.5482023110668,53.4070751110265),
 .UNSPECIFIED.);
#5734=B_SPLINE_CURVE_WITH_KNOTS('',3,(#38743,#38744,#38745,#38746,#38747,
#38748,#38749,#38750,#38751,#38752,#38753),.UNSPECIFIED.,.F.,.F.,(4,1,1,
1,1,1,1,1,4),(47.1238898038468,47.1482548540218,48.1406746942354,49.1330945344491,
50.1255143746627,51.1179342148763,52.11035405509,53.1027738953036,53.4070751110265),
 .UNSPECIFIED.);
#5735=B_SPLINE_CURVE_WITH_KNOTS('',3,(#38758,#38759,#38760,#38761,#38762,
#38763,#38764,#38765,#38766,#38767),.UNSPECIFIED.,.F.,.F.,(4,1,1,1,1,1,
1,4),(40.8407044966672,41.6315840687168,42.6240039089304,43.6164237491441,
44.6088435893577,45.6012634295713,46.593683269785,47.1238898038468),
 .UNSPECIFIED.);
#5736=B_SPLINE_CURVE_WITH_KNOTS('',3,(#38768,#38769,#38770,#38771,#38772,
#38773,#38774,#38775,#38776,#38777),.UNSPECIFIED.,.F.,.F.,(4,1,1,1,1,1,
1,4),(40.8407044966672,41.19373581274,42.1861556529536,43.1785754931673,
44.1709953333809,45.1634151735945,46.1558350138082,47.1238898038468),
 .UNSPECIFIED.);
#5737=B_SPLINE_CURVE_WITH_KNOTS('',3,(#38782,#38783,#38784,#38785,#38786,
#38787,#38788,#38789,#38790,#38791,#38792),.UNSPECIFIED.,.F.,.F.,(4,1,1,
1,1,1,1,1,4),(34.5575191894877,34.6846451872214,35.677065027435,36.6694848676486,
37.6619047078623,38.6543245480759,39.6467443882895,40.6391642285032,40.8407044966672),
 .UNSPECIFIED.);
#5738=B_SPLINE_CURVE_WITH_KNOTS('',3,(#38793,#38794,#38795,#38796,#38797,
#38798,#38799,#38800,#38801,#38802),.UNSPECIFIED.,.F.,.F.,(4,1,1,1,1,1,
1,4),(34.5575191894877,35.2392167714582,36.2316366116718,37.2240564518855,
38.2164762920991,39.2088961323127,40.2013159725264,40.8407044966672),
 .UNSPECIFIED.);
#5739=B_SPLINE_CURVE_WITH_KNOTS('',3,(#38807,#38808,#38809,#38810,#38811,
#38812,#38813,#38814,#38815,#38816),.UNSPECIFIED.,.F.,.F.,(4,1,1,1,1,1,
1,4),(28.2743338823081,28.7301261459396,29.7225459861532,30.7149658263668,
31.7073856665805,32.6998055067941,33.6922253470077,34.5575191894877),
 .UNSPECIFIED.);
#5740=B_SPLINE_CURVE_WITH_KNOTS('',3,(#38817,#38818,#38819,#38820,#38821,
#38822,#38823,#38824,#38825,#38826,#38827),.UNSPECIFIED.,.F.,.F.,(4,1,1,
1,1,1,1,1,4),(28.2743338823081,28.2922778899628,29.2846977301764,30.2771175703901,
31.2695374106037,32.2619572508173,33.2543770910309,34.2467969312446,34.5575191894877),
 .UNSPECIFIED.);
#5741=B_SPLINE_CURVE_WITH_KNOTS('',3,(#38832,#38833,#38834,#38835,#38836,
#38837,#38838,#38839,#38840,#38841),.UNSPECIFIED.,.F.,.F.,(4,1,1,1,1,1,
1,4),(21.9911485751285,22.7756071046578,23.7680269448714,24.760446785085,
25.7528666252987,26.7452864655123,27.7377063057259,28.2743338823081),
 .UNSPECIFIED.);
#5742=B_SPLINE_CURVE_WITH_KNOTS('',3,(#38842,#38843,#38844,#38845,#38846,
#38847,#38848,#38849,#38850,#38851),.UNSPECIFIED.,.F.,.F.,(4,1,1,1,1,1,
1,4),(21.9911485751284,22.337758848681,23.3301786888946,24.3225985291083,
25.3150183693219,26.3074382095355,27.2998580497492,28.2743338823081),
 .UNSPECIFIED.);
#5743=B_SPLINE_CURVE_WITH_KNOTS('',3,(#38857,#38858,#38859,#38860,#38861),
 .UNSPECIFIED.,.F.,.F.,(4,1,4),(14.3984001269719,15.3908199671856,15.7079632679489),
 .UNSPECIFIED.);
#5744=B_SPLINE_CURVE_WITH_KNOTS('',3,(#38864,#38865,#38866,#38867,#38868),
 .UNSPECIFIED.,.F.,.F.,(4,1,4),(13.8759337553364,14.8362483829487,15.7079632679489),
 .UNSPECIFIED.);
#5745=B_SPLINE_CURVE_WITH_KNOTS('',3,(#38874,#38875,#38876,#38877),
 .UNSPECIFIED.,.F.,.F.,(4,4),(95.5573427486708,96.2647245007226),
 .UNSPECIFIED.);
#5746=B_SPLINE_CURVE_WITH_KNOTS('',3,(#38885,#38886,#38887,#38888,#38889,
#38890,#38891,#38892,#38893,#38894),.UNSPECIFIED.,.F.,.F.,(4,3,3,4),(-94.2477796076939,
-93.2874649800816,-92.295045139868,-91.8135687061555),.UNSPECIFIED.);
#5747=B_SPLINE_CURVE_WITH_KNOTS('',3,(#38899,#38900,#38901,#38902,#38903,
#38904,#38905,#38906,#38907,#38908,#38909,#38910,#38911,#38912,#38913,#38914,
#38915,#38916,#38917,#38918,#38919,#38920,#38921,#38922,#38923),
 .UNSPECIFIED.,.F.,.F.,(4,3,3,3,3,3,3,3,4),(89.2741574414912,89.3177856192271,
90.3102054594407,91.3026252996543,92.295045139868,93.2874649800816,94.2798848202952,
95.2723046605089,95.5573427486708),.UNSPECIFIED.);
#5748=B_SPLINE_CURVE_WITH_KNOTS('',3,(#38924,#38925,#38926,#38927,#38928,
#38929,#38930,#38931,#38932,#38933,#38934,#38935,#38936,#38937,#38938,#38939,
#38940,#38941,#38942,#38943,#38944,#38945),.UNSPECIFIED.,.F.,.F.,(4,3,3,
3,3,3,3,4),(-91.8135687061555,-91.3026252996543,-90.3102054594407,-89.3177856192271,
-88.3253657790134,-87.3329459387998,-86.3405260985862,-85.5303833989759),
 .UNSPECIFIED.);
#5749=B_SPLINE_CURVE_WITH_KNOTS('',3,(#38950,#38951,#38952,#38953,#38954,
#38955,#38956,#38957,#38958,#38959,#38960,#38961,#38962,#38963,#38964,#38965,
#38966,#38967,#38968,#38969,#38970,#38971),.UNSPECIFIED.,.F.,.F.,(4,3,3,
3,3,3,3,4),(82.9909721343117,83.3632665779453,84.3556864181589,85.3481062583725,
86.3405260985862,87.3329459387998,88.3253657790134,89.2741574414912),
 .UNSPECIFIED.);
#5750=B_SPLINE_CURVE_WITH_KNOTS('',3,(#38972,#38973,#38974,#38975,#38976,
#38977,#38978,#38979,#38980,#38981,#38982,#38983,#38984,#38985,#38986,#38987,
#38988,#38989,#38990,#38991,#38992,#38993,#38994,#38995,#38996),
 .UNSPECIFIED.,.F.,.F.,(4,3,3,3,3,3,3,3,4),(-85.5303833989759,-85.3481062583725,
-84.3556864181589,-83.3632665779453,-82.3708467377316,-81.378426897518,
-80.3860070573044,-79.3935872170907,-79.2471980917962),.UNSPECIFIED.);
#5751=B_SPLINE_CURVE_WITH_KNOTS('',3,(#39001,#39002,#39003,#39004,#39005,
#39006,#39007,#39008,#39009,#39010,#39011,#39012,#39013,#39014,#39015,#39016,
#39017,#39018,#39019,#39020,#39021,#39022),.UNSPECIFIED.,.F.,.F.,(4,3,3,
3,3,3,3,4),(76.707786827132,77.4087475366635,78.4011673768771,79.3935872170907,
80.3860070573044,81.378426897518,82.3708467377316,82.9909721343117),
 .UNSPECIFIED.);
#5752=B_SPLINE_CURVE_WITH_KNOTS('',3,(#39023,#39024,#39025,#39026,#39027,
#39028,#39029,#39030,#39031,#39032,#39033,#39034,#39035,#39036,#39037,#39038,
#39039,#39040,#39041,#39042,#39043,#39044),.UNSPECIFIED.,.F.,.F.,(4,3,3,
3,3,3,3,4),(-79.2471980917962,-78.4011673768771,-77.4087475366635,-76.4163276964498,
-75.4239078562362,-74.4314880160225,-73.4390681758089,-72.9640127846167),
 .UNSPECIFIED.);
#5753=B_SPLINE_CURVE_WITH_KNOTS('',3,(#39049,#39050,#39051,#39052,#39053,
#39054,#39055,#39056,#39057,#39058,#39059,#39060,#39061,#39062,#39063,#39064,
#39065,#39066,#39067,#39068,#39069,#39070,#39071,#39072,#39073),
 .UNSPECIFIED.,.F.,.F.,(4,3,3,3,3,3,3,3,4),(70.4246015199524,70.461808655168,
71.4542284953816,72.4466483355953,73.4390681758089,74.4314880160225,75.4239078562362,
76.4163276964498,76.707786827132),.UNSPECIFIED.);
#5754=B_SPLINE_CURVE_WITH_KNOTS('',3,(#39074,#39075,#39076,#39077,#39078,
#39079,#39080,#39081,#39082,#39083,#39084,#39085,#39086,#39087,#39088,#39089,
#39090,#39091,#39092,#39093,#39094,#39095),.UNSPECIFIED.,.F.,.F.,(4,3,3,
3,3,3,3,4),(-72.9640127846167,-72.4466483355953,-71.4542284953816,-70.461808655168,
-69.4693888149544,-68.4769689747407,-67.4845491345271,-66.6808274774371),
 .UNSPECIFIED.);
#5755=B_SPLINE_CURVE_WITH_KNOTS('',3,(#39100,#39101,#39102,#39103,#39104,
#39105,#39106,#39107,#39108,#39109,#39110,#39111,#39112,#39113,#39114,#39115,
#39116,#39117,#39118,#39119,#39120,#39121),.UNSPECIFIED.,.F.,.F.,(4,3,3,
3,3,3,3,4),(64.1414162127729,64.5072896138862,65.4997094540998,66.4921292943135,
67.4845491345271,68.4769689747407,69.4693888149544,70.4246015199524),
 .UNSPECIFIED.);
#5756=B_SPLINE_CURVE_WITH_KNOTS('',3,(#39122,#39123,#39124,#39125,#39126,
#39127,#39128,#39129,#39130,#39131,#39132,#39133,#39134,#39135,#39136,#39137,
#39138,#39139,#39140,#39141,#39142,#39143,#39144,#39145,#39146),
 .UNSPECIFIED.,.F.,.F.,(4,3,3,3,3,3,3,3,4),(-66.6808274774371,-66.4921292943135,
-65.4997094540998,-64.5072896138862,-63.5148697736726,-62.5224499334589,
-61.5300300932453,-60.5376102530317,-60.3976421702575),.UNSPECIFIED.);
#5757=B_SPLINE_CURVE_WITH_KNOTS('',3,(#39151,#39152,#39153,#39154,#39155,
#39156,#39157,#39158,#39159,#39160,#39161,#39162,#39163,#39164,#39165,#39166,
#39167,#39168,#39169,#39170,#39171,#39172),.UNSPECIFIED.,.F.,.F.,(4,3,3,
3,3,3,3,4),(57.8582309055933,58.5527705726044,59.545190412818,60.5376102530317,
61.5300300932453,62.5224499334589,63.5148697736726,64.1414162127729),
 .UNSPECIFIED.);
#5758=B_SPLINE_CURVE_WITH_KNOTS('',3,(#39173,#39174,#39175,#39176,#39177,
#39178,#39179,#39180,#39181,#39182,#39183,#39184,#39185,#39186,#39187,#39188,
#39189,#39190,#39191,#39192,#39193,#39194),.UNSPECIFIED.,.F.,.F.,(4,3,3,
3,3,3,3,4),(-60.3976421702575,-59.545190412818,-58.5527705726044,-57.5603507323908,
-56.5679308921771,-55.5755110519635,-54.5830912117499,-54.1144568630778),
 .UNSPECIFIED.);
#5759=B_SPLINE_CURVE_WITH_KNOTS('',3,(#39199,#39200,#39201,#39202,#39203,
#39204,#39205,#39206,#39207,#39208,#39209,#39210,#39211,#39212,#39213,#39214,
#39215,#39216,#39217,#39218,#39219,#39220,#39221,#39222,#39223),
 .UNSPECIFIED.,.F.,.F.,(4,3,3,3,3,3,3,3,4),(51.5750455984136,51.605831691109,
52.5982515313226,53.5906713715362,54.5830912117499,55.5755110519635,56.5679308921771,
57.5603507323908,57.8582309055933),.UNSPECIFIED.);
#5760=B_SPLINE_CURVE_WITH_KNOTS('',3,(#39224,#39225,#39226,#39227,#39228,
#39229,#39230,#39231,#39232,#39233,#39234,#39235,#39236,#39237,#39238,#39239,
#39240,#39241,#39242,#39243,#39244,#39245),.UNSPECIFIED.,.F.,.F.,(4,3,3,
3,3,3,3,4),(-54.1144568630778,-53.5906713715362,-52.5982515313226,-51.605831691109,
-50.6134118508953,-49.6209920106817,-48.6285721704681,-47.8312715558983),
 .UNSPECIFIED.);
#5761=B_SPLINE_CURVE_WITH_KNOTS('',3,(#39250,#39251,#39252,#39253,#39254,
#39255,#39256,#39257,#39258,#39259,#39260,#39261,#39262,#39263,#39264,#39265,
#39266,#39267,#39268,#39269,#39270,#39271),.UNSPECIFIED.,.F.,.F.,(4,3,3,
3,3,3,3,4),(45.2918602912341,45.6513126498272,46.6437324900408,47.6361523302544,
48.6285721704681,49.6209920106817,50.6134118508953,51.5750455984136),
 .UNSPECIFIED.);
#5762=B_SPLINE_CURVE_WITH_KNOTS('',3,(#39272,#39273,#39274,#39275,#39276,
#39277,#39278,#39279,#39280,#39281,#39282,#39283,#39284,#39285,#39286,#39287,
#39288,#39289,#39290,#39291,#39292,#39293,#39294,#39295,#39296),
 .UNSPECIFIED.,.F.,.F.,(4,3,3,3,3,3,3,3,4),(-47.8312715558983,-47.6361523302544,
-46.6437324900408,-45.6513126498271,-44.6588928096135,-43.6664729693999,
-42.6740531291862,-41.6816332889726,-41.5480862487187),.UNSPECIFIED.);
#5763=B_SPLINE_CURVE_WITH_KNOTS('',3,(#39301,#39302,#39303,#39304,#39305,
#39306,#39307,#39308,#39309,#39310,#39311,#39312,#39313,#39314,#39315,#39316,
#39317,#39318,#39319,#39320,#39321,#39322),.UNSPECIFIED.,.F.,.F.,(4,3,3,
3,3,3,3,4),(39.0086749840545,39.6967936085454,40.689213448759,41.6816332889726,
42.6740531291863,43.6664729693999,44.6588928096135,45.2918602912341),
 .UNSPECIFIED.);
#5764=B_SPLINE_CURVE_WITH_KNOTS('',3,(#39323,#39324,#39325,#39326,#39327,
#39328,#39329,#39330,#39331,#39332,#39333,#39334,#39335,#39336,#39337,#39338,
#39339,#39340,#39341,#39342,#39343,#39344),.UNSPECIFIED.,.F.,.F.,(4,3,3,
3,3,3,3,4),(-41.5480862487187,-40.689213448759,-39.6967936085453,-38.7043737683317,
-37.7119539281181,-36.7195340879044,-35.7271142476908,-35.2649009415392),
 .UNSPECIFIED.);
#5765=B_SPLINE_CURVE_WITH_KNOTS('',3,(#39349,#39350,#39351,#39352,#39353,
#39354,#39355,#39356,#39357,#39358,#39359,#39360,#39361,#39362,#39363,#39364,
#39365,#39366,#39367,#39368,#39369,#39370,#39371,#39372,#39373),
 .UNSPECIFIED.,.F.,.F.,(4,3,3,3,3,3,3,3,4),(32.725489676875,32.7498547270499,
33.7422745672636,34.7346944074772,35.7271142476908,36.7195340879045,37.7119539281181,
38.7043737683317,39.0086749840545),.UNSPECIFIED.);
#5766=B_SPLINE_CURVE_WITH_KNOTS('',3,(#39374,#39375,#39376,#39377,#39378,
#39379,#39380,#39381,#39382,#39383,#39384,#39385,#39386,#39387,#39388,#39389,
#39390,#39391,#39392,#39393,#39394,#39395),.UNSPECIFIED.,.F.,.F.,(4,3,3,
3,3,3,3,4),(-35.2649009415392,-34.7346944074772,-33.7422745672636,-32.7498547270499,
-31.7574348868363,-30.7650150466226,-29.772595206409,-28.9817156343595),
 .UNSPECIFIED.);
#5767=B_SPLINE_CURVE_WITH_KNOTS('',3,(#39400,#39401,#39402,#39403,#39404,
#39405,#39406,#39407,#39408,#39409,#39410,#39411,#39412,#39413,#39414,#39415,
#39416,#39417,#39418,#39419,#39420,#39421),.UNSPECIFIED.,.F.,.F.,(4,3,3,
3,3,3,3,4),(26.4423043696953,26.7953356857681,27.7877555259818,28.7801753661954,
29.772595206409,30.7650150466227,31.7574348868363,32.725489676875),
 .UNSPECIFIED.);
#5768=B_SPLINE_CURVE_WITH_KNOTS('',3,(#39422,#39423,#39424,#39425,#39426,
#39427,#39428,#39429,#39430,#39431,#39432,#39433,#39434,#39435,#39436,#39437,
#39438,#39439,#39440,#39441,#39442,#39443,#39444,#39445,#39446),
 .UNSPECIFIED.,.F.,.F.,(4,3,3,3,3,3,3,3,4),(-28.9817156343595,-28.7801753661954,
-27.7877555259817,-26.7953356857681,-25.8029158455545,-24.8104960053408,
-23.8180761651272,-22.8256563249136,-22.6985303271799),.UNSPECIFIED.);
#5769=B_SPLINE_CURVE_WITH_KNOTS('',3,(#39451,#39452,#39453,#39454,#39455,
#39456,#39457,#39458,#39459,#39460,#39461,#39462,#39463,#39464,#39465,#39466,
#39467,#39468,#39469,#39470,#39471,#39472),.UNSPECIFIED.,.F.,.F.,(4,3,3,
3,3,3,3,4),(20.1591190625157,20.8408166444863,21.8332364847,22.8256563249136,
23.8180761651272,24.8104960053409,25.8029158455545,26.4423043696953),
 .UNSPECIFIED.);
#5770=B_SPLINE_CURVE_WITH_KNOTS('',3,(#39473,#39474,#39475,#39476,#39477,
#39478,#39479,#39480,#39481,#39482,#39483,#39484,#39485,#39486,#39487,#39488,
#39489,#39490,#39491,#39492,#39493,#39494),.UNSPECIFIED.,.F.,.F.,(4,3,3,
3,3,3,3,4),(-22.6985303271799,-21.8332364846999,-20.8408166444863,-19.8483968042727,
-18.855976964059,-17.8635571238454,-16.8711372836318,-16.4153450200004),
 .UNSPECIFIED.);
#5771=B_SPLINE_CURVE_WITH_KNOTS('',3,(#39499,#39500,#39501,#39502,#39503,
#39504,#39505,#39506,#39507,#39508,#39509,#39510,#39511,#39512,#39513,#39514,
#39515,#39516,#39517,#39518,#39519,#39520,#39521,#39522,#39523),
 .UNSPECIFIED.,.F.,.F.,(4,3,3,3,3,3,3,3,4),(13.8759337553361,13.8938777629909,
14.8862976032045,15.8787174434181,16.8711372836318,17.8635571238454,18.8559769640591,
19.8483968042727,20.1591190625157),.UNSPECIFIED.);
#5772=B_SPLINE_CURVE_WITH_KNOTS('',3,(#39524,#39525,#39526,#39527,#39528,
#39529,#39530,#39531,#39532,#39533,#39534,#39535,#39536,#39537,#39538,#39539,
#39540,#39541,#39542,#39543,#39544,#39545),.UNSPECIFIED.,.F.,.F.,(4,3,3,
3,3,3,3,4),(-16.4153450200004,-15.8787174434181,-14.8862976032045,-13.8938777629909,
-12.9014579227772,-11.9090380825636,-10.91661824235,-10.1321597128208),
 .UNSPECIFIED.);
#5773=B_SPLINE_CURVE_WITH_KNOTS('',3,(#39551,#39552,#39553,#39554,#39555,
#39556,#39557,#39558,#39559,#39560,#39561,#39562,#39563),.UNSPECIFIED.,
 .F.,.F.,(4,3,3,3,4),(-3.84897440564123,-2.9772595206409,-1.98483968042727,
-0.992419840213635,0.),.UNSPECIFIED.);
#5774=B_SPLINE_CURVE_WITH_KNOTS('',3,(#39566,#39567,#39568,#39569,#39570,
#39571,#39572,#39573,#39574,#39575,#39576,#39577,#39578,#39579,#39580,#39581,
#39582,#39583,#39584),.UNSPECIFIED.,.F.,.F.,(4,3,3,3,3,3,4),(2.01694489302852,
2.9772595206409,3.96967936085453,4.96209920106817,5.9545190412818,6.94693888149544,
7.59274844815659),.UNSPECIFIED.);
#5775=B_SPLINE_CURVE_WITH_KNOTS('',3,(#39590,#39591,#39592,#39593,#39594,
#39595,#39596,#39597),.UNSPECIFIED.,.F.,.F.,(4,1,1,1,1,4),(103.672557568463,
104.154034002176,105.146453842389,106.138873682603,107.131293522817,108.12371336303),
 .UNSPECIFIED.);
#5776=B_SPLINE_CURVE_WITH_KNOTS('',3,(#39600,#39601,#39602,#39603,#39604,
#39605,#39606,#39607,#39608),.UNSPECIFIED.,.F.,.F.,(4,1,1,1,1,1,4),(103.672557568463,
103.716185746199,104.708605586413,105.701025426626,106.69344526684,107.685865107053,
108.646179734666),.UNSPECIFIED.);
#5777=B_SPLINE_CURVE_WITH_KNOTS('',3,(#39613,#39614,#39615,#39616,#39617,
#39618,#39619,#39620,#39621,#39622),.UNSPECIFIED.,.F.,.F.,(4,1,1,1,1,1,
1,4),(97.3893722612835,98.1995149608939,99.1919348011075,100.184354641321,
101.176774481535,102.169194321748,103.161614161962,103.672557568463),
 .UNSPECIFIED.);
#5778=B_SPLINE_CURVE_WITH_KNOTS('',3,(#39623,#39624,#39625,#39626,#39627,
#39628,#39629,#39630,#39631,#39632),.UNSPECIFIED.,.F.,.F.,(4,1,1,1,1,1,
1,4),(97.3893722612835,97.7616667049171,98.7540865451307,99.7465063853443,
100.738926225558,101.731346065772,102.723765905985,103.672557568463),
 .UNSPECIFIED.);
#5779=B_SPLINE_CURVE_WITH_KNOTS('',3,(#39637,#39638,#39639,#39640,#39641,
#39642,#39643,#39644,#39645,#39646,#39647),.UNSPECIFIED.,.F.,.F.,(4,1,1,
1,1,1,1,1,4),(91.106186954104,91.2525760793984,92.2449959196121,93.2374157598257,
94.2298356000393,95.222255440253,96.2146752804666,97.2070951206802,97.3893722612835),
 .UNSPECIFIED.);
#5780=B_SPLINE_CURVE_WITH_KNOTS('',3,(#39648,#39649,#39650,#39651,#39652,
#39653,#39654,#39655,#39656,#39657),.UNSPECIFIED.,.F.,.F.,(4,1,1,1,1,1,
1,4),(91.106186954104,91.8071476636353,92.7995675038489,93.7919873440625,
94.7844071842762,95.7768270244898,96.7692468647034,97.3893722612835),
 .UNSPECIFIED.);
#5781=B_SPLINE_CURVE_WITH_KNOTS('',3,(#39662,#39663,#39664,#39665,#39666,
#39667,#39668,#39669,#39670,#39671),.UNSPECIFIED.,.F.,.F.,(4,1,1,1,1,1,
1,4),(84.8230016469244,85.2980570381166,86.2904768783303,87.2828967185439,
88.2753165587575,89.2677363989712,90.2601562391848,91.106186954104),
 .UNSPECIFIED.);
#5782=B_SPLINE_CURVE_WITH_KNOTS('',3,(#39672,#39673,#39674,#39675,#39676,
#39677,#39678,#39679,#39680,#39681,#39682),.UNSPECIFIED.,.F.,.F.,(4,1,1,
1,1,1,1,1,4),(84.8230016469244,84.8602087821398,85.8526286223535,86.8450484625671,
87.8374683027807,88.8298881429944,89.822307983208,90.8147278234216,91.106186954104),
 .UNSPECIFIED.);
#5783=B_SPLINE_CURVE_WITH_KNOTS('',3,(#39687,#39688,#39689,#39690,#39691,
#39692,#39693,#39694,#39695,#39696),.UNSPECIFIED.,.F.,.F.,(4,1,1,1,1,1,
1,4),(78.5398163397448,79.3435379968348,80.3359578370484,81.3283776772621,
82.3207975174757,83.3132173576894,84.305637197903,84.8230016469244),
 .UNSPECIFIED.);
#5784=B_SPLINE_CURVE_WITH_KNOTS('',3,(#39697,#39698,#39699,#39700,#39701,
#39702,#39703,#39704,#39705,#39706),.UNSPECIFIED.,.F.,.F.,(4,1,1,1,1,1,
1,4),(78.5398163397448,78.905689740858,79.8981095810717,80.8905294212853,
81.8829492614989,82.8753691017126,83.8677889419262,84.8230016469244),
 .UNSPECIFIED.);
#5785=B_SPLINE_CURVE_WITH_KNOTS('',3,(#39711,#39712,#39713,#39714,#39715,
#39716,#39717,#39718,#39719,#39720,#39721),.UNSPECIFIED.,.F.,.F.,(4,1,1,
1,1,1,1,1,4),(72.2566310325651,72.3965991153394,73.389018955553,74.3814387957666,
75.3738586359803,76.3662784761939,77.3586983164075,78.3511181566212,78.5398163397448),
 .UNSPECIFIED.);
#5786=B_SPLINE_CURVE_WITH_KNOTS('',3,(#39722,#39723,#39724,#39725,#39726,
#39727,#39728,#39729,#39730,#39731),.UNSPECIFIED.,.F.,.F.,(4,1,1,1,1,1,
1,4),(72.2566310325651,72.9511706995762,73.9435905397899,74.9360103800035,
75.9284302202171,76.9208500604308,77.9132699006444,78.5398163397448),
 .UNSPECIFIED.);
#5787=B_SPLINE_CURVE_WITH_KNOTS('',3,(#39736,#39737,#39738,#39739,#39740,
#39741,#39742,#39743,#39744,#39745),.UNSPECIFIED.,.F.,.F.,(4,1,1,1,1,1,
1,4),(65.9734457253856,66.4420800740576,67.4344999142712,68.4269197544848,
69.4193395946985,70.4117594349121,71.4041792751257,72.2566310325651),
 .UNSPECIFIED.);
#5788=B_SPLINE_CURVE_WITH_KNOTS('',3,(#39746,#39747,#39748,#39749,#39750,
#39751,#39752,#39753,#39754,#39755,#39756),.UNSPECIFIED.,.F.,.F.,(4,1,1,
1,1,1,1,1,4),(65.9734457253856,66.0042318180808,66.9966516582944,67.9890714985081,
68.9814913387217,69.9739111789353,70.966331019149,71.9587508593626,72.2566310325651),
 .UNSPECIFIED.);
#5789=B_SPLINE_CURVE_WITH_KNOTS('',3,(#39761,#39762,#39763,#39764,#39765,
#39766,#39767,#39768,#39769,#39770),.UNSPECIFIED.,.F.,.F.,(4,1,1,1,1,1,
1,4),(59.690260418206,60.4875610327758,61.4799808729894,62.472400713203,
63.4648205534167,64.4572403936303,65.4496602338439,65.9734457253856),
 .UNSPECIFIED.);
#5790=B_SPLINE_CURVE_WITH_KNOTS('',3,(#39771,#39772,#39773,#39774,#39775,
#39776,#39777,#39778,#39779,#39780),.UNSPECIFIED.,.F.,.F.,(4,1,1,1,1,1,
1,4),(59.690260418206,60.049712776799,61.0421326170126,62.0345524572262,
63.0269722974399,64.0193921376535,65.0118119778672,65.9734457253856),
 .UNSPECIFIED.);
#5791=B_SPLINE_CURVE_WITH_KNOTS('',3,(#39785,#39786,#39787,#39788,#39789,
#39790,#39791,#39792,#39793,#39794,#39795),.UNSPECIFIED.,.F.,.F.,(4,1,1,
1,1,1,1,1,4),(53.4070751110265,53.5406221512803,54.533041991494,55.5254618317076,
56.5178816719212,57.5103015121349,58.5027213523485,59.4951411925621,59.690260418206),
 .UNSPECIFIED.);
#5792=B_SPLINE_CURVE_WITH_KNOTS('',3,(#39796,#39797,#39798,#39799,#39800,
#39801,#39802,#39803,#39804,#39805),.UNSPECIFIED.,.F.,.F.,(4,1,1,1,1,1,
1,4),(53.4070751110265,54.0951937355172,55.0876135757308,56.0800334159444,
57.0724532561581,58.0648730963717,59.0572929365853,59.690260418206),
 .UNSPECIFIED.);
#5793=B_SPLINE_CURVE_WITH_KNOTS('',3,(#39810,#39811,#39812,#39813,#39814,
#39815,#39816,#39817,#39818,#39819),.UNSPECIFIED.,.F.,.F.,(4,1,1,1,1,1,
1,4),(47.1238898038468,47.5861031099985,48.5785229502122,49.5709427904258,
50.5633626306394,51.5557824708531,52.5482023110667,53.4070751110265),
 .UNSPECIFIED.);
#5794=B_SPLINE_CURVE_WITH_KNOTS('',3,(#39820,#39821,#39822,#39823,#39824,
#39825,#39826,#39827,#39828,#39829,#39830),.UNSPECIFIED.,.F.,.F.,(4,1,1,
1,1,1,1,1,4),(47.1238898038468,47.1482548540217,48.1406746942354,49.133094534449,
50.1255143746626,51.1179342148763,52.1103540550899,53.1027738953035,53.4070751110265),
 .UNSPECIFIED.);
#5795=B_SPLINE_CURVE_WITH_KNOTS('',3,(#39835,#39836,#39837,#39838,#39839,
#39840,#39841,#39842,#39843,#39844),.UNSPECIFIED.,.F.,.F.,(4,1,1,1,1,1,
1,4),(40.8407044966672,41.6315840687167,42.6240039089304,43.616423749144,
44.6088435893576,45.6012634295713,46.5936832697849,47.1238898038468),
 .UNSPECIFIED.);
#5796=B_SPLINE_CURVE_WITH_KNOTS('',3,(#39845,#39846,#39847,#39848,#39849,
#39850,#39851,#39852,#39853,#39854),.UNSPECIFIED.,.F.,.F.,(4,1,1,1,1,1,
1,4),(40.8407044966672,41.1937358127399,42.1861556529536,43.1785754931672,
44.1709953333808,45.1634151735945,46.1558350138081,47.1238898038468),
 .UNSPECIFIED.);
#5797=B_SPLINE_CURVE_WITH_KNOTS('',3,(#39859,#39860,#39861,#39862,#39863,
#39864,#39865,#39866,#39867,#39868,#39869),.UNSPECIFIED.,.F.,.F.,(4,1,1,
1,1,1,1,1,4),(34.5575191894877,34.6846451872213,35.6770650274349,36.6694848676485,
37.6619047078622,38.6543245480758,39.6467443882895,40.6391642285031,40.8407044966672),
 .UNSPECIFIED.);
#5798=B_SPLINE_CURVE_WITH_KNOTS('',3,(#39870,#39871,#39872,#39873,#39874,
#39875,#39876,#39877,#39878,#39879),.UNSPECIFIED.,.F.,.F.,(4,1,1,1,1,1,
1,4),(34.5575191894877,35.2392167714581,36.2316366116718,37.2240564518854,
38.216476292099,39.2088961323127,40.2013159725263,40.8407044966672),
 .UNSPECIFIED.);
#5799=B_SPLINE_CURVE_WITH_KNOTS('',3,(#39884,#39885,#39886,#39887,#39888,
#39889,#39890,#39891,#39892,#39893),.UNSPECIFIED.,.F.,.F.,(4,1,1,1,1,1,
1,4),(28.2743338823081,28.7301261459395,29.7225459861531,30.7149658263668,
31.7073856665804,32.699805506794,33.6922253470076,34.5575191894877),
 .UNSPECIFIED.);
#5800=B_SPLINE_CURVE_WITH_KNOTS('',3,(#39894,#39895,#39896,#39897,#39898,
#39899,#39900,#39901,#39902,#39903,#39904),.UNSPECIFIED.,.F.,.F.,(4,1,1,
1,1,1,1,1,4),(28.2743338823081,28.2922778899627,29.2846977301763,30.27711757039,
31.2695374106036,32.2619572508172,33.2543770910309,34.2467969312445,34.5575191894877),
 .UNSPECIFIED.);
#5801=B_SPLINE_CURVE_WITH_KNOTS('',3,(#39909,#39910,#39911,#39912,#39913,
#39914,#39915,#39916,#39917,#39918),.UNSPECIFIED.,.F.,.F.,(4,1,1,1,1,1,
1,4),(21.9911485751284,22.7756071046577,23.7680269448713,24.7604467850849,
25.7528666252986,26.7452864655122,27.7377063057259,28.2743338823081),
 .UNSPECIFIED.);
#5802=B_SPLINE_CURVE_WITH_KNOTS('',3,(#39919,#39920,#39921,#39922,#39923,
#39924,#39925,#39926,#39927,#39928),.UNSPECIFIED.,.F.,.F.,(4,1,1,1,1,1,
1,4),(21.9911485751284,22.3377588486809,23.3301786888945,24.3225985291082,
25.3150183693218,26.3074382095354,27.2998580497491,28.2743338823081),
 .UNSPECIFIED.);
#5803=B_SPLINE_CURVE_WITH_KNOTS('',3,(#39934,#39935,#39936,#39937,#39938),
 .UNSPECIFIED.,.F.,.F.,(4,1,4),(14.3984001269718,15.3908199671854,15.7079632679489),
 .UNSPECIFIED.);
#5804=B_SPLINE_CURVE_WITH_KNOTS('',3,(#39941,#39942,#39943,#39944,#39945),
 .UNSPECIFIED.,.F.,.F.,(4,1,4),(13.8759337553363,14.8362483829486,15.7079632679489),
 .UNSPECIFIED.);
#5805=B_SPLINE_CURVE_WITH_KNOTS('',3,(#39951,#39952,#39953,#39954),
 .UNSPECIFIED.,.F.,.F.,(4,4),(95.5573427486708,96.2647245007222),
 .UNSPECIFIED.);
#5806=B_SPLINE_CURVE_WITH_KNOTS('',3,(#39962,#39963,#39964,#39965,#39966,
#39967,#39968,#39969,#39970,#39971),.UNSPECIFIED.,.F.,.F.,(4,3,3,4),(-94.2477796076937,
-93.2874649800814,-92.2950451398677,-91.8135687061555),.UNSPECIFIED.);
#5807=B_SPLINE_CURVE_WITH_KNOTS('',3,(#39976,#39977,#39978,#39979,#39980,
#39981,#39982,#39983,#39984,#39985,#39986,#39987,#39988,#39989,#39990,#39991,
#39992,#39993,#39994,#39995,#39996,#39997,#39998,#39999,#40000),
 .UNSPECIFIED.,.F.,.F.,(4,3,3,3,3,3,3,3,4),(89.2741574414912,89.3177856192269,
90.3102054594405,91.3026252996541,92.2950451398678,93.2874649800814,94.279884820295,
95.2723046605086,95.5573427486708),.UNSPECIFIED.);
#5808=B_SPLINE_CURVE_WITH_KNOTS('',3,(#40001,#40002,#40003,#40004,#40005,
#40006,#40007,#40008,#40009,#40010,#40011,#40012,#40013,#40014,#40015,#40016,
#40017,#40018,#40019,#40020,#40021,#40022),.UNSPECIFIED.,.F.,.F.,(4,3,3,
3,3,3,3,4),(-91.8135687061555,-91.3026252996541,-90.3102054594405,-89.3177856192268,
-88.3253657790132,-87.3329459387996,-86.340526098586,-85.5303833989758),
 .UNSPECIFIED.);
#5809=B_SPLINE_CURVE_WITH_KNOTS('',3,(#40027,#40028,#40029,#40030,#40031,
#40032,#40033,#40034,#40035,#40036,#40037,#40038,#40039,#40040,#40041,#40042,
#40043,#40044,#40045,#40046,#40047,#40048),.UNSPECIFIED.,.F.,.F.,(4,3,3,
3,3,3,3,4),(82.9909721343117,83.3632665779451,84.3556864181587,85.3481062583723,
86.340526098586,87.3329459387996,88.3253657790132,89.2741574414912),
 .UNSPECIFIED.);
#5810=B_SPLINE_CURVE_WITH_KNOTS('',3,(#40049,#40050,#40051,#40052,#40053,
#40054,#40055,#40056,#40057,#40058,#40059,#40060,#40061,#40062,#40063,#40064,
#40065,#40066,#40067,#40068,#40069,#40070,#40071,#40072,#40073),
 .UNSPECIFIED.,.F.,.F.,(4,3,3,3,3,3,3,3,4),(-85.5303833989758,-85.3481062583723,
-84.3556864181587,-83.3632665779451,-82.3708467377314,-81.3784268975178,
-80.3860070573042,-79.3935872170905,-79.2471980917962),.UNSPECIFIED.);
#5811=B_SPLINE_CURVE_WITH_KNOTS('',3,(#40078,#40079,#40080,#40081,#40082,
#40083,#40084,#40085,#40086,#40087,#40088,#40089,#40090,#40091,#40092,#40093,
#40094,#40095,#40096,#40097,#40098,#40099),.UNSPECIFIED.,.F.,.F.,(4,3,3,
3,3,3,3,4),(76.707786827132,77.4087475366633,78.4011673768769,79.3935872170906,
80.3860070573042,81.3784268975178,82.3708467377314,82.9909721343117),
 .UNSPECIFIED.);
#5812=B_SPLINE_CURVE_WITH_KNOTS('',3,(#40100,#40101,#40102,#40103,#40104,
#40105,#40106,#40107,#40108,#40109,#40110,#40111,#40112,#40113,#40114,#40115,
#40116,#40117,#40118,#40119,#40120,#40121),.UNSPECIFIED.,.F.,.F.,(4,3,3,
3,3,3,3,4),(-79.2471980917962,-78.4011673768769,-77.4087475366633,-76.4163276964496,
-75.423907856236,-74.4314880160224,-73.4390681758087,-72.9640127846167),
 .UNSPECIFIED.);
#5813=B_SPLINE_CURVE_WITH_KNOTS('',3,(#40126,#40127,#40128,#40129,#40130,
#40131,#40132,#40133,#40134,#40135,#40136,#40137,#40138,#40139,#40140,#40141,
#40142,#40143,#40144,#40145,#40146,#40147,#40148,#40149,#40150),
 .UNSPECIFIED.,.F.,.F.,(4,3,3,3,3,3,3,3,4),(70.4246015199524,70.4618086551678,
71.4542284953815,72.4466483355951,73.4390681758087,74.4314880160224,75.423907856236,
76.4163276964497,76.707786827132),.UNSPECIFIED.);
#5814=B_SPLINE_CURVE_WITH_KNOTS('',3,(#40151,#40152,#40153,#40154,#40155,
#40156,#40157,#40158,#40159,#40160,#40161,#40162,#40163,#40164,#40165,#40166,
#40167,#40168,#40169,#40170,#40171,#40172),.UNSPECIFIED.,.F.,.F.,(4,3,3,
3,3,3,3,4),(-72.9640127846167,-72.4466483355951,-71.4542284953815,-70.4618086551678,
-69.4693888149542,-68.4769689747406,-67.4845491345269,-66.6808274774371),
 .UNSPECIFIED.);
#5815=B_SPLINE_CURVE_WITH_KNOTS('',3,(#40177,#40178,#40179,#40180,#40181,
#40182,#40183,#40184,#40185,#40186,#40187,#40188,#40189,#40190,#40191,#40192,
#40193,#40194,#40195,#40196,#40197,#40198),.UNSPECIFIED.,.F.,.F.,(4,3,3,
3,3,3,3,4),(64.1414162127729,64.5072896138861,65.4997094540997,66.4921292943133,
67.4845491345269,68.4769689747406,69.4693888149542,70.4246015199524),
 .UNSPECIFIED.);
#5816=B_SPLINE_CURVE_WITH_KNOTS('',3,(#40199,#40200,#40201,#40202,#40203,
#40204,#40205,#40206,#40207,#40208,#40209,#40210,#40211,#40212,#40213,#40214,
#40215,#40216,#40217,#40218,#40219,#40220,#40221,#40222,#40223),
 .UNSPECIFIED.,.F.,.F.,(4,3,3,3,3,3,3,3,4),(-66.6808274774371,-66.4921292943133,
-65.4997094540997,-64.507289613886,-63.5148697736724,-62.5224499334588,
-61.5300300932452,-60.5376102530315,-60.3976421702574),.UNSPECIFIED.);
#5817=B_SPLINE_CURVE_WITH_KNOTS('',3,(#40228,#40229,#40230,#40231,#40232,
#40233,#40234,#40235,#40236,#40237,#40238,#40239,#40240,#40241,#40242,#40243,
#40244,#40245,#40246,#40247,#40248,#40249),.UNSPECIFIED.,.F.,.F.,(4,3,3,
3,3,3,3,4),(57.8582309055933,58.5527705726043,59.5451904128179,60.5376102530315,
61.5300300932452,62.5224499334588,63.5148697736725,64.1414162127729),
 .UNSPECIFIED.);
#5818=B_SPLINE_CURVE_WITH_KNOTS('',3,(#40250,#40251,#40252,#40253,#40254,
#40255,#40256,#40257,#40258,#40259,#40260,#40261,#40262,#40263,#40264,#40265,
#40266,#40267,#40268,#40269,#40270,#40271),.UNSPECIFIED.,.F.,.F.,(4,3,3,
3,3,3,3,4),(-60.3976421702574,-59.5451904128179,-58.5527705726043,-57.5603507323906,
-56.567930892177,-55.5755110519634,-54.5830912117497,-54.1144568630778),
 .UNSPECIFIED.);
#5819=B_SPLINE_CURVE_WITH_KNOTS('',3,(#40276,#40277,#40278,#40279,#40280,
#40281,#40282,#40283,#40284,#40285,#40286,#40287,#40288,#40289,#40290,#40291,
#40292,#40293,#40294,#40295,#40296,#40297,#40298,#40299,#40300),
 .UNSPECIFIED.,.F.,.F.,(4,3,3,3,3,3,3,3,4),(51.5750455984136,51.6058316911088,
52.5982515313225,53.5906713715361,54.5830912117497,55.5755110519634,56.567930892177,
57.5603507323906,57.8582309055933),.UNSPECIFIED.);
#5820=B_SPLINE_CURVE_WITH_KNOTS('',3,(#40301,#40302,#40303,#40304,#40305,
#40306,#40307,#40308,#40309,#40310,#40311,#40312,#40313,#40314,#40315,#40316,
#40317,#40318,#40319,#40320,#40321,#40322),.UNSPECIFIED.,.F.,.F.,(4,3,3,
3,3,3,3,4),(-54.1144568630778,-53.5906713715361,-52.5982515313225,-51.6058316911088,
-50.6134118508952,-49.6209920106816,-48.6285721704679,-47.8312715558983),
 .UNSPECIFIED.);
#5821=B_SPLINE_CURVE_WITH_KNOTS('',3,(#40327,#40328,#40329,#40330,#40331,
#40332,#40333,#40334,#40335,#40336,#40337,#40338,#40339,#40340,#40341,#40342,
#40343,#40344,#40345,#40346,#40347,#40348),.UNSPECIFIED.,.F.,.F.,(4,3,3,
3,3,3,3,4),(45.2918602912341,45.6513126498271,46.6437324900407,47.6361523302543,
48.628572170468,49.6209920106816,50.6134118508952,51.5750455984136),
 .UNSPECIFIED.);
#5822=B_SPLINE_CURVE_WITH_KNOTS('',3,(#40349,#40350,#40351,#40352,#40353,
#40354,#40355,#40356,#40357,#40358,#40359,#40360,#40361,#40362,#40363,#40364,
#40365,#40366,#40367,#40368,#40369,#40370,#40371,#40372,#40373),
 .UNSPECIFIED.,.F.,.F.,(4,3,3,3,3,3,3,3,4),(-47.8312715558983,-47.6361523302543,
-46.6437324900407,-45.651312649827,-44.6588928096134,-43.6664729693998,
-42.6740531291861,-41.6816332889725,-41.5480862487187),.UNSPECIFIED.);
#5823=B_SPLINE_CURVE_WITH_KNOTS('',3,(#40378,#40379,#40380,#40381,#40382,
#40383,#40384,#40385,#40386,#40387,#40388,#40389,#40390,#40391,#40392,#40393,
#40394,#40395,#40396,#40397,#40398,#40399),.UNSPECIFIED.,.F.,.F.,(4,3,3,
3,3,3,3,4),(39.0086749840545,39.6967936085453,40.6892134487589,41.6816332889725,
42.6740531291862,43.6664729693998,44.6588928096134,45.2918602912341),
 .UNSPECIFIED.);
#5824=B_SPLINE_CURVE_WITH_KNOTS('',3,(#40400,#40401,#40402,#40403,#40404,
#40405,#40406,#40407,#40408,#40409,#40410,#40411,#40412,#40413,#40414,#40415,
#40416,#40417,#40418,#40419,#40420,#40421),.UNSPECIFIED.,.F.,.F.,(4,3,3,
3,3,3,3,4),(-41.5480862487187,-40.6892134487589,-39.6967936085453,-38.7043737683316,
-37.711953928118,-36.7195340879044,-35.7271142476907,-35.264900941539),
 .UNSPECIFIED.);
#5825=B_SPLINE_CURVE_WITH_KNOTS('',3,(#40426,#40427,#40428,#40429,#40430,
#40431,#40432,#40433,#40434,#40435,#40436,#40437,#40438,#40439,#40440,#40441,
#40442,#40443,#40444,#40445,#40446,#40447,#40448,#40449,#40450),
 .UNSPECIFIED.,.F.,.F.,(4,3,3,3,3,3,3,3,4),(32.725489676875,32.7498547270498,
33.7422745672635,34.7346944074771,35.7271142476907,36.7195340879044,37.711953928118,
38.7043737683316,39.0086749840545),.UNSPECIFIED.);
#5826=B_SPLINE_CURVE_WITH_KNOTS('',3,(#40451,#40452,#40453,#40454,#40455,
#40456,#40457,#40458,#40459,#40460,#40461,#40462,#40463,#40464,#40465,#40466,
#40467,#40468,#40469,#40470,#40471,#40472),.UNSPECIFIED.,.F.,.F.,(4,3,3,
3,3,3,3,4),(-35.264900941539,-34.7346944074771,-33.7422745672635,-32.7498547270498,
-31.7574348868362,-30.7650150466226,-29.7725952064089,-28.9817156343595),
 .UNSPECIFIED.);
#5827=B_SPLINE_CURVE_WITH_KNOTS('',3,(#40477,#40478,#40479,#40480,#40481,
#40482,#40483,#40484,#40485,#40486,#40487,#40488,#40489,#40490,#40491,#40492,
#40493,#40494,#40495,#40496,#40497,#40498),.UNSPECIFIED.,.F.,.F.,(4,3,3,
3,3,3,3,4),(26.4423043696953,26.7953356857681,27.7877555259817,28.7801753661953,
29.772595206409,30.7650150466226,31.7574348868362,32.725489676875),
 .UNSPECIFIED.);
#5828=B_SPLINE_CURVE_WITH_KNOTS('',3,(#40499,#40500,#40501,#40502,#40503,
#40504,#40505,#40506,#40507,#40508,#40509,#40510,#40511,#40512,#40513,#40514,
#40515,#40516,#40517,#40518,#40519,#40520,#40521,#40522,#40523),
 .UNSPECIFIED.,.F.,.F.,(4,3,3,3,3,3,3,3,4),(-28.9817156343595,-28.7801753661953,
-27.7877555259817,-26.7953356857681,-25.8029158455544,-24.8104960053408,
-23.8180761651271,-22.8256563249135,-22.6985303271799),.UNSPECIFIED.);
#5829=B_SPLINE_CURVE_WITH_KNOTS('',3,(#40528,#40529,#40530,#40531,#40532,
#40533,#40534,#40535,#40536,#40537,#40538,#40539,#40540,#40541,#40542,#40543,
#40544,#40545,#40546,#40547,#40548,#40549),.UNSPECIFIED.,.F.,.F.,(4,3,3,
3,3,3,3,4),(20.1591190625157,20.8408166444863,21.8332364846999,22.8256563249135,
23.8180761651272,24.8104960053408,25.8029158455544,26.4423043696953),
 .UNSPECIFIED.);
#5830=B_SPLINE_CURVE_WITH_KNOTS('',3,(#40550,#40551,#40552,#40553,#40554,
#40555,#40556,#40557,#40558,#40559,#40560,#40561,#40562,#40563,#40564,#40565,
#40566,#40567,#40568,#40569,#40570,#40571),.UNSPECIFIED.,.F.,.F.,(4,3,3,
3,3,3,3,4),(-22.6985303271799,-21.8332364846999,-20.8408166444862,-19.8483968042726,
-18.855976964059,-17.8635571238454,-16.8711372836317,-16.4153450200004),
 .UNSPECIFIED.);
#5831=B_SPLINE_CURVE_WITH_KNOTS('',3,(#40576,#40577,#40578,#40579,#40580,
#40581,#40582,#40583,#40584,#40585,#40586,#40587,#40588,#40589,#40590,#40591,
#40592,#40593,#40594,#40595,#40596,#40597,#40598,#40599,#40600),
 .UNSPECIFIED.,.F.,.F.,(4,3,3,3,3,3,3,3,4),(13.8759337553361,13.8938777629908,
14.8862976032045,15.8787174434181,16.8711372836317,17.8635571238454,18.855976964059,
19.8483968042726,20.1591190625157),.UNSPECIFIED.);
#5832=B_SPLINE_CURVE_WITH_KNOTS('',3,(#40601,#40602,#40603,#40604,#40605,
#40606,#40607,#40608,#40609,#40610,#40611,#40612,#40613,#40614,#40615,#40616,
#40617,#40618,#40619,#40620,#40621,#40622),.UNSPECIFIED.,.F.,.F.,(4,3,3,
3,3,3,3,4),(-16.4153450200004,-15.8787174434181,-14.8862976032045,-13.8938777629908,
-12.9014579227772,-11.9090380825636,-10.9166182423499,-10.1321597128208),
 .UNSPECIFIED.);
#5833=B_SPLINE_CURVE_WITH_KNOTS('',3,(#40628,#40629,#40630,#40631,#40632,
#40633,#40634,#40635,#40636,#40637,#40638,#40639,#40640),.UNSPECIFIED.,
 .F.,.F.,(4,3,3,3,4),(-3.84897440564112,-2.97725952064089,-1.98483968042726,
-0.992419840213629,0.),.UNSPECIFIED.);
#5834=B_SPLINE_CURVE_WITH_KNOTS('',3,(#40643,#40644,#40645,#40646,#40647,
#40648,#40649,#40650,#40651,#40652,#40653,#40654,#40655,#40656,#40657,#40658,
#40659,#40660,#40661),.UNSPECIFIED.,.F.,.F.,(4,3,3,3,3,3,4),(2.01694489302852,
2.9772595206409,3.96967936085453,4.96209920106816,5.95451904128179,6.94693888149542,
7.59274844815659),.UNSPECIFIED.);
#5835=B_SPLINE_CURVE_WITH_KNOTS('',3,(#40667,#40668,#40669,#40670,#40671,
#40672,#40673,#40674),.UNSPECIFIED.,.F.,.F.,(4,1,1,1,1,4),(103.672557568463,
104.154034002175,105.146453842389,106.138873682603,107.131293522816,108.12371336303),
 .UNSPECIFIED.);
#5836=B_SPLINE_CURVE_WITH_KNOTS('',3,(#40677,#40678,#40679,#40680,#40681,
#40682,#40683,#40684,#40685),.UNSPECIFIED.,.F.,.F.,(4,1,1,1,1,1,4),(103.672557568463,
103.716185746199,104.708605586412,105.701025426626,106.69344526684,107.685865107053,
108.646179734666),.UNSPECIFIED.);
#5837=B_SPLINE_CURVE_WITH_KNOTS('',3,(#40690,#40691,#40692,#40693,#40694,
#40695,#40696,#40697,#40698,#40699),.UNSPECIFIED.,.F.,.F.,(4,1,1,1,1,1,
1,4),(97.3893722612835,98.1995149608937,99.1919348011073,100.184354641321,
101.176774481535,102.169194321748,103.161614161962,103.672557568463),
 .UNSPECIFIED.);
#5838=B_SPLINE_CURVE_WITH_KNOTS('',3,(#40700,#40701,#40702,#40703,#40704,
#40705,#40706,#40707,#40708,#40709),.UNSPECIFIED.,.F.,.F.,(4,1,1,1,1,1,
1,4),(97.3893722612835,97.7616667049169,98.7540865451305,99.7465063853441,
100.738926225558,101.731346065771,102.723765905985,103.672557568463),
 .UNSPECIFIED.);
#5839=B_SPLINE_CURVE_WITH_KNOTS('',3,(#40714,#40715,#40716,#40717,#40718,
#40719,#40720,#40721,#40722,#40723,#40724),.UNSPECIFIED.,.F.,.F.,(4,1,1,
1,1,1,1,1,4),(91.106186954104,91.2525760793982,92.2449959196119,93.2374157598255,
94.2298356000391,95.2222554402528,96.2146752804664,97.20709512068,97.3893722612835),
 .UNSPECIFIED.);
#5840=B_SPLINE_CURVE_WITH_KNOTS('',3,(#40725,#40726,#40727,#40728,#40729,
#40730,#40731,#40732,#40733,#40734),.UNSPECIFIED.,.F.,.F.,(4,1,1,1,1,1,
1,4),(91.106186954104,91.8071476636351,92.7995675038487,93.7919873440624,
94.784407184276,95.7768270244896,96.7692468647032,97.3893722612835),
 .UNSPECIFIED.);
#5841=B_SPLINE_CURVE_WITH_KNOTS('',3,(#40739,#40740,#40741,#40742,#40743,
#40744,#40745,#40746,#40747,#40748),.UNSPECIFIED.,.F.,.F.,(4,1,1,1,1,1,
1,4),(84.8230016469244,85.2980570381164,86.2904768783301,87.2828967185437,
88.2753165587573,89.267736398971,90.2601562391846,91.106186954104),
 .UNSPECIFIED.);
#5842=B_SPLINE_CURVE_WITH_KNOTS('',3,(#40749,#40750,#40751,#40752,#40753,
#40754,#40755,#40756,#40757,#40758,#40759),.UNSPECIFIED.,.F.,.F.,(4,1,1,
1,1,1,1,1,4),(84.8230016469244,84.8602087821397,85.8526286223533,86.8450484625669,
87.8374683027806,88.8298881429942,89.8223079832078,90.8147278234215,91.106186954104),
 .UNSPECIFIED.);
#5843=B_SPLINE_CURVE_WITH_KNOTS('',3,(#40764,#40765,#40766,#40767,#40768,
#40769,#40770,#40771,#40772,#40773),.UNSPECIFIED.,.F.,.F.,(4,1,1,1,1,1,
1,4),(78.5398163397448,79.3435379968347,80.3359578370483,81.3283776772619,
82.3207975174756,83.3132173576892,84.3056371979028,84.8230016469244),
 .UNSPECIFIED.);
#5844=B_SPLINE_CURVE_WITH_KNOTS('',3,(#40774,#40775,#40776,#40777,#40778,
#40779,#40780,#40781,#40782,#40783),.UNSPECIFIED.,.F.,.F.,(4,1,1,1,1,1,
1,4),(78.5398163397448,78.9056897408579,79.8981095810715,80.8905294212852,
81.8829492614988,82.8753691017124,83.867788941926,84.8230016469244),
 .UNSPECIFIED.);
#5845=B_SPLINE_CURVE_WITH_KNOTS('',3,(#40788,#40789,#40790,#40791,#40792,
#40793,#40794,#40795,#40796,#40797,#40798),.UNSPECIFIED.,.F.,.F.,(4,1,1,
1,1,1,1,1,4),(72.2566310325653,72.3965991153392,73.3890189555529,74.3814387957665,
75.3738586359801,76.3662784761938,77.3586983164074,78.351118156621,78.5398163397448),
 .UNSPECIFIED.);
#5846=B_SPLINE_CURVE_WITH_KNOTS('',3,(#40799,#40800,#40801,#40802,#40803,
#40804,#40805,#40806,#40807,#40808),.UNSPECIFIED.,.F.,.F.,(4,1,1,1,1,1,
1,4),(72.2566310325651,72.9511706995761,73.9435905397897,74.9360103800034,
75.928430220217,76.9208500604306,77.9132699006443,78.5398163397448),
 .UNSPECIFIED.);
#5847=B_SPLINE_CURVE_WITH_KNOTS('',3,(#40813,#40814,#40815,#40816,#40817,
#40818,#40819,#40820,#40821,#40822),.UNSPECIFIED.,.F.,.F.,(4,1,1,1,1,1,
1,4),(65.9734457253856,66.4420800740574,67.4344999142711,68.4269197544847,
69.4193395946983,70.411759434912,71.4041792751256,72.2566310325653),
 .UNSPECIFIED.);
#5848=B_SPLINE_CURVE_WITH_KNOTS('',3,(#40823,#40824,#40825,#40826,#40827,
#40828,#40829,#40830,#40831,#40832,#40833),.UNSPECIFIED.,.F.,.F.,(4,1,1,
1,1,1,1,1,4),(65.9734457253856,66.0042318180807,66.9966516582943,67.9890714985079,
68.9814913387216,69.9739111789352,70.9663310191488,71.9587508593625,72.2566310325651),
 .UNSPECIFIED.);
#5849=B_SPLINE_CURVE_WITH_KNOTS('',3,(#40838,#40839,#40840,#40841,#40842,
#40843,#40844,#40845,#40846,#40847),.UNSPECIFIED.,.F.,.F.,(4,1,1,1,1,1,
1,4),(59.690260418206,60.4875610327756,61.4799808729893,62.4724007132029,
63.4648205534165,64.4572403936302,65.4496602338438,65.9734457253856),
 .UNSPECIFIED.);
#5850=B_SPLINE_CURVE_WITH_KNOTS('',3,(#40848,#40849,#40850,#40851,#40852,
#40853,#40854,#40855,#40856,#40857),.UNSPECIFIED.,.F.,.F.,(4,1,1,1,1,1,
1,4),(59.690260418206,60.0497127767989,61.0421326170125,62.0345524572261,
63.0269722974398,64.0193921376534,65.011811977867,65.9734457253856),
 .UNSPECIFIED.);
#5851=B_SPLINE_CURVE_WITH_KNOTS('',3,(#40862,#40863,#40864,#40865,#40866,
#40867,#40868,#40869,#40870,#40871,#40872),.UNSPECIFIED.,.F.,.F.,(4,1,1,
1,1,1,1,1,4),(53.4070751110265,53.5406221512802,54.5330419914939,55.5254618317075,
56.5178816719211,57.5103015121348,58.5027213523484,59.495141192562,59.690260418206),
 .UNSPECIFIED.);
#5852=B_SPLINE_CURVE_WITH_KNOTS('',3,(#40873,#40874,#40875,#40876,#40877,
#40878,#40879,#40880,#40881,#40882),.UNSPECIFIED.,.F.,.F.,(4,1,1,1,1,1,
1,4),(53.4070751110265,54.0951937355171,55.0876135757307,56.0800334159443,
57.072453256158,58.0648730963716,59.0572929365852,59.690260418206),
 .UNSPECIFIED.);
#5853=B_SPLINE_CURVE_WITH_KNOTS('',3,(#40887,#40888,#40889,#40890,#40891,
#40892,#40893,#40894,#40895,#40896),.UNSPECIFIED.,.F.,.F.,(4,1,1,1,1,1,
1,4),(47.1238898038468,47.5861031099984,48.5785229502121,49.5709427904257,
50.5633626306393,51.555782470853,52.5482023110666,53.4070751110265),
 .UNSPECIFIED.);
#5854=B_SPLINE_CURVE_WITH_KNOTS('',3,(#40897,#40898,#40899,#40900,#40901,
#40902,#40903,#40904,#40905,#40906,#40907),.UNSPECIFIED.,.F.,.F.,(4,1,1,
1,1,1,1,1,4),(47.1238898038468,47.1482548540217,48.1406746942353,49.1330945344489,
50.1255143746626,51.1179342148762,52.1103540550898,53.1027738953035,53.4070751110265),
 .UNSPECIFIED.);
#5855=B_SPLINE_CURVE_WITH_KNOTS('',3,(#40912,#40913,#40914,#40915,#40916,
#40917,#40918,#40919,#40920,#40921),.UNSPECIFIED.,.F.,.F.,(4,1,1,1,1,1,
1,4),(40.8407044966672,41.6315840687166,42.6240039089303,43.6164237491439,
44.6088435893575,45.6012634295712,46.5936832697848,47.1238898038468),
 .UNSPECIFIED.);
#5856=B_SPLINE_CURVE_WITH_KNOTS('',3,(#40922,#40923,#40924,#40925,#40926,
#40927,#40928,#40929,#40930,#40931),.UNSPECIFIED.,.F.,.F.,(4,1,1,1,1,1,
1,4),(40.8407044966672,41.1937358127399,42.1861556529535,43.1785754931671,
44.1709953333808,45.1634151735944,46.155835013808,47.1238898038468),
 .UNSPECIFIED.);
#5857=B_SPLINE_CURVE_WITH_KNOTS('',3,(#40936,#40937,#40938,#40939,#40940,
#40941,#40942,#40943,#40944,#40945,#40946),.UNSPECIFIED.,.F.,.F.,(4,1,1,
1,1,1,1,1,4),(34.5575191894877,34.6846451872212,35.6770650274349,36.6694848676485,
37.6619047078621,38.6543245480758,39.6467443882894,40.639164228503,40.8407044966672),
 .UNSPECIFIED.);
#5858=B_SPLINE_CURVE_WITH_KNOTS('',3,(#40947,#40948,#40949,#40950,#40951,
#40952,#40953,#40954,#40955,#40956),.UNSPECIFIED.,.F.,.F.,(4,1,1,1,1,1,
1,4),(34.5575191894877,35.2392167714581,36.2316366116717,37.2240564518853,
38.216476292099,39.2088961323126,40.2013159725262,40.8407044966672),
 .UNSPECIFIED.);
#5859=B_SPLINE_CURVE_WITH_KNOTS('',3,(#40961,#40962,#40963,#40964,#40965,
#40966,#40967,#40968,#40969,#40970),.UNSPECIFIED.,.F.,.F.,(4,1,1,1,1,1,
1,4),(28.2743338823081,28.7301261459394,29.7225459861531,30.7149658263667,
31.7073856665803,32.699805506794,33.6922253470076,34.5575191894877),
 .UNSPECIFIED.);
#5860=B_SPLINE_CURVE_WITH_KNOTS('',3,(#40971,#40972,#40973,#40974,#40975,
#40976,#40977,#40978,#40979,#40980,#40981),.UNSPECIFIED.,.F.,.F.,(4,1,1,
1,1,1,1,1,4),(28.2743338823081,28.2922778899627,29.2846977301763,30.2771175703899,
31.2695374106036,32.2619572508172,33.2543770910308,34.2467969312444,34.5575191894877),
 .UNSPECIFIED.);
#5861=B_SPLINE_CURVE_WITH_KNOTS('',3,(#40986,#40987,#40988,#40989,#40990,
#40991,#40992,#40993,#40994,#40995),.UNSPECIFIED.,.F.,.F.,(4,1,1,1,1,1,
1,4),(21.9911485751285,22.7756071046577,23.7680269448713,24.7604467850849,
25.7528666252985,26.7452864655122,27.7377063057258,28.2743338823081),
 .UNSPECIFIED.);
#5862=B_SPLINE_CURVE_WITH_KNOTS('',3,(#40996,#40997,#40998,#40999,#41000,
#41001,#41002,#41003,#41004,#41005),.UNSPECIFIED.,.F.,.F.,(4,1,1,1,1,1,
1,4),(21.9911485751284,22.3377588486809,23.3301786888945,24.3225985291081,
25.3150183693218,26.3074382095354,27.299858049749,28.2743338823081),
 .UNSPECIFIED.);
#5863=B_SPLINE_CURVE_WITH_KNOTS('',3,(#41011,#41012,#41013,#41014,#41015),
 .UNSPECIFIED.,.F.,.F.,(4,1,4),(14.3984001269718,15.3908199671854,15.7079632679489),
 .UNSPECIFIED.);
#5864=B_SPLINE_CURVE_WITH_KNOTS('',3,(#41018,#41019,#41020,#41021,#41022),
 .UNSPECIFIED.,.F.,.F.,(4,1,4),(13.8759337553363,14.8362483829486,15.7079632679489),
 .UNSPECIFIED.);
#5865=B_SPLINE_CURVE_WITH_KNOTS('',3,(#41026,#41027,#41028,#41029,#41030,
#41031,#41032,#41033,#41034,#41035,#41036,#41037,#41038,#41039,#41040,#41041,
#41042,#41043),.UNSPECIFIED.,.F.,.F.,(4,2,2,2,2,2,2,2,4),(0.301357973509756,
0.376697466683881,0.452036959858006,0.527376453438759,0.602715947019511,
0.678055440600264,0.753394934181017,0.828734427355142,0.904073920529267),
 .UNSPECIFIED.);
#5866=B_SPLINE_CURVE_WITH_KNOTS('',3,(#41047,#41048,#41049,#41050,#41051,
#41052,#41053,#41054,#41055,#41056,#41057,#41058,#41059,#41060,#41061,#41062,
#41063,#41064,#41065,#41066,#41067,#41068,#41069,#41070,#41071,#41072),
 .UNSPECIFIED.,.F.,.F.,(4,2,2,2,2,2,2,2,2,2,2,2,4),(0.,0.0753399990358931,
0.150679998071786,0.226019996487856,0.301359994903926,0.376699993319996,
0.452039991736066,0.527379990771959,0.602719989807852,0.678059988843745,
0.753399987879638,0.828739986295708,0.904079984711778),.UNSPECIFIED.);
#5867=B_SPLINE_CURVE_WITH_KNOTS('',3,(#41073,#41074,#41075,#41076,#41077,
#41078,#41079,#41080,#41081,#41082),.UNSPECIFIED.,.F.,.F.,(4,2,2,2,4),(0.904079984711778,
0.979419983127848,1.05475998154392,1.13009998057981,1.2054399796157),
 .UNSPECIFIED.);
#5868=B_SPLINE_CURVE_WITH_KNOTS('',3,(#41083,#41084,#41085,#41086,#41087,
#41088,#41089,#41090,#41091,#41092,#41093,#41094,#41095,#41096,#41097,#41098,
#41099,#41100,#41101),.UNSPECIFIED.,.F.,.F.,(4,2,2,2,3,2,2,2,4),(0.904073920529267,
0.979413413703392,1.05475290687752,1.13009240045827,1.20543189403902,1.28077138761978,
1.35611088120053,1.43145037437465,1.50678986754878),.UNSPECIFIED.);
#5869=B_SPLINE_CURVE_WITH_KNOTS('',3,(#41105,#41106,#41107,#41108,#41109,
#41110,#41111,#41112,#41113,#41114,#41115,#41116,#41117,#41118,#41119,#41120,
#41121,#41122),.UNSPECIFIED.,.F.,.F.,(4,2,2,2,2,2,2,2,4),(0.301357973509756,
0.376697466683881,0.452036959858006,0.527376453438759,0.602715947019511,
0.678055440600264,0.753394934181017,0.828734427355142,0.904073920529267),
 .UNSPECIFIED.);
#5870=B_SPLINE_CURVE_WITH_KNOTS('',3,(#41123,#41124,#41125,#41126,#41127,
#41128,#41129,#41130,#41131,#41132,#41133,#41134,#41135,#41136,#41137,#41138,
#41139,#41140,#41141),.UNSPECIFIED.,.F.,.F.,(4,2,2,2,3,2,2,2,4),(0.904073920529267,
0.979413413703392,1.05475290687752,1.13009240045827,1.20543189403902,1.28077138761978,
1.35611088120053,1.43145037437465,1.50678986754878),.UNSPECIFIED.);
#5871=B_SPLINE_CURVE_WITH_KNOTS('',3,(#41145,#41146,#41147,#41148,#41149,
#41150,#41151,#41152,#41153,#41154),.UNSPECIFIED.,.F.,.F.,(4,2,2,2,4),(0.,
0.0753399990358931,0.150679998071786,0.226019996487856,0.301359994903926),
 .UNSPECIFIED.);
#5872=B_SPLINE_CURVE_WITH_KNOTS('',3,(#41155,#41156,#41157,#41158,#41159,
#41160,#41161,#41162,#41163,#41164,#41165,#41166,#41167,#41168,#41169,#41170,
#41171,#41172,#41173,#41174,#41175,#41176,#41177,#41178,#41179,#41180),
 .UNSPECIFIED.,.F.,.F.,(4,2,2,2,2,2,2,2,2,2,2,2,4),(0.301359994903926,0.376699993319996,
0.452039991736066,0.527379990771959,0.602719989807852,0.678059988843745,
0.753399987879638,0.828739986295708,0.904079984711778,0.979419983127848,
1.05475998154392,1.13009998057981,1.2054399796157),.UNSPECIFIED.);
#5873=B_SPLINE_CURVE_WITH_KNOTS('',3,(#41184,#41185,#41186,#41187,#41188,
#41189,#41190,#41191,#41192,#41193,#41194,#41195,#41196,#41197,#41198,#41199,
#41200,#41201),.UNSPECIFIED.,.F.,.F.,(4,2,2,2,2,2,2,2,4),(0.301357973509756,
0.376697466683881,0.452036959858006,0.527376453438759,0.602715947019511,
0.678055440600264,0.753394934181017,0.828734427355142,0.904073920529267),
 .UNSPECIFIED.);
#5874=B_SPLINE_CURVE_WITH_KNOTS('',3,(#41203,#41204,#41205,#41206,#41207,
#41208,#41209,#41210,#41211,#41212),.UNSPECIFIED.,.F.,.F.,(4,2,2,2,4),(1.20543189403902,
1.28077138761978,1.35611088120053,1.43145037437465,1.50678986754878),
 .UNSPECIFIED.);
#5875=B_SPLINE_CURVE_WITH_KNOTS('',3,(#41216,#41217,#41218,#41219,#41220,
#41221,#41222,#41223,#41224,#41225),.UNSPECIFIED.,.F.,.F.,(4,2,2,2,4),(0.904079984711778,
0.979419983127848,1.05475998154392,1.13009998057981,1.2054399796157),
 .UNSPECIFIED.);
#5876=B_SPLINE_CURVE_WITH_KNOTS('',3,(#41227,#41228,#41229,#41230,#41231,
#41232,#41233,#41234,#41235,#41236,#41237,#41238,#41239,#41240,#41241,#41242,
#41243,#41244),.UNSPECIFIED.,.F.,.F.,(4,2,2,2,2,2,2,2,4),(0.301359994903926,
0.376699993319996,0.452039991736066,0.527379990771959,0.602719989807852,
0.678059988843745,0.753399987879638,0.828739986295708,0.904079984711778),
 .UNSPECIFIED.);
#5877=B_SPLINE_CURVE_WITH_KNOTS('',3,(#41245,#41246,#41247,#41248,#41249,
#41250,#41251,#41252,#41253,#41254),.UNSPECIFIED.,.F.,.F.,(4,2,2,2,4),(0.,
0.0753399990358931,0.150679998071786,0.226019996487856,0.301359994903926),
 .UNSPECIFIED.);
#5878=B_SPLINE_CURVE_WITH_KNOTS('',3,(#41255,#41256,#41257,#41258,#41259,
#41260,#41261,#41262,#41263,#41264),.UNSPECIFIED.,.F.,.F.,(4,2,2,2,4),(0.904073920529267,
0.979413413703392,1.05475290687752,1.13009240045827,1.20543189403902),
 .UNSPECIFIED.);
#5879=B_SPLINE_CURVE_WITH_KNOTS('',3,(#41268,#41269,#41270,#41271,#41272,
#41273,#41274,#41275,#41276,#41277,#41278,#41279,#41280,#41281,#41282,#41283,
#41284,#41285),.UNSPECIFIED.,.F.,.F.,(4,2,2,2,2,2,2,2,4),(0.301357973509756,
0.376697466683881,0.452036959858006,0.527376453438759,0.602715947019511,
0.678055440600264,0.753394934181017,0.828734427355142,0.904073920529267),
 .UNSPECIFIED.);
#5880=B_SPLINE_CURVE_WITH_KNOTS('',3,(#41287,#41288,#41289,#41290,#41291,
#41292,#41293,#41294,#41295,#41296),.UNSPECIFIED.,.F.,.F.,(4,2,2,2,4),(1.20543189403902,
1.28077138761978,1.35611088120053,1.43145037437465,1.50678986754878),
 .UNSPECIFIED.);
#5881=B_SPLINE_CURVE_WITH_KNOTS('',3,(#41299,#41300,#41301,#41302,#41303,
#41304,#41305,#41306,#41307,#41308,#41309,#41310,#41311,#41312,#41313,#41314,
#41315,#41316,#41317,#41318,#41319,#41320,#41321,#41322,#41323,#41324,#41325,
#41326,#41327,#41328,#41329,#41330,#41331,#41332),.UNSPECIFIED.,.T.,.F.,
(4,2,2,2,2,2,2,2,2,2,2,2,2,2,2,2,4),(0.,0.0753399990358931,0.150679998071786,
0.226019996487856,0.301359994903926,0.376699993319996,0.452039991736066,
0.527379990771959,0.602719989807852,0.678059988843745,0.753399987879638,
0.828739986295708,0.904079984711778,0.979419983127848,1.05475998154392,
1.13009998057981,1.2054399796157),.UNSPECIFIED.);
#5882=B_SPLINE_CURVE_WITH_KNOTS('',3,(#41333,#41334,#41335,#41336,#41337,
#41338,#41339,#41340,#41341,#41342),.UNSPECIFIED.,.F.,.F.,(4,2,2,2,4),(0.904073920529267,
0.979413413703392,1.05475290687752,1.13009240045827,1.20543189403902),
 .UNSPECIFIED.);
#5883=B_SPLINE_CURVE_WITH_KNOTS('',3,(#41346,#41347,#41348,#41349,#41350,
#41351,#41352,#41353,#41354,#41355,#41356,#41357,#41358,#41359,#41360,#41361,
#41362,#41363),.UNSPECIFIED.,.F.,.F.,(4,2,2,2,2,2,2,2,4),(0.301357973509756,
0.376697466683881,0.452036959858007,0.52737645343876,0.602715947019512,
0.678055440600265,0.753394934181018,0.828734427355143,0.904073920529268),
 .UNSPECIFIED.);
#5884=B_SPLINE_CURVE_WITH_KNOTS('',3,(#41367,#41368,#41369,#41370,#41371,
#41372,#41373,#41374,#41375,#41376,#41377,#41378,#41379,#41380,#41381,#41382,
#41383,#41384,#41385,#41386,#41387,#41388,#41389,#41390,#41391,#41392),
 .UNSPECIFIED.,.F.,.F.,(4,2,2,2,2,2,2,2,2,2,2,2,4),(0.,0.0753399990358932,
0.150679998071786,0.226019996487856,0.301359994903927,0.376699993319997,
0.452039991736067,0.52737999077196,0.602719989807853,0.678059988843746,
0.753399987879639,0.828739986295709,0.90407998471178),.UNSPECIFIED.);
#5885=B_SPLINE_CURVE_WITH_KNOTS('',3,(#41393,#41394,#41395,#41396,#41397,
#41398,#41399,#41400,#41401,#41402),.UNSPECIFIED.,.F.,.F.,(4,2,2,2,4),(0.90407998471178,
0.97941998312785,1.05475998154392,1.13009998057981,1.20543997961571),
 .UNSPECIFIED.);
#5886=B_SPLINE_CURVE_WITH_KNOTS('',3,(#41403,#41404,#41405,#41406,#41407,
#41408,#41409,#41410,#41411,#41412,#41413,#41414,#41415,#41416,#41417,#41418,
#41419,#41420,#41421),.UNSPECIFIED.,.F.,.F.,(4,2,2,2,3,2,2,2,4),(0.904073920529268,
0.979413413703393,1.05475290687752,1.13009240045827,1.20543189403902,1.28077138761978,
1.35611088120053,1.43145037437465,1.50678986754878),.UNSPECIFIED.);
#5887=B_SPLINE_CURVE_WITH_KNOTS('',3,(#41425,#41426,#41427,#41428,#41429,
#41430,#41431,#41432,#41433,#41434,#41435,#41436,#41437,#41438,#41439,#41440,
#41441,#41442),.UNSPECIFIED.,.F.,.F.,(4,2,2,2,2,2,2,2,4),(0.301357973509756,
0.376697466683882,0.452036959858007,0.52737645343876,0.602715947019512,
0.678055440600265,0.753394934181018,0.828734427355143,0.904073920529268),
 .UNSPECIFIED.);
#5888=B_SPLINE_CURVE_WITH_KNOTS('',3,(#41443,#41444,#41445,#41446,#41447,
#41448,#41449,#41450,#41451,#41452,#41453,#41454,#41455,#41456,#41457,#41458,
#41459,#41460,#41461),.UNSPECIFIED.,.F.,.F.,(4,2,2,2,3,2,2,2,4),(0.904073920529268,
0.979413413703394,1.05475290687752,1.13009240045827,1.20543189403902,1.28077138761978,
1.35611088120053,1.43145037437466,1.50678986754878),.UNSPECIFIED.);
#5889=B_SPLINE_CURVE_WITH_KNOTS('',3,(#41465,#41466,#41467,#41468,#41469,
#41470,#41471,#41472,#41473,#41474),.UNSPECIFIED.,.F.,.F.,(4,2,2,2,4),(0.,
0.0753399990358932,0.150679998071786,0.226019996487856,0.301359994903927),
 .UNSPECIFIED.);
#5890=B_SPLINE_CURVE_WITH_KNOTS('',3,(#41475,#41476,#41477,#41478,#41479,
#41480,#41481,#41482,#41483,#41484,#41485,#41486,#41487,#41488,#41489,#41490,
#41491,#41492,#41493,#41494,#41495,#41496,#41497,#41498,#41499,#41500),
 .UNSPECIFIED.,.F.,.F.,(4,2,2,2,2,2,2,2,2,2,2,2,4),(0.301359994903927,0.376699993319997,
0.452039991736067,0.52737999077196,0.602719989807853,0.678059988843746,
0.75339998787964,0.82873998629571,0.90407998471178,0.97941998312785,1.05475998154392,
1.13009998057981,1.20543997961571),.UNSPECIFIED.);
#5891=B_SPLINE_CURVE_WITH_KNOTS('',3,(#41504,#41505,#41506,#41507,#41508,
#41509,#41510,#41511,#41512,#41513,#41514,#41515,#41516,#41517,#41518,#41519,
#41520,#41521),.UNSPECIFIED.,.F.,.F.,(4,2,2,2,2,2,2,2,4),(0.301357973509756,
0.376697466683882,0.452036959858007,0.52737645343876,0.602715947019512,
0.678055440600265,0.753394934181018,0.828734427355143,0.904073920529268),
 .UNSPECIFIED.);
#5892=B_SPLINE_CURVE_WITH_KNOTS('',3,(#41523,#41524,#41525,#41526,#41527,
#41528,#41529,#41530,#41531,#41532),.UNSPECIFIED.,.F.,.F.,(4,2,2,2,4),(1.20543189403902,
1.28077138761978,1.35611088120053,1.43145037437466,1.50678986754878),
 .UNSPECIFIED.);
#5893=B_SPLINE_CURVE_WITH_KNOTS('',3,(#41536,#41537,#41538,#41539,#41540,
#41541,#41542,#41543,#41544,#41545),.UNSPECIFIED.,.F.,.F.,(4,2,2,2,4),(0.90407998471178,
0.97941998312785,1.05475998154392,1.13009998057981,1.20543997961571),
 .UNSPECIFIED.);
#5894=B_SPLINE_CURVE_WITH_KNOTS('',3,(#41547,#41548,#41549,#41550,#41551,
#41552,#41553,#41554,#41555,#41556,#41557,#41558,#41559,#41560,#41561,#41562,
#41563,#41564),.UNSPECIFIED.,.F.,.F.,(4,2,2,2,2,2,2,2,4),(0.301359994903927,
0.376699993319997,0.452039991736067,0.52737999077196,0.602719989807853,
0.678059988843746,0.753399987879639,0.828739986295709,0.90407998471178),
 .UNSPECIFIED.);
#5895=B_SPLINE_CURVE_WITH_KNOTS('',3,(#41565,#41566,#41567,#41568,#41569,
#41570,#41571,#41572,#41573,#41574),.UNSPECIFIED.,.F.,.F.,(4,2,2,2,4),(0.,
0.0753399990358932,0.150679998071786,0.226019996487856,0.301359994903927),
 .UNSPECIFIED.);
#5896=B_SPLINE_CURVE_WITH_KNOTS('',3,(#41575,#41576,#41577,#41578,#41579,
#41580,#41581,#41582,#41583,#41584),.UNSPECIFIED.,.F.,.F.,(4,2,2,2,4),(0.904073920529268,
0.979413413703393,1.05475290687752,1.13009240045827,1.20543189403902),
 .UNSPECIFIED.);
#5897=B_SPLINE_CURVE_WITH_KNOTS('',3,(#41588,#41589,#41590,#41591,#41592,
#41593,#41594,#41595,#41596,#41597,#41598,#41599,#41600,#41601,#41602,#41603,
#41604,#41605),.UNSPECIFIED.,.F.,.F.,(4,2,2,2,2,2,2,2,4),(0.301357973509756,
0.376697466683882,0.452036959858007,0.52737645343876,0.602715947019512,
0.678055440600265,0.753394934181018,0.828734427355143,0.904073920529268),
 .UNSPECIFIED.);
#5898=B_SPLINE_CURVE_WITH_KNOTS('',3,(#41607,#41608,#41609,#41610,#41611,
#41612,#41613,#41614,#41615,#41616),.UNSPECIFIED.,.F.,.F.,(4,2,2,2,4),(1.20543189403902,
1.28077138761978,1.35611088120053,1.43145037437466,1.50678986754878),
 .UNSPECIFIED.);
#5899=B_SPLINE_CURVE_WITH_KNOTS('',3,(#41619,#41620,#41621,#41622,#41623,
#41624,#41625,#41626,#41627,#41628,#41629,#41630,#41631,#41632,#41633,#41634,
#41635,#41636,#41637,#41638,#41639,#41640,#41641,#41642,#41643,#41644,#41645,
#41646,#41647,#41648,#41649,#41650,#41651,#41652),.UNSPECIFIED.,.T.,.F.,
(4,2,2,2,2,2,2,2,2,2,2,2,2,2,2,2,4),(0.,0.0753399990358932,0.150679998071786,
0.226019996487856,0.301359994903927,0.376699993319997,0.452039991736067,
0.52737999077196,0.602719989807853,0.678059988843746,0.753399987879639,
0.828739986295709,0.90407998471178,0.97941998312785,1.05475998154392,1.13009998057981,
1.20543997961571),.UNSPECIFIED.);
#5900=B_SPLINE_CURVE_WITH_KNOTS('',3,(#41653,#41654,#41655,#41656,#41657,
#41658,#41659,#41660,#41661,#41662),.UNSPECIFIED.,.F.,.F.,(4,2,2,2,4),(0.904073920529268,
0.979413413703393,1.05475290687752,1.13009240045827,1.20543189403902),
 .UNSPECIFIED.);
#5901=B_SPLINE_CURVE_WITH_KNOTS('',3,(#41666,#41667,#41668,#41669,#41670,
#41671,#41672,#41673,#41674,#41675,#41676,#41677,#41678,#41679,#41680,#41681,
#41682,#41683),.UNSPECIFIED.,.F.,.F.,(4,2,2,2,2,2,2,2,4),(0.301357973509755,
0.37669746668388,0.452036959858005,0.527376453438758,0.602715947019511,
0.678055440600264,0.753394934181017,0.828734427355142,0.904073920529267),
 .UNSPECIFIED.);
#5902=B_SPLINE_CURVE_WITH_KNOTS('',3,(#41687,#41688,#41689,#41690,#41691,
#41692,#41693,#41694,#41695,#41696,#41697,#41698,#41699,#41700,#41701,#41702,
#41703,#41704,#41705,#41706,#41707,#41708,#41709,#41710,#41711,#41712),
 .UNSPECIFIED.,.F.,.F.,(4,2,2,2,2,2,2,2,2,2,2,2,4),(0.,0.0753399990358932,
0.150679998071786,0.226019996487857,0.301359994903927,0.376699993319997,
0.452039991736067,0.52737999077196,0.602719989807853,0.678059988843747,
0.75339998787964,0.828739986295709,0.904079984711779),.UNSPECIFIED.);
#5903=B_SPLINE_CURVE_WITH_KNOTS('',3,(#41713,#41714,#41715,#41716,#41717,
#41718,#41719,#41720,#41721,#41722),.UNSPECIFIED.,.F.,.F.,(4,2,2,2,4),(0.904079984711779,
0.979419983127849,1.05475998154392,1.13009998057981,1.20543997961571),
 .UNSPECIFIED.);
#5904=B_SPLINE_CURVE_WITH_KNOTS('',3,(#41723,#41724,#41725,#41726,#41727,
#41728,#41729,#41730,#41731,#41732,#41733,#41734,#41735,#41736,#41737,#41738,
#41739,#41740,#41741),.UNSPECIFIED.,.F.,.F.,(4,2,2,2,3,2,2,2,4),(0.904073920529267,
0.979413413703393,1.05475290687752,1.13009240045827,1.20543189403902,1.28077138761978,
1.35611088120053,1.43145037437465,1.50678986754878),.UNSPECIFIED.);
#5905=B_SPLINE_CURVE_WITH_KNOTS('',3,(#41745,#41746,#41747,#41748,#41749,
#41750,#41751,#41752,#41753,#41754,#41755,#41756,#41757,#41758,#41759,#41760,
#41761,#41762),.UNSPECIFIED.,.F.,.F.,(4,2,2,2,2,2,2,2,4),(0.301357973509756,
0.37669746668388,0.452036959858006,0.527376453438758,0.602715947019511,
0.678055440600264,0.753394934181016,0.828734427355142,0.904073920529267),
 .UNSPECIFIED.);
#5906=B_SPLINE_CURVE_WITH_KNOTS('',3,(#41763,#41764,#41765,#41766,#41767,
#41768,#41769,#41770,#41771,#41772,#41773,#41774,#41775,#41776,#41777,#41778,
#41779,#41780,#41781),.UNSPECIFIED.,.F.,.F.,(4,2,2,2,3,2,2,2,4),(0.904073920529267,
0.979413413703393,1.05475290687752,1.13009240045827,1.20543189403902,1.28077138761978,
1.35611088120053,1.43145037437465,1.50678986754878),.UNSPECIFIED.);
#5907=B_SPLINE_CURVE_WITH_KNOTS('',3,(#41785,#41786,#41787,#41788,#41789,
#41790,#41791,#41792,#41793,#41794),.UNSPECIFIED.,.F.,.F.,(4,2,2,2,4),(0.,
0.0753399990358931,0.150679998071786,0.226019996487856,0.301359994903927),
 .UNSPECIFIED.);
#5908=B_SPLINE_CURVE_WITH_KNOTS('',3,(#41795,#41796,#41797,#41798,#41799,
#41800,#41801,#41802,#41803,#41804,#41805,#41806,#41807,#41808,#41809,#41810,
#41811,#41812,#41813,#41814,#41815,#41816,#41817,#41818,#41819,#41820),
 .UNSPECIFIED.,.F.,.F.,(4,2,2,2,2,2,2,2,2,2,2,2,4),(0.301359994903927,0.376699993319997,
0.452039991736067,0.52737999077196,0.602719989807853,0.678059988843746,
0.75339998787964,0.828739986295709,0.904079984711779,0.979419983127849,
1.05475998154392,1.13009998057981,1.2054399796157),.UNSPECIFIED.);
#5909=B_SPLINE_CURVE_WITH_KNOTS('',3,(#41824,#41825,#41826,#41827,#41828,
#41829,#41830,#41831,#41832,#41833,#41834,#41835,#41836,#41837,#41838,#41839,
#41840,#41841),.UNSPECIFIED.,.F.,.F.,(4,2,2,2,2,2,2,2,4),(0.301357973509755,
0.37669746668388,0.452036959858005,0.527376453438758,0.602715947019511,
0.678055440600264,0.753394934181016,0.828734427355142,0.904073920529267),
 .UNSPECIFIED.);
#5910=B_SPLINE_CURVE_WITH_KNOTS('',3,(#41843,#41844,#41845,#41846,#41847,
#41848,#41849,#41850,#41851,#41852),.UNSPECIFIED.,.F.,.F.,(4,2,2,2,4),(1.20543189403902,
1.28077138761978,1.35611088120053,1.43145037437465,1.50678986754878),
 .UNSPECIFIED.);
#5911=B_SPLINE_CURVE_WITH_KNOTS('',3,(#41856,#41857,#41858,#41859,#41860,
#41861,#41862,#41863,#41864,#41865),.UNSPECIFIED.,.F.,.F.,(4,2,2,2,4),(0.904079984711779,
0.979419983127849,1.05475998154392,1.13009998057981,1.2054399796157),
 .UNSPECIFIED.);
#5912=B_SPLINE_CURVE_WITH_KNOTS('',3,(#41867,#41868,#41869,#41870,#41871,
#41872,#41873,#41874,#41875,#41876,#41877,#41878,#41879,#41880,#41881,#41882,
#41883,#41884),.UNSPECIFIED.,.F.,.F.,(4,2,2,2,2,2,2,2,4),(0.301359994903927,
0.376699993319997,0.452039991736067,0.52737999077196,0.602719989807853,
0.678059988843746,0.75339998787964,0.828739986295709,0.904079984711779),
 .UNSPECIFIED.);
#5913=B_SPLINE_CURVE_WITH_KNOTS('',3,(#41885,#41886,#41887,#41888,#41889,
#41890,#41891,#41892,#41893,#41894),.UNSPECIFIED.,.F.,.F.,(4,2,2,2,4),(0.,
0.0753399990358931,0.150679998071786,0.226019996487856,0.301359994903927),
 .UNSPECIFIED.);
#5914=B_SPLINE_CURVE_WITH_KNOTS('',3,(#41895,#41896,#41897,#41898,#41899,
#41900,#41901,#41902,#41903,#41904),.UNSPECIFIED.,.F.,.F.,(4,2,2,2,4),(0.904073920529267,
0.979413413703393,1.05475290687752,1.13009240045827,1.20543189403902),
 .UNSPECIFIED.);
#5915=B_SPLINE_CURVE_WITH_KNOTS('',3,(#41908,#41909,#41910,#41911,#41912,
#41913,#41914,#41915,#41916,#41917,#41918,#41919,#41920,#41921,#41922,#41923,
#41924,#41925),.UNSPECIFIED.,.F.,.F.,(4,2,2,2,2,2,2,2,4),(0.301357973509755,
0.37669746668388,0.452036959858005,0.527376453438758,0.602715947019511,
0.678055440600264,0.753394934181016,0.828734427355142,0.904073920529267),
 .UNSPECIFIED.);
#5916=B_SPLINE_CURVE_WITH_KNOTS('',3,(#41927,#41928,#41929,#41930,#41931,
#41932,#41933,#41934,#41935,#41936),.UNSPECIFIED.,.F.,.F.,(4,2,2,2,4),(1.20543189403902,
1.28077138761978,1.35611088120053,1.43145037437465,1.50678986754878),
 .UNSPECIFIED.);
#5917=B_SPLINE_CURVE_WITH_KNOTS('',3,(#41939,#41940,#41941,#41942,#41943,
#41944,#41945,#41946,#41947,#41948,#41949,#41950,#41951,#41952,#41953,#41954,
#41955,#41956,#41957,#41958,#41959,#41960,#41961,#41962,#41963,#41964,#41965,
#41966,#41967,#41968,#41969,#41970,#41971,#41972),.UNSPECIFIED.,.T.,.F.,
(4,2,2,2,2,2,2,2,2,2,2,2,2,2,2,2,4),(0.,0.0753399990358931,0.150679998071786,
0.226019996487856,0.301359994903927,0.376699993319997,0.452039991736067,
0.52737999077196,0.602719989807853,0.678059988843746,0.75339998787964,0.828739986295709,
0.904079984711779,0.979419983127849,1.05475998154392,1.13009998057981,1.2054399796157),
 .UNSPECIFIED.);
#5918=B_SPLINE_CURVE_WITH_KNOTS('',3,(#41973,#41974,#41975,#41976,#41977,
#41978,#41979,#41980,#41981,#41982),.UNSPECIFIED.,.F.,.F.,(4,2,2,2,4),(0.904073920529267,
0.979413413703393,1.05475290687752,1.13009240045827,1.20543189403902),
 .UNSPECIFIED.);
#5919=B_SPLINE_CURVE_WITH_KNOTS('',3,(#41984,#41985,#41986,#41987,#41988,
#41989,#41990,#41991,#41992,#41993,#41994,#41995,#41996,#41997,#41998,#41999,
#42000,#42001,#42002,#42003,#42004,#42005,#42006,#42007,#42008,#42009,#42010,
#42011,#42012,#42013,#42014,#42015,#42016,#42017,#42018,#42019,#42020,#42021,
#42022,#42023,#42024,#42025,#42026,#42027,#42028,#42029,#42030,#42031,#42032,
#42033,#42034,#42035,#42036,#42037,#42038,#42039,#42040,#42041,#42042,#42043,
#42044,#42045,#42046,#42047,#42048,#42049,#42050,#42051,#42052,#42053,#42054,
#42055,#42056,#42057,#42058,#42059,#42060,#42061,#42062,#42063,#42064,#42065,
#42066,#42067,#42068,#42069,#42070,#42071,#42072,#42073,#42074,#42075,#42076,
#42077,#42078,#42079,#42080),.UNSPECIFIED.,.F.,.F.,(4,3,3,3,3,3,3,3,3,3,
3,3,3,3,3,3,3,3,3,3,3,3,3,3,3,3,3,3,3,3,3,3,4),(-0.569248610399337,-0.543574665913807,
-0.51727245328848,-0.510408802663154,-0.504800523775832,-0.47773970928715,
-0.455902642111078,-0.447185941747197,-0.442501781607008,-0.414772156692359,
-0.386610546537412,-0.358667936434586,-0.344761745295583,-0.340663182606779,
-0.336259776461384,-0.307329116975324,-0.303043171878573,-0.27522662276973,
-0.246781267954678,-0.236972518199776,-0.232129158585461,-0.228298533654497,
-0.199315149767015,-0.169756960554979,-0.139958455388845,-0.123701275093121,
-0.118725825268248,-0.114410875368034,-0.0838707291780127,-0.053291589117924,
-0.0233203534222033,-0.00990101302305402,0.),.UNSPECIFIED.);
#5920=B_SPLINE_CURVE_WITH_KNOTS('',3,(#42081,#42082,#42083,#42084,#42085,
#42086,#42087,#42088,#42089,#42090,#42091,#42092,#42093,#42094,#42095,#42096,
#42097,#42098,#42099,#42100,#42101,#42102,#42103,#42104,#42105,#42106,#42107,
#42108,#42109,#42110,#42111,#42112,#42113,#42114,#42115,#42116,#42117,#42118,
#42119,#42120,#42121,#42122,#42123,#42124,#42125,#42126,#42127,#42128,#42129,
#42130,#42131,#42132,#42133,#42134,#42135,#42136,#42137,#42138,#42139,#42140,
#42141,#42142,#42143,#42144,#42145,#42146,#42147,#42148,#42149,#42150,#42151,
#42152,#42153,#42154,#42155,#42156,#42157,#42158,#42159,#42160,#42161,#42162,
#42163,#42164,#42165,#42166,#42167,#42168,#42169,#42170,#42171,#42172,#42173,
#42174),.UNSPECIFIED.,.F.,.F.,(4,3,3,3,3,3,3,3,3,3,3,3,3,3,3,3,3,3,3,3,
3,3,3,3,3,3,3,3,3,3,3,4),(-0.56684730604813,-0.536665862167618,-0.506059953422707,
-0.497416406503416,-0.490479621633712,-0.460332810122765,-0.437094434682836,
-0.424724933789942,-0.420483367383437,-0.391058514880852,-0.361900337811473,
-0.333575724283842,-0.318788244863715,-0.31312587650193,-0.30869595256902,
-0.280705563216954,-0.274425806603334,-0.245949103512894,-0.216224273057835,
-0.204597316409418,-0.200878698435462,-0.17304519623036,-0.145277260413139,
-0.117980535703011,-0.104251776224188,-0.100006100346348,-0.0958284117611523,
-0.0691557510127404,-0.0429305470424711,-0.0175053685333362,-0.00815045987242433,
0.),.UNSPECIFIED.);
#5921=B_SPLINE_CURVE_WITH_KNOTS('',3,(#42176,#42177,#42178,#42179,#42180,
#42181,#42182,#42183,#42184,#42185,#42186),.UNSPECIFIED.,.F.,.F.,(4,1,1,
1,1,1,1,1,4),(15.7079632679489,15.8286682231622,16.8210880633759,17.8135079035895,
18.8059277438031,19.7983475840168,20.7907674242304,21.783187264444,21.9911485751285),
 .UNSPECIFIED.);
#5922=B_SPLINE_CURVE_WITH_KNOTS('',3,(#42187,#42188,#42189,#42190,#42191,
#42192,#42193,#42194,#42195,#42196),.UNSPECIFIED.,.F.,.F.,(4,1,1,1,1,1,
1,4),(15.7079632679489,16.3832398073991,17.3756596476127,18.3680794878263,
19.36049932804,20.3529191682536,21.3453390084672,21.9911485751284),
 .UNSPECIFIED.);
#5923=B_SPLINE_CURVE_WITH_KNOTS('',3,(#42597,#42598,#42599,#42600,#42601,
#42602,#42603,#42604,#42605,#42606,#42607,#42608,#42609,#42610,#42611,#42612,
#42613,#42614,#42615,#42616,#42617,#42618,#42619,#42620,#42621,#42622,#42623,
#42624,#42625,#42626,#42627,#42628,#42629,#42630,#42631,#42632,#42633,#42634,
#42635,#42636,#42637,#42638,#42639,#42640,#42641,#42642,#42643,#42644,#42645,
#42646,#42647,#42648,#42649,#42650,#42651,#42652,#42653,#42654,#42655,#42656,
#42657,#42658,#42659,#42660,#42661,#42662,#42663,#42664,#42665,#42666,#42667,
#42668,#42669,#42670,#42671,#42672,#42673,#42674,#42675,#42676,#42677,#42678,
#42679,#42680,#42681,#42682,#42683,#42684,#42685,#42686,#42687,#42688,#42689,
#42690),.UNSPECIFIED.,.F.,.F.,(4,3,3,3,3,3,3,3,3,3,3,3,3,3,3,3,3,3,3,3,
3,3,3,3,3,3,3,3,3,3,3,4),(0.,0.0253630259498556,0.0513976226489003,0.0781462280587279,
0.0899194383258336,0.0966315939993256,0.102678021611066,0.129978487836714,
0.157730214206848,0.184644277137016,0.19593207222776,0.203012844728639,
0.207156655375447,0.236271560651484,0.265386465927521,0.293279271834908,
0.302554877553506,0.311292566193412,0.315704524166816,0.343817419217604,
0.372959123929891,0.402412672778624,0.4133424655252,0.422898831534667,0.428117874468216,
0.458184918270041,0.482885311859882,0.492048607646526,0.498170307491992,
0.528680781133954,0.556986492629404,0.566847306048082),.UNSPECIFIED.);
#5924=B_SPLINE_CURVE_WITH_KNOTS('',3,(#42691,#42692,#42693,#42694,#42695,
#42696,#42697,#42698,#42699,#42700,#42701,#42702,#42703,#42704,#42705,#42706,
#42707,#42708,#42709,#42710,#42711,#42712,#42713,#42714,#42715),
 .UNSPECIFIED.,.F.,.F.,(4,3,3,3,3,3,3,3,4),(-10.1321597128208,-9.92419840213631,
-8.93177856192268,-7.93935872170905,-6.94693888149542,-5.95451904128179,
-4.96209920106816,-3.96967936085453,-3.84897440564112),.UNSPECIFIED.);
#5925=B_SPLINE_CURVE_WITH_KNOTS('',3,(#43116,#43117,#43118,#43119,#43120,
#43121,#43122,#43123,#43124,#43125,#43126,#43127,#43128,#43129,#43130,#43131,
#43132,#43133,#43134,#43135,#43136,#43137),.UNSPECIFIED.,.F.,.F.,(4,3,3,
3,3,3,3,4),(7.59274844815659,7.93935872170906,8.93177856192269,9.92419840213632,
10.9166182423499,11.9090380825636,12.9014579227772,13.8759337553361),
 .UNSPECIFIED.);
#5926=B_SPLINE_CURVE_WITH_KNOTS('',3,(#43138,#43139,#43140,#43141,#43142,
#43143,#43144,#43145,#43146,#43147,#43148,#43149,#43150,#43151,#43152,#43153,
#43154,#43155,#43156,#43157,#43158,#43159,#43160,#43161,#43162,#43163,#43164,
#43165,#43166,#43167,#43168,#43169,#43170,#43171,#43172,#43173,#43174,#43175,
#43176,#43177,#43178,#43179,#43180,#43181,#43182,#43183,#43184,#43185,#43186,
#43187,#43188,#43189,#43190,#43191,#43192,#43193,#43194,#43195,#43196,#43197,
#43198,#43199,#43200,#43201,#43202,#43203,#43204,#43205,#43206,#43207,#43208,
#43209,#43210,#43211,#43212,#43213,#43214,#43215,#43216,#43217,#43218,#43219,
#43220,#43221,#43222,#43223,#43224,#43225,#43226,#43227,#43228),
 .UNSPECIFIED.,.F.,.F.,(4,3,3,3,3,3,3,3,3,3,3,3,3,3,3,3,3,3,3,3,3,3,3,3,
3,3,3,3,3,3,4),(0.,0.0297240839684256,0.0601072325498447,0.0893395071893512,
0.114917747498919,0.120626859687113,0.150385989363053,0.179981400050151,
0.208477407454087,0.22042950374967,0.228738548914548,0.234134417006902,
0.264049923336399,0.291955958271147,0.293965429665896,0.322911496990148,
0.339206044994607,0.343413985005071,0.37150622848317,0.399645181299159,
0.427381812169266,0.437705393072651,0.444698500366259,0.448877446518554,
0.476925760110501,0.497961995304462,0.506030983450329,0.511791121632976,
0.537728941220283,0.561070700886344,0.569248610399446),.UNSPECIFIED.);
#5927=B_SPLINE_CURVE_WITH_KNOTS('',3,(#43231,#43232,#43233,#43234,#43235,
#43236,#43237,#43238,#43239,#43240,#43241,#43242,#43243,#43244,#43245,#43246,
#43247,#43248,#43249,#43250,#43251,#43252,#43253,#43254,#43255,#43256,#43257,
#43258,#43259,#43260,#43261,#43262,#43263,#43264,#43265,#43266,#43267,#43268,
#43269,#43270,#43271,#43272,#43273,#43274,#43275,#43276,#43277,#43278,#43279,
#43280,#43281,#43282,#43283,#43284,#43285,#43286,#43287,#43288,#43289,#43290,
#43291,#43292,#43293,#43294,#43295,#43296,#43297,#43298,#43299,#43300,#43301,
#43302,#43303,#43304,#43305,#43306,#43307,#43308,#43309,#43310,#43311,#43312,
#43313,#43314,#43315,#43316,#43317,#43318,#43319,#43320,#43321,#43322,#43323,
#43324,#43325,#43326,#43327),.UNSPECIFIED.,.F.,.F.,(4,3,3,3,3,3,3,3,3,3,
3,3,3,3,3,3,3,3,3,3,3,3,3,3,3,3,3,3,3,3,3,3,4),(-0.569248610399399,-0.543574645887706,
-0.517272416441957,-0.510408710919313,-0.50480052039467,-0.477739691816766,
-0.455902626824495,-0.447185798618006,-0.442501671257752,-0.414772030968201,
-0.386610421128685,-0.358667819158644,-0.344761657338633,-0.340663036091181,
-0.336259738054214,-0.307329079232925,-0.3030431718786,-0.27522663544686,
-0.246781288661493,-0.236972581300584,-0.232129263502791,-0.228298636689681,
-0.199315265324891,-0.169757082759818,-0.139958578416395,-0.123701382742228,
-0.11872612058217,-0.114411165373038,-0.0838710232821164,-0.0532918814757283,
-0.023320643283923,-0.00990101302305864,0.),.UNSPECIFIED.);
#5928=B_SPLINE_CURVE_WITH_KNOTS('',3,(#43328,#43329,#43330,#43331,#43332,
#43333,#43334,#43335,#43336,#43337,#43338,#43339,#43340,#43341,#43342,#43343,
#43344,#43345,#43346,#43347,#43348,#43349,#43350,#43351,#43352,#43353,#43354,
#43355,#43356,#43357,#43358,#43359,#43360,#43361,#43362,#43363,#43364,#43365,
#43366,#43367,#43368,#43369,#43370,#43371,#43372,#43373,#43374,#43375,#43376,
#43377,#43378,#43379,#43380,#43381,#43382,#43383,#43384,#43385,#43386,#43387,
#43388,#43389,#43390,#43391,#43392,#43393,#43394,#43395,#43396,#43397,#43398,
#43399,#43400,#43401,#43402,#43403,#43404,#43405,#43406,#43407,#43408,#43409,
#43410,#43411,#43412,#43413,#43414,#43415,#43416,#43417,#43418,#43419,#43420,
#43421),.UNSPECIFIED.,.F.,.F.,(4,3,3,3,3,3,3,3,3,3,3,3,3,3,3,3,3,3,3,3,
3,3,3,3,3,3,3,3,3,3,3,4),(-0.566847306047971,-0.53666587364779,-0.506059968026337,
-0.497416424417392,-0.490479625055067,-0.460332813265244,-0.437094437432501,
-0.424724940231172,-0.420483374246613,-0.391058520491087,-0.361900342019141,
-0.333575724639118,-0.318788245130165,-0.313125879786658,-0.308695953827476,
-0.280705559915183,-0.274425806603304,-0.245949103194913,-0.216224272779601,
-0.204597317066248,-0.200878698444207,-0.173045197056922,-0.145277260918581,
-0.117980532340416,-0.104251773281916,-0.100006089570323,-0.095828408862559,
-0.0691557456961475,-0.0429305361237256,-0.0175053478877417,-0.0081504598724134,
0.),.UNSPECIFIED.);
#5929=B_SPLINE_CURVE_WITH_KNOTS('',3,(#43423,#43424,#43425,#43426,#43427,
#43428,#43429,#43430,#43431,#43432,#43433),.UNSPECIFIED.,.F.,.F.,(4,1,1,
1,1,1,1,1,4),(15.7079632679489,15.8286682231622,16.8210880633759,17.8135079035895,
18.8059277438031,19.7983475840168,20.7907674242304,21.783187264444,21.9911485751284),
 .UNSPECIFIED.);
#5930=B_SPLINE_CURVE_WITH_KNOTS('',3,(#43434,#43435,#43436,#43437,#43438,
#43439,#43440,#43441,#43442,#43443),.UNSPECIFIED.,.F.,.F.,(4,1,1,1,1,1,
1,4),(15.7079632679489,16.3832398073991,17.3756596476127,18.3680794878263,
19.36049932804,20.3529191682536,21.3453390084673,21.9911485751284),
 .UNSPECIFIED.);
#5931=B_SPLINE_CURVE_WITH_KNOTS('',3,(#43844,#43845,#43846,#43847,#43848,
#43849,#43850,#43851,#43852,#43853,#43854,#43855,#43856,#43857,#43858,#43859,
#43860,#43861,#43862,#43863,#43864,#43865,#43866,#43867,#43868,#43869,#43870,
#43871,#43872,#43873,#43874,#43875,#43876,#43877,#43878,#43879,#43880,#43881,
#43882,#43883,#43884,#43885,#43886,#43887,#43888,#43889,#43890,#43891,#43892,
#43893,#43894,#43895,#43896,#43897,#43898,#43899,#43900,#43901,#43902,#43903,
#43904,#43905,#43906,#43907,#43908,#43909,#43910,#43911,#43912,#43913,#43914,
#43915,#43916,#43917,#43918,#43919,#43920,#43921,#43922,#43923,#43924,#43925,
#43926,#43927,#43928,#43929,#43930,#43931,#43932,#43933,#43934,#43935,#43936,
#43937),.UNSPECIFIED.,.F.,.F.,(4,3,3,3,3,3,3,3,3,3,3,3,3,3,3,3,3,3,3,3,
3,3,3,3,3,3,3,3,3,3,3,4),(0.,0.0253630076180288,0.0513975877046809,0.0781461974825396,
0.0899194311896693,0.0966315930649138,0.102678021603326,0.129978474904837,
0.157730194774643,0.18464426256287,0.195932069023516,0.203012843388201,
0.20715665261236,0.236271559269955,0.26538646592755,0.293279280417395,0.302554895181128,
0.311292641824619,0.315704538622333,0.343817446040152,0.372959156505691,
0.402412706796253,0.413342529374516,0.4228990774176,0.428117895612503,0.458184942155295,
0.482885329773834,0.492048651182197,0.498170303933628,0.528680777336123,
0.556986492629451,0.566847306048124),.UNSPECIFIED.);
#5932=B_SPLINE_CURVE_WITH_KNOTS('',3,(#43938,#43939,#43940,#43941,#43942,
#43943,#43944,#43945,#43946,#43947,#43948,#43949,#43950,#43951,#43952,#43953,
#43954,#43955,#43956,#43957,#43958,#43959,#43960,#43961,#43962),
 .UNSPECIFIED.,.F.,.F.,(4,3,3,3,3,3,3,3,4),(-10.1321597128208,-9.92419840213634,
-8.93177856192271,-7.93935872170907,-6.94693888149544,-5.9545190412818,
-4.96209920106817,-3.96967936085453,-3.84897440564123),.UNSPECIFIED.);
#5933=B_SPLINE_CURVE_WITH_KNOTS('',3,(#44363,#44364,#44365,#44366,#44367,
#44368,#44369,#44370,#44371,#44372,#44373,#44374,#44375,#44376,#44377,#44378,
#44379,#44380,#44381,#44382,#44383,#44384),.UNSPECIFIED.,.F.,.F.,(4,3,3,
3,3,3,3,4),(7.59274844815659,7.93935872170907,8.9317785619227,9.92419840213634,
10.91661824235,11.9090380825636,12.9014579227772,13.8759337553361),
 .UNSPECIFIED.);
#5934=B_SPLINE_CURVE_WITH_KNOTS('',3,(#44385,#44386,#44387,#44388,#44389,
#44390,#44391,#44392,#44393,#44394,#44395,#44396,#44397,#44398,#44399,#44400,
#44401,#44402,#44403,#44404,#44405,#44406,#44407,#44408,#44409,#44410,#44411,
#44412,#44413,#44414,#44415,#44416,#44417,#44418,#44419,#44420,#44421,#44422,
#44423,#44424,#44425,#44426,#44427,#44428,#44429,#44430,#44431,#44432,#44433,
#44434,#44435,#44436,#44437,#44438,#44439,#44440,#44441,#44442,#44443,#44444,
#44445,#44446,#44447,#44448,#44449,#44450,#44451,#44452,#44453,#44454,#44455,
#44456,#44457,#44458,#44459,#44460,#44461,#44462,#44463,#44464,#44465,#44466,
#44467,#44468,#44469,#44470,#44471,#44472,#44473,#44474,#44475),
 .UNSPECIFIED.,.F.,.F.,(4,3,3,3,3,3,3,3,3,3,3,3,3,3,3,3,3,3,3,3,3,3,3,3,
3,3,3,3,3,3,4),(0.,0.0297241015280599,0.0601072589092367,0.089339530253816,
0.114917767680323,0.120626861021768,0.150385991078755,0.179981397219412,
0.208477405331027,0.220429498709529,0.228738535617177,0.234134414459521,
0.264049922062696,0.291955952722432,0.293965429665871,0.322911497915157,
0.339206043082875,0.343413983241414,0.371506227313122,0.399645180488026,
0.427381808130137,0.437705383100523,0.444698406356017,0.448877348536544,
0.476925686623981,0.497961940189559,0.506030881403263,0.51179113945871,
0.537728950453386,0.561070700886291,0.569248610399393),.UNSPECIFIED.);
#5935=B_SPLINE_CURVE_WITH_KNOTS('',3,(#44478,#44479,#44480,#44481,#44482,
#44483,#44484,#44485,#44486,#44487,#44488,#44489,#44490,#44491,#44492,#44493,
#44494,#44495,#44496,#44497,#44498,#44499,#44500,#44501,#44502,#44503,#44504,
#44505,#44506,#44507,#44508,#44509,#44510,#44511,#44512,#44513,#44514,#44515,
#44516,#44517,#44518,#44519,#44520,#44521,#44522,#44523,#44524,#44525,#44526,
#44527,#44528,#44529,#44530,#44531,#44532,#44533,#44534,#44535,#44536,#44537,
#44538,#44539,#44540,#44541,#44542,#44543,#44544,#44545,#44546,#44547,#44548,
#44549,#44550,#44551,#44552,#44553,#44554,#44555,#44556,#44557,#44558,#44559,
#44560,#44561,#44562,#44563,#44564,#44565,#44566,#44567,#44568,#44569,#44570,
#44571,#44572,#44573,#44574),.UNSPECIFIED.,.F.,.F.,(4,3,3,3,3,3,3,3,3,3,
3,3,3,3,3,3,3,3,3,3,3,3,3,3,3,3,3,3,3,3,3,3,4),(-0.569248610399393,-0.543574674480804,
-0.517272469051126,-0.510408841912501,-0.504800525129289,-0.477739716670525,
-0.455902648571535,-0.447186002233845,-0.442501828177038,-0.414772209830522,
-0.386610599542292,-0.358667985965373,-0.344761782443679,-0.340663244529424,
-0.336259792696339,-0.30732913293683,-0.303043171878598,-0.275226617339747,
-0.246781259091957,-0.236972491194407,-0.232129113765856,-0.228298489515272,
-0.199315100266808,-0.169756908209147,-0.139958402689496,-0.123701228981192,
-0.118725698812402,-0.114410751166567,-0.0838706032234413,-0.0532914639090378,
-0.0233202292854336,-0.00990101302306306,0.),.UNSPECIFIED.);
#5936=B_SPLINE_CURVE_WITH_KNOTS('',3,(#44575,#44576,#44577,#44578,#44579,
#44580,#44581,#44582,#44583,#44584,#44585,#44586,#44587,#44588,#44589,#44590,
#44591,#44592,#44593,#44594,#44595,#44596,#44597,#44598,#44599,#44600,#44601,
#44602,#44603,#44604,#44605,#44606,#44607,#44608,#44609,#44610,#44611,#44612,
#44613,#44614,#44615,#44616,#44617,#44618,#44619,#44620,#44621,#44622,#44623,
#44624,#44625,#44626,#44627,#44628,#44629,#44630,#44631,#44632,#44633,#44634,
#44635,#44636,#44637,#44638,#44639,#44640,#44641,#44642,#44643,#44644,#44645,
#44646,#44647,#44648,#44649,#44650,#44651,#44652,#44653,#44654,#44655,#44656,
#44657,#44658,#44659,#44660,#44661,#44662,#44663,#44664,#44665,#44666,#44667,
#44668),.UNSPECIFIED.,.F.,.F.,(4,3,3,3,3,3,3,3,3,3,3,3,3,3,3,3,3,3,3,3,
3,3,3,3,3,3,3,3,3,3,3,4),(-0.566847306048015,-0.536665868221327,-0.506059961122649,
-0.497416415953207,-0.490479623350436,-0.460332811693897,-0.437094436057574,
-0.424724937050165,-0.42048337099133,-0.391058517828774,-0.361900340022409,
-0.333575724459701,-0.318788244995605,-0.313125878209896,-0.308695953223835,
-0.280705561460601,-0.274425806603314,-0.245949103343717,-0.216224272909805,
-0.204597316755682,-0.20087869834534,-0.173045196570911,-0.145277260583828,
-0.117980533828581,-0.10425177458406,-0.100006094404146,-0.0958284101891435,
-0.0691557481657235,-0.0429305412409989,-0.0175053576029524,-0.00815045987241369,
0.),.UNSPECIFIED.);
#5937=B_SPLINE_CURVE_WITH_KNOTS('',3,(#44670,#44671,#44672,#44673,#44674,
#44675,#44676,#44677,#44678,#44679,#44680),.UNSPECIFIED.,.F.,.F.,(4,1,1,
1,1,1,1,1,4),(15.7079632679489,15.8286682231624,16.821088063376,17.8135079035896,
18.8059277438032,19.7983475840169,20.7907674242305,21.7831872644441,21.9911485751285),
 .UNSPECIFIED.);
#5938=B_SPLINE_CURVE_WITH_KNOTS('',3,(#44681,#44682,#44683,#44684,#44685,
#44686,#44687,#44688,#44689,#44690),.UNSPECIFIED.,.F.,.F.,(4,1,1,1,1,1,
1,4),(15.7079632679489,16.3832398073992,17.3756596476128,18.3680794878265,
19.3604993280401,20.3529191682537,21.3453390084674,21.9911485751284),
 .UNSPECIFIED.);
#5939=B_SPLINE_CURVE_WITH_KNOTS('',3,(#45091,#45092,#45093,#45094,#45095,
#45096,#45097,#45098,#45099,#45100,#45101,#45102,#45103,#45104,#45105,#45106,
#45107,#45108,#45109,#45110,#45111,#45112,#45113,#45114,#45115,#45116,#45117,
#45118,#45119,#45120,#45121,#45122,#45123,#45124,#45125,#45126,#45127,#45128,
#45129,#45130,#45131,#45132,#45133,#45134,#45135,#45136,#45137,#45138,#45139,
#45140,#45141,#45142,#45143,#45144,#45145,#45146,#45147,#45148,#45149,#45150,
#45151,#45152,#45153,#45154,#45155,#45156,#45157,#45158,#45159,#45160,#45161,
#45162,#45163,#45164,#45165,#45166,#45167,#45168,#45169,#45170,#45171,#45172,
#45173,#45174,#45175,#45176,#45177,#45178,#45179,#45180,#45181,#45182,#45183,
#45184),.UNSPECIFIED.,.F.,.F.,(4,3,3,3,3,3,3,3,3,3,3,3,3,3,3,3,3,3,3,3,
3,3,3,3,3,3,3,3,3,3,3,4),(0.,0.0253630162810394,0.0513976042172585,0.078146211931042,
0.0899194345617105,0.0966315935064485,0.102678021607179,0.129978481016302,
0.157730203957742,0.184644269450188,0.195932070537851,0.203012844021181,
0.207156653941548,0.236271559934537,0.265386465927526,0.293279276361684,
0.302554886851352,0.31129260608518,0.315704531791299,0.343817433364416,
0.372959141111239,0.402412690720333,0.41334249920042,0.422898961216315,
0.428117885617758,0.458184930864427,0.482885321305682,0.492048630602995,
0.498170305601047,0.528680779114337,0.556986492629444,0.566847306048072),
 .UNSPECIFIED.);
#5940=B_SPLINE_CURVE_WITH_KNOTS('',3,(#45185,#45186,#45187,#45188,#45189,
#45190,#45191,#45192,#45193,#45194,#45195,#45196,#45197,#45198,#45199,#45200,
#45201,#45202,#45203,#45204,#45205,#45206,#45207,#45208,#45209),
 .UNSPECIFIED.,.F.,.F.,(4,3,3,3,3,3,3,3,4),(-10.1321597128207,-9.92419840213633,
-8.93177856192269,-7.93935872170906,-6.94693888149543,-5.9545190412818,
-4.96209920106816,-3.96967936085453,-3.848974405641),.UNSPECIFIED.);
#5941=B_SPLINE_CURVE_WITH_KNOTS('',3,(#45610,#45611,#45612,#45613,#45614,
#45615,#45616,#45617,#45618,#45619,#45620,#45621,#45622,#45623,#45624,#45625,
#45626,#45627,#45628,#45629,#45630,#45631),.UNSPECIFIED.,.F.,.F.,(4,3,3,
3,3,3,3,4),(7.59274844815647,7.93935872170906,8.93177856192269,9.92419840213633,
10.91661824235,11.9090380825636,12.9014579227772,13.875933755336),
 .UNSPECIFIED.);
#5942=B_SPLINE_CURVE_WITH_KNOTS('',3,(#45632,#45633,#45634,#45635,#45636,
#45637,#45638,#45639,#45640,#45641,#45642,#45643,#45644,#45645,#45646,#45647,
#45648,#45649,#45650,#45651,#45652,#45653,#45654,#45655,#45656,#45657,#45658,
#45659,#45660,#45661,#45662,#45663,#45664,#45665,#45666,#45667,#45668,#45669,
#45670,#45671,#45672,#45673,#45674,#45675,#45676,#45677,#45678,#45679,#45680,
#45681,#45682,#45683,#45684,#45685,#45686,#45687,#45688,#45689,#45690,#45691,
#45692,#45693,#45694,#45695,#45696,#45697,#45698,#45699,#45700,#45701,#45702,
#45703,#45704,#45705,#45706,#45707,#45708,#45709,#45710,#45711,#45712,#45713,
#45714,#45715,#45716,#45717,#45718,#45719,#45720,#45721,#45722),
 .UNSPECIFIED.,.F.,.F.,(4,3,3,3,3,3,3,3,3,3,3,3,3,3,3,3,3,3,3,3,3,3,3,3,
3,3,3,3,3,3,4),(0.,0.0297240764494745,0.0601072212620576,0.0893394973125421,
0.114917738856716,0.120626859131278,0.150385988643545,0.179981401276396,
0.20847740837378,0.220429505923984,0.228738554654763,0.234134418137665,
0.264049923901799,0.291955960666471,0.293965429665934,0.322911496593631,
0.339206045811635,0.343413985730059,0.371506228953445,0.399645181615295,
0.427381813866647,0.437705397278763,0.44469853997657,0.448877487839921,
0.47692579110155,0.497962018547772,0.506031026512302,0.511791114109563,
0.537728937371717,0.561070700886438,0.569248610399523),.UNSPECIFIED.);
#5943=B_SPLINE_CURVE_WITH_KNOTS('',3,(#45725,#45726,#45727,#45728,#45729,
#45730,#45731,#45732,#45733,#45734,#45735,#45736,#45737,#45738,#45739,#45740,
#45741,#45742,#45743,#45744,#45745,#45746,#45747,#45748,#45749,#45750,#45751,
#45752,#45753,#45754,#45755,#45756,#45757,#45758,#45759,#45760,#45761,#45762,
#45763,#45764,#45765,#45766,#45767,#45768,#45769,#45770,#45771,#45772,#45773,
#45774,#45775,#45776,#45777,#45778,#45779,#45780,#45781,#45782,#45783,#45784,
#45785,#45786,#45787,#45788,#45789,#45790,#45791,#45792,#45793,#45794,#45795,
#45796,#45797,#45798,#45799,#45800,#45801,#45802,#45803,#45804,#45805,#45806,
#45807,#45808,#45809,#45810,#45811,#45812,#45813,#45814,#45815,#45816,#45817,
#45818,#45819,#45820,#45821),.UNSPECIFIED.,.F.,.F.,(4,3,3,3,3,3,3,3,3,3,
3,3,3,3,3,3,3,3,3,3,3,3,3,3,3,3,3,3,3,3,3,3,4),(-0.569248610399377,-0.54357467448165,
-0.517272469053758,-0.510408841918492,-0.50480052502851,-0.477739716567738,
-0.455902648481596,-0.447186001443042,-0.44250182771911,-0.414772209355928,
-0.386610599068325,-0.358667985497239,-0.34476178209258,-0.340663244000883,
-0.336259792559757,-0.30732913279944,-0.303043171878604,-0.2752266173411,
-0.246781259100878,-0.236972491217739,-0.232129113745793,-0.228298489561011,
-0.199315100312039,-0.169756908254245,-0.139958402733899,-0.123701229020045,
-0.118725698872309,-0.114410751243681,-0.083870603296885,-0.0532914639826537,
-0.0233202293554824,-0.00990101302306316,0.),.UNSPECIFIED.);
#5944=B_SPLINE_CURVE_WITH_KNOTS('',3,(#45822,#45823,#45824,#45825,#45826,
#45827,#45828,#45829,#45830,#45831,#45832,#45833,#45834,#45835,#45836,#45837,
#45838,#45839,#45840,#45841,#45842,#45843,#45844,#45845,#45846,#45847,#45848,
#45849,#45850,#45851,#45852,#45853,#45854,#45855,#45856,#45857,#45858,#45859,
#45860,#45861,#45862,#45863,#45864,#45865,#45866,#45867,#45868,#45869,#45870,
#45871,#45872,#45873,#45874,#45875,#45876,#45877,#45878,#45879,#45880,#45881,
#45882,#45883,#45884,#45885,#45886,#45887,#45888,#45889,#45890,#45891,#45892,
#45893,#45894,#45895,#45896,#45897,#45898,#45899,#45900,#45901,#45902,#45903,
#45904,#45905,#45906,#45907,#45908,#45909,#45910,#45911,#45912,#45913,#45914,
#45915),.UNSPECIFIED.,.F.,.F.,(4,3,3,3,3,3,3,3,3,3,3,3,3,3,3,3,3,3,3,3,
3,3,3,3,3,3,3,3,3,3,3,4),(-0.566847306047991,-0.53666586821921,-0.506059961126055,
-0.497416415953077,-0.49047962338091,-0.460332811721525,-0.43709443608175,
-0.424724937095777,-0.420483370923851,-0.391058517764092,-0.3619003399739,
-0.333575724413931,-0.318788244961279,-0.31312587811604,-0.308695953184524,
-0.280705561426923,-0.274425806603322,-0.245949103340888,-0.216224272907329,
-0.204597316758108,-0.200878698422677,-0.17304519665064,-0.145277260663322,
-0.117980533917273,-0.104251774661665,-0.100006094574606,-0.0958284102179013,
-0.0691557481942624,-0.0429305412697575,-0.0175053576280775,-0.00815045987241409,
0.),.UNSPECIFIED.);
#5945=B_SPLINE_CURVE_WITH_KNOTS('',3,(#45917,#45918,#45919,#45920,#45921,
#45922,#45923,#45924,#45925,#45926,#45927),.UNSPECIFIED.,.F.,.F.,(4,1,1,
1,1,1,1,1,4),(15.7079632679488,15.8286682231622,16.8210880633759,17.8135079035895,
18.8059277438031,19.7983475840168,20.7907674242304,21.783187264444,21.9911485751285),
 .UNSPECIFIED.);
#5946=B_SPLINE_CURVE_WITH_KNOTS('',3,(#45928,#45929,#45930,#45931,#45932,
#45933,#45934,#45935,#45936,#45937),.UNSPECIFIED.,.F.,.F.,(4,1,1,1,1,1,
1,4),(15.7079632679489,16.3832398073991,17.3756596476127,18.3680794878263,
19.36049932804,20.3529191682536,21.3453390084673,21.9911485751284),
 .UNSPECIFIED.);
#5947=B_SPLINE_CURVE_WITH_KNOTS('',3,(#46338,#46339,#46340,#46341,#46342,
#46343,#46344,#46345,#46346,#46347,#46348,#46349,#46350,#46351,#46352,#46353,
#46354,#46355,#46356,#46357,#46358,#46359,#46360,#46361,#46362,#46363,#46364,
#46365,#46366,#46367,#46368,#46369,#46370,#46371,#46372,#46373,#46374,#46375,
#46376,#46377,#46378,#46379,#46380,#46381,#46382,#46383,#46384,#46385,#46386,
#46387,#46388,#46389,#46390,#46391,#46392,#46393,#46394,#46395,#46396,#46397,
#46398,#46399,#46400,#46401,#46402,#46403,#46404,#46405,#46406,#46407,#46408,
#46409,#46410,#46411,#46412,#46413,#46414,#46415,#46416,#46417,#46418,#46419,
#46420,#46421,#46422,#46423,#46424,#46425,#46426,#46427,#46428,#46429,#46430,
#46431),.UNSPECIFIED.,.F.,.F.,(4,3,3,3,3,3,3,3,3,3,3,3,3,3,3,3,3,3,3,3,
3,3,3,3,3,3,3,3,3,3,3,4),(0.,0.0253630162801341,0.051397604216831,0.0781462119306684,
0.0899194345617906,0.0966315935064221,0.102678021611154,0.129978481020733,
0.157730203962062,0.184644269453429,0.195932070538785,0.20301284402031,
0.207156653926934,0.236271559927232,0.26538646592753,0.293279276361627,
0.302554886851072,0.311292606084599,0.315704531791214,0.343817433364128,
0.372959141111098,0.402412690720469,0.413342499200516,0.422898961216301,
0.428117885617808,0.458184930864438,0.482885321305687,0.49204863060229,
0.498170305654284,0.528680779169399,0.556986492629434,0.566847306048108),
 .UNSPECIFIED.);
#5948=B_SPLINE_CURVE_WITH_KNOTS('',3,(#46432,#46433,#46434,#46435,#46436,
#46437,#46438,#46439,#46440,#46441,#46442,#46443,#46444,#46445,#46446,#46447,
#46448,#46449,#46450,#46451,#46452,#46453,#46454,#46455,#46456),
 .UNSPECIFIED.,.F.,.F.,(4,3,3,3,3,3,3,3,4),(-10.1321597128208,-9.92419840213633,
-8.9317785619227,-7.93935872170907,-6.94693888149544,-5.9545190412818,-4.96209920106817,
-3.96967936085453,-3.84897440564123),.UNSPECIFIED.);
#5949=B_SPLINE_CURVE_WITH_KNOTS('',3,(#46857,#46858,#46859,#46860,#46861,
#46862,#46863,#46864,#46865,#46866,#46867,#46868,#46869,#46870,#46871,#46872,
#46873,#46874,#46875,#46876,#46877,#46878),.UNSPECIFIED.,.F.,.F.,(4,3,3,
3,3,3,3,4),(7.59274844815659,7.93935872170907,8.9317785619227,9.92419840213634,
10.91661824235,11.9090380825636,12.9014579227772,13.8759337553361),
 .UNSPECIFIED.);
#5950=B_SPLINE_CURVE_WITH_KNOTS('',3,(#46879,#46880,#46881,#46882,#46883,
#46884,#46885,#46886,#46887,#46888,#46889,#46890,#46891,#46892,#46893,#46894,
#46895,#46896,#46897,#46898,#46899,#46900,#46901,#46902,#46903,#46904,#46905,
#46906,#46907,#46908,#46909,#46910,#46911,#46912,#46913,#46914,#46915,#46916,
#46917,#46918,#46919,#46920,#46921,#46922,#46923,#46924,#46925,#46926,#46927,
#46928,#46929,#46930,#46931,#46932,#46933,#46934,#46935,#46936,#46937,#46938,
#46939,#46940,#46941,#46942,#46943,#46944,#46945,#46946,#46947,#46948,#46949,
#46950,#46951,#46952,#46953,#46954,#46955,#46956,#46957,#46958,#46959,#46960,
#46961,#46962,#46963,#46964,#46965,#46966,#46967,#46968,#46969),
 .UNSPECIFIED.,.F.,.F.,(4,3,3,3,3,3,3,3,3,3,3,3,3,3,3,3,3,3,3,3,3,3,3,3,
3,3,3,3,3,3,4),(0.,0.029724076449364,0.0601072212623451,0.0893394973127924,
0.114917738856934,0.120626859134211,0.150385988646724,0.179981401279999,
0.20847740837648,0.220429505928215,0.228738554666963,0.234134418130225,
0.264049923898074,0.291955960662473,0.293965429665923,0.322911496595274,
0.339206045815667,0.34341398573459,0.371506228958071,0.399645181620042,
0.427381813870245,0.43770539728599,0.444698540053498,0.448877487941438,
0.476925791177684,0.497962018604869,0.506031026616555,0.511791114086853,
0.537728937350807,0.561070700886424,0.569248610399524),.UNSPECIFIED.);
#5951=B_SPLINE_CURVE_WITH_KNOTS('',3,(#46972,#46973,#46974,#46975,#46976,
#46977,#46978,#46979,#46980,#46981,#46982,#46983,#46984,#46985,#46986,#46987,
#46988,#46989,#46990,#46991,#46992,#46993,#46994,#46995,#46996,#46997,#46998,
#46999,#47000,#47001,#47002,#47003,#47004,#47005,#47006,#47007,#47008,#47009,
#47010,#47011,#47012,#47013,#47014,#47015,#47016,#47017,#47018,#47019,#47020,
#47021,#47022,#47023,#47024,#47025,#47026,#47027,#47028,#47029,#47030,#47031,
#47032,#47033,#47034,#47035,#47036,#47037,#47038,#47039,#47040,#47041,#47042,
#47043,#47044,#47045,#47046,#47047,#47048,#47049,#47050,#47051,#47052,#47053,
#47054,#47055,#47056,#47057,#47058,#47059,#47060,#47061,#47062,#47063,#47064,
#47065,#47066,#47067,#47068),.UNSPECIFIED.,.F.,.F.,(4,3,3,3,3,3,3,3,3,3,
3,3,3,3,3,3,3,3,3,3,3,3,3,3,3,3,3,3,3,3,3,3,4),(-0.569248610399425,-0.543574656378576,
-0.517272435738008,-0.510408758966565,-0.504800522056745,-0.477739700856869,
-0.45590263473459,-0.447185872707102,-0.44250172837546,-0.414772096122201,
-0.386610486117207,-0.358667879895409,-0.344761702891216,-0.340663112078979,
-0.336259757977141,-0.307329098806346,-0.303043171878636,-0.275226628804691,
-0.246781277807599,-0.236972548226137,-0.232129208542884,-0.228298582742164,
-0.199315204818196,-0.169757018770865,-0.13995851399337,-0.123701326372081,
-0.118725966008134,-0.114411013541681,-0.0838708693004695,-0.0532917284052035,
-0.0233204915173235,-0.0099010130230586,0.),.UNSPECIFIED.);
#5952=B_SPLINE_CURVE_WITH_KNOTS('',3,(#47069,#47070,#47071,#47072,#47073,
#47074,#47075,#47076,#47077,#47078,#47079,#47080,#47081,#47082,#47083,#47084,
#47085,#47086,#47087,#47088,#47089,#47090,#47091,#47092,#47093,#47094,#47095,
#47096,#47097,#47098,#47099,#47100,#47101,#47102,#47103,#47104,#47105,#47106,
#47107,#47108,#47109,#47110,#47111,#47112,#47113,#47114,#47115,#47116,#47117,
#47118,#47119,#47120,#47121,#47122,#47123,#47124,#47125,#47126,#47127,#47128,
#47129,#47130,#47131,#47132,#47133,#47134,#47135,#47136,#47137,#47138,#47139,
#47140,#47141,#47142,#47143,#47144,#47145,#47146,#47147,#47148,#47149,#47150,
#47151,#47152,#47153,#47154,#47155,#47156,#47157,#47158,#47159,#47160,#47161,
#47162),.UNSPECIFIED.,.F.,.F.,(4,3,3,3,3,3,3,3,3,3,3,3,3,3,3,3,3,3,3,3,
3,3,3,3,3,3,3,3,3,3,3,4),(-0.566847306048015,-0.536665878440076,-0.50605997412493,
-0.497416431897616,-0.490479626448282,-0.460332814543148,-0.437094438550669,
-0.424724942866698,-0.420483377128068,-0.391058522848951,-0.361900343787542,
-0.333575724793978,-0.318788245246312,-0.313125881168901,-0.308695954326937,
-0.280705558504757,-0.274425806603314,-0.245949103059473,-0.21622427266109,
-0.204597317336048,-0.200878698329781,-0.173045197282773,-0.145277261013689,
-0.117980530827865,-0.104251771958434,-0.100006084890927,-0.0958284076234192,
-0.0691557434471268,-0.042930531532881,-0.017505339237663,-0.00815045987241369,
0.),.UNSPECIFIED.);
#5953=B_SPLINE_CURVE_WITH_KNOTS('',3,(#47164,#47165,#47166,#47167,#47168,
#47169,#47170,#47171,#47172,#47173,#47174),.UNSPECIFIED.,.F.,.F.,(4,1,1,
1,1,1,1,1,4),(15.7079632679489,15.8286682231624,16.821088063376,17.8135079035896,
18.8059277438032,19.7983475840169,20.7907674242305,21.7831872644441,21.9911485751285),
 .UNSPECIFIED.);
#5954=B_SPLINE_CURVE_WITH_KNOTS('',3,(#47175,#47176,#47177,#47178,#47179,
#47180,#47181,#47182,#47183,#47184),.UNSPECIFIED.,.F.,.F.,(4,1,1,1,1,1,
1,4),(15.7079632679489,16.3832398073992,17.3756596476128,18.3680794878265,
19.3604993280401,20.3529191682537,21.3453390084674,21.9911485751284),
 .UNSPECIFIED.);
#5955=B_SPLINE_CURVE_WITH_KNOTS('',3,(#47585,#47586,#47587,#47588,#47589,
#47590,#47591,#47592,#47593,#47594,#47595,#47596,#47597,#47598,#47599,#47600,
#47601,#47602,#47603,#47604,#47605,#47606,#47607,#47608,#47609,#47610,#47611,
#47612,#47613,#47614,#47615,#47616,#47617,#47618,#47619,#47620,#47621,#47622,
#47623,#47624,#47625,#47626,#47627,#47628,#47629,#47630,#47631,#47632,#47633,
#47634,#47635,#47636,#47637,#47638,#47639,#47640,#47641,#47642,#47643,#47644,
#47645,#47646,#47647,#47648,#47649,#47650,#47651,#47652,#47653,#47654,#47655,
#47656,#47657,#47658,#47659,#47660,#47661,#47662,#47663,#47664,#47665,#47666,
#47667,#47668,#47669,#47670,#47671,#47672,#47673,#47674,#47675,#47676,#47677,
#47678),.UNSPECIFIED.,.F.,.F.,(4,3,3,3,3,3,3,3,3,3,3,3,3,3,3,3,3,3,3,3,
3,3,3,3,3,3,3,3,3,3,3,4),(0.,0.0253629999646348,0.0513975731150082,0.078146184716573,
0.0899194282101026,0.0966315926743291,0.102678021610072,0.129978469516054,
0.157730186671017,0.184644256485144,0.195932067687582,0.203012842825234,
0.207156651488905,0.236271558708216,0.265386465927526,0.293279283999271,
0.30255490253839,0.311292673391874,0.315704544656251,0.34381745723653,0.372959170103633,
0.402412720995891,0.413342556026173,0.422899180057392,0.428117904444282,
0.458184952131496,0.482885337255983,0.492048669366015,0.498170302461157,
0.528680775761109,0.556986492629444,0.566847306048072),.UNSPECIFIED.);
#5956=B_SPLINE_CURVE_WITH_KNOTS('',3,(#47679,#47680,#47681,#47682,#47683,
#47684,#47685,#47686,#47687,#47688,#47689,#47690,#47691,#47692,#47693,#47694,
#47695,#47696,#47697,#47698,#47699,#47700,#47701,#47702,#47703),
 .UNSPECIFIED.,.F.,.F.,(4,3,3,3,3,3,3,3,4),(-10.1321597128207,-9.92419840213633,
-8.93177856192269,-7.93935872170906,-6.94693888149543,-5.9545190412818,
-4.96209920106816,-3.96967936085453,-3.848974405641),.UNSPECIFIED.);
#5957=B_SPLINE_CURVE_WITH_KNOTS('',3,(#48104,#48105,#48106,#48107,#48108,
#48109,#48110,#48111,#48112,#48113,#48114,#48115,#48116,#48117,#48118,#48119,
#48120,#48121,#48122,#48123,#48124,#48125),.UNSPECIFIED.,.F.,.F.,(4,3,3,
3,3,3,3,4),(7.59274844815647,7.93935872170906,8.93177856192269,9.92419840213633,
10.91661824235,11.9090380825636,12.9014579227772,13.875933755336),
 .UNSPECIFIED.);
#5958=B_SPLINE_CURVE_WITH_KNOTS('',3,(#48126,#48127,#48128,#48129,#48130,
#48131,#48132,#48133,#48134,#48135,#48136,#48137,#48138,#48139,#48140,#48141,
#48142,#48143,#48144,#48145,#48146,#48147,#48148,#48149,#48150,#48151,#48152,
#48153,#48154,#48155,#48156,#48157,#48158,#48159,#48160,#48161,#48162,#48163,
#48164,#48165,#48166,#48167,#48168,#48169,#48170,#48171,#48172,#48173,#48174,
#48175,#48176,#48177,#48178,#48179,#48180,#48181,#48182,#48183,#48184,#48185,
#48186,#48187,#48188,#48189,#48190,#48191,#48192,#48193,#48194,#48195,#48196,
#48197,#48198,#48199,#48200,#48201,#48202,#48203,#48204,#48205,#48206,#48207,
#48208,#48209,#48210,#48211,#48212,#48213,#48214,#48215,#48216),
 .UNSPECIFIED.,.F.,.F.,(4,3,3,3,3,3,3,3,3,3,3,3,3,3,3,3,3,3,3,3,3,3,3,3,
3,3,3,3,3,3,4),(0.,0.0297240923307022,0.0601072451031547,0.0893395181734978,
0.114917757110048,0.120626860335535,0.150385990192878,0.179981398714595,
0.208477406452421,0.220429501364369,0.228738542625386,0.234134415814125,
0.264049922740012,0.29195595563805,0.293965429665899,0.32291149743097,0.339206044085149,
0.343413984151255,0.371506227912012,0.399645180899159,0.427381810232926,
0.437705388298364,0.444698455347404,0.448877399571227,0.476925724900021,
0.497961968896616,0.506030934564902,0.51179113018769,0.537728945681625,
0.561070700886401,0.569248610399486),.UNSPECIFIED.);
#5959=B_SPLINE_CURVE_WITH_KNOTS('',3,(#48219,#48220,#48221,#48222,#48223,
#48224,#48225,#48226,#48227,#48228,#48229,#48230,#48231,#48232,#48233,#48234,
#48235,#48236,#48237,#48238,#48239,#48240,#48241,#48242,#48243,#48244,#48245,
#48246,#48247,#48248,#48249,#48250,#48251,#48252,#48253,#48254,#48255,#48256,
#48257,#48258,#48259,#48260,#48261,#48262,#48263,#48264,#48265,#48266,#48267,
#48268,#48269,#48270,#48271,#48272,#48273,#48274,#48275,#48276,#48277,#48278,
#48279,#48280,#48281,#48282,#48283,#48284,#48285,#48286,#48287,#48288,#48289,
#48290,#48291,#48292,#48293,#48294,#48295,#48296,#48297,#48298,#48299,#48300,
#48301,#48302,#48303,#48304,#48305,#48306,#48307,#48308,#48309,#48310,#48311,
#48312,#48313,#48314,#48315),.UNSPECIFIED.,.F.,.F.,(4,3,3,3,3,3,3,3,3,3,
3,3,3,3,3,3,3,3,3,3,3,3,3,3,3,3,3,3,3,3,3,3,4),(-0.569248610399326,-0.543574656371614,
-0.517272435735161,-0.510408758961596,-0.504800521992165,-0.477739700790141,
-0.455902634676197,-0.447185872187875,-0.442501727990217,-0.414772095728046,
-0.386610485723793,-0.358667879508254,-0.344761702600837,-0.340663111536621,
-0.336259757837447,-0.30732909867532,-0.303043171878586,-0.275226628803054,
-0.246781277807813,-0.236972548227735,-0.232129208596512,-0.22829858282377,
-0.199315204899583,-0.169757018852598,-0.139958514082241,-0.123701326449843,
-0.11872596618965,-0.114411013673191,-0.0838708694366423,-0.0532917285417125,
-0.0233204916530961,-0.0099010130230633,0.),.UNSPECIFIED.);
#5960=B_SPLINE_CURVE_WITH_KNOTS('',3,(#48316,#48317,#48318,#48319,#48320,
#48321,#48322,#48323,#48324,#48325,#48326,#48327,#48328,#48329,#48330,#48331,
#48332,#48333,#48334,#48335,#48336,#48337,#48338,#48339,#48340,#48341,#48342,
#48343,#48344,#48345,#48346,#48347,#48348,#48349,#48350,#48351,#48352,#48353,
#48354,#48355,#48356,#48357,#48358,#48359,#48360,#48361,#48362,#48363,#48364,
#48365,#48366,#48367,#48368,#48369,#48370,#48371,#48372,#48373,#48374,#48375,
#48376,#48377,#48378,#48379,#48380,#48381,#48382,#48383,#48384,#48385,#48386,
#48387,#48388,#48389,#48390,#48391,#48392,#48393,#48394,#48395,#48396,#48397,
#48398,#48399,#48400,#48401,#48402,#48403,#48404,#48405,#48406,#48407,#48408,
#48409),.UNSPECIFIED.,.F.,.F.,(4,3,3,3,3,3,3,3,3,3,3,3,3,3,3,3,3,3,3,3,
3,3,3,3,3,3,3,3,3,3,3,4),(-0.566847306048114,-0.536665878440344,-0.506059974122399,
-0.497416431894722,-0.490479626354958,-0.460332814450562,-0.437094438469659,
-0.424724942717478,-0.420483376948718,-0.391058522671577,-0.361900343654519,
-0.333575724664248,-0.318788245149022,-0.313125880904265,-0.308695954272495,
-0.280705558454138,-0.274425806603343,-0.245949103055171,-0.216224272657327,
-0.204597317339409,-0.200878698484612,-0.173045197439613,-0.145277261167582,
-0.117980530976068,-0.104251772088112,-0.100006085217883,-0.0958284076765524,
-0.0691557434985927,-0.0429305315826143,-0.0175053392821834,-0.00815045987241368,
0.),.UNSPECIFIED.);
#5961=B_SPLINE_CURVE_WITH_KNOTS('',3,(#48411,#48412,#48413,#48414,#48415,
#48416,#48417,#48418,#48419,#48420,#48421),.UNSPECIFIED.,.F.,.F.,(4,1,1,
1,1,1,1,1,4),(15.7079632679489,15.8286682231622,16.8210880633759,17.8135079035895,
18.8059277438031,19.7983475840168,20.7907674242304,21.783187264444,21.9911485751285),
 .UNSPECIFIED.);
#5962=B_SPLINE_CURVE_WITH_KNOTS('',3,(#48422,#48423,#48424,#48425,#48426,
#48427,#48428,#48429,#48430,#48431),.UNSPECIFIED.,.F.,.F.,(4,1,1,1,1,1,
1,4),(15.7079632679489,16.3832398073991,17.3756596476127,18.3680794878263,
19.36049932804,20.3529191682536,21.3453390084673,21.9911485751284),
 .UNSPECIFIED.);
#5963=B_SPLINE_CURVE_WITH_KNOTS('',3,(#48832,#48833,#48834,#48835,#48836,
#48837,#48838,#48839,#48840,#48841,#48842,#48843,#48844,#48845,#48846,#48847,
#48848,#48849,#48850,#48851,#48852,#48853,#48854,#48855,#48856,#48857,#48858,
#48859,#48860,#48861,#48862,#48863,#48864,#48865,#48866,#48867,#48868,#48869,
#48870,#48871,#48872,#48873,#48874,#48875,#48876,#48877,#48878,#48879,#48880,
#48881,#48882,#48883,#48884,#48885,#48886,#48887,#48888,#48889,#48890,#48891,
#48892,#48893,#48894,#48895,#48896,#48897,#48898,#48899,#48900,#48901,#48902,
#48903,#48904,#48905,#48906,#48907,#48908,#48909,#48910,#48911,#48912,#48913,
#48914,#48915,#48916,#48917,#48918,#48919,#48920,#48921,#48922,#48923,#48924,
#48925),.UNSPECIFIED.,.F.,.F.,(4,3,3,3,3,3,3,3,3,3,3,3,3,3,3,3,3,3,3,3,
3,3,3,3,3,3,3,3,3,3,3,4),(0.,0.0253629999638193,0.0513975731141745,0.0781461847158463,
0.0899194282101058,0.0966315926746491,0.102678021599935,0.129978469505849,
0.157730186661174,0.184644256477768,0.19593206768551,0.203012842827579,
0.207156651488323,0.236271558707936,0.265386465927549,0.293279283999287,
0.302554902538345,0.311292673391422,0.315704544656186,0.343817457237586,
0.372959170104838,0.402412720997358,0.413342556028948,0.422899180067306,
0.428117904445187,0.45818495213231,0.482885337256607,0.492048669366648,
0.498170302461362,0.528680775763151,0.5569864926295,0.566847306048176),
 .UNSPECIFIED.);
#5964=B_SPLINE_CURVE_WITH_KNOTS('',3,(#48926,#48927,#48928,#48929,#48930,
#48931,#48932,#48933,#48934,#48935,#48936,#48937,#48938,#48939,#48940,#48941,
#48942,#48943,#48944,#48945,#48946,#48947,#48948,#48949,#48950),
 .UNSPECIFIED.,.F.,.F.,(4,3,3,3,3,3,3,3,4),(-10.1321597128207,-9.92419840213634,
-8.93177856192271,-7.93935872170907,-6.94693888149544,-5.9545190412818,
-4.96209920106817,-3.96967936085453,-3.84897440564112),.UNSPECIFIED.);
#5965=B_SPLINE_CURVE_WITH_KNOTS('',3,(#49351,#49352,#49353,#49354,#49355,
#49356,#49357,#49358,#49359,#49360,#49361,#49362,#49363,#49364,#49365,#49366,
#49367,#49368,#49369,#49370,#49371,#49372),.UNSPECIFIED.,.F.,.F.,(4,3,3,
3,3,3,3,4),(7.59274844815659,7.93935872170907,8.93177856192271,9.92419840213634,
10.91661824235,11.9090380825636,12.9014579227772,13.8759337553361),
 .UNSPECIFIED.);
#5966=B_SPLINE_CURVE_WITH_KNOTS('',3,(#49373,#49374,#49375,#49376,#49377,
#49378,#49379,#49380,#49381,#49382,#49383,#49384,#49385,#49386,#49387,#49388,
#49389,#49390,#49391,#49392,#49393,#49394,#49395,#49396,#49397,#49398,#49399,
#49400,#49401,#49402,#49403,#49404,#49405,#49406,#49407,#49408,#49409,#49410,
#49411,#49412,#49413,#49414,#49415,#49416,#49417,#49418,#49419,#49420,#49421,
#49422,#49423,#49424,#49425,#49426,#49427,#49428,#49429,#49430,#49431,#49432,
#49433,#49434,#49435,#49436,#49437,#49438,#49439,#49440,#49441,#49442,#49443,
#49444,#49445,#49446,#49447,#49448,#49449,#49450,#49451,#49452,#49453,#49454,
#49455,#49456,#49457,#49458,#49459,#49460,#49461,#49462,#49463),
 .UNSPECIFIED.,.F.,.F.,(4,3,3,3,3,3,3,3,3,3,3,3,3,3,3,3,3,3,3,3,3,3,3,3,
3,3,3,3,3,3,4),(0.,0.0297240923312089,0.0601072451030124,0.0893395181733674,
0.114917757109928,0.120626860329316,0.15038599018687,0.179981398708653,
0.208477406447952,0.220429501357406,0.228738542605281,0.234134415810311,
0.264049922738082,0.291955955636873,0.293965429665852,0.322911497430439,
0.33920604408414,0.343413984146313,0.371506227907014,0.399645180894377,
0.427381810227985,0.437705388288875,0.444698455295926,0.448877399529997,
0.476925724869063,0.497961968873363,0.506030934526871,0.511791130158556,
0.537728945654397,0.561070700886262,0.56924861039936),.UNSPECIFIED.);
#5967=B_SPLINE_CURVE_WITH_KNOTS('',3,(#49466,#49467,#49468,#49469,#49470,
#49471,#49472,#49473,#49474,#49475,#49476,#49477,#49478,#49479,#49480,#49481,
#49482,#49483,#49484,#49485,#49486,#49487,#49488,#49489,#49490,#49491,#49492,
#49493,#49494,#49495,#49496,#49497,#49498,#49499,#49500,#49501,#49502,#49503,
#49504,#49505,#49506,#49507,#49508,#49509,#49510,#49511,#49512,#49513,#49514,
#49515,#49516,#49517,#49518,#49519,#49520,#49521,#49522,#49523,#49524,#49525,
#49526,#49527,#49528,#49529,#49530,#49531,#49532,#49533,#49534,#49535,#49536,
#49537,#49538,#49539,#49540,#49541,#49542,#49543,#49544,#49545,#49546,#49547,
#49548,#49549,#49550,#49551,#49552,#49553,#49554,#49555,#49556,#49557,#49558,
#49559,#49560,#49561,#49562),.UNSPECIFIED.,.F.,.F.,(4,3,3,3,3,3,3,3,3,3,
3,3,3,3,3,3,3,3,3,3,3,3,3,3,3,3,3,3,3,3,3,3,4),(-0.569248610399423,-0.543574645891778,
-0.51727241644857,-0.510408710942387,-0.504800520393797,-0.477739691817378,
-0.455902626825033,-0.44718579861244,-0.442501671168929,-0.414772030874631,
-0.386610421034913,-0.358667819068152,-0.344761657270767,-0.34066303604345,
-0.336259738041431,-0.307329079225934,-0.303043171878612,-0.275226635447314,
-0.246781288655212,-0.236972581282364,-0.232129263600874,-0.22829863691149,
-0.199315265549529,-0.169757082987585,-0.139958578646832,-0.123701382943861,
-0.118726121129318,-0.11441116589234,-0.0838710238026174,-0.0532918819919743,
-0.0233206437919336,-0.00990101302306326,0.),.UNSPECIFIED.);
#5968=B_SPLINE_CURVE_WITH_KNOTS('',3,(#49563,#49564,#49565,#49566,#49567,
#49568,#49569,#49570,#49571,#49572,#49573,#49574,#49575,#49576,#49577,#49578,
#49579,#49580,#49581,#49582,#49583,#49584,#49585,#49586,#49587,#49588,#49589,
#49590,#49591,#49592,#49593,#49594,#49595,#49596,#49597,#49598,#49599,#49600,
#49601,#49602,#49603,#49604,#49605,#49606,#49607,#49608,#49609,#49610,#49611,
#49612,#49613,#49614,#49615,#49616,#49617,#49618,#49619,#49620,#49621,#49622,
#49623,#49624,#49625,#49626,#49627,#49628,#49629,#49630,#49631,#49632,#49633,
#49634,#49635,#49636,#49637,#49638,#49639,#49640,#49641,#49642,#49643,#49644,
#49645,#49646,#49647,#49648,#49649,#49650,#49651,#49652,#49653,#49654,#49655,
#49656),.UNSPECIFIED.,.F.,.F.,(4,3,3,3,3,3,3,3,3,3,3,3,3,3,3,3,3,3,3,3,
3,3,3,3,3,3,3,3,3,3,3,4),(-0.566847306048056,-0.536665873647055,-0.506059968025301,
-0.497416424413022,-0.490479625005237,-0.460332813217141,-0.437094437390416,
-0.424724940155325,-0.420483374200065,-0.391058520446558,-0.361900341985754,
-0.333575724604661,-0.318788245104331,-0.31312587971415,-0.308695953790866,
-0.280705559878078,-0.274425806603343,-0.245949103196031,-0.21622427278058,
-0.204597317060357,-0.200878698417494,-0.173045197029915,-0.145277260891852,
-0.117980532310966,-0.104251773256148,-0.100006089486155,-0.0958284088489193,
-0.0691557456817196,-0.0429305361063101,-0.0175053478708221,-0.00815045987242113,
0.),.UNSPECIFIED.);
#5969=B_SPLINE_CURVE_WITH_KNOTS('',3,(#49658,#49659,#49660,#49661,#49662,
#49663,#49664,#49665,#49666,#49667,#49668),.UNSPECIFIED.,.F.,.F.,(4,1,1,
1,1,1,1,1,4),(15.7079632679489,15.8286682231624,16.821088063376,17.8135079035896,
18.8059277438032,19.7983475840169,20.7907674242305,21.7831872644441,21.9911485751285),
 .UNSPECIFIED.);
#5970=B_SPLINE_CURVE_WITH_KNOTS('',3,(#49669,#49670,#49671,#49672,#49673,
#49674,#49675,#49676,#49677,#49678),.UNSPECIFIED.,.F.,.F.,(4,1,1,1,1,1,
1,4),(15.7079632679489,16.3832398073992,17.3756596476128,18.3680794878265,
19.3604993280401,20.3529191682537,21.3453390084674,21.9911485751284),
 .UNSPECIFIED.);
#5971=B_SPLINE_CURVE_WITH_KNOTS('',3,(#50079,#50080,#50081,#50082,#50083,
#50084,#50085,#50086,#50087,#50088,#50089,#50090,#50091,#50092,#50093,#50094,
#50095,#50096,#50097,#50098,#50099,#50100,#50101,#50102,#50103,#50104,#50105,
#50106,#50107,#50108,#50109,#50110,#50111,#50112,#50113,#50114,#50115,#50116,
#50117,#50118,#50119,#50120,#50121,#50122,#50123,#50124,#50125,#50126,#50127,
#50128,#50129,#50130,#50131,#50132,#50133,#50134,#50135,#50136,#50137,#50138,
#50139,#50140,#50141,#50142,#50143,#50144,#50145,#50146,#50147,#50148,#50149,
#50150,#50151,#50152,#50153,#50154,#50155,#50156,#50157,#50158,#50159,#50160,
#50161,#50162,#50163,#50164,#50165,#50166,#50167,#50168,#50169,#50170,#50171,
#50172),.UNSPECIFIED.,.F.,.F.,(4,3,3,3,3,3,3,3,3,3,3,3,3,3,3,3,3,3,3,3,
3,3,3,3,3,3,3,3,3,3,3,4),(0.,0.0253630076183808,0.0513975877048671,0.0781461974827044,
0.0899194311895631,0.0966315930648587,0.102678021607527,0.129978474909251,
0.157730194778542,0.184644262565798,0.195932069024234,0.203012843385935,
0.20715665262694,0.236271559277253,0.265386465927566,0.293279280416962,
0.302554895180608,0.311292641822859,0.31570453862194,0.343817446039294,
0.372959156504723,0.402412706795326,0.413342529372535,0.422899077410131,
0.428117895611974,0.458184942153285,0.482885329772337,0.492048651178443,
0.498170303955202,0.528680777355495,0.556986492629494,0.56684730604812),
 .UNSPECIFIED.);
#5972=B_SPLINE_CURVE_WITH_KNOTS('',3,(#50173,#50174,#50175,#50176,#50177,
#50178,#50179,#50180,#50181,#50182,#50183,#50184,#50185,#50186,#50187,#50188,
#50189,#50190,#50191,#50192,#50193,#50194,#50195,#50196,#50197),
 .UNSPECIFIED.,.F.,.F.,(4,3,3,3,3,3,3,3,4),(-10.1321597128207,-9.92419840213632,
-8.93177856192269,-7.93935872170906,-6.94693888149543,-5.95451904128179,
-4.96209920106816,-3.96967936085453,-3.848974405641),.UNSPECIFIED.);
#5973=B_SPLINE_CURVE_WITH_KNOTS('',3,(#50598,#50599,#50600,#50601,#50602,
#50603,#50604,#50605,#50606,#50607,#50608,#50609,#50610,#50611,#50612,#50613,
#50614,#50615,#50616,#50617,#50618,#50619),.UNSPECIFIED.,.F.,.F.,(4,3,3,
3,3,3,3,4),(7.59274844815647,7.93935872170907,8.9317785619227,9.92419840213634,
10.91661824235,11.9090380825636,12.9014579227772,13.875933755336),
 .UNSPECIFIED.);
#5974=B_SPLINE_CURVE_WITH_KNOTS('',3,(#50620,#50621,#50622,#50623,#50624,
#50625,#50626,#50627,#50628,#50629,#50630,#50631,#50632,#50633,#50634,#50635,
#50636,#50637,#50638,#50639,#50640,#50641,#50642,#50643,#50644,#50645,#50646,
#50647,#50648,#50649,#50650,#50651,#50652,#50653,#50654,#50655,#50656,#50657,
#50658,#50659,#50660,#50661,#50662,#50663,#50664,#50665,#50666,#50667,#50668,
#50669,#50670,#50671,#50672,#50673,#50674,#50675,#50676,#50677,#50678,#50679,
#50680,#50681,#50682,#50683,#50684,#50685,#50686,#50687,#50688,#50689,#50690,
#50691,#50692,#50693,#50694,#50695,#50696,#50697,#50698,#50699,#50700,#50701,
#50702,#50703,#50704,#50705,#50706,#50707,#50708,#50709,#50710),
 .UNSPECIFIED.,.F.,.F.,(4,3,3,3,3,3,3,3,3,3,3,3,3,3,3,3,3,3,3,3,3,3,3,3,
3,3,3,3,3,3,4),(0.,0.0297241015279183,0.0601072589089457,0.0893395302535658,
0.114917767680108,0.120626861018893,0.150385991075238,0.179981397216016,
0.208477405328489,0.220429498705637,0.228738535605999,0.234134414463615,
0.264049922064761,0.291955952723935,0.293965429665907,0.322911497914105,
0.339206043080533,0.343413983249963,0.371506227321681,0.39964518049671,
0.427381808138431,0.437705383117277,0.444698406530902,0.44887734867021,
0.476925686724255,0.497961940264788,0.506030881533375,0.511791139434088,
0.537728950428119,0.561070700886389,0.569248610399474),.UNSPECIFIED.);
#5975=B_SPLINE_CURVE_WITH_KNOTS('',3,(#50713,#50714,#50715,#50716,#50717,
#50718,#50719,#50720,#50721,#50722,#50723,#50724,#50725,#50726,#50727,#50728,
#50729,#50730,#50731,#50732,#50733,#50734,#50735,#50736,#50737,#50738,#50739,
#50740,#50741,#50742,#50743,#50744,#50745,#50746,#50747,#50748,#50749,#50750,
#50751,#50752,#50753,#50754,#50755,#50756,#50757,#50758,#50759,#50760,#50761,
#50762,#50763,#50764,#50765,#50766,#50767,#50768,#50769,#50770,#50771,#50772,
#50773,#50774,#50775,#50776,#50777,#50778,#50779,#50780,#50781,#50782,#50783,
#50784,#50785,#50786,#50787,#50788,#50789,#50790,#50791,#50792,#50793,#50794,
#50795,#50796,#50797,#50798,#50799,#50800,#50801,#50802,#50803,#50804,#50805,
#50806,#50807,#50808,#50809),.UNSPECIFIED.,.F.,.F.,(4,3,3,3,3,3,3,3,3,3,
3,3,3,3,3,3,3,3,3,3,3,3,3,3,3,3,3,3,3,3,3,3,4),(-0.569248610399393,-0.5435746659104,
-0.517272453279993,-0.510408802643641,-0.504800523617045,-0.477739709125334,
-0.455902641969492,-0.447185940467556,-0.442501780583286,-0.414772155649295,
-0.386610545496204,-0.358667935404984,-0.344761744523387,-0.340663181383466,
-0.33625977614692,-0.307329116668616,-0.303043171878598,-0.275226622766843,
-0.2467812679575,-0.236972518209036,-0.232129158610577,-0.22829853363839,
-0.199315149750587,-0.169756960537854,-0.1399584553707,-0.123701275077245,
-0.118725825220484,-0.114410875346345,-0.0838707291517932,-0.05329158908994,
-0.0233203533939032,-0.00990101302306306,0.),.UNSPECIFIED.);
#5976=B_SPLINE_CURVE_WITH_KNOTS('',3,(#50810,#50811,#50812,#50813,#50814,
#50815,#50816,#50817,#50818,#50819,#50820,#50821,#50822,#50823,#50824,#50825,
#50826,#50827,#50828,#50829,#50830,#50831,#50832,#50833,#50834,#50835,#50836,
#50837,#50838,#50839,#50840,#50841,#50842,#50843,#50844,#50845,#50846,#50847,
#50848,#50849,#50850,#50851,#50852,#50853,#50854,#50855,#50856,#50857,#50858,
#50859,#50860,#50861,#50862,#50863,#50864,#50865,#50866,#50867,#50868,#50869,
#50870,#50871,#50872,#50873,#50874,#50875,#50876,#50877,#50878,#50879,#50880,
#50881,#50882,#50883,#50884,#50885,#50886,#50887,#50888,#50889,#50890,#50891,
#50892,#50893,#50894,#50895,#50896,#50897,#50898,#50899,#50900,#50901,#50902,
#50903),.UNSPECIFIED.,.F.,.F.,(4,3,3,3,3,3,3,3,3,3,3,3,3,3,3,3,3,3,3,3,
3,3,3,3,3,3,3,3,3,3,3,4),(-0.566847306048015,-0.536665862165872,-0.506059953424534,
-0.497416406509601,-0.49047962159474,-0.460332810086325,-0.437094434650949,
-0.424724933731654,-0.420483367445324,-0.391058514938839,-0.361900337854958,
-0.333575724322276,-0.318788244892536,-0.313125876579605,-0.308695952531969,
-0.280705563178002,-0.274425806603314,-0.245949103512341,-0.21622427305735,
-0.204597316412413,-0.200878698510381,-0.173045196304837,-0.145277260484532,
-0.117980535767822,-0.104251776280896,-0.100006100365259,-0.0958284117637648,
-0.0691557510171672,-0.0429305470482147,-0.0175053685433162,-0.00815045987241369,
0.),.UNSPECIFIED.);
#5977=B_SPLINE_CURVE_WITH_KNOTS('',3,(#50905,#50906,#50907,#50908,#50909,
#50910,#50911,#50912,#50913,#50914,#50915),.UNSPECIFIED.,.F.,.F.,(4,1,1,
1,1,1,1,1,4),(15.7079632679489,15.8286682231624,16.821088063376,17.8135079035896,
18.8059277438032,19.7983475840169,20.7907674242305,21.7831872644441,21.9911485751285),
 .UNSPECIFIED.);
#5978=B_SPLINE_CURVE_WITH_KNOTS('',3,(#50916,#50917,#50918,#50919,#50920,
#50921,#50922,#50923,#50924,#50925),.UNSPECIFIED.,.F.,.F.,(4,1,1,1,1,1,
1,4),(15.7079632679489,16.3832398073992,17.3756596476128,18.3680794878265,
19.3604993280401,20.3529191682537,21.3453390084674,21.9911485751284),
 .UNSPECIFIED.);
#5979=B_SPLINE_CURVE_WITH_KNOTS('',3,(#51326,#51327,#51328,#51329,#51330,
#51331,#51332,#51333,#51334,#51335,#51336,#51337,#51338,#51339,#51340,#51341,
#51342,#51343,#51344,#51345,#51346,#51347,#51348,#51349,#51350,#51351,#51352,
#51353,#51354,#51355,#51356,#51357,#51358,#51359,#51360,#51361,#51362,#51363,
#51364,#51365,#51366,#51367,#51368,#51369,#51370,#51371,#51372,#51373,#51374,
#51375,#51376,#51377,#51378,#51379,#51380,#51381,#51382,#51383,#51384,#51385,
#51386,#51387,#51388,#51389,#51390,#51391,#51392,#51393,#51394,#51395,#51396,
#51397,#51398,#51399,#51400,#51401,#51402,#51403,#51404,#51405,#51406,#51407,
#51408,#51409,#51410,#51411,#51412,#51413,#51414,#51415,#51416,#51417,#51418,
#51419),.UNSPECIFIED.,.F.,.F.,(4,3,3,3,3,3,3,3,3,3,3,3,3,3,3,3,3,3,3,3,
3,3,3,3,3,3,3,3,3,3,3,4),(0.,0.025363025950112,0.0513976226497874,0.0781462280595047,
0.0899194383261542,0.0966315939995796,0.10267802161317,0.129978487838588,
0.157730214208604,0.184644277138334,0.195932072228315,0.20301284472711,
0.207156655403901,0.236271560665714,0.265386465927526,0.293279271834944,
0.302554877553594,0.311292566193282,0.315704524166865,0.343817419216937,
0.372959123929272,0.402412672778162,0.413342465523867,0.422898831529328,
0.428117874467775,0.458184918270669,0.482885311860363,0.492048607647558,
0.498170307466128,0.528680781105472,0.556986492629444,0.566847306048072),
 .UNSPECIFIED.);
#5980=B_SPLINE_CURVE_WITH_KNOTS('',3,(#51420,#51421,#51422,#51423,#51424,
#51425,#51426,#51427,#51428,#51429,#51430,#51431,#51432,#51433,#51434,#51435,
#51436,#51437,#51438,#51439,#51440,#51441,#51442,#51443,#51444),
 .UNSPECIFIED.,.F.,.F.,(4,3,3,3,3,3,3,3,4),(-10.1321597128207,-9.92419840213633,
-8.93177856192269,-7.93935872170906,-6.94693888149543,-5.9545190412818,
-4.96209920106816,-3.96967936085453,-3.848974405641),.UNSPECIFIED.);
#5981=B_SPLINE_CURVE_WITH_KNOTS('',3,(#51845,#51846,#51847,#51848,#51849,
#51850,#51851,#51852,#51853,#51854,#51855,#51856,#51857,#51858,#51859,#51860,
#51861,#51862,#51863,#51864,#51865,#51866),.UNSPECIFIED.,.F.,.F.,(4,3,3,
3,3,3,3,4),(7.59274844815647,7.93935872170906,8.93177856192269,9.92419840213633,
10.91661824235,11.9090380825636,12.9014579227772,13.875933755336),
 .UNSPECIFIED.);
#5982=B_SPLINE_CURVE_WITH_KNOTS('',3,(#51867,#51868,#51869,#51870,#51871,
#51872,#51873,#51874,#51875,#51876,#51877,#51878,#51879,#51880,#51881,#51882,
#51883,#51884,#51885,#51886,#51887,#51888,#51889,#51890,#51891,#51892,#51893,
#51894,#51895,#51896,#51897,#51898,#51899,#51900,#51901,#51902,#51903,#51904,
#51905,#51906,#51907,#51908,#51909,#51910,#51911,#51912,#51913,#51914,#51915,
#51916,#51917,#51918,#51919,#51920,#51921,#51922,#51923,#51924,#51925,#51926,
#51927,#51928,#51929,#51930,#51931,#51932,#51933,#51934,#51935,#51936,#51937,
#51938,#51939,#51940,#51941,#51942,#51943,#51944,#51945,#51946,#51947,#51948,
#51949,#51950,#51951,#51952,#51953,#51954,#51955,#51956,#51957),
 .UNSPECIFIED.,.F.,.F.,(4,3,3,3,3,3,3,3,3,3,3,3,3,3,3,3,3,3,3,3,3,3,3,3,
3,3,3,3,3,3,4),(0.,0.0297240839681494,0.0601072325488629,0.0893395071884968,
0.114917747498176,0.120626859693154,0.150385989369229,0.179981400055904,
0.208477407458411,0.220429503756483,0.228738548934207,0.234134417028589,
0.264049923347261,0.291955958282,0.293965429665934,0.322911496989362,0.339206044992874,
0.343413984993647,0.371506228471583,0.399645181287735,0.42738181215757,
0.437705393049684,0.444698500099991,0.448877446256884,0.476925759914272,
0.497961995157314,0.506030983187008,0.511791121700786,0.537728941286451,
0.561070700886438,0.569248610399523),.UNSPECIFIED.);
#6667=LINE('',#32410,#7852);
#6668=LINE('',#32419,#7853);
#6669=LINE('',#32436,#7854);
#6670=LINE('',#32487,#7855);
#6671=LINE('',#32538,#7856);
#6672=LINE('',#32586,#7857);
#6673=LINE('',#32637,#7858);
#6674=LINE('',#32688,#7859);
#6675=LINE('',#32736,#7860);
#6676=LINE('',#32787,#7861);
#6677=LINE('',#32838,#7862);
#6678=LINE('',#32886,#7863);
#6679=LINE('',#32937,#7864);
#6680=LINE('',#32988,#7865);
#6681=LINE('',#33036,#7866);
#6682=LINE('',#33087,#7867);
#6683=LINE('',#33126,#7868);
#6684=LINE('',#33150,#7869);
#6685=LINE('',#33174,#7870);
#6686=LINE('',#33199,#7871);
#6687=LINE('',#33224,#7872);
#6688=LINE('',#33248,#7873);
#6689=LINE('',#33273,#7874);
#6690=LINE('',#33298,#7875);
#6691=LINE('',#33322,#7876);
#6692=LINE('',#33347,#7877);
#6693=LINE('',#33372,#7878);
#6694=LINE('',#33396,#7879);
#6695=LINE('',#33421,#7880);
#6696=LINE('',#33446,#7881);
#6697=LINE('',#33470,#7882);
#6698=LINE('',#33487,#7883);
#6699=LINE('',#33496,#7884);
#6700=LINE('',#33513,#7885);
#6701=LINE('',#33564,#7886);
#6702=LINE('',#33615,#7887);
#6703=LINE('',#33663,#7888);
#6704=LINE('',#33714,#7889);
#6705=LINE('',#33765,#7890);
#6706=LINE('',#33813,#7891);
#6707=LINE('',#33864,#7892);
#6708=LINE('',#33915,#7893);
#6709=LINE('',#33963,#7894);
#6710=LINE('',#34014,#7895);
#6711=LINE('',#34065,#7896);
#6712=LINE('',#34113,#7897);
#6713=LINE('',#34164,#7898);
#6714=LINE('',#34203,#7899);
#6715=LINE('',#34227,#7900);
#6716=LINE('',#34251,#7901);
#6717=LINE('',#34276,#7902);
#6718=LINE('',#34301,#7903);
#6719=LINE('',#34325,#7904);
#6720=LINE('',#34350,#7905);
#6721=LINE('',#34375,#7906);
#6722=LINE('',#34399,#7907);
#6723=LINE('',#34424,#7908);
#6724=LINE('',#34449,#7909);
#6725=LINE('',#34473,#7910);
#6726=LINE('',#34498,#7911);
#6727=LINE('',#34523,#7912);
#6728=LINE('',#34547,#7913);
#6729=LINE('',#34564,#7914);
#6730=LINE('',#34573,#7915);
#6731=LINE('',#34590,#7916);
#6732=LINE('',#34641,#7917);
#6733=LINE('',#34692,#7918);
#6734=LINE('',#34740,#7919);
#6735=LINE('',#34791,#7920);
#6736=LINE('',#34842,#7921);
#6737=LINE('',#34890,#7922);
#6738=LINE('',#34941,#7923);
#6739=LINE('',#34992,#7924);
#6740=LINE('',#35040,#7925);
#6741=LINE('',#35091,#7926);
#6742=LINE('',#35142,#7927);
#6743=LINE('',#35190,#7928);
#6744=LINE('',#35241,#7929);
#6745=LINE('',#35280,#7930);
#6746=LINE('',#35304,#7931);
#6747=LINE('',#35328,#7932);
#6748=LINE('',#35353,#7933);
#6749=LINE('',#35378,#7934);
#6750=LINE('',#35402,#7935);
#6751=LINE('',#35427,#7936);
#6752=LINE('',#35452,#7937);
#6753=LINE('',#35476,#7938);
#6754=LINE('',#35501,#7939);
#6755=LINE('',#35526,#7940);
#6756=LINE('',#35550,#7941);
#6757=LINE('',#35575,#7942);
#6758=LINE('',#35600,#7943);
#6759=LINE('',#35624,#7944);
#6760=LINE('',#35641,#7945);
#6761=LINE('',#35650,#7946);
#6762=LINE('',#35667,#7947);
#6763=LINE('',#35718,#7948);
#6764=LINE('',#35769,#7949);
#6765=LINE('',#35817,#7950);
#6766=LINE('',#35868,#7951);
#6767=LINE('',#35919,#7952);
#6768=LINE('',#35967,#7953);
#6769=LINE('',#36018,#7954);
#6770=LINE('',#36069,#7955);
#6771=LINE('',#36117,#7956);
#6772=LINE('',#36168,#7957);
#6773=LINE('',#36219,#7958);
#6774=LINE('',#36267,#7959);
#6775=LINE('',#36318,#7960);
#6776=LINE('',#36357,#7961);
#6777=LINE('',#36381,#7962);
#6778=LINE('',#36405,#7963);
#6779=LINE('',#36430,#7964);
#6780=LINE('',#36455,#7965);
#6781=LINE('',#36479,#7966);
#6782=LINE('',#36504,#7967);
#6783=LINE('',#36529,#7968);
#6784=LINE('',#36553,#7969);
#6785=LINE('',#36578,#7970);
#6786=LINE('',#36603,#7971);
#6787=LINE('',#36627,#7972);
#6788=LINE('',#36652,#7973);
#6789=LINE('',#36677,#7974);
#6790=LINE('',#36701,#7975);
#6791=LINE('',#36718,#7976);
#6792=LINE('',#36727,#7977);
#6793=LINE('',#36744,#7978);
#6794=LINE('',#36795,#7979);
#6795=LINE('',#36846,#7980);
#6796=LINE('',#36894,#7981);
#6797=LINE('',#36945,#7982);
#6798=LINE('',#36996,#7983);
#6799=LINE('',#37044,#7984);
#6800=LINE('',#37095,#7985);
#6801=LINE('',#37146,#7986);
#6802=LINE('',#37194,#7987);
#6803=LINE('',#37245,#7988);
#6804=LINE('',#37296,#7989);
#6805=LINE('',#37344,#7990);
#6806=LINE('',#37395,#7991);
#6807=LINE('',#37434,#7992);
#6808=LINE('',#37458,#7993);
#6809=LINE('',#37482,#7994);
#6810=LINE('',#37507,#7995);
#6811=LINE('',#37532,#7996);
#6812=LINE('',#37556,#7997);
#6813=LINE('',#37581,#7998);
#6814=LINE('',#37606,#7999);
#6815=LINE('',#37630,#8000);
#6816=LINE('',#37655,#8001);
#6817=LINE('',#37680,#8002);
#6818=LINE('',#37704,#8003);
#6819=LINE('',#37729,#8004);
#6820=LINE('',#37754,#8005);
#6821=LINE('',#37778,#8006);
#6822=LINE('',#37795,#8007);
#6823=LINE('',#37804,#8008);
#6824=LINE('',#37821,#8009);
#6825=LINE('',#37872,#8010);
#6826=LINE('',#37923,#8011);
#6827=LINE('',#37971,#8012);
#6828=LINE('',#38022,#8013);
#6829=LINE('',#38073,#8014);
#6830=LINE('',#38121,#8015);
#6831=LINE('',#38172,#8016);
#6832=LINE('',#38223,#8017);
#6833=LINE('',#38271,#8018);
#6834=LINE('',#38322,#8019);
#6835=LINE('',#38373,#8020);
#6836=LINE('',#38421,#8021);
#6837=LINE('',#38472,#8022);
#6838=LINE('',#38511,#8023);
#6839=LINE('',#38535,#8024);
#6840=LINE('',#38559,#8025);
#6841=LINE('',#38584,#8026);
#6842=LINE('',#38609,#8027);
#6843=LINE('',#38633,#8028);
#6844=LINE('',#38658,#8029);
#6845=LINE('',#38683,#8030);
#6846=LINE('',#38707,#8031);
#6847=LINE('',#38732,#8032);
#6848=LINE('',#38757,#8033);
#6849=LINE('',#38781,#8034);
#6850=LINE('',#38806,#8035);
#6851=LINE('',#38831,#8036);
#6852=LINE('',#38855,#8037);
#6853=LINE('',#38872,#8038);
#6854=LINE('',#38881,#8039);
#6855=LINE('',#38898,#8040);
#6856=LINE('',#38949,#8041);
#6857=LINE('',#39000,#8042);
#6858=LINE('',#39048,#8043);
#6859=LINE('',#39099,#8044);
#6860=LINE('',#39150,#8045);
#6861=LINE('',#39198,#8046);
#6862=LINE('',#39249,#8047);
#6863=LINE('',#39300,#8048);
#6864=LINE('',#39348,#8049);
#6865=LINE('',#39399,#8050);
#6866=LINE('',#39450,#8051);
#6867=LINE('',#39498,#8052);
#6868=LINE('',#39549,#8053);
#6869=LINE('',#39588,#8054);
#6870=LINE('',#39612,#8055);
#6871=LINE('',#39636,#8056);
#6872=LINE('',#39661,#8057);
#6873=LINE('',#39686,#8058);
#6874=LINE('',#39710,#8059);
#6875=LINE('',#39735,#8060);
#6876=LINE('',#39760,#8061);
#6877=LINE('',#39784,#8062);
#6878=LINE('',#39809,#8063);
#6879=LINE('',#39834,#8064);
#6880=LINE('',#39858,#8065);
#6881=LINE('',#39883,#8066);
#6882=LINE('',#39908,#8067);
#6883=LINE('',#39932,#8068);
#6884=LINE('',#39949,#8069);
#6885=LINE('',#39958,#8070);
#6886=LINE('',#39975,#8071);
#6887=LINE('',#40026,#8072);
#6888=LINE('',#40077,#8073);
#6889=LINE('',#40125,#8074);
#6890=LINE('',#40176,#8075);
#6891=LINE('',#40227,#8076);
#6892=LINE('',#40275,#8077);
#6893=LINE('',#40326,#8078);
#6894=LINE('',#40377,#8079);
#6895=LINE('',#40425,#8080);
#6896=LINE('',#40476,#8081);
#6897=LINE('',#40527,#8082);
#6898=LINE('',#40575,#8083);
#6899=LINE('',#40626,#8084);
#6900=LINE('',#40665,#8085);
#6901=LINE('',#40689,#8086);
#6902=LINE('',#40713,#8087);
#6903=LINE('',#40738,#8088);
#6904=LINE('',#40763,#8089);
#6905=LINE('',#40787,#8090);
#6906=LINE('',#40812,#8091);
#6907=LINE('',#40837,#8092);
#6908=LINE('',#40861,#8093);
#6909=LINE('',#40886,#8094);
#6910=LINE('',#40911,#8095);
#6911=LINE('',#40935,#8096);
#6912=LINE('',#40960,#8097);
#6913=LINE('',#40985,#8098);
#6914=LINE('',#41009,#8099);
#6915=LINE('',#41045,#8100);
#6916=LINE('',#41143,#8101);
#6917=LINE('',#41214,#8102);
#6918=LINE('',#41298,#8103);
#6919=LINE('',#41365,#8104);
#6920=LINE('',#41463,#8105);
#6921=LINE('',#41534,#8106);
#6922=LINE('',#41618,#8107);
#6923=LINE('',#41685,#8108);
#6924=LINE('',#41783,#8109);
#6925=LINE('',#41854,#8110);
#6926=LINE('',#41938,#8111);
#6927=LINE('',#51971,#8112);
#6928=LINE('',#51977,#8113);
#6929=LINE('',#51983,#8114);
#6930=LINE('',#51989,#8115);
#6931=LINE('',#51995,#8116);
#6932=LINE('',#52003,#8117);
#6933=LINE('',#52004,#8118);
#6934=LINE('',#52005,#8119);
#6935=LINE('',#52007,#8120);
#6936=LINE('',#52012,#8121);
#6937=LINE('',#52013,#8122);
#6938=LINE('',#52014,#8123);
#6939=LINE('',#52016,#8124);
#6940=LINE('',#52024,#8125);
#6941=LINE('',#52028,#8126);
#7852=VECTOR('',#27340,3.);
#7853=VECTOR('',#27343,3.);
#7854=VECTOR('',#27350,3.);
#7855=VECTOR('',#27353,3.);
#7856=VECTOR('',#27356,3.);
#7857=VECTOR('',#27359,3.);
#7858=VECTOR('',#27362,3.);
#7859=VECTOR('',#27365,3.);
#7860=VECTOR('',#27368,3.);
#7861=VECTOR('',#27371,3.);
#7862=VECTOR('',#27374,3.);
#7863=VECTOR('',#27377,3.);
#7864=VECTOR('',#27380,3.);
#7865=VECTOR('',#27383,3.);
#7866=VECTOR('',#27386,3.);
#7867=VECTOR('',#27389,3.);
#7868=VECTOR('',#27394,3.0735);
#7869=VECTOR('',#27399,3.0735);
#7870=VECTOR('',#27402,3.0735);
#7871=VECTOR('',#27405,3.0735);
#7872=VECTOR('',#27408,3.0735);
#7873=VECTOR('',#27411,3.0735);
#7874=VECTOR('',#27414,3.0735);
#7875=VECTOR('',#27417,3.0735);
#7876=VECTOR('',#27420,3.0735);
#7877=VECTOR('',#27423,3.0735);
#7878=VECTOR('',#27426,3.0735);
#7879=VECTOR('',#27429,3.0735);
#7880=VECTOR('',#27432,3.0735);
#7881=VECTOR('',#27435,3.0735);
#7882=VECTOR('',#27438,3.0735);
#7883=VECTOR('',#27443,3.);
#7884=VECTOR('',#27446,3.);
#7885=VECTOR('',#27453,3.);
#7886=VECTOR('',#27456,3.);
#7887=VECTOR('',#27459,3.);
#7888=VECTOR('',#27462,3.);
#7889=VECTOR('',#27465,3.);
#7890=VECTOR('',#27468,3.);
#7891=VECTOR('',#27471,3.);
#7892=VECTOR('',#27474,3.);
#7893=VECTOR('',#27477,3.);
#7894=VECTOR('',#27480,3.);
#7895=VECTOR('',#27483,3.);
#7896=VECTOR('',#27486,3.);
#7897=VECTOR('',#27489,3.);
#7898=VECTOR('',#27492,3.);
#7899=VECTOR('',#27497,3.0735);
#7900=VECTOR('',#27502,3.0735);
#7901=VECTOR('',#27505,3.0735);
#7902=VECTOR('',#27508,3.0735);
#7903=VECTOR('',#27511,3.0735);
#7904=VECTOR('',#27514,3.0735);
#7905=VECTOR('',#27517,3.0735);
#7906=VECTOR('',#27520,3.0735);
#7907=VECTOR('',#27523,3.0735);
#7908=VECTOR('',#27526,3.0735);
#7909=VECTOR('',#27529,3.0735);
#7910=VECTOR('',#27532,3.0735);
#7911=VECTOR('',#27535,3.0735);
#7912=VECTOR('',#27538,3.0735);
#7913=VECTOR('',#27541,3.0735);
#7914=VECTOR('',#27546,3.);
#7915=VECTOR('',#27549,3.);
#7916=VECTOR('',#27556,3.);
#7917=VECTOR('',#27559,3.);
#7918=VECTOR('',#27562,3.);
#7919=VECTOR('',#27565,3.);
#7920=VECTOR('',#27568,3.);
#7921=VECTOR('',#27571,3.);
#7922=VECTOR('',#27574,3.);
#7923=VECTOR('',#27577,3.);
#7924=VECTOR('',#27580,3.);
#7925=VECTOR('',#27583,3.);
#7926=VECTOR('',#27586,3.);
#7927=VECTOR('',#27589,3.);
#7928=VECTOR('',#27592,3.);
#7929=VECTOR('',#27595,3.);
#7930=VECTOR('',#27600,3.0735);
#7931=VECTOR('',#27605,3.0735);
#7932=VECTOR('',#27608,3.0735);
#7933=VECTOR('',#27611,3.0735);
#7934=VECTOR('',#27614,3.0735);
#7935=VECTOR('',#27617,3.0735);
#7936=VECTOR('',#27620,3.0735);
#7937=VECTOR('',#27623,3.0735);
#7938=VECTOR('',#27626,3.0735);
#7939=VECTOR('',#27629,3.0735);
#7940=VECTOR('',#27632,3.0735);
#7941=VECTOR('',#27635,3.0735);
#7942=VECTOR('',#27638,3.0735);
#7943=VECTOR('',#27641,3.0735);
#7944=VECTOR('',#27644,3.0735);
#7945=VECTOR('',#27649,3.);
#7946=VECTOR('',#27652,3.);
#7947=VECTOR('',#27659,3.);
#7948=VECTOR('',#27662,3.);
#7949=VECTOR('',#27665,3.);
#7950=VECTOR('',#27668,3.);
#7951=VECTOR('',#27671,3.);
#7952=VECTOR('',#27674,3.);
#7953=VECTOR('',#27677,3.);
#7954=VECTOR('',#27680,3.);
#7955=VECTOR('',#27683,3.);
#7956=VECTOR('',#27686,3.);
#7957=VECTOR('',#27689,3.);
#7958=VECTOR('',#27692,3.);
#7959=VECTOR('',#27695,3.);
#7960=VECTOR('',#27698,3.);
#7961=VECTOR('',#27703,3.0735);
#7962=VECTOR('',#27708,3.0735);
#7963=VECTOR('',#27711,3.0735);
#7964=VECTOR('',#27714,3.0735);
#7965=VECTOR('',#27717,3.0735);
#7966=VECTOR('',#27720,3.0735);
#7967=VECTOR('',#27723,3.0735);
#7968=VECTOR('',#27726,3.0735);
#7969=VECTOR('',#27729,3.0735);
#7970=VECTOR('',#27732,3.0735);
#7971=VECTOR('',#27735,3.0735);
#7972=VECTOR('',#27738,3.0735);
#7973=VECTOR('',#27741,3.0735);
#7974=VECTOR('',#27744,3.0735);
#7975=VECTOR('',#27747,3.0735);
#7976=VECTOR('',#27752,3.);
#7977=VECTOR('',#27755,3.);
#7978=VECTOR('',#27762,3.);
#7979=VECTOR('',#27765,3.);
#7980=VECTOR('',#27768,3.);
#7981=VECTOR('',#27771,3.);
#7982=VECTOR('',#27774,3.);
#7983=VECTOR('',#27777,3.);
#7984=VECTOR('',#27780,3.);
#7985=VECTOR('',#27783,3.);
#7986=VECTOR('',#27786,3.);
#7987=VECTOR('',#27789,3.);
#7988=VECTOR('',#27792,3.);
#7989=VECTOR('',#27795,3.);
#7990=VECTOR('',#27798,3.);
#7991=VECTOR('',#27801,3.);
#7992=VECTOR('',#27806,3.0735);
#7993=VECTOR('',#27811,3.0735);
#7994=VECTOR('',#27814,3.0735);
#7995=VECTOR('',#27817,3.0735);
#7996=VECTOR('',#27820,3.0735);
#7997=VECTOR('',#27823,3.0735);
#7998=VECTOR('',#27826,3.0735);
#7999=VECTOR('',#27829,3.0735);
#8000=VECTOR('',#27832,3.0735);
#8001=VECTOR('',#27835,3.0735);
#8002=VECTOR('',#27838,3.0735);
#8003=VECTOR('',#27841,3.0735);
#8004=VECTOR('',#27844,3.0735);
#8005=VECTOR('',#27847,3.0735);
#8006=VECTOR('',#27850,3.0735);
#8007=VECTOR('',#27855,3.);
#8008=VECTOR('',#27858,3.);
#8009=VECTOR('',#27865,3.);
#8010=VECTOR('',#27868,3.);
#8011=VECTOR('',#27871,3.);
#8012=VECTOR('',#27874,3.);
#8013=VECTOR('',#27877,3.);
#8014=VECTOR('',#27880,3.);
#8015=VECTOR('',#27883,3.);
#8016=VECTOR('',#27886,3.);
#8017=VECTOR('',#27889,3.);
#8018=VECTOR('',#27892,3.);
#8019=VECTOR('',#27895,3.);
#8020=VECTOR('',#27898,3.);
#8021=VECTOR('',#27901,3.);
#8022=VECTOR('',#27904,3.);
#8023=VECTOR('',#27909,3.0735);
#8024=VECTOR('',#27914,3.0735);
#8025=VECTOR('',#27917,3.0735);
#8026=VECTOR('',#27920,3.0735);
#8027=VECTOR('',#27923,3.0735);
#8028=VECTOR('',#27926,3.0735);
#8029=VECTOR('',#27929,3.0735);
#8030=VECTOR('',#27932,3.0735);
#8031=VECTOR('',#27935,3.0735);
#8032=VECTOR('',#27938,3.0735);
#8033=VECTOR('',#27941,3.0735);
#8034=VECTOR('',#27944,3.0735);
#8035=VECTOR('',#27947,3.0735);
#8036=VECTOR('',#27950,3.0735);
#8037=VECTOR('',#27953,3.0735);
#8038=VECTOR('',#27958,3.);
#8039=VECTOR('',#27961,3.);
#8040=VECTOR('',#27968,3.);
#8041=VECTOR('',#27971,3.);
#8042=VECTOR('',#27974,3.);
#8043=VECTOR('',#27977,3.);
#8044=VECTOR('',#27980,3.);
#8045=VECTOR('',#27983,3.);
#8046=VECTOR('',#27986,3.);
#8047=VECTOR('',#27989,3.);
#8048=VECTOR('',#27992,3.);
#8049=VECTOR('',#27995,3.);
#8050=VECTOR('',#27998,3.);
#8051=VECTOR('',#28001,3.);
#8052=VECTOR('',#28004,3.);
#8053=VECTOR('',#28007,3.);
#8054=VECTOR('',#28012,3.0735);
#8055=VECTOR('',#28017,3.0735);
#8056=VECTOR('',#28020,3.0735);
#8057=VECTOR('',#28023,3.0735);
#8058=VECTOR('',#28026,3.0735);
#8059=VECTOR('',#28029,3.0735);
#8060=VECTOR('',#28032,3.0735);
#8061=VECTOR('',#28035,3.0735);
#8062=VECTOR('',#28038,3.0735);
#8063=VECTOR('',#28041,3.0735);
#8064=VECTOR('',#28044,3.0735);
#8065=VECTOR('',#28047,3.0735);
#8066=VECTOR('',#28050,3.0735);
#8067=VECTOR('',#28053,3.0735);
#8068=VECTOR('',#28056,3.0735);
#8069=VECTOR('',#28061,3.);
#8070=VECTOR('',#28064,3.);
#8071=VECTOR('',#28071,3.);
#8072=VECTOR('',#28074,3.);
#8073=VECTOR('',#28077,3.);
#8074=VECTOR('',#28080,3.);
#8075=VECTOR('',#28083,3.);
#8076=VECTOR('',#28086,3.);
#8077=VECTOR('',#28089,3.);
#8078=VECTOR('',#28092,3.);
#8079=VECTOR('',#28095,3.);
#8080=VECTOR('',#28098,3.);
#8081=VECTOR('',#28101,3.);
#8082=VECTOR('',#28104,3.);
#8083=VECTOR('',#28107,3.);
#8084=VECTOR('',#28110,3.);
#8085=VECTOR('',#28115,3.0735);
#8086=VECTOR('',#28120,3.0735);
#8087=VECTOR('',#28123,3.0735);
#8088=VECTOR('',#28126,3.0735);
#8089=VECTOR('',#28129,3.0735);
#8090=VECTOR('',#28132,3.0735);
#8091=VECTOR('',#28135,3.0735);
#8092=VECTOR('',#28138,3.0735);
#8093=VECTOR('',#28141,3.0735);
#8094=VECTOR('',#28144,3.0735);
#8095=VECTOR('',#28147,3.0735);
#8096=VECTOR('',#28150,3.0735);
#8097=VECTOR('',#28153,3.0735);
#8098=VECTOR('',#28156,3.0735);
#8099=VECTOR('',#28159,3.0735);
#8100=VECTOR('',#28164,2.);
#8101=VECTOR('',#28167,2.);
#8102=VECTOR('',#28170,2.);
#8103=VECTOR('',#28173,2.);
#8104=VECTOR('',#28176,2.);
#8105=VECTOR('',#28179,2.);
#8106=VECTOR('',#28182,2.);
#8107=VECTOR('',#28185,2.);
#8108=VECTOR('',#28188,2.);
#8109=VECTOR('',#28191,2.);
#8110=VECTOR('',#28194,2.);
#8111=VECTOR('',#28197,2.);
#8112=VECTOR('',#28266,5.5);
#8113=VECTOR('',#28273,5.5);
#8114=VECTOR('',#28280,5.5);
#8115=VECTOR('',#28287,5.5);
#8116=VECTOR('',#28294,18.);
#8117=VECTOR('',#28305,90.);
#8118=VECTOR('',#28306,90.);
#8119=VECTOR('',#28307,90.);
#8120=VECTOR('',#28308,90.);
#8121=VECTOR('',#28315,100.);
#8122=VECTOR('',#28316,100.);
#8123=VECTOR('',#28317,100.);
#8124=VECTOR('',#28318,100.);
#8125=VECTOR('',#28329,17.);
#8126=VECTOR('',#28334,130.);
#9037=VERTEX_POINT('',#32408);
#9038=VERTEX_POINT('',#32409);
#9039=VERTEX_POINT('',#32411);
#9040=VERTEX_POINT('',#32416);
#9041=VERTEX_POINT('',#32418);
#9042=VERTEX_POINT('',#32421);
#9043=VERTEX_POINT('',#32434);
#9044=VERTEX_POINT('',#32435);
#9045=VERTEX_POINT('',#32485);
#9046=VERTEX_POINT('',#32486);
#9047=VERTEX_POINT('',#32536);
#9048=VERTEX_POINT('',#32537);
#9049=VERTEX_POINT('',#32584);
#9050=VERTEX_POINT('',#32585);
#9051=VERTEX_POINT('',#32635);
#9052=VERTEX_POINT('',#32636);
#9053=VERTEX_POINT('',#32686);
#9054=VERTEX_POINT('',#32687);
#9055=VERTEX_POINT('',#32734);
#9056=VERTEX_POINT('',#32735);
#9057=VERTEX_POINT('',#32785);
#9058=VERTEX_POINT('',#32786);
#9059=VERTEX_POINT('',#32836);
#9060=VERTEX_POINT('',#32837);
#9061=VERTEX_POINT('',#32884);
#9062=VERTEX_POINT('',#32885);
#9063=VERTEX_POINT('',#32935);
#9064=VERTEX_POINT('',#32936);
#9065=VERTEX_POINT('',#32986);
#9066=VERTEX_POINT('',#32987);
#9067=VERTEX_POINT('',#33034);
#9068=VERTEX_POINT('',#33035);
#9069=VERTEX_POINT('',#33085);
#9070=VERTEX_POINT('',#33086);
#9071=VERTEX_POINT('',#33088);
#9072=VERTEX_POINT('',#33102);
#9073=VERTEX_POINT('',#33124);
#9074=VERTEX_POINT('',#33125);
#9075=VERTEX_POINT('',#33127);
#9076=VERTEX_POINT('',#33136);
#9077=VERTEX_POINT('',#33148);
#9078=VERTEX_POINT('',#33149);
#9079=VERTEX_POINT('',#33172);
#9080=VERTEX_POINT('',#33173);
#9081=VERTEX_POINT('',#33197);
#9082=VERTEX_POINT('',#33198);
#9083=VERTEX_POINT('',#33222);
#9084=VERTEX_POINT('',#33223);
#9085=VERTEX_POINT('',#33246);
#9086=VERTEX_POINT('',#33247);
#9087=VERTEX_POINT('',#33271);
#9088=VERTEX_POINT('',#33272);
#9089=VERTEX_POINT('',#33296);
#9090=VERTEX_POINT('',#33297);
#9091=VERTEX_POINT('',#33320);
#9092=VERTEX_POINT('',#33321);
#9093=VERTEX_POINT('',#33345);
#9094=VERTEX_POINT('',#33346);
#9095=VERTEX_POINT('',#33370);
#9096=VERTEX_POINT('',#33371);
#9097=VERTEX_POINT('',#33394);
#9098=VERTEX_POINT('',#33395);
#9099=VERTEX_POINT('',#33419);
#9100=VERTEX_POINT('',#33420);
#9101=VERTEX_POINT('',#33444);
#9102=VERTEX_POINT('',#33445);
#9103=VERTEX_POINT('',#33468);
#9104=VERTEX_POINT('',#33469);
#9105=VERTEX_POINT('',#33471);
#9106=VERTEX_POINT('',#33477);
#9107=VERTEX_POINT('',#33485);
#9108=VERTEX_POINT('',#33486);
#9109=VERTEX_POINT('',#33488);
#9110=VERTEX_POINT('',#33493);
#9111=VERTEX_POINT('',#33495);
#9112=VERTEX_POINT('',#33498);
#9113=VERTEX_POINT('',#33511);
#9114=VERTEX_POINT('',#33512);
#9115=VERTEX_POINT('',#33562);
#9116=VERTEX_POINT('',#33563);
#9117=VERTEX_POINT('',#33613);
#9118=VERTEX_POINT('',#33614);
#9119=VERTEX_POINT('',#33661);
#9120=VERTEX_POINT('',#33662);
#9121=VERTEX_POINT('',#33712);
#9122=VERTEX_POINT('',#33713);
#9123=VERTEX_POINT('',#33763);
#9124=VERTEX_POINT('',#33764);
#9125=VERTEX_POINT('',#33811);
#9126=VERTEX_POINT('',#33812);
#9127=VERTEX_POINT('',#33862);
#9128=VERTEX_POINT('',#33863);
#9129=VERTEX_POINT('',#33913);
#9130=VERTEX_POINT('',#33914);
#9131=VERTEX_POINT('',#33961);
#9132=VERTEX_POINT('',#33962);
#9133=VERTEX_POINT('',#34012);
#9134=VERTEX_POINT('',#34013);
#9135=VERTEX_POINT('',#34063);
#9136=VERTEX_POINT('',#34064);
#9137=VERTEX_POINT('',#34111);
#9138=VERTEX_POINT('',#34112);
#9139=VERTEX_POINT('',#34162);
#9140=VERTEX_POINT('',#34163);
#9141=VERTEX_POINT('',#34165);
#9142=VERTEX_POINT('',#34179);
#9143=VERTEX_POINT('',#34201);
#9144=VERTEX_POINT('',#34202);
#9145=VERTEX_POINT('',#34204);
#9146=VERTEX_POINT('',#34213);
#9147=VERTEX_POINT('',#34225);
#9148=VERTEX_POINT('',#34226);
#9149=VERTEX_POINT('',#34249);
#9150=VERTEX_POINT('',#34250);
#9151=VERTEX_POINT('',#34274);
#9152=VERTEX_POINT('',#34275);
#9153=VERTEX_POINT('',#34299);
#9154=VERTEX_POINT('',#34300);
#9155=VERTEX_POINT('',#34323);
#9156=VERTEX_POINT('',#34324);
#9157=VERTEX_POINT('',#34348);
#9158=VERTEX_POINT('',#34349);
#9159=VERTEX_POINT('',#34373);
#9160=VERTEX_POINT('',#34374);
#9161=VERTEX_POINT('',#34397);
#9162=VERTEX_POINT('',#34398);
#9163=VERTEX_POINT('',#34422);
#9164=VERTEX_POINT('',#34423);
#9165=VERTEX_POINT('',#34447);
#9166=VERTEX_POINT('',#34448);
#9167=VERTEX_POINT('',#34471);
#9168=VERTEX_POINT('',#34472);
#9169=VERTEX_POINT('',#34496);
#9170=VERTEX_POINT('',#34497);
#9171=VERTEX_POINT('',#34521);
#9172=VERTEX_POINT('',#34522);
#9173=VERTEX_POINT('',#34545);
#9174=VERTEX_POINT('',#34546);
#9175=VERTEX_POINT('',#34548);
#9176=VERTEX_POINT('',#34554);
#9177=VERTEX_POINT('',#34562);
#9178=VERTEX_POINT('',#34563);
#9179=VERTEX_POINT('',#34565);
#9180=VERTEX_POINT('',#34570);
#9181=VERTEX_POINT('',#34572);
#9182=VERTEX_POINT('',#34575);
#9183=VERTEX_POINT('',#34588);
#9184=VERTEX_POINT('',#34589);
#9185=VERTEX_POINT('',#34639);
#9186=VERTEX_POINT('',#34640);
#9187=VERTEX_POINT('',#34690);
#9188=VERTEX_POINT('',#34691);
#9189=VERTEX_POINT('',#34738);
#9190=VERTEX_POINT('',#34739);
#9191=VERTEX_POINT('',#34789);
#9192=VERTEX_POINT('',#34790);
#9193=VERTEX_POINT('',#34840);
#9194=VERTEX_POINT('',#34841);
#9195=VERTEX_POINT('',#34888);
#9196=VERTEX_POINT('',#34889);
#9197=VERTEX_POINT('',#34939);
#9198=VERTEX_POINT('',#34940);
#9199=VERTEX_POINT('',#34990);
#9200=VERTEX_POINT('',#34991);
#9201=VERTEX_POINT('',#35038);
#9202=VERTEX_POINT('',#35039);
#9203=VERTEX_POINT('',#35089);
#9204=VERTEX_POINT('',#35090);
#9205=VERTEX_POINT('',#35140);
#9206=VERTEX_POINT('',#35141);
#9207=VERTEX_POINT('',#35188);
#9208=VERTEX_POINT('',#35189);
#9209=VERTEX_POINT('',#35239);
#9210=VERTEX_POINT('',#35240);
#9211=VERTEX_POINT('',#35242);
#9212=VERTEX_POINT('',#35256);
#9213=VERTEX_POINT('',#35278);
#9214=VERTEX_POINT('',#35279);
#9215=VERTEX_POINT('',#35281);
#9216=VERTEX_POINT('',#35290);
#9217=VERTEX_POINT('',#35302);
#9218=VERTEX_POINT('',#35303);
#9219=VERTEX_POINT('',#35326);
#9220=VERTEX_POINT('',#35327);
#9221=VERTEX_POINT('',#35351);
#9222=VERTEX_POINT('',#35352);
#9223=VERTEX_POINT('',#35376);
#9224=VERTEX_POINT('',#35377);
#9225=VERTEX_POINT('',#35400);
#9226=VERTEX_POINT('',#35401);
#9227=VERTEX_POINT('',#35425);
#9228=VERTEX_POINT('',#35426);
#9229=VERTEX_POINT('',#35450);
#9230=VERTEX_POINT('',#35451);
#9231=VERTEX_POINT('',#35474);
#9232=VERTEX_POINT('',#35475);
#9233=VERTEX_POINT('',#35499);
#9234=VERTEX_POINT('',#35500);
#9235=VERTEX_POINT('',#35524);
#9236=VERTEX_POINT('',#35525);
#9237=VERTEX_POINT('',#35548);
#9238=VERTEX_POINT('',#35549);
#9239=VERTEX_POINT('',#35573);
#9240=VERTEX_POINT('',#35574);
#9241=VERTEX_POINT('',#35598);
#9242=VERTEX_POINT('',#35599);
#9243=VERTEX_POINT('',#35622);
#9244=VERTEX_POINT('',#35623);
#9245=VERTEX_POINT('',#35625);
#9246=VERTEX_POINT('',#35631);
#9247=VERTEX_POINT('',#35639);
#9248=VERTEX_POINT('',#35640);
#9249=VERTEX_POINT('',#35642);
#9250=VERTEX_POINT('',#35647);
#9251=VERTEX_POINT('',#35649);
#9252=VERTEX_POINT('',#35652);
#9253=VERTEX_POINT('',#35665);
#9254=VERTEX_POINT('',#35666);
#9255=VERTEX_POINT('',#35716);
#9256=VERTEX_POINT('',#35717);
#9257=VERTEX_POINT('',#35767);
#9258=VERTEX_POINT('',#35768);
#9259=VERTEX_POINT('',#35815);
#9260=VERTEX_POINT('',#35816);
#9261=VERTEX_POINT('',#35866);
#9262=VERTEX_POINT('',#35867);
#9263=VERTEX_POINT('',#35917);
#9264=VERTEX_POINT('',#35918);
#9265=VERTEX_POINT('',#35965);
#9266=VERTEX_POINT('',#35966);
#9267=VERTEX_POINT('',#36016);
#9268=VERTEX_POINT('',#36017);
#9269=VERTEX_POINT('',#36067);
#9270=VERTEX_POINT('',#36068);
#9271=VERTEX_POINT('',#36115);
#9272=VERTEX_POINT('',#36116);
#9273=VERTEX_POINT('',#36166);
#9274=VERTEX_POINT('',#36167);
#9275=VERTEX_POINT('',#36217);
#9276=VERTEX_POINT('',#36218);
#9277=VERTEX_POINT('',#36265);
#9278=VERTEX_POINT('',#36266);
#9279=VERTEX_POINT('',#36316);
#9280=VERTEX_POINT('',#36317);
#9281=VERTEX_POINT('',#36319);
#9282=VERTEX_POINT('',#36333);
#9283=VERTEX_POINT('',#36355);
#9284=VERTEX_POINT('',#36356);
#9285=VERTEX_POINT('',#36358);
#9286=VERTEX_POINT('',#36367);
#9287=VERTEX_POINT('',#36379);
#9288=VERTEX_POINT('',#36380);
#9289=VERTEX_POINT('',#36403);
#9290=VERTEX_POINT('',#36404);
#9291=VERTEX_POINT('',#36428);
#9292=VERTEX_POINT('',#36429);
#9293=VERTEX_POINT('',#36453);
#9294=VERTEX_POINT('',#36454);
#9295=VERTEX_POINT('',#36477);
#9296=VERTEX_POINT('',#36478);
#9297=VERTEX_POINT('',#36502);
#9298=VERTEX_POINT('',#36503);
#9299=VERTEX_POINT('',#36527);
#9300=VERTEX_POINT('',#36528);
#9301=VERTEX_POINT('',#36551);
#9302=VERTEX_POINT('',#36552);
#9303=VERTEX_POINT('',#36576);
#9304=VERTEX_POINT('',#36577);
#9305=VERTEX_POINT('',#36601);
#9306=VERTEX_POINT('',#36602);
#9307=VERTEX_POINT('',#36625);
#9308=VERTEX_POINT('',#36626);
#9309=VERTEX_POINT('',#36650);
#9310=VERTEX_POINT('',#36651);
#9311=VERTEX_POINT('',#36675);
#9312=VERTEX_POINT('',#36676);
#9313=VERTEX_POINT('',#36699);
#9314=VERTEX_POINT('',#36700);
#9315=VERTEX_POINT('',#36702);
#9316=VERTEX_POINT('',#36708);
#9317=VERTEX_POINT('',#36716);
#9318=VERTEX_POINT('',#36717);
#9319=VERTEX_POINT('',#36719);
#9320=VERTEX_POINT('',#36724);
#9321=VERTEX_POINT('',#36726);
#9322=VERTEX_POINT('',#36729);
#9323=VERTEX_POINT('',#36742);
#9324=VERTEX_POINT('',#36743);
#9325=VERTEX_POINT('',#36793);
#9326=VERTEX_POINT('',#36794);
#9327=VERTEX_POINT('',#36844);
#9328=VERTEX_POINT('',#36845);
#9329=VERTEX_POINT('',#36892);
#9330=VERTEX_POINT('',#36893);
#9331=VERTEX_POINT('',#36943);
#9332=VERTEX_POINT('',#36944);
#9333=VERTEX_POINT('',#36994);
#9334=VERTEX_POINT('',#36995);
#9335=VERTEX_POINT('',#37042);
#9336=VERTEX_POINT('',#37043);
#9337=VERTEX_POINT('',#37093);
#9338=VERTEX_POINT('',#37094);
#9339=VERTEX_POINT('',#37144);
#9340=VERTEX_POINT('',#37145);
#9341=VERTEX_POINT('',#37192);
#9342=VERTEX_POINT('',#37193);
#9343=VERTEX_POINT('',#37243);
#9344=VERTEX_POINT('',#37244);
#9345=VERTEX_POINT('',#37294);
#9346=VERTEX_POINT('',#37295);
#9347=VERTEX_POINT('',#37342);
#9348=VERTEX_POINT('',#37343);
#9349=VERTEX_POINT('',#37393);
#9350=VERTEX_POINT('',#37394);
#9351=VERTEX_POINT('',#37396);
#9352=VERTEX_POINT('',#37410);
#9353=VERTEX_POINT('',#37432);
#9354=VERTEX_POINT('',#37433);
#9355=VERTEX_POINT('',#37435);
#9356=VERTEX_POINT('',#37444);
#9357=VERTEX_POINT('',#37456);
#9358=VERTEX_POINT('',#37457);
#9359=VERTEX_POINT('',#37480);
#9360=VERTEX_POINT('',#37481);
#9361=VERTEX_POINT('',#37505);
#9362=VERTEX_POINT('',#37506);
#9363=VERTEX_POINT('',#37530);
#9364=VERTEX_POINT('',#37531);
#9365=VERTEX_POINT('',#37554);
#9366=VERTEX_POINT('',#37555);
#9367=VERTEX_POINT('',#37579);
#9368=VERTEX_POINT('',#37580);
#9369=VERTEX_POINT('',#37604);
#9370=VERTEX_POINT('',#37605);
#9371=VERTEX_POINT('',#37628);
#9372=VERTEX_POINT('',#37629);
#9373=VERTEX_POINT('',#37653);
#9374=VERTEX_POINT('',#37654);
#9375=VERTEX_POINT('',#37678);
#9376=VERTEX_POINT('',#37679);
#9377=VERTEX_POINT('',#37702);
#9378=VERTEX_POINT('',#37703);
#9379=VERTEX_POINT('',#37727);
#9380=VERTEX_POINT('',#37728);
#9381=VERTEX_POINT('',#37752);
#9382=VERTEX_POINT('',#37753);
#9383=VERTEX_POINT('',#37776);
#9384=VERTEX_POINT('',#37777);
#9385=VERTEX_POINT('',#37779);
#9386=VERTEX_POINT('',#37785);
#9387=VERTEX_POINT('',#37793);
#9388=VERTEX_POINT('',#37794);
#9389=VERTEX_POINT('',#37796);
#9390=VERTEX_POINT('',#37801);
#9391=VERTEX_POINT('',#37803);
#9392=VERTEX_POINT('',#37806);
#9393=VERTEX_POINT('',#37819);
#9394=VERTEX_POINT('',#37820);
#9395=VERTEX_POINT('',#37870);
#9396=VERTEX_POINT('',#37871);
#9397=VERTEX_POINT('',#37921);
#9398=VERTEX_POINT('',#37922);
#9399=VERTEX_POINT('',#37969);
#9400=VERTEX_POINT('',#37970);
#9401=VERTEX_POINT('',#38020);
#9402=VERTEX_POINT('',#38021);
#9403=VERTEX_POINT('',#38071);
#9404=VERTEX_POINT('',#38072);
#9405=VERTEX_POINT('',#38119);
#9406=VERTEX_POINT('',#38120);
#9407=VERTEX_POINT('',#38170);
#9408=VERTEX_POINT('',#38171);
#9409=VERTEX_POINT('',#38221);
#9410=VERTEX_POINT('',#38222);
#9411=VERTEX_POINT('',#38269);
#9412=VERTEX_POINT('',#38270);
#9413=VERTEX_POINT('',#38320);
#9414=VERTEX_POINT('',#38321);
#9415=VERTEX_POINT('',#38371);
#9416=VERTEX_POINT('',#38372);
#9417=VERTEX_POINT('',#38419);
#9418=VERTEX_POINT('',#38420);
#9419=VERTEX_POINT('',#38470);
#9420=VERTEX_POINT('',#38471);
#9421=VERTEX_POINT('',#38473);
#9422=VERTEX_POINT('',#38487);
#9423=VERTEX_POINT('',#38509);
#9424=VERTEX_POINT('',#38510);
#9425=VERTEX_POINT('',#38512);
#9426=VERTEX_POINT('',#38521);
#9427=VERTEX_POINT('',#38533);
#9428=VERTEX_POINT('',#38534);
#9429=VERTEX_POINT('',#38557);
#9430=VERTEX_POINT('',#38558);
#9431=VERTEX_POINT('',#38582);
#9432=VERTEX_POINT('',#38583);
#9433=VERTEX_POINT('',#38607);
#9434=VERTEX_POINT('',#38608);
#9435=VERTEX_POINT('',#38631);
#9436=VERTEX_POINT('',#38632);
#9437=VERTEX_POINT('',#38656);
#9438=VERTEX_POINT('',#38657);
#9439=VERTEX_POINT('',#38681);
#9440=VERTEX_POINT('',#38682);
#9441=VERTEX_POINT('',#38705);
#9442=VERTEX_POINT('',#38706);
#9443=VERTEX_POINT('',#38730);
#9444=VERTEX_POINT('',#38731);
#9445=VERTEX_POINT('',#38755);
#9446=VERTEX_POINT('',#38756);
#9447=VERTEX_POINT('',#38779);
#9448=VERTEX_POINT('',#38780);
#9449=VERTEX_POINT('',#38804);
#9450=VERTEX_POINT('',#38805);
#9451=VERTEX_POINT('',#38829);
#9452=VERTEX_POINT('',#38830);
#9453=VERTEX_POINT('',#38853);
#9454=VERTEX_POINT('',#38854);
#9455=VERTEX_POINT('',#38856);
#9456=VERTEX_POINT('',#38862);
#9457=VERTEX_POINT('',#38870);
#9458=VERTEX_POINT('',#38871);
#9459=VERTEX_POINT('',#38873);
#9460=VERTEX_POINT('',#38878);
#9461=VERTEX_POINT('',#38880);
#9462=VERTEX_POINT('',#38883);
#9463=VERTEX_POINT('',#38896);
#9464=VERTEX_POINT('',#38897);
#9465=VERTEX_POINT('',#38947);
#9466=VERTEX_POINT('',#38948);
#9467=VERTEX_POINT('',#38998);
#9468=VERTEX_POINT('',#38999);
#9469=VERTEX_POINT('',#39046);
#9470=VERTEX_POINT('',#39047);
#9471=VERTEX_POINT('',#39097);
#9472=VERTEX_POINT('',#39098);
#9473=VERTEX_POINT('',#39148);
#9474=VERTEX_POINT('',#39149);
#9475=VERTEX_POINT('',#39196);
#9476=VERTEX_POINT('',#39197);
#9477=VERTEX_POINT('',#39247);
#9478=VERTEX_POINT('',#39248);
#9479=VERTEX_POINT('',#39298);
#9480=VERTEX_POINT('',#39299);
#9481=VERTEX_POINT('',#39346);
#9482=VERTEX_POINT('',#39347);
#9483=VERTEX_POINT('',#39397);
#9484=VERTEX_POINT('',#39398);
#9485=VERTEX_POINT('',#39448);
#9486=VERTEX_POINT('',#39449);
#9487=VERTEX_POINT('',#39496);
#9488=VERTEX_POINT('',#39497);
#9489=VERTEX_POINT('',#39547);
#9490=VERTEX_POINT('',#39548);
#9491=VERTEX_POINT('',#39550);
#9492=VERTEX_POINT('',#39564);
#9493=VERTEX_POINT('',#39586);
#9494=VERTEX_POINT('',#39587);
#9495=VERTEX_POINT('',#39589);
#9496=VERTEX_POINT('',#39598);
#9497=VERTEX_POINT('',#39610);
#9498=VERTEX_POINT('',#39611);
#9499=VERTEX_POINT('',#39634);
#9500=VERTEX_POINT('',#39635);
#9501=VERTEX_POINT('',#39659);
#9502=VERTEX_POINT('',#39660);
#9503=VERTEX_POINT('',#39684);
#9504=VERTEX_POINT('',#39685);
#9505=VERTEX_POINT('',#39708);
#9506=VERTEX_POINT('',#39709);
#9507=VERTEX_POINT('',#39733);
#9508=VERTEX_POINT('',#39734);
#9509=VERTEX_POINT('',#39758);
#9510=VERTEX_POINT('',#39759);
#9511=VERTEX_POINT('',#39782);
#9512=VERTEX_POINT('',#39783);
#9513=VERTEX_POINT('',#39807);
#9514=VERTEX_POINT('',#39808);
#9515=VERTEX_POINT('',#39832);
#9516=VERTEX_POINT('',#39833);
#9517=VERTEX_POINT('',#39856);
#9518=VERTEX_POINT('',#39857);
#9519=VERTEX_POINT('',#39881);
#9520=VERTEX_POINT('',#39882);
#9521=VERTEX_POINT('',#39906);
#9522=VERTEX_POINT('',#39907);
#9523=VERTEX_POINT('',#39930);
#9524=VERTEX_POINT('',#39931);
#9525=VERTEX_POINT('',#39933);
#9526=VERTEX_POINT('',#39939);
#9527=VERTEX_POINT('',#39947);
#9528=VERTEX_POINT('',#39948);
#9529=VERTEX_POINT('',#39950);
#9530=VERTEX_POINT('',#39955);
#9531=VERTEX_POINT('',#39957);
#9532=VERTEX_POINT('',#39960);
#9533=VERTEX_POINT('',#39973);
#9534=VERTEX_POINT('',#39974);
#9535=VERTEX_POINT('',#40024);
#9536=VERTEX_POINT('',#40025);
#9537=VERTEX_POINT('',#40075);
#9538=VERTEX_POINT('',#40076);
#9539=VERTEX_POINT('',#40123);
#9540=VERTEX_POINT('',#40124);
#9541=VERTEX_POINT('',#40174);
#9542=VERTEX_POINT('',#40175);
#9543=VERTEX_POINT('',#40225);
#9544=VERTEX_POINT('',#40226);
#9545=VERTEX_POINT('',#40273);
#9546=VERTEX_POINT('',#40274);
#9547=VERTEX_POINT('',#40324);
#9548=VERTEX_POINT('',#40325);
#9549=VERTEX_POINT('',#40375);
#9550=VERTEX_POINT('',#40376);
#9551=VERTEX_POINT('',#40423);
#9552=VERTEX_POINT('',#40424);
#9553=VERTEX_POINT('',#40474);
#9554=VERTEX_POINT('',#40475);
#9555=VERTEX_POINT('',#40525);
#9556=VERTEX_POINT('',#40526);
#9557=VERTEX_POINT('',#40573);
#9558=VERTEX_POINT('',#40574);
#9559=VERTEX_POINT('',#40624);
#9560=VERTEX_POINT('',#40625);
#9561=VERTEX_POINT('',#40627);
#9562=VERTEX_POINT('',#40641);
#9563=VERTEX_POINT('',#40663);
#9564=VERTEX_POINT('',#40664);
#9565=VERTEX_POINT('',#40666);
#9566=VERTEX_POINT('',#40675);
#9567=VERTEX_POINT('',#40687);
#9568=VERTEX_POINT('',#40688);
#9569=VERTEX_POINT('',#40711);
#9570=VERTEX_POINT('',#40712);
#9571=VERTEX_POINT('',#40736);
#9572=VERTEX_POINT('',#40737);
#9573=VERTEX_POINT('',#40761);
#9574=VERTEX_POINT('',#40762);
#9575=VERTEX_POINT('',#40785);
#9576=VERTEX_POINT('',#40786);
#9577=VERTEX_POINT('',#40810);
#9578=VERTEX_POINT('',#40811);
#9579=VERTEX_POINT('',#40835);
#9580=VERTEX_POINT('',#40836);
#9581=VERTEX_POINT('',#40859);
#9582=VERTEX_POINT('',#40860);
#9583=VERTEX_POINT('',#40884);
#9584=VERTEX_POINT('',#40885);
#9585=VERTEX_POINT('',#40909);
#9586=VERTEX_POINT('',#40910);
#9587=VERTEX_POINT('',#40933);
#9588=VERTEX_POINT('',#40934);
#9589=VERTEX_POINT('',#40958);
#9590=VERTEX_POINT('',#40959);
#9591=VERTEX_POINT('',#40983);
#9592=VERTEX_POINT('',#40984);
#9593=VERTEX_POINT('',#41007);
#9594=VERTEX_POINT('',#41008);
#9595=VERTEX_POINT('',#41010);
#9596=VERTEX_POINT('',#41016);
#9597=VERTEX_POINT('',#41024);
#9598=VERTEX_POINT('',#41025);
#9599=VERTEX_POINT('',#41044);
#9600=VERTEX_POINT('',#41046);
#9601=VERTEX_POINT('',#41103);
#9602=VERTEX_POINT('',#41104);
#9603=VERTEX_POINT('',#41142);
#9604=VERTEX_POINT('',#41144);
#9605=VERTEX_POINT('',#41182);
#9606=VERTEX_POINT('',#41183);
#9607=VERTEX_POINT('',#41202);
#9608=VERTEX_POINT('',#41213);
#9609=VERTEX_POINT('',#41215);
#9610=VERTEX_POINT('',#41226);
#9611=VERTEX_POINT('',#41266);
#9612=VERTEX_POINT('',#41267);
#9613=VERTEX_POINT('',#41286);
#9614=VERTEX_POINT('',#41297);
#9615=VERTEX_POINT('',#41344);
#9616=VERTEX_POINT('',#41345);
#9617=VERTEX_POINT('',#41364);
#9618=VERTEX_POINT('',#41366);
#9619=VERTEX_POINT('',#41423);
#9620=VERTEX_POINT('',#41424);
#9621=VERTEX_POINT('',#41462);
#9622=VERTEX_POINT('',#41464);
#9623=VERTEX_POINT('',#41502);
#9624=VERTEX_POINT('',#41503);
#9625=VERTEX_POINT('',#41522);
#9626=VERTEX_POINT('',#41533);
#9627=VERTEX_POINT('',#41535);
#9628=VERTEX_POINT('',#41546);
#9629=VERTEX_POINT('',#41586);
#9630=VERTEX_POINT('',#41587);
#9631=VERTEX_POINT('',#41606);
#9632=VERTEX_POINT('',#41617);
#9633=VERTEX_POINT('',#41664);
#9634=VERTEX_POINT('',#41665);
#9635=VERTEX_POINT('',#41684);
#9636=VERTEX_POINT('',#41686);
#9637=VERTEX_POINT('',#41743);
#9638=VERTEX_POINT('',#41744);
#9639=VERTEX_POINT('',#41782);
#9640=VERTEX_POINT('',#41784);
#9641=VERTEX_POINT('',#41822);
#9642=VERTEX_POINT('',#41823);
#9643=VERTEX_POINT('',#41842);
#9644=VERTEX_POINT('',#41853);
#9645=VERTEX_POINT('',#41855);
#9646=VERTEX_POINT('',#41866);
#9647=VERTEX_POINT('',#41906);
#9648=VERTEX_POINT('',#41907);
#9649=VERTEX_POINT('',#41926);
#9650=VERTEX_POINT('',#41937);
#9651=VERTEX_POINT('',#51968);
#9652=VERTEX_POINT('',#51970);
#9653=VERTEX_POINT('',#51974);
#9654=VERTEX_POINT('',#51976);
#9655=VERTEX_POINT('',#51980);
#9656=VERTEX_POINT('',#51982);
#9657=VERTEX_POINT('',#51986);
#9658=VERTEX_POINT('',#51988);
#9659=VERTEX_POINT('',#51992);
#9660=VERTEX_POINT('',#51994);
#9661=VERTEX_POINT('',#51998);
#9662=VERTEX_POINT('',#52001);
#9663=VERTEX_POINT('',#52006);
#9664=VERTEX_POINT('',#52010);
#9665=VERTEX_POINT('',#52015);
#9666=VERTEX_POINT('',#52020);
#9667=VERTEX_POINT('',#52023);
#9668=VERTEX_POINT('',#52027);
#11597=EDGE_CURVE('',#9037,#9038,#6667,.T.);
#11598=EDGE_CURVE('',#9038,#9039,#5385,.T.);
#11599=EDGE_CURVE('',#9039,#9040,#4505,.T.);
#11600=EDGE_CURVE('',#9040,#9041,#6668,.T.);
#11601=EDGE_CURVE('',#9041,#9041,#4506,.F.);
#11602=EDGE_CURVE('',#9040,#9042,#4507,.T.);
#11603=EDGE_CURVE('',#9042,#9037,#5386,.T.);
#11604=EDGE_CURVE('',#9043,#9044,#6669,.T.);
#11605=EDGE_CURVE('',#9044,#9038,#5387,.T.);
#11606=EDGE_CURVE('',#9037,#9043,#5388,.T.);
#11607=EDGE_CURVE('',#9045,#9046,#6670,.T.);
#11608=EDGE_CURVE('',#9046,#9044,#5389,.T.);
#11609=EDGE_CURVE('',#9043,#9045,#5390,.T.);
#11610=EDGE_CURVE('',#9047,#9048,#6671,.T.);
#11611=EDGE_CURVE('',#9048,#9046,#5391,.T.);
#11612=EDGE_CURVE('',#9045,#9047,#5392,.T.);
#11613=EDGE_CURVE('',#9049,#9050,#6672,.T.);
#11614=EDGE_CURVE('',#9050,#9048,#5393,.T.);
#11615=EDGE_CURVE('',#9047,#9049,#5394,.T.);
#11616=EDGE_CURVE('',#9051,#9052,#6673,.T.);
#11617=EDGE_CURVE('',#9052,#9050,#5395,.T.);
#11618=EDGE_CURVE('',#9049,#9051,#5396,.T.);
#11619=EDGE_CURVE('',#9053,#9054,#6674,.T.);
#11620=EDGE_CURVE('',#9054,#9052,#5397,.T.);
#11621=EDGE_CURVE('',#9051,#9053,#5398,.T.);
#11622=EDGE_CURVE('',#9055,#9056,#6675,.T.);
#11623=EDGE_CURVE('',#9056,#9054,#5399,.T.);
#11624=EDGE_CURVE('',#9053,#9055,#5400,.T.);
#11625=EDGE_CURVE('',#9057,#9058,#6676,.T.);
#11626=EDGE_CURVE('',#9058,#9056,#5401,.T.);
#11627=EDGE_CURVE('',#9055,#9057,#5402,.T.);
#11628=EDGE_CURVE('',#9059,#9060,#6677,.T.);
#11629=EDGE_CURVE('',#9060,#9058,#5403,.T.);
#11630=EDGE_CURVE('',#9057,#9059,#5404,.T.);
#11631=EDGE_CURVE('',#9061,#9062,#6678,.T.);
#11632=EDGE_CURVE('',#9062,#9060,#5405,.T.);
#11633=EDGE_CURVE('',#9059,#9061,#5406,.T.);
#11634=EDGE_CURVE('',#9063,#9064,#6679,.T.);
#11635=EDGE_CURVE('',#9064,#9062,#5407,.T.);
#11636=EDGE_CURVE('',#9061,#9063,#5408,.T.);
#11637=EDGE_CURVE('',#9065,#9066,#6680,.T.);
#11638=EDGE_CURVE('',#9066,#9064,#5409,.T.);
#11639=EDGE_CURVE('',#9063,#9065,#5410,.T.);
#11640=EDGE_CURVE('',#9067,#9068,#6681,.T.);
#11641=EDGE_CURVE('',#9068,#9066,#5411,.T.);
#11642=EDGE_CURVE('',#9065,#9067,#5412,.T.);
#11643=EDGE_CURVE('',#9069,#9070,#6682,.T.);
#11644=EDGE_CURVE('',#9069,#9071,#5413,.T.);
#11645=EDGE_CURVE('',#9072,#9071,#4508,.T.);
#11646=EDGE_CURVE('',#9072,#9070,#5414,.T.);
#11647=EDGE_CURVE('',#9073,#9074,#6683,.T.);
#11648=EDGE_CURVE('',#9074,#9075,#5415,.T.);
#11649=EDGE_CURVE('',#9076,#9075,#4509,.T.);
#11650=EDGE_CURVE('',#9073,#9076,#5416,.T.);
#11651=EDGE_CURVE('',#9077,#9078,#6684,.T.);
#11652=EDGE_CURVE('',#9078,#9074,#5417,.T.);
#11653=EDGE_CURVE('',#9077,#9073,#5418,.T.);
#11654=EDGE_CURVE('',#9079,#9080,#6685,.T.);
#11655=EDGE_CURVE('',#9080,#9078,#5419,.T.);
#11656=EDGE_CURVE('',#9079,#9077,#5420,.T.);
#11657=EDGE_CURVE('',#9081,#9082,#6686,.T.);
#11658=EDGE_CURVE('',#9082,#9080,#5421,.T.);
#11659=EDGE_CURVE('',#9081,#9079,#5422,.T.);
#11660=EDGE_CURVE('',#9083,#9084,#6687,.T.);
#11661=EDGE_CURVE('',#9084,#9082,#5423,.T.);
#11662=EDGE_CURVE('',#9083,#9081,#5424,.T.);
#11663=EDGE_CURVE('',#9085,#9086,#6688,.T.);
#11664=EDGE_CURVE('',#9086,#9084,#5425,.T.);
#11665=EDGE_CURVE('',#9085,#9083,#5426,.T.);
#11666=EDGE_CURVE('',#9087,#9088,#6689,.T.);
#11667=EDGE_CURVE('',#9088,#9086,#5427,.T.);
#11668=EDGE_CURVE('',#9087,#9085,#5428,.T.);
#11669=EDGE_CURVE('',#9089,#9090,#6690,.T.);
#11670=EDGE_CURVE('',#9090,#9088,#5429,.T.);
#11671=EDGE_CURVE('',#9089,#9087,#5430,.T.);
#11672=EDGE_CURVE('',#9091,#9092,#6691,.T.);
#11673=EDGE_CURVE('',#9092,#9090,#5431,.T.);
#11674=EDGE_CURVE('',#9091,#9089,#5432,.T.);
#11675=EDGE_CURVE('',#9093,#9094,#6692,.T.);
#11676=EDGE_CURVE('',#9094,#9092,#5433,.T.);
#11677=EDGE_CURVE('',#9093,#9091,#5434,.T.);
#11678=EDGE_CURVE('',#9095,#9096,#6693,.T.);
#11679=EDGE_CURVE('',#9096,#9094,#5435,.T.);
#11680=EDGE_CURVE('',#9095,#9093,#5436,.T.);
#11681=EDGE_CURVE('',#9097,#9098,#6694,.T.);
#11682=EDGE_CURVE('',#9098,#9096,#5437,.T.);
#11683=EDGE_CURVE('',#9097,#9095,#5438,.T.);
#11684=EDGE_CURVE('',#9099,#9100,#6695,.T.);
#11685=EDGE_CURVE('',#9100,#9098,#5439,.T.);
#11686=EDGE_CURVE('',#9099,#9097,#5440,.T.);
#11687=EDGE_CURVE('',#9101,#9102,#6696,.T.);
#11688=EDGE_CURVE('',#9102,#9100,#5441,.T.);
#11689=EDGE_CURVE('',#9101,#9099,#5442,.T.);
#11690=EDGE_CURVE('',#9103,#9104,#6697,.T.);
#11691=EDGE_CURVE('',#9105,#9103,#5443,.T.);
#11692=EDGE_CURVE('',#9106,#9105,#4510,.T.);
#11693=EDGE_CURVE('',#9106,#9104,#5444,.T.);
#11694=EDGE_CURVE('',#9107,#9108,#6698,.T.);
#11695=EDGE_CURVE('',#9108,#9109,#5445,.T.);
#11696=EDGE_CURVE('',#9109,#9110,#4511,.T.);
#11697=EDGE_CURVE('',#9110,#9111,#6699,.T.);
#11698=EDGE_CURVE('',#9111,#9111,#4512,.F.);
#11699=EDGE_CURVE('',#9110,#9112,#4513,.T.);
#11700=EDGE_CURVE('',#9112,#9107,#5446,.T.);
#11701=EDGE_CURVE('',#9113,#9114,#6700,.T.);
#11702=EDGE_CURVE('',#9114,#9108,#5447,.T.);
#11703=EDGE_CURVE('',#9107,#9113,#5448,.T.);
#11704=EDGE_CURVE('',#9115,#9116,#6701,.T.);
#11705=EDGE_CURVE('',#9116,#9114,#5449,.T.);
#11706=EDGE_CURVE('',#9113,#9115,#5450,.T.);
#11707=EDGE_CURVE('',#9117,#9118,#6702,.T.);
#11708=EDGE_CURVE('',#9118,#9116,#5451,.T.);
#11709=EDGE_CURVE('',#9115,#9117,#5452,.T.);
#11710=EDGE_CURVE('',#9119,#9120,#6703,.T.);
#11711=EDGE_CURVE('',#9120,#9118,#5453,.T.);
#11712=EDGE_CURVE('',#9117,#9119,#5454,.T.);
#11713=EDGE_CURVE('',#9121,#9122,#6704,.T.);
#11714=EDGE_CURVE('',#9122,#9120,#5455,.T.);
#11715=EDGE_CURVE('',#9119,#9121,#5456,.T.);
#11716=EDGE_CURVE('',#9123,#9124,#6705,.T.);
#11717=EDGE_CURVE('',#9124,#9122,#5457,.T.);
#11718=EDGE_CURVE('',#9121,#9123,#5458,.T.);
#11719=EDGE_CURVE('',#9125,#9126,#6706,.T.);
#11720=EDGE_CURVE('',#9126,#9124,#5459,.T.);
#11721=EDGE_CURVE('',#9123,#9125,#5460,.T.);
#11722=EDGE_CURVE('',#9127,#9128,#6707,.T.);
#11723=EDGE_CURVE('',#9128,#9126,#5461,.T.);
#11724=EDGE_CURVE('',#9125,#9127,#5462,.T.);
#11725=EDGE_CURVE('',#9129,#9130,#6708,.T.);
#11726=EDGE_CURVE('',#9130,#9128,#5463,.T.);
#11727=EDGE_CURVE('',#9127,#9129,#5464,.T.);
#11728=EDGE_CURVE('',#9131,#9132,#6709,.T.);
#11729=EDGE_CURVE('',#9132,#9130,#5465,.T.);
#11730=EDGE_CURVE('',#9129,#9131,#5466,.T.);
#11731=EDGE_CURVE('',#9133,#9134,#6710,.T.);
#11732=EDGE_CURVE('',#9134,#9132,#5467,.T.);
#11733=EDGE_CURVE('',#9131,#9133,#5468,.T.);
#11734=EDGE_CURVE('',#9135,#9136,#6711,.T.);
#11735=EDGE_CURVE('',#9136,#9134,#5469,.T.);
#11736=EDGE_CURVE('',#9133,#9135,#5470,.T.);
#11737=EDGE_CURVE('',#9137,#9138,#6712,.T.);
#11738=EDGE_CURVE('',#9138,#9136,#5471,.T.);
#11739=EDGE_CURVE('',#9135,#9137,#5472,.T.);
#11740=EDGE_CURVE('',#9139,#9140,#6713,.T.);
#11741=EDGE_CURVE('',#9139,#9141,#5473,.T.);
#11742=EDGE_CURVE('',#9142,#9141,#4514,.T.);
#11743=EDGE_CURVE('',#9142,#9140,#5474,.T.);
#11744=EDGE_CURVE('',#9143,#9144,#6714,.T.);
#11745=EDGE_CURVE('',#9144,#9145,#5475,.T.);
#11746=EDGE_CURVE('',#9146,#9145,#4515,.T.);
#11747=EDGE_CURVE('',#9143,#9146,#5476,.T.);
#11748=EDGE_CURVE('',#9147,#9148,#6715,.T.);
#11749=EDGE_CURVE('',#9148,#9144,#5477,.T.);
#11750=EDGE_CURVE('',#9147,#9143,#5478,.T.);
#11751=EDGE_CURVE('',#9149,#9150,#6716,.T.);
#11752=EDGE_CURVE('',#9150,#9148,#5479,.T.);
#11753=EDGE_CURVE('',#9149,#9147,#5480,.T.);
#11754=EDGE_CURVE('',#9151,#9152,#6717,.T.);
#11755=EDGE_CURVE('',#9152,#9150,#5481,.T.);
#11756=EDGE_CURVE('',#9151,#9149,#5482,.T.);
#11757=EDGE_CURVE('',#9153,#9154,#6718,.T.);
#11758=EDGE_CURVE('',#9154,#9152,#5483,.T.);
#11759=EDGE_CURVE('',#9153,#9151,#5484,.T.);
#11760=EDGE_CURVE('',#9155,#9156,#6719,.T.);
#11761=EDGE_CURVE('',#9156,#9154,#5485,.T.);
#11762=EDGE_CURVE('',#9155,#9153,#5486,.T.);
#11763=EDGE_CURVE('',#9157,#9158,#6720,.T.);
#11764=EDGE_CURVE('',#9158,#9156,#5487,.T.);
#11765=EDGE_CURVE('',#9157,#9155,#5488,.T.);
#11766=EDGE_CURVE('',#9159,#9160,#6721,.T.);
#11767=EDGE_CURVE('',#9160,#9158,#5489,.T.);
#11768=EDGE_CURVE('',#9159,#9157,#5490,.T.);
#11769=EDGE_CURVE('',#9161,#9162,#6722,.T.);
#11770=EDGE_CURVE('',#9162,#9160,#5491,.T.);
#11771=EDGE_CURVE('',#9161,#9159,#5492,.T.);
#11772=EDGE_CURVE('',#9163,#9164,#6723,.T.);
#11773=EDGE_CURVE('',#9164,#9162,#5493,.T.);
#11774=EDGE_CURVE('',#9163,#9161,#5494,.T.);
#11775=EDGE_CURVE('',#9165,#9166,#6724,.T.);
#11776=EDGE_CURVE('',#9166,#9164,#5495,.T.);
#11777=EDGE_CURVE('',#9165,#9163,#5496,.T.);
#11778=EDGE_CURVE('',#9167,#9168,#6725,.T.);
#11779=EDGE_CURVE('',#9168,#9166,#5497,.T.);
#11780=EDGE_CURVE('',#9167,#9165,#5498,.T.);
#11781=EDGE_CURVE('',#9169,#9170,#6726,.T.);
#11782=EDGE_CURVE('',#9170,#9168,#5499,.T.);
#11783=EDGE_CURVE('',#9169,#9167,#5500,.T.);
#11784=EDGE_CURVE('',#9171,#9172,#6727,.T.);
#11785=EDGE_CURVE('',#9172,#9170,#5501,.T.);
#11786=EDGE_CURVE('',#9171,#9169,#5502,.T.);
#11787=EDGE_CURVE('',#9173,#9174,#6728,.T.);
#11788=EDGE_CURVE('',#9175,#9173,#5503,.T.);
#11789=EDGE_CURVE('',#9176,#9175,#4516,.T.);
#11790=EDGE_CURVE('',#9176,#9174,#5504,.T.);
#11791=EDGE_CURVE('',#9177,#9178,#6729,.T.);
#11792=EDGE_CURVE('',#9178,#9179,#5505,.T.);
#11793=EDGE_CURVE('',#9179,#9180,#4517,.T.);
#11794=EDGE_CURVE('',#9180,#9181,#6730,.T.);
#11795=EDGE_CURVE('',#9181,#9181,#4518,.F.);
#11796=EDGE_CURVE('',#9180,#9182,#4519,.T.);
#11797=EDGE_CURVE('',#9182,#9177,#5506,.T.);
#11798=EDGE_CURVE('',#9183,#9184,#6731,.T.);
#11799=EDGE_CURVE('',#9184,#9178,#5507,.T.);
#11800=EDGE_CURVE('',#9177,#9183,#5508,.T.);
#11801=EDGE_CURVE('',#9185,#9186,#6732,.T.);
#11802=EDGE_CURVE('',#9186,#9184,#5509,.T.);
#11803=EDGE_CURVE('',#9183,#9185,#5510,.T.);
#11804=EDGE_CURVE('',#9187,#9188,#6733,.T.);
#11805=EDGE_CURVE('',#9188,#9186,#5511,.T.);
#11806=EDGE_CURVE('',#9185,#9187,#5512,.T.);
#11807=EDGE_CURVE('',#9189,#9190,#6734,.T.);
#11808=EDGE_CURVE('',#9190,#9188,#5513,.T.);
#11809=EDGE_CURVE('',#9187,#9189,#5514,.T.);
#11810=EDGE_CURVE('',#9191,#9192,#6735,.T.);
#11811=EDGE_CURVE('',#9192,#9190,#5515,.T.);
#11812=EDGE_CURVE('',#9189,#9191,#5516,.T.);
#11813=EDGE_CURVE('',#9193,#9194,#6736,.T.);
#11814=EDGE_CURVE('',#9194,#9192,#5517,.T.);
#11815=EDGE_CURVE('',#9191,#9193,#5518,.T.);
#11816=EDGE_CURVE('',#9195,#9196,#6737,.T.);
#11817=EDGE_CURVE('',#9196,#9194,#5519,.T.);
#11818=EDGE_CURVE('',#9193,#9195,#5520,.T.);
#11819=EDGE_CURVE('',#9197,#9198,#6738,.T.);
#11820=EDGE_CURVE('',#9198,#9196,#5521,.T.);
#11821=EDGE_CURVE('',#9195,#9197,#5522,.T.);
#11822=EDGE_CURVE('',#9199,#9200,#6739,.T.);
#11823=EDGE_CURVE('',#9200,#9198,#5523,.T.);
#11824=EDGE_CURVE('',#9197,#9199,#5524,.T.);
#11825=EDGE_CURVE('',#9201,#9202,#6740,.T.);
#11826=EDGE_CURVE('',#9202,#9200,#5525,.T.);
#11827=EDGE_CURVE('',#9199,#9201,#5526,.T.);
#11828=EDGE_CURVE('',#9203,#9204,#6741,.T.);
#11829=EDGE_CURVE('',#9204,#9202,#5527,.T.);
#11830=EDGE_CURVE('',#9201,#9203,#5528,.T.);
#11831=EDGE_CURVE('',#9205,#9206,#6742,.T.);
#11832=EDGE_CURVE('',#9206,#9204,#5529,.T.);
#11833=EDGE_CURVE('',#9203,#9205,#5530,.T.);
#11834=EDGE_CURVE('',#9207,#9208,#6743,.T.);
#11835=EDGE_CURVE('',#9208,#9206,#5531,.T.);
#11836=EDGE_CURVE('',#9205,#9207,#5532,.T.);
#11837=EDGE_CURVE('',#9209,#9210,#6744,.T.);
#11838=EDGE_CURVE('',#9209,#9211,#5533,.T.);
#11839=EDGE_CURVE('',#9212,#9211,#4520,.T.);
#11840=EDGE_CURVE('',#9212,#9210,#5534,.T.);
#11841=EDGE_CURVE('',#9213,#9214,#6745,.T.);
#11842=EDGE_CURVE('',#9214,#9215,#5535,.T.);
#11843=EDGE_CURVE('',#9216,#9215,#4521,.T.);
#11844=EDGE_CURVE('',#9213,#9216,#5536,.T.);
#11845=EDGE_CURVE('',#9217,#9218,#6746,.T.);
#11846=EDGE_CURVE('',#9218,#9214,#5537,.T.);
#11847=EDGE_CURVE('',#9217,#9213,#5538,.T.);
#11848=EDGE_CURVE('',#9219,#9220,#6747,.T.);
#11849=EDGE_CURVE('',#9220,#9218,#5539,.T.);
#11850=EDGE_CURVE('',#9219,#9217,#5540,.T.);
#11851=EDGE_CURVE('',#9221,#9222,#6748,.T.);
#11852=EDGE_CURVE('',#9222,#9220,#5541,.T.);
#11853=EDGE_CURVE('',#9221,#9219,#5542,.T.);
#11854=EDGE_CURVE('',#9223,#9224,#6749,.T.);
#11855=EDGE_CURVE('',#9224,#9222,#5543,.T.);
#11856=EDGE_CURVE('',#9223,#9221,#5544,.T.);
#11857=EDGE_CURVE('',#9225,#9226,#6750,.T.);
#11858=EDGE_CURVE('',#9226,#9224,#5545,.T.);
#11859=EDGE_CURVE('',#9225,#9223,#5546,.T.);
#11860=EDGE_CURVE('',#9227,#9228,#6751,.T.);
#11861=EDGE_CURVE('',#9228,#9226,#5547,.T.);
#11862=EDGE_CURVE('',#9227,#9225,#5548,.T.);
#11863=EDGE_CURVE('',#9229,#9230,#6752,.T.);
#11864=EDGE_CURVE('',#9230,#9228,#5549,.T.);
#11865=EDGE_CURVE('',#9229,#9227,#5550,.T.);
#11866=EDGE_CURVE('',#9231,#9232,#6753,.T.);
#11867=EDGE_CURVE('',#9232,#9230,#5551,.T.);
#11868=EDGE_CURVE('',#9231,#9229,#5552,.T.);
#11869=EDGE_CURVE('',#9233,#9234,#6754,.T.);
#11870=EDGE_CURVE('',#9234,#9232,#5553,.T.);
#11871=EDGE_CURVE('',#9233,#9231,#5554,.T.);
#11872=EDGE_CURVE('',#9235,#9236,#6755,.T.);
#11873=EDGE_CURVE('',#9236,#9234,#5555,.T.);
#11874=EDGE_CURVE('',#9235,#9233,#5556,.T.);
#11875=EDGE_CURVE('',#9237,#9238,#6756,.T.);
#11876=EDGE_CURVE('',#9238,#9236,#5557,.T.);
#11877=EDGE_CURVE('',#9237,#9235,#5558,.T.);
#11878=EDGE_CURVE('',#9239,#9240,#6757,.T.);
#11879=EDGE_CURVE('',#9240,#9238,#5559,.T.);
#11880=EDGE_CURVE('',#9239,#9237,#5560,.T.);
#11881=EDGE_CURVE('',#9241,#9242,#6758,.T.);
#11882=EDGE_CURVE('',#9242,#9240,#5561,.T.);
#11883=EDGE_CURVE('',#9241,#9239,#5562,.T.);
#11884=EDGE_CURVE('',#9243,#9244,#6759,.T.);
#11885=EDGE_CURVE('',#9245,#9243,#5563,.T.);
#11886=EDGE_CURVE('',#9246,#9245,#4522,.T.);
#11887=EDGE_CURVE('',#9246,#9244,#5564,.T.);
#11888=EDGE_CURVE('',#9247,#9248,#6760,.T.);
#11889=EDGE_CURVE('',#9248,#9249,#5565,.T.);
#11890=EDGE_CURVE('',#9249,#9250,#4523,.T.);
#11891=EDGE_CURVE('',#9250,#9251,#6761,.T.);
#11892=EDGE_CURVE('',#9251,#9251,#4524,.F.);
#11893=EDGE_CURVE('',#9250,#9252,#4525,.T.);
#11894=EDGE_CURVE('',#9252,#9247,#5566,.T.);
#11895=EDGE_CURVE('',#9253,#9254,#6762,.T.);
#11896=EDGE_CURVE('',#9254,#9248,#5567,.T.);
#11897=EDGE_CURVE('',#9247,#9253,#5568,.T.);
#11898=EDGE_CURVE('',#9255,#9256,#6763,.T.);
#11899=EDGE_CURVE('',#9256,#9254,#5569,.T.);
#11900=EDGE_CURVE('',#9253,#9255,#5570,.T.);
#11901=EDGE_CURVE('',#9257,#9258,#6764,.T.);
#11902=EDGE_CURVE('',#9258,#9256,#5571,.T.);
#11903=EDGE_CURVE('',#9255,#9257,#5572,.T.);
#11904=EDGE_CURVE('',#9259,#9260,#6765,.T.);
#11905=EDGE_CURVE('',#9260,#9258,#5573,.T.);
#11906=EDGE_CURVE('',#9257,#9259,#5574,.T.);
#11907=EDGE_CURVE('',#9261,#9262,#6766,.T.);
#11908=EDGE_CURVE('',#9262,#9260,#5575,.T.);
#11909=EDGE_CURVE('',#9259,#9261,#5576,.T.);
#11910=EDGE_CURVE('',#9263,#9264,#6767,.T.);
#11911=EDGE_CURVE('',#9264,#9262,#5577,.T.);
#11912=EDGE_CURVE('',#9261,#9263,#5578,.T.);
#11913=EDGE_CURVE('',#9265,#9266,#6768,.T.);
#11914=EDGE_CURVE('',#9266,#9264,#5579,.T.);
#11915=EDGE_CURVE('',#9263,#9265,#5580,.T.);
#11916=EDGE_CURVE('',#9267,#9268,#6769,.T.);
#11917=EDGE_CURVE('',#9268,#9266,#5581,.T.);
#11918=EDGE_CURVE('',#9265,#9267,#5582,.T.);
#11919=EDGE_CURVE('',#9269,#9270,#6770,.T.);
#11920=EDGE_CURVE('',#9270,#9268,#5583,.T.);
#11921=EDGE_CURVE('',#9267,#9269,#5584,.T.);
#11922=EDGE_CURVE('',#9271,#9272,#6771,.T.);
#11923=EDGE_CURVE('',#9272,#9270,#5585,.T.);
#11924=EDGE_CURVE('',#9269,#9271,#5586,.T.);
#11925=EDGE_CURVE('',#9273,#9274,#6772,.T.);
#11926=EDGE_CURVE('',#9274,#9272,#5587,.T.);
#11927=EDGE_CURVE('',#9271,#9273,#5588,.T.);
#11928=EDGE_CURVE('',#9275,#9276,#6773,.T.);
#11929=EDGE_CURVE('',#9276,#9274,#5589,.T.);
#11930=EDGE_CURVE('',#9273,#9275,#5590,.T.);
#11931=EDGE_CURVE('',#9277,#9278,#6774,.T.);
#11932=EDGE_CURVE('',#9278,#9276,#5591,.T.);
#11933=EDGE_CURVE('',#9275,#9277,#5592,.T.);
#11934=EDGE_CURVE('',#9279,#9280,#6775,.T.);
#11935=EDGE_CURVE('',#9279,#9281,#5593,.T.);
#11936=EDGE_CURVE('',#9282,#9281,#4526,.T.);
#11937=EDGE_CURVE('',#9282,#9280,#5594,.T.);
#11938=EDGE_CURVE('',#9283,#9284,#6776,.T.);
#11939=EDGE_CURVE('',#9284,#9285,#5595,.T.);
#11940=EDGE_CURVE('',#9286,#9285,#4527,.T.);
#11941=EDGE_CURVE('',#9283,#9286,#5596,.T.);
#11942=EDGE_CURVE('',#9287,#9288,#6777,.T.);
#11943=EDGE_CURVE('',#9288,#9284,#5597,.T.);
#11944=EDGE_CURVE('',#9287,#9283,#5598,.T.);
#11945=EDGE_CURVE('',#9289,#9290,#6778,.T.);
#11946=EDGE_CURVE('',#9290,#9288,#5599,.T.);
#11947=EDGE_CURVE('',#9289,#9287,#5600,.T.);
#11948=EDGE_CURVE('',#9291,#9292,#6779,.T.);
#11949=EDGE_CURVE('',#9292,#9290,#5601,.T.);
#11950=EDGE_CURVE('',#9291,#9289,#5602,.T.);
#11951=EDGE_CURVE('',#9293,#9294,#6780,.T.);
#11952=EDGE_CURVE('',#9294,#9292,#5603,.T.);
#11953=EDGE_CURVE('',#9293,#9291,#5604,.T.);
#11954=EDGE_CURVE('',#9295,#9296,#6781,.T.);
#11955=EDGE_CURVE('',#9296,#9294,#5605,.T.);
#11956=EDGE_CURVE('',#9295,#9293,#5606,.T.);
#11957=EDGE_CURVE('',#9297,#9298,#6782,.T.);
#11958=EDGE_CURVE('',#9298,#9296,#5607,.T.);
#11959=EDGE_CURVE('',#9297,#9295,#5608,.T.);
#11960=EDGE_CURVE('',#9299,#9300,#6783,.T.);
#11961=EDGE_CURVE('',#9300,#9298,#5609,.T.);
#11962=EDGE_CURVE('',#9299,#9297,#5610,.T.);
#11963=EDGE_CURVE('',#9301,#9302,#6784,.T.);
#11964=EDGE_CURVE('',#9302,#9300,#5611,.T.);
#11965=EDGE_CURVE('',#9301,#9299,#5612,.T.);
#11966=EDGE_CURVE('',#9303,#9304,#6785,.T.);
#11967=EDGE_CURVE('',#9304,#9302,#5613,.T.);
#11968=EDGE_CURVE('',#9303,#9301,#5614,.T.);
#11969=EDGE_CURVE('',#9305,#9306,#6786,.T.);
#11970=EDGE_CURVE('',#9306,#9304,#5615,.T.);
#11971=EDGE_CURVE('',#9305,#9303,#5616,.T.);
#11972=EDGE_CURVE('',#9307,#9308,#6787,.T.);
#11973=EDGE_CURVE('',#9308,#9306,#5617,.T.);
#11974=EDGE_CURVE('',#9307,#9305,#5618,.T.);
#11975=EDGE_CURVE('',#9309,#9310,#6788,.T.);
#11976=EDGE_CURVE('',#9310,#9308,#5619,.T.);
#11977=EDGE_CURVE('',#9309,#9307,#5620,.T.);
#11978=EDGE_CURVE('',#9311,#9312,#6789,.T.);
#11979=EDGE_CURVE('',#9312,#9310,#5621,.T.);
#11980=EDGE_CURVE('',#9311,#9309,#5622,.T.);
#11981=EDGE_CURVE('',#9313,#9314,#6790,.T.);
#11982=EDGE_CURVE('',#9315,#9313,#5623,.T.);
#11983=EDGE_CURVE('',#9316,#9315,#4528,.T.);
#11984=EDGE_CURVE('',#9316,#9314,#5624,.T.);
#11985=EDGE_CURVE('',#9317,#9318,#6791,.T.);
#11986=EDGE_CURVE('',#9318,#9319,#5625,.T.);
#11987=EDGE_CURVE('',#9319,#9320,#4529,.T.);
#11988=EDGE_CURVE('',#9320,#9321,#6792,.T.);
#11989=EDGE_CURVE('',#9321,#9321,#4530,.F.);
#11990=EDGE_CURVE('',#9320,#9322,#4531,.T.);
#11991=EDGE_CURVE('',#9322,#9317,#5626,.T.);
#11992=EDGE_CURVE('',#9323,#9324,#6793,.T.);
#11993=EDGE_CURVE('',#9324,#9318,#5627,.T.);
#11994=EDGE_CURVE('',#9317,#9323,#5628,.T.);
#11995=EDGE_CURVE('',#9325,#9326,#6794,.T.);
#11996=EDGE_CURVE('',#9326,#9324,#5629,.T.);
#11997=EDGE_CURVE('',#9323,#9325,#5630,.T.);
#11998=EDGE_CURVE('',#9327,#9328,#6795,.T.);
#11999=EDGE_CURVE('',#9328,#9326,#5631,.T.);
#12000=EDGE_CURVE('',#9325,#9327,#5632,.T.);
#12001=EDGE_CURVE('',#9329,#9330,#6796,.T.);
#12002=EDGE_CURVE('',#9330,#9328,#5633,.T.);
#12003=EDGE_CURVE('',#9327,#9329,#5634,.T.);
#12004=EDGE_CURVE('',#9331,#9332,#6797,.T.);
#12005=EDGE_CURVE('',#9332,#9330,#5635,.T.);
#12006=EDGE_CURVE('',#9329,#9331,#5636,.T.);
#12007=EDGE_CURVE('',#9333,#9334,#6798,.T.);
#12008=EDGE_CURVE('',#9334,#9332,#5637,.T.);
#12009=EDGE_CURVE('',#9331,#9333,#5638,.T.);
#12010=EDGE_CURVE('',#9335,#9336,#6799,.T.);
#12011=EDGE_CURVE('',#9336,#9334,#5639,.T.);
#12012=EDGE_CURVE('',#9333,#9335,#5640,.T.);
#12013=EDGE_CURVE('',#9337,#9338,#6800,.T.);
#12014=EDGE_CURVE('',#9338,#9336,#5641,.T.);
#12015=EDGE_CURVE('',#9335,#9337,#5642,.T.);
#12016=EDGE_CURVE('',#9339,#9340,#6801,.T.);
#12017=EDGE_CURVE('',#9340,#9338,#5643,.T.);
#12018=EDGE_CURVE('',#9337,#9339,#5644,.T.);
#12019=EDGE_CURVE('',#9341,#9342,#6802,.T.);
#12020=EDGE_CURVE('',#9342,#9340,#5645,.T.);
#12021=EDGE_CURVE('',#9339,#9341,#5646,.T.);
#12022=EDGE_CURVE('',#9343,#9344,#6803,.T.);
#12023=EDGE_CURVE('',#9344,#9342,#5647,.T.);
#12024=EDGE_CURVE('',#9341,#9343,#5648,.T.);
#12025=EDGE_CURVE('',#9345,#9346,#6804,.T.);
#12026=EDGE_CURVE('',#9346,#9344,#5649,.T.);
#12027=EDGE_CURVE('',#9343,#9345,#5650,.T.);
#12028=EDGE_CURVE('',#9347,#9348,#6805,.T.);
#12029=EDGE_CURVE('',#9348,#9346,#5651,.T.);
#12030=EDGE_CURVE('',#9345,#9347,#5652,.T.);
#12031=EDGE_CURVE('',#9349,#9350,#6806,.T.);
#12032=EDGE_CURVE('',#9349,#9351,#5653,.T.);
#12033=EDGE_CURVE('',#9352,#9351,#4532,.T.);
#12034=EDGE_CURVE('',#9352,#9350,#5654,.T.);
#12035=EDGE_CURVE('',#9353,#9354,#6807,.T.);
#12036=EDGE_CURVE('',#9354,#9355,#5655,.T.);
#12037=EDGE_CURVE('',#9356,#9355,#4533,.T.);
#12038=EDGE_CURVE('',#9353,#9356,#5656,.T.);
#12039=EDGE_CURVE('',#9357,#9358,#6808,.T.);
#12040=EDGE_CURVE('',#9358,#9354,#5657,.T.);
#12041=EDGE_CURVE('',#9357,#9353,#5658,.T.);
#12042=EDGE_CURVE('',#9359,#9360,#6809,.T.);
#12043=EDGE_CURVE('',#9360,#9358,#5659,.T.);
#12044=EDGE_CURVE('',#9359,#9357,#5660,.T.);
#12045=EDGE_CURVE('',#9361,#9362,#6810,.T.);
#12046=EDGE_CURVE('',#9362,#9360,#5661,.T.);
#12047=EDGE_CURVE('',#9361,#9359,#5662,.T.);
#12048=EDGE_CURVE('',#9363,#9364,#6811,.T.);
#12049=EDGE_CURVE('',#9364,#9362,#5663,.T.);
#12050=EDGE_CURVE('',#9363,#9361,#5664,.T.);
#12051=EDGE_CURVE('',#9365,#9366,#6812,.T.);
#12052=EDGE_CURVE('',#9366,#9364,#5665,.T.);
#12053=EDGE_CURVE('',#9365,#9363,#5666,.T.);
#12054=EDGE_CURVE('',#9367,#9368,#6813,.T.);
#12055=EDGE_CURVE('',#9368,#9366,#5667,.T.);
#12056=EDGE_CURVE('',#9367,#9365,#5668,.T.);
#12057=EDGE_CURVE('',#9369,#9370,#6814,.T.);
#12058=EDGE_CURVE('',#9370,#9368,#5669,.T.);
#12059=EDGE_CURVE('',#9369,#9367,#5670,.T.);
#12060=EDGE_CURVE('',#9371,#9372,#6815,.T.);
#12061=EDGE_CURVE('',#9372,#9370,#5671,.T.);
#12062=EDGE_CURVE('',#9371,#9369,#5672,.T.);
#12063=EDGE_CURVE('',#9373,#9374,#6816,.T.);
#12064=EDGE_CURVE('',#9374,#9372,#5673,.T.);
#12065=EDGE_CURVE('',#9373,#9371,#5674,.T.);
#12066=EDGE_CURVE('',#9375,#9376,#6817,.T.);
#12067=EDGE_CURVE('',#9376,#9374,#5675,.T.);
#12068=EDGE_CURVE('',#9375,#9373,#5676,.T.);
#12069=EDGE_CURVE('',#9377,#9378,#6818,.T.);
#12070=EDGE_CURVE('',#9378,#9376,#5677,.T.);
#12071=EDGE_CURVE('',#9377,#9375,#5678,.T.);
#12072=EDGE_CURVE('',#9379,#9380,#6819,.T.);
#12073=EDGE_CURVE('',#9380,#9378,#5679,.T.);
#12074=EDGE_CURVE('',#9379,#9377,#5680,.T.);
#12075=EDGE_CURVE('',#9381,#9382,#6820,.T.);
#12076=EDGE_CURVE('',#9382,#9380,#5681,.T.);
#12077=EDGE_CURVE('',#9381,#9379,#5682,.T.);
#12078=EDGE_CURVE('',#9383,#9384,#6821,.T.);
#12079=EDGE_CURVE('',#9385,#9383,#5683,.T.);
#12080=EDGE_CURVE('',#9386,#9385,#4534,.T.);
#12081=EDGE_CURVE('',#9386,#9384,#5684,.T.);
#12082=EDGE_CURVE('',#9387,#9388,#6822,.T.);
#12083=EDGE_CURVE('',#9388,#9389,#5685,.T.);
#12084=EDGE_CURVE('',#9389,#9390,#4535,.T.);
#12085=EDGE_CURVE('',#9390,#9391,#6823,.T.);
#12086=EDGE_CURVE('',#9391,#9391,#4536,.F.);
#12087=EDGE_CURVE('',#9390,#9392,#4537,.T.);
#12088=EDGE_CURVE('',#9392,#9387,#5686,.T.);
#12089=EDGE_CURVE('',#9393,#9394,#6824,.T.);
#12090=EDGE_CURVE('',#9394,#9388,#5687,.T.);
#12091=EDGE_CURVE('',#9387,#9393,#5688,.T.);
#12092=EDGE_CURVE('',#9395,#9396,#6825,.T.);
#12093=EDGE_CURVE('',#9396,#9394,#5689,.T.);
#12094=EDGE_CURVE('',#9393,#9395,#5690,.T.);
#12095=EDGE_CURVE('',#9397,#9398,#6826,.T.);
#12096=EDGE_CURVE('',#9398,#9396,#5691,.T.);
#12097=EDGE_CURVE('',#9395,#9397,#5692,.T.);
#12098=EDGE_CURVE('',#9399,#9400,#6827,.T.);
#12099=EDGE_CURVE('',#9400,#9398,#5693,.T.);
#12100=EDGE_CURVE('',#9397,#9399,#5694,.T.);
#12101=EDGE_CURVE('',#9401,#9402,#6828,.T.);
#12102=EDGE_CURVE('',#9402,#9400,#5695,.T.);
#12103=EDGE_CURVE('',#9399,#9401,#5696,.T.);
#12104=EDGE_CURVE('',#9403,#9404,#6829,.T.);
#12105=EDGE_CURVE('',#9404,#9402,#5697,.T.);
#12106=EDGE_CURVE('',#9401,#9403,#5698,.T.);
#12107=EDGE_CURVE('',#9405,#9406,#6830,.T.);
#12108=EDGE_CURVE('',#9406,#9404,#5699,.T.);
#12109=EDGE_CURVE('',#9403,#9405,#5700,.T.);
#12110=EDGE_CURVE('',#9407,#9408,#6831,.T.);
#12111=EDGE_CURVE('',#9408,#9406,#5701,.T.);
#12112=EDGE_CURVE('',#9405,#9407,#5702,.T.);
#12113=EDGE_CURVE('',#9409,#9410,#6832,.T.);
#12114=EDGE_CURVE('',#9410,#9408,#5703,.T.);
#12115=EDGE_CURVE('',#9407,#9409,#5704,.T.);
#12116=EDGE_CURVE('',#9411,#9412,#6833,.T.);
#12117=EDGE_CURVE('',#9412,#9410,#5705,.T.);
#12118=EDGE_CURVE('',#9409,#9411,#5706,.T.);
#12119=EDGE_CURVE('',#9413,#9414,#6834,.T.);
#12120=EDGE_CURVE('',#9414,#9412,#5707,.T.);
#12121=EDGE_CURVE('',#9411,#9413,#5708,.T.);
#12122=EDGE_CURVE('',#9415,#9416,#6835,.T.);
#12123=EDGE_CURVE('',#9416,#9414,#5709,.T.);
#12124=EDGE_CURVE('',#9413,#9415,#5710,.T.);
#12125=EDGE_CURVE('',#9417,#9418,#6836,.T.);
#12126=EDGE_CURVE('',#9418,#9416,#5711,.T.);
#12127=EDGE_CURVE('',#9415,#9417,#5712,.T.);
#12128=EDGE_CURVE('',#9419,#9420,#6837,.T.);
#12129=EDGE_CURVE('',#9419,#9421,#5713,.T.);
#12130=EDGE_CURVE('',#9422,#9421,#4538,.T.);
#12131=EDGE_CURVE('',#9422,#9420,#5714,.T.);
#12132=EDGE_CURVE('',#9423,#9424,#6838,.T.);
#12133=EDGE_CURVE('',#9424,#9425,#5715,.T.);
#12134=EDGE_CURVE('',#9426,#9425,#4539,.T.);
#12135=EDGE_CURVE('',#9423,#9426,#5716,.T.);
#12136=EDGE_CURVE('',#9427,#9428,#6839,.T.);
#12137=EDGE_CURVE('',#9428,#9424,#5717,.T.);
#12138=EDGE_CURVE('',#9427,#9423,#5718,.T.);
#12139=EDGE_CURVE('',#9429,#9430,#6840,.T.);
#12140=EDGE_CURVE('',#9430,#9428,#5719,.T.);
#12141=EDGE_CURVE('',#9429,#9427,#5720,.T.);
#12142=EDGE_CURVE('',#9431,#9432,#6841,.T.);
#12143=EDGE_CURVE('',#9432,#9430,#5721,.T.);
#12144=EDGE_CURVE('',#9431,#9429,#5722,.T.);
#12145=EDGE_CURVE('',#9433,#9434,#6842,.T.);
#12146=EDGE_CURVE('',#9434,#9432,#5723,.T.);
#12147=EDGE_CURVE('',#9433,#9431,#5724,.T.);
#12148=EDGE_CURVE('',#9435,#9436,#6843,.T.);
#12149=EDGE_CURVE('',#9436,#9434,#5725,.T.);
#12150=EDGE_CURVE('',#9435,#9433,#5726,.T.);
#12151=EDGE_CURVE('',#9437,#9438,#6844,.T.);
#12152=EDGE_CURVE('',#9438,#9436,#5727,.T.);
#12153=EDGE_CURVE('',#9437,#9435,#5728,.T.);
#12154=EDGE_CURVE('',#9439,#9440,#6845,.T.);
#12155=EDGE_CURVE('',#9440,#9438,#5729,.T.);
#12156=EDGE_CURVE('',#9439,#9437,#5730,.T.);
#12157=EDGE_CURVE('',#9441,#9442,#6846,.T.);
#12158=EDGE_CURVE('',#9442,#9440,#5731,.T.);
#12159=EDGE_CURVE('',#9441,#9439,#5732,.T.);
#12160=EDGE_CURVE('',#9443,#9444,#6847,.T.);
#12161=EDGE_CURVE('',#9444,#9442,#5733,.T.);
#12162=EDGE_CURVE('',#9443,#9441,#5734,.T.);
#12163=EDGE_CURVE('',#9445,#9446,#6848,.T.);
#12164=EDGE_CURVE('',#9446,#9444,#5735,.T.);
#12165=EDGE_CURVE('',#9445,#9443,#5736,.T.);
#12166=EDGE_CURVE('',#9447,#9448,#6849,.T.);
#12167=EDGE_CURVE('',#9448,#9446,#5737,.T.);
#12168=EDGE_CURVE('',#9447,#9445,#5738,.T.);
#12169=EDGE_CURVE('',#9449,#9450,#6850,.T.);
#12170=EDGE_CURVE('',#9450,#9448,#5739,.T.);
#12171=EDGE_CURVE('',#9449,#9447,#5740,.T.);
#12172=EDGE_CURVE('',#9451,#9452,#6851,.T.);
#12173=EDGE_CURVE('',#9452,#9450,#5741,.T.);
#12174=EDGE_CURVE('',#9451,#9449,#5742,.T.);
#12175=EDGE_CURVE('',#9453,#9454,#6852,.T.);
#12176=EDGE_CURVE('',#9455,#9453,#5743,.T.);
#12177=EDGE_CURVE('',#9456,#9455,#4540,.T.);
#12178=EDGE_CURVE('',#9456,#9454,#5744,.T.);
#12179=EDGE_CURVE('',#9457,#9458,#6853,.T.);
#12180=EDGE_CURVE('',#9458,#9459,#5745,.T.);
#12181=EDGE_CURVE('',#9459,#9460,#4541,.T.);
#12182=EDGE_CURVE('',#9460,#9461,#6854,.T.);
#12183=EDGE_CURVE('',#9461,#9461,#4542,.F.);
#12184=EDGE_CURVE('',#9460,#9462,#4543,.T.);
#12185=EDGE_CURVE('',#9462,#9457,#5746,.T.);
#12186=EDGE_CURVE('',#9463,#9464,#6855,.T.);
#12187=EDGE_CURVE('',#9464,#9458,#5747,.T.);
#12188=EDGE_CURVE('',#9457,#9463,#5748,.T.);
#12189=EDGE_CURVE('',#9465,#9466,#6856,.T.);
#12190=EDGE_CURVE('',#9466,#9464,#5749,.T.);
#12191=EDGE_CURVE('',#9463,#9465,#5750,.T.);
#12192=EDGE_CURVE('',#9467,#9468,#6857,.T.);
#12193=EDGE_CURVE('',#9468,#9466,#5751,.T.);
#12194=EDGE_CURVE('',#9465,#9467,#5752,.T.);
#12195=EDGE_CURVE('',#9469,#9470,#6858,.T.);
#12196=EDGE_CURVE('',#9470,#9468,#5753,.T.);
#12197=EDGE_CURVE('',#9467,#9469,#5754,.T.);
#12198=EDGE_CURVE('',#9471,#9472,#6859,.T.);
#12199=EDGE_CURVE('',#9472,#9470,#5755,.T.);
#12200=EDGE_CURVE('',#9469,#9471,#5756,.T.);
#12201=EDGE_CURVE('',#9473,#9474,#6860,.T.);
#12202=EDGE_CURVE('',#9474,#9472,#5757,.T.);
#12203=EDGE_CURVE('',#9471,#9473,#5758,.T.);
#12204=EDGE_CURVE('',#9475,#9476,#6861,.T.);
#12205=EDGE_CURVE('',#9476,#9474,#5759,.T.);
#12206=EDGE_CURVE('',#9473,#9475,#5760,.T.);
#12207=EDGE_CURVE('',#9477,#9478,#6862,.T.);
#12208=EDGE_CURVE('',#9478,#9476,#5761,.T.);
#12209=EDGE_CURVE('',#9475,#9477,#5762,.T.);
#12210=EDGE_CURVE('',#9479,#9480,#6863,.T.);
#12211=EDGE_CURVE('',#9480,#9478,#5763,.T.);
#12212=EDGE_CURVE('',#9477,#9479,#5764,.T.);
#12213=EDGE_CURVE('',#9481,#9482,#6864,.T.);
#12214=EDGE_CURVE('',#9482,#9480,#5765,.T.);
#12215=EDGE_CURVE('',#9479,#9481,#5766,.T.);
#12216=EDGE_CURVE('',#9483,#9484,#6865,.T.);
#12217=EDGE_CURVE('',#9484,#9482,#5767,.T.);
#12218=EDGE_CURVE('',#9481,#9483,#5768,.T.);
#12219=EDGE_CURVE('',#9485,#9486,#6866,.T.);
#12220=EDGE_CURVE('',#9486,#9484,#5769,.T.);
#12221=EDGE_CURVE('',#9483,#9485,#5770,.T.);
#12222=EDGE_CURVE('',#9487,#9488,#6867,.T.);
#12223=EDGE_CURVE('',#9488,#9486,#5771,.T.);
#12224=EDGE_CURVE('',#9485,#9487,#5772,.T.);
#12225=EDGE_CURVE('',#9489,#9490,#6868,.T.);
#12226=EDGE_CURVE('',#9489,#9491,#5773,.T.);
#12227=EDGE_CURVE('',#9492,#9491,#4544,.T.);
#12228=EDGE_CURVE('',#9492,#9490,#5774,.T.);
#12229=EDGE_CURVE('',#9493,#9494,#6869,.T.);
#12230=EDGE_CURVE('',#9494,#9495,#5775,.T.);
#12231=EDGE_CURVE('',#9496,#9495,#4545,.T.);
#12232=EDGE_CURVE('',#9493,#9496,#5776,.T.);
#12233=EDGE_CURVE('',#9497,#9498,#6870,.T.);
#12234=EDGE_CURVE('',#9498,#9494,#5777,.T.);
#12235=EDGE_CURVE('',#9497,#9493,#5778,.T.);
#12236=EDGE_CURVE('',#9499,#9500,#6871,.T.);
#12237=EDGE_CURVE('',#9500,#9498,#5779,.T.);
#12238=EDGE_CURVE('',#9499,#9497,#5780,.T.);
#12239=EDGE_CURVE('',#9501,#9502,#6872,.T.);
#12240=EDGE_CURVE('',#9502,#9500,#5781,.T.);
#12241=EDGE_CURVE('',#9501,#9499,#5782,.T.);
#12242=EDGE_CURVE('',#9503,#9504,#6873,.T.);
#12243=EDGE_CURVE('',#9504,#9502,#5783,.T.);
#12244=EDGE_CURVE('',#9503,#9501,#5784,.T.);
#12245=EDGE_CURVE('',#9505,#9506,#6874,.T.);
#12246=EDGE_CURVE('',#9506,#9504,#5785,.T.);
#12247=EDGE_CURVE('',#9505,#9503,#5786,.T.);
#12248=EDGE_CURVE('',#9507,#9508,#6875,.T.);
#12249=EDGE_CURVE('',#9508,#9506,#5787,.T.);
#12250=EDGE_CURVE('',#9507,#9505,#5788,.T.);
#12251=EDGE_CURVE('',#9509,#9510,#6876,.T.);
#12252=EDGE_CURVE('',#9510,#9508,#5789,.T.);
#12253=EDGE_CURVE('',#9509,#9507,#5790,.T.);
#12254=EDGE_CURVE('',#9511,#9512,#6877,.T.);
#12255=EDGE_CURVE('',#9512,#9510,#5791,.T.);
#12256=EDGE_CURVE('',#9511,#9509,#5792,.T.);
#12257=EDGE_CURVE('',#9513,#9514,#6878,.T.);
#12258=EDGE_CURVE('',#9514,#9512,#5793,.T.);
#12259=EDGE_CURVE('',#9513,#9511,#5794,.T.);
#12260=EDGE_CURVE('',#9515,#9516,#6879,.T.);
#12261=EDGE_CURVE('',#9516,#9514,#5795,.T.);
#12262=EDGE_CURVE('',#9515,#9513,#5796,.T.);
#12263=EDGE_CURVE('',#9517,#9518,#6880,.T.);
#12264=EDGE_CURVE('',#9518,#9516,#5797,.T.);
#12265=EDGE_CURVE('',#9517,#9515,#5798,.T.);
#12266=EDGE_CURVE('',#9519,#9520,#6881,.T.);
#12267=EDGE_CURVE('',#9520,#9518,#5799,.T.);
#12268=EDGE_CURVE('',#9519,#9517,#5800,.T.);
#12269=EDGE_CURVE('',#9521,#9522,#6882,.T.);
#12270=EDGE_CURVE('',#9522,#9520,#5801,.T.);
#12271=EDGE_CURVE('',#9521,#9519,#5802,.T.);
#12272=EDGE_CURVE('',#9523,#9524,#6883,.T.);
#12273=EDGE_CURVE('',#9525,#9523,#5803,.T.);
#12274=EDGE_CURVE('',#9526,#9525,#4546,.T.);
#12275=EDGE_CURVE('',#9526,#9524,#5804,.T.);
#12276=EDGE_CURVE('',#9527,#9528,#6884,.T.);
#12277=EDGE_CURVE('',#9528,#9529,#5805,.T.);
#12278=EDGE_CURVE('',#9529,#9530,#4547,.T.);
#12279=EDGE_CURVE('',#9530,#9531,#6885,.T.);
#12280=EDGE_CURVE('',#9531,#9531,#4548,.F.);
#12281=EDGE_CURVE('',#9530,#9532,#4549,.T.);
#12282=EDGE_CURVE('',#9532,#9527,#5806,.T.);
#12283=EDGE_CURVE('',#9533,#9534,#6886,.T.);
#12284=EDGE_CURVE('',#9534,#9528,#5807,.T.);
#12285=EDGE_CURVE('',#9527,#9533,#5808,.T.);
#12286=EDGE_CURVE('',#9535,#9536,#6887,.T.);
#12287=EDGE_CURVE('',#9536,#9534,#5809,.T.);
#12288=EDGE_CURVE('',#9533,#9535,#5810,.T.);
#12289=EDGE_CURVE('',#9537,#9538,#6888,.T.);
#12290=EDGE_CURVE('',#9538,#9536,#5811,.T.);
#12291=EDGE_CURVE('',#9535,#9537,#5812,.T.);
#12292=EDGE_CURVE('',#9539,#9540,#6889,.T.);
#12293=EDGE_CURVE('',#9540,#9538,#5813,.T.);
#12294=EDGE_CURVE('',#9537,#9539,#5814,.T.);
#12295=EDGE_CURVE('',#9541,#9542,#6890,.T.);
#12296=EDGE_CURVE('',#9542,#9540,#5815,.T.);
#12297=EDGE_CURVE('',#9539,#9541,#5816,.T.);
#12298=EDGE_CURVE('',#9543,#9544,#6891,.T.);
#12299=EDGE_CURVE('',#9544,#9542,#5817,.T.);
#12300=EDGE_CURVE('',#9541,#9543,#5818,.T.);
#12301=EDGE_CURVE('',#9545,#9546,#6892,.T.);
#12302=EDGE_CURVE('',#9546,#9544,#5819,.T.);
#12303=EDGE_CURVE('',#9543,#9545,#5820,.T.);
#12304=EDGE_CURVE('',#9547,#9548,#6893,.T.);
#12305=EDGE_CURVE('',#9548,#9546,#5821,.T.);
#12306=EDGE_CURVE('',#9545,#9547,#5822,.T.);
#12307=EDGE_CURVE('',#9549,#9550,#6894,.T.);
#12308=EDGE_CURVE('',#9550,#9548,#5823,.T.);
#12309=EDGE_CURVE('',#9547,#9549,#5824,.T.);
#12310=EDGE_CURVE('',#9551,#9552,#6895,.T.);
#12311=EDGE_CURVE('',#9552,#9550,#5825,.T.);
#12312=EDGE_CURVE('',#9549,#9551,#5826,.T.);
#12313=EDGE_CURVE('',#9553,#9554,#6896,.T.);
#12314=EDGE_CURVE('',#9554,#9552,#5827,.T.);
#12315=EDGE_CURVE('',#9551,#9553,#5828,.T.);
#12316=EDGE_CURVE('',#9555,#9556,#6897,.T.);
#12317=EDGE_CURVE('',#9556,#9554,#5829,.T.);
#12318=EDGE_CURVE('',#9553,#9555,#5830,.T.);
#12319=EDGE_CURVE('',#9557,#9558,#6898,.T.);
#12320=EDGE_CURVE('',#9558,#9556,#5831,.T.);
#12321=EDGE_CURVE('',#9555,#9557,#5832,.T.);
#12322=EDGE_CURVE('',#9559,#9560,#6899,.T.);
#12323=EDGE_CURVE('',#9559,#9561,#5833,.T.);
#12324=EDGE_CURVE('',#9562,#9561,#4550,.T.);
#12325=EDGE_CURVE('',#9562,#9560,#5834,.T.);
#12326=EDGE_CURVE('',#9563,#9564,#6900,.T.);
#12327=EDGE_CURVE('',#9564,#9565,#5835,.T.);
#12328=EDGE_CURVE('',#9566,#9565,#4551,.T.);
#12329=EDGE_CURVE('',#9563,#9566,#5836,.T.);
#12330=EDGE_CURVE('',#9567,#9568,#6901,.T.);
#12331=EDGE_CURVE('',#9568,#9564,#5837,.T.);
#12332=EDGE_CURVE('',#9567,#9563,#5838,.T.);
#12333=EDGE_CURVE('',#9569,#9570,#6902,.T.);
#12334=EDGE_CURVE('',#9570,#9568,#5839,.T.);
#12335=EDGE_CURVE('',#9569,#9567,#5840,.T.);
#12336=EDGE_CURVE('',#9571,#9572,#6903,.T.);
#12337=EDGE_CURVE('',#9572,#9570,#5841,.T.);
#12338=EDGE_CURVE('',#9571,#9569,#5842,.T.);
#12339=EDGE_CURVE('',#9573,#9574,#6904,.T.);
#12340=EDGE_CURVE('',#9574,#9572,#5843,.T.);
#12341=EDGE_CURVE('',#9573,#9571,#5844,.T.);
#12342=EDGE_CURVE('',#9575,#9576,#6905,.T.);
#12343=EDGE_CURVE('',#9576,#9574,#5845,.T.);
#12344=EDGE_CURVE('',#9575,#9573,#5846,.T.);
#12345=EDGE_CURVE('',#9577,#9578,#6906,.T.);
#12346=EDGE_CURVE('',#9578,#9576,#5847,.T.);
#12347=EDGE_CURVE('',#9577,#9575,#5848,.T.);
#12348=EDGE_CURVE('',#9579,#9580,#6907,.T.);
#12349=EDGE_CURVE('',#9580,#9578,#5849,.T.);
#12350=EDGE_CURVE('',#9579,#9577,#5850,.T.);
#12351=EDGE_CURVE('',#9581,#9582,#6908,.T.);
#12352=EDGE_CURVE('',#9582,#9580,#5851,.T.);
#12353=EDGE_CURVE('',#9581,#9579,#5852,.T.);
#12354=EDGE_CURVE('',#9583,#9584,#6909,.T.);
#12355=EDGE_CURVE('',#9584,#9582,#5853,.T.);
#12356=EDGE_CURVE('',#9583,#9581,#5854,.T.);
#12357=EDGE_CURVE('',#9585,#9586,#6910,.T.);
#12358=EDGE_CURVE('',#9586,#9584,#5855,.T.);
#12359=EDGE_CURVE('',#9585,#9583,#5856,.T.);
#12360=EDGE_CURVE('',#9587,#9588,#6911,.T.);
#12361=EDGE_CURVE('',#9588,#9586,#5857,.T.);
#12362=EDGE_CURVE('',#9587,#9585,#5858,.T.);
#12363=EDGE_CURVE('',#9589,#9590,#6912,.T.);
#12364=EDGE_CURVE('',#9590,#9588,#5859,.T.);
#12365=EDGE_CURVE('',#9589,#9587,#5860,.T.);
#12366=EDGE_CURVE('',#9591,#9592,#6913,.T.);
#12367=EDGE_CURVE('',#9592,#9590,#5861,.T.);
#12368=EDGE_CURVE('',#9591,#9589,#5862,.T.);
#12369=EDGE_CURVE('',#9593,#9594,#6914,.T.);
#12370=EDGE_CURVE('',#9595,#9593,#5863,.T.);
#12371=EDGE_CURVE('',#9596,#9595,#4552,.T.);
#12372=EDGE_CURVE('',#9596,#9594,#5864,.T.);
#12373=EDGE_CURVE('',#9597,#9598,#5865,.T.);
#12374=EDGE_CURVE('',#9597,#9599,#6915,.T.);
#12375=EDGE_CURVE('',#9600,#9599,#5866,.T.);
#12376=EDGE_CURVE('',#9599,#9600,#5867,.T.);
#12377=EDGE_CURVE('',#9598,#9597,#5868,.T.);
#12378=EDGE_CURVE('',#9601,#9602,#5869,.T.);
#12379=EDGE_CURVE('',#9602,#9601,#5870,.T.);
#12380=EDGE_CURVE('',#9602,#9603,#6916,.T.);
#12381=EDGE_CURVE('',#9604,#9603,#5871,.T.);
#12382=EDGE_CURVE('',#9603,#9604,#5872,.T.);
#12383=EDGE_CURVE('',#9605,#9606,#5873,.T.);
#12384=EDGE_CURVE('',#9607,#9605,#5874,.T.);
#12385=EDGE_CURVE('',#9607,#9608,#6917,.T.);
#12386=EDGE_CURVE('',#9609,#9608,#5875,.T.);
#12387=EDGE_CURVE('',#9610,#9609,#5876,.T.);
#12388=EDGE_CURVE('',#9608,#9610,#5877,.T.);
#12389=EDGE_CURVE('',#9606,#9607,#5878,.T.);
#12390=EDGE_CURVE('',#9611,#9612,#5879,.T.);
#12391=EDGE_CURVE('',#9613,#9611,#5880,.T.);
#12392=EDGE_CURVE('',#9613,#9614,#6918,.T.);
#12393=EDGE_CURVE('',#9614,#9614,#5881,.T.);
#12394=EDGE_CURVE('',#9612,#9613,#5882,.T.);
#12395=EDGE_CURVE('',#9615,#9616,#5883,.T.);
#12396=EDGE_CURVE('',#9615,#9617,#6919,.T.);
#12397=EDGE_CURVE('',#9618,#9617,#5884,.T.);
#12398=EDGE_CURVE('',#9617,#9618,#5885,.T.);
#12399=EDGE_CURVE('',#9616,#9615,#5886,.T.);
#12400=EDGE_CURVE('',#9619,#9620,#5887,.T.);
#12401=EDGE_CURVE('',#9620,#9619,#5888,.T.);
#12402=EDGE_CURVE('',#9620,#9621,#6920,.T.);
#12403=EDGE_CURVE('',#9622,#9621,#5889,.T.);
#12404=EDGE_CURVE('',#9621,#9622,#5890,.T.);
#12405=EDGE_CURVE('',#9623,#9624,#5891,.T.);
#12406=EDGE_CURVE('',#9625,#9623,#5892,.T.);
#12407=EDGE_CURVE('',#9625,#9626,#6921,.T.);
#12408=EDGE_CURVE('',#9627,#9626,#5893,.T.);
#12409=EDGE_CURVE('',#9628,#9627,#5894,.T.);
#12410=EDGE_CURVE('',#9626,#9628,#5895,.T.);
#12411=EDGE_CURVE('',#9624,#9625,#5896,.T.);
#12412=EDGE_CURVE('',#9629,#9630,#5897,.T.);
#12413=EDGE_CURVE('',#9631,#9629,#5898,.T.);
#12414=EDGE_CURVE('',#9631,#9632,#6922,.T.);
#12415=EDGE_CURVE('',#9632,#9632,#5899,.T.);
#12416=EDGE_CURVE('',#9630,#9631,#5900,.T.);
#12417=EDGE_CURVE('',#9633,#9634,#5901,.T.);
#12418=EDGE_CURVE('',#9633,#9635,#6923,.T.);
#12419=EDGE_CURVE('',#9636,#9635,#5902,.T.);
#12420=EDGE_CURVE('',#9635,#9636,#5903,.T.);
#12421=EDGE_CURVE('',#9634,#9633,#5904,.T.);
#12422=EDGE_CURVE('',#9637,#9638,#5905,.T.);
#12423=EDGE_CURVE('',#9638,#9637,#5906,.T.);
#12424=EDGE_CURVE('',#9638,#9639,#6924,.T.);
#12425=EDGE_CURVE('',#9640,#9639,#5907,.T.);
#12426=EDGE_CURVE('',#9639,#9640,#5908,.T.);
#12427=EDGE_CURVE('',#9641,#9642,#5909,.T.);
#12428=EDGE_CURVE('',#9643,#9641,#5910,.T.);
#12429=EDGE_CURVE('',#9643,#9644,#6925,.T.);
#12430=EDGE_CURVE('',#9645,#9644,#5911,.T.);
#12431=EDGE_CURVE('',#9646,#9645,#5912,.T.);
#12432=EDGE_CURVE('',#9644,#9646,#5913,.T.);
#12433=EDGE_CURVE('',#9642,#9643,#5914,.T.);
#12434=EDGE_CURVE('',#9647,#9648,#5915,.T.);
#12435=EDGE_CURVE('',#9649,#9647,#5916,.T.);
#12436=EDGE_CURVE('',#9649,#9650,#6926,.T.);
#12437=EDGE_CURVE('',#9650,#9650,#5917,.T.);
#12438=EDGE_CURVE('',#9648,#9649,#5918,.T.);
#12439=EDGE_CURVE('',#9529,#9566,#5919,.T.);
#12440=EDGE_CURVE('',#9565,#9532,#5920,.T.);
#12441=EDGE_CURVE('',#9594,#9592,#5921,.T.);
#12442=EDGE_CURVE('',#9593,#9591,#5922,.T.);
#12443=EDGE_CURVE('',#9561,#9596,#5923,.T.);
#12444=EDGE_CURVE('',#9557,#9559,#5924,.T.);
#12445=EDGE_CURVE('',#9560,#9558,#5925,.T.);
#12446=EDGE_CURVE('',#9595,#9562,#5926,.T.);
#12447=EDGE_CURVE('',#9459,#9496,#5927,.T.);
#12448=EDGE_CURVE('',#9495,#9462,#5928,.T.);
#12449=EDGE_CURVE('',#9524,#9522,#5929,.T.);
#12450=EDGE_CURVE('',#9523,#9521,#5930,.T.);
#12451=EDGE_CURVE('',#9491,#9526,#5931,.T.);
#12452=EDGE_CURVE('',#9487,#9489,#5932,.T.);
#12453=EDGE_CURVE('',#9490,#9488,#5933,.T.);
#12454=EDGE_CURVE('',#9525,#9492,#5934,.T.);
#12455=EDGE_CURVE('',#9389,#9426,#5935,.T.);
#12456=EDGE_CURVE('',#9425,#9392,#5936,.T.);
#12457=EDGE_CURVE('',#9454,#9452,#5937,.T.);
#12458=EDGE_CURVE('',#9453,#9451,#5938,.T.);
#12459=EDGE_CURVE('',#9421,#9456,#5939,.T.);
#12460=EDGE_CURVE('',#9417,#9419,#5940,.T.);
#12461=EDGE_CURVE('',#9420,#9418,#5941,.T.);
#12462=EDGE_CURVE('',#9455,#9422,#5942,.T.);
#12463=EDGE_CURVE('',#9319,#9356,#5943,.T.);
#12464=EDGE_CURVE('',#9355,#9322,#5944,.T.);
#12465=EDGE_CURVE('',#9384,#9382,#5945,.T.);
#12466=EDGE_CURVE('',#9383,#9381,#5946,.T.);
#12467=EDGE_CURVE('',#9351,#9386,#5947,.T.);
#12468=EDGE_CURVE('',#9347,#9349,#5948,.T.);
#12469=EDGE_CURVE('',#9350,#9348,#5949,.T.);
#12470=EDGE_CURVE('',#9385,#9352,#5950,.T.);
#12471=EDGE_CURVE('',#9249,#9286,#5951,.T.);
#12472=EDGE_CURVE('',#9285,#9252,#5952,.T.);
#12473=EDGE_CURVE('',#9314,#9312,#5953,.T.);
#12474=EDGE_CURVE('',#9313,#9311,#5954,.T.);
#12475=EDGE_CURVE('',#9281,#9316,#5955,.T.);
#12476=EDGE_CURVE('',#9277,#9279,#5956,.T.);
#12477=EDGE_CURVE('',#9280,#9278,#5957,.T.);
#12478=EDGE_CURVE('',#9315,#9282,#5958,.T.);
#12479=EDGE_CURVE('',#9179,#9216,#5959,.T.);
#12480=EDGE_CURVE('',#9215,#9182,#5960,.T.);
#12481=EDGE_CURVE('',#9244,#9242,#5961,.T.);
#12482=EDGE_CURVE('',#9243,#9241,#5962,.T.);
#12483=EDGE_CURVE('',#9211,#9246,#5963,.T.);
#12484=EDGE_CURVE('',#9207,#9209,#5964,.T.);
#12485=EDGE_CURVE('',#9210,#9208,#5965,.T.);
#12486=EDGE_CURVE('',#9245,#9212,#5966,.T.);
#12487=EDGE_CURVE('',#9109,#9146,#5967,.T.);
#12488=EDGE_CURVE('',#9145,#9112,#5968,.T.);
#12489=EDGE_CURVE('',#9174,#9172,#5969,.T.);
#12490=EDGE_CURVE('',#9173,#9171,#5970,.T.);
#12491=EDGE_CURVE('',#9141,#9176,#5971,.T.);
#12492=EDGE_CURVE('',#9137,#9139,#5972,.T.);
#12493=EDGE_CURVE('',#9140,#9138,#5973,.T.);
#12494=EDGE_CURVE('',#9175,#9142,#5974,.T.);
#12495=EDGE_CURVE('',#9039,#9076,#5975,.T.);
#12496=EDGE_CURVE('',#9075,#9042,#5976,.T.);
#12497=EDGE_CURVE('',#9104,#9102,#5977,.T.);
#12498=EDGE_CURVE('',#9103,#9101,#5978,.T.);
#12499=EDGE_CURVE('',#9071,#9106,#5979,.T.);
#12500=EDGE_CURVE('',#9067,#9069,#5980,.T.);
#12501=EDGE_CURVE('',#9070,#9068,#5981,.T.);
#12502=EDGE_CURVE('',#9105,#9072,#5982,.T.);
#12503=EDGE_CURVE('',#9651,#9651,#4553,.T.);
#12504=EDGE_CURVE('',#9651,#9652,#6927,.T.);
#12505=EDGE_CURVE('',#9652,#9652,#4554,.T.);
#12506=EDGE_CURVE('',#9653,#9653,#4555,.T.);
#12507=EDGE_CURVE('',#9653,#9654,#6928,.T.);
#12508=EDGE_CURVE('',#9654,#9654,#4556,.T.);
#12509=EDGE_CURVE('',#9655,#9655,#4557,.T.);
#12510=EDGE_CURVE('',#9655,#9656,#6929,.T.);
#12511=EDGE_CURVE('',#9656,#9656,#4558,.T.);
#12512=EDGE_CURVE('',#9657,#9657,#4559,.T.);
#12513=EDGE_CURVE('',#9657,#9658,#6930,.T.);
#12514=EDGE_CURVE('',#9658,#9658,#4560,.T.);
#12515=EDGE_CURVE('',#9659,#9659,#4561,.T.);
#12516=EDGE_CURVE('',#9659,#9660,#6931,.T.);
#12517=EDGE_CURVE('',#9660,#9660,#4562,.T.);
#12518=EDGE_CURVE('',#9661,#9661,#4563,.T.);
#12519=EDGE_CURVE('',#9662,#9662,#4564,.T.);
#12520=EDGE_CURVE('',#9662,#9609,#6932,.T.);
#12521=EDGE_CURVE('',#9610,#9627,#6933,.T.);
#12522=EDGE_CURVE('',#9628,#9645,#6934,.T.);
#12523=EDGE_CURVE('',#9646,#9663,#6935,.T.);
#12524=EDGE_CURVE('',#9663,#9663,#4565,.T.);
#12525=EDGE_CURVE('',#9664,#9664,#4566,.T.);
#12526=EDGE_CURVE('',#9664,#9605,#6936,.T.);
#12527=EDGE_CURVE('',#9606,#9623,#6937,.T.);
#12528=EDGE_CURVE('',#9624,#9641,#6938,.T.);
#12529=EDGE_CURVE('',#9642,#9665,#6939,.T.);
#12530=EDGE_CURVE('',#9665,#9665,#4567,.T.);
#12531=EDGE_CURVE('',#9666,#9666,#4568,.F.);
#12532=EDGE_CURVE('',#9661,#9667,#6940,.T.);
#12533=EDGE_CURVE('',#9667,#9667,#4569,.T.);
#12534=EDGE_CURVE('',#9666,#9668,#6941,.T.);
#12535=EDGE_CURVE('',#9668,#9668,#4570,.F.);
#15424=ORIENTED_EDGE('',*,*,#11597,.T.);
#15425=ORIENTED_EDGE('',*,*,#11598,.T.);
#15426=ORIENTED_EDGE('',*,*,#11599,.T.);
#15427=ORIENTED_EDGE('',*,*,#11600,.T.);
#15428=ORIENTED_EDGE('',*,*,#11601,.T.);
#15429=ORIENTED_EDGE('',*,*,#11600,.F.);
#15430=ORIENTED_EDGE('',*,*,#11602,.T.);
#15431=ORIENTED_EDGE('',*,*,#11603,.T.);
#15432=ORIENTED_EDGE('',*,*,#11604,.T.);
#15433=ORIENTED_EDGE('',*,*,#11605,.T.);
#15434=ORIENTED_EDGE('',*,*,#11597,.F.);
#15435=ORIENTED_EDGE('',*,*,#11606,.T.);
#15436=ORIENTED_EDGE('',*,*,#11607,.T.);
#15437=ORIENTED_EDGE('',*,*,#11608,.T.);
#15438=ORIENTED_EDGE('',*,*,#11604,.F.);
#15439=ORIENTED_EDGE('',*,*,#11609,.T.);
#15440=ORIENTED_EDGE('',*,*,#11610,.T.);
#15441=ORIENTED_EDGE('',*,*,#11611,.T.);
#15442=ORIENTED_EDGE('',*,*,#11607,.F.);
#15443=ORIENTED_EDGE('',*,*,#11612,.T.);
#15444=ORIENTED_EDGE('',*,*,#11613,.T.);
#15445=ORIENTED_EDGE('',*,*,#11614,.T.);
#15446=ORIENTED_EDGE('',*,*,#11610,.F.);
#15447=ORIENTED_EDGE('',*,*,#11615,.T.);
#15448=ORIENTED_EDGE('',*,*,#11616,.T.);
#15449=ORIENTED_EDGE('',*,*,#11617,.T.);
#15450=ORIENTED_EDGE('',*,*,#11613,.F.);
#15451=ORIENTED_EDGE('',*,*,#11618,.T.);
#15452=ORIENTED_EDGE('',*,*,#11619,.T.);
#15453=ORIENTED_EDGE('',*,*,#11620,.T.);
#15454=ORIENTED_EDGE('',*,*,#11616,.F.);
#15455=ORIENTED_EDGE('',*,*,#11621,.T.);
#15456=ORIENTED_EDGE('',*,*,#11622,.T.);
#15457=ORIENTED_EDGE('',*,*,#11623,.T.);
#15458=ORIENTED_EDGE('',*,*,#11619,.F.);
#15459=ORIENTED_EDGE('',*,*,#11624,.T.);
#15460=ORIENTED_EDGE('',*,*,#11625,.T.);
#15461=ORIENTED_EDGE('',*,*,#11626,.T.);
#15462=ORIENTED_EDGE('',*,*,#11622,.F.);
#15463=ORIENTED_EDGE('',*,*,#11627,.T.);
#15464=ORIENTED_EDGE('',*,*,#11628,.T.);
#15465=ORIENTED_EDGE('',*,*,#11629,.T.);
#15466=ORIENTED_EDGE('',*,*,#11625,.F.);
#15467=ORIENTED_EDGE('',*,*,#11630,.T.);
#15468=ORIENTED_EDGE('',*,*,#11631,.T.);
#15469=ORIENTED_EDGE('',*,*,#11632,.T.);
#15470=ORIENTED_EDGE('',*,*,#11628,.F.);
#15471=ORIENTED_EDGE('',*,*,#11633,.T.);
#15472=ORIENTED_EDGE('',*,*,#11634,.T.);
#15473=ORIENTED_EDGE('',*,*,#11635,.T.);
#15474=ORIENTED_EDGE('',*,*,#11631,.F.);
#15475=ORIENTED_EDGE('',*,*,#11636,.T.);
#15476=ORIENTED_EDGE('',*,*,#11637,.T.);
#15477=ORIENTED_EDGE('',*,*,#11638,.T.);
#15478=ORIENTED_EDGE('',*,*,#11634,.F.);
#15479=ORIENTED_EDGE('',*,*,#11639,.T.);
#15480=ORIENTED_EDGE('',*,*,#11640,.T.);
#15481=ORIENTED_EDGE('',*,*,#11641,.T.);
#15482=ORIENTED_EDGE('',*,*,#11637,.F.);
#15483=ORIENTED_EDGE('',*,*,#11642,.T.);
#15484=ORIENTED_EDGE('',*,*,#11643,.F.);
#15485=ORIENTED_EDGE('',*,*,#11644,.T.);
#15486=ORIENTED_EDGE('',*,*,#11645,.F.);
#15487=ORIENTED_EDGE('',*,*,#11646,.T.);
#15488=ORIENTED_EDGE('',*,*,#11647,.T.);
#15489=ORIENTED_EDGE('',*,*,#11648,.T.);
#15490=ORIENTED_EDGE('',*,*,#11649,.F.);
#15491=ORIENTED_EDGE('',*,*,#11650,.F.);
#15492=ORIENTED_EDGE('',*,*,#11651,.T.);
#15493=ORIENTED_EDGE('',*,*,#11652,.T.);
#15494=ORIENTED_EDGE('',*,*,#11647,.F.);
#15495=ORIENTED_EDGE('',*,*,#11653,.F.);
#15496=ORIENTED_EDGE('',*,*,#11654,.T.);
#15497=ORIENTED_EDGE('',*,*,#11655,.T.);
#15498=ORIENTED_EDGE('',*,*,#11651,.F.);
#15499=ORIENTED_EDGE('',*,*,#11656,.F.);
#15500=ORIENTED_EDGE('',*,*,#11657,.T.);
#15501=ORIENTED_EDGE('',*,*,#11658,.T.);
#15502=ORIENTED_EDGE('',*,*,#11654,.F.);
#15503=ORIENTED_EDGE('',*,*,#11659,.F.);
#15504=ORIENTED_EDGE('',*,*,#11660,.T.);
#15505=ORIENTED_EDGE('',*,*,#11661,.T.);
#15506=ORIENTED_EDGE('',*,*,#11657,.F.);
#15507=ORIENTED_EDGE('',*,*,#11662,.F.);
#15508=ORIENTED_EDGE('',*,*,#11663,.T.);
#15509=ORIENTED_EDGE('',*,*,#11664,.T.);
#15510=ORIENTED_EDGE('',*,*,#11660,.F.);
#15511=ORIENTED_EDGE('',*,*,#11665,.F.);
#15512=ORIENTED_EDGE('',*,*,#11666,.T.);
#15513=ORIENTED_EDGE('',*,*,#11667,.T.);
#15514=ORIENTED_EDGE('',*,*,#11663,.F.);
#15515=ORIENTED_EDGE('',*,*,#11668,.F.);
#15516=ORIENTED_EDGE('',*,*,#11669,.T.);
#15517=ORIENTED_EDGE('',*,*,#11670,.T.);
#15518=ORIENTED_EDGE('',*,*,#11666,.F.);
#15519=ORIENTED_EDGE('',*,*,#11671,.F.);
#15520=ORIENTED_EDGE('',*,*,#11672,.T.);
#15521=ORIENTED_EDGE('',*,*,#11673,.T.);
#15522=ORIENTED_EDGE('',*,*,#11669,.F.);
#15523=ORIENTED_EDGE('',*,*,#11674,.F.);
#15524=ORIENTED_EDGE('',*,*,#11675,.T.);
#15525=ORIENTED_EDGE('',*,*,#11676,.T.);
#15526=ORIENTED_EDGE('',*,*,#11672,.F.);
#15527=ORIENTED_EDGE('',*,*,#11677,.F.);
#15528=ORIENTED_EDGE('',*,*,#11678,.T.);
#15529=ORIENTED_EDGE('',*,*,#11679,.T.);
#15530=ORIENTED_EDGE('',*,*,#11675,.F.);
#15531=ORIENTED_EDGE('',*,*,#11680,.F.);
#15532=ORIENTED_EDGE('',*,*,#11681,.T.);
#15533=ORIENTED_EDGE('',*,*,#11682,.T.);
#15534=ORIENTED_EDGE('',*,*,#11678,.F.);
#15535=ORIENTED_EDGE('',*,*,#11683,.F.);
#15536=ORIENTED_EDGE('',*,*,#11684,.T.);
#15537=ORIENTED_EDGE('',*,*,#11685,.T.);
#15538=ORIENTED_EDGE('',*,*,#11681,.F.);
#15539=ORIENTED_EDGE('',*,*,#11686,.F.);
#15540=ORIENTED_EDGE('',*,*,#11687,.T.);
#15541=ORIENTED_EDGE('',*,*,#11688,.T.);
#15542=ORIENTED_EDGE('',*,*,#11684,.F.);
#15543=ORIENTED_EDGE('',*,*,#11689,.F.);
#15544=ORIENTED_EDGE('',*,*,#11690,.F.);
#15545=ORIENTED_EDGE('',*,*,#11691,.F.);
#15546=ORIENTED_EDGE('',*,*,#11692,.F.);
#15547=ORIENTED_EDGE('',*,*,#11693,.T.);
#15548=ORIENTED_EDGE('',*,*,#11694,.T.);
#15549=ORIENTED_EDGE('',*,*,#11695,.T.);
#15550=ORIENTED_EDGE('',*,*,#11696,.T.);
#15551=ORIENTED_EDGE('',*,*,#11697,.T.);
#15552=ORIENTED_EDGE('',*,*,#11698,.T.);
#15553=ORIENTED_EDGE('',*,*,#11697,.F.);
#15554=ORIENTED_EDGE('',*,*,#11699,.T.);
#15555=ORIENTED_EDGE('',*,*,#11700,.T.);
#15556=ORIENTED_EDGE('',*,*,#11701,.T.);
#15557=ORIENTED_EDGE('',*,*,#11702,.T.);
#15558=ORIENTED_EDGE('',*,*,#11694,.F.);
#15559=ORIENTED_EDGE('',*,*,#11703,.T.);
#15560=ORIENTED_EDGE('',*,*,#11704,.T.);
#15561=ORIENTED_EDGE('',*,*,#11705,.T.);
#15562=ORIENTED_EDGE('',*,*,#11701,.F.);
#15563=ORIENTED_EDGE('',*,*,#11706,.T.);
#15564=ORIENTED_EDGE('',*,*,#11707,.T.);
#15565=ORIENTED_EDGE('',*,*,#11708,.T.);
#15566=ORIENTED_EDGE('',*,*,#11704,.F.);
#15567=ORIENTED_EDGE('',*,*,#11709,.T.);
#15568=ORIENTED_EDGE('',*,*,#11710,.T.);
#15569=ORIENTED_EDGE('',*,*,#11711,.T.);
#15570=ORIENTED_EDGE('',*,*,#11707,.F.);
#15571=ORIENTED_EDGE('',*,*,#11712,.T.);
#15572=ORIENTED_EDGE('',*,*,#11713,.T.);
#15573=ORIENTED_EDGE('',*,*,#11714,.T.);
#15574=ORIENTED_EDGE('',*,*,#11710,.F.);
#15575=ORIENTED_EDGE('',*,*,#11715,.T.);
#15576=ORIENTED_EDGE('',*,*,#11716,.T.);
#15577=ORIENTED_EDGE('',*,*,#11717,.T.);
#15578=ORIENTED_EDGE('',*,*,#11713,.F.);
#15579=ORIENTED_EDGE('',*,*,#11718,.T.);
#15580=ORIENTED_EDGE('',*,*,#11719,.T.);
#15581=ORIENTED_EDGE('',*,*,#11720,.T.);
#15582=ORIENTED_EDGE('',*,*,#11716,.F.);
#15583=ORIENTED_EDGE('',*,*,#11721,.T.);
#15584=ORIENTED_EDGE('',*,*,#11722,.T.);
#15585=ORIENTED_EDGE('',*,*,#11723,.T.);
#15586=ORIENTED_EDGE('',*,*,#11719,.F.);
#15587=ORIENTED_EDGE('',*,*,#11724,.T.);
#15588=ORIENTED_EDGE('',*,*,#11725,.T.);
#15589=ORIENTED_EDGE('',*,*,#11726,.T.);
#15590=ORIENTED_EDGE('',*,*,#11722,.F.);
#15591=ORIENTED_EDGE('',*,*,#11727,.T.);
#15592=ORIENTED_EDGE('',*,*,#11728,.T.);
#15593=ORIENTED_EDGE('',*,*,#11729,.T.);
#15594=ORIENTED_EDGE('',*,*,#11725,.F.);
#15595=ORIENTED_EDGE('',*,*,#11730,.T.);
#15596=ORIENTED_EDGE('',*,*,#11731,.T.);
#15597=ORIENTED_EDGE('',*,*,#11732,.T.);
#15598=ORIENTED_EDGE('',*,*,#11728,.F.);
#15599=ORIENTED_EDGE('',*,*,#11733,.T.);
#15600=ORIENTED_EDGE('',*,*,#11734,.T.);
#15601=ORIENTED_EDGE('',*,*,#11735,.T.);
#15602=ORIENTED_EDGE('',*,*,#11731,.F.);
#15603=ORIENTED_EDGE('',*,*,#11736,.T.);
#15604=ORIENTED_EDGE('',*,*,#11737,.T.);
#15605=ORIENTED_EDGE('',*,*,#11738,.T.);
#15606=ORIENTED_EDGE('',*,*,#11734,.F.);
#15607=ORIENTED_EDGE('',*,*,#11739,.T.);
#15608=ORIENTED_EDGE('',*,*,#11740,.F.);
#15609=ORIENTED_EDGE('',*,*,#11741,.T.);
#15610=ORIENTED_EDGE('',*,*,#11742,.F.);
#15611=ORIENTED_EDGE('',*,*,#11743,.T.);
#15612=ORIENTED_EDGE('',*,*,#11744,.T.);
#15613=ORIENTED_EDGE('',*,*,#11745,.T.);
#15614=ORIENTED_EDGE('',*,*,#11746,.F.);
#15615=ORIENTED_EDGE('',*,*,#11747,.F.);
#15616=ORIENTED_EDGE('',*,*,#11748,.T.);
#15617=ORIENTED_EDGE('',*,*,#11749,.T.);
#15618=ORIENTED_EDGE('',*,*,#11744,.F.);
#15619=ORIENTED_EDGE('',*,*,#11750,.F.);
#15620=ORIENTED_EDGE('',*,*,#11751,.T.);
#15621=ORIENTED_EDGE('',*,*,#11752,.T.);
#15622=ORIENTED_EDGE('',*,*,#11748,.F.);
#15623=ORIENTED_EDGE('',*,*,#11753,.F.);
#15624=ORIENTED_EDGE('',*,*,#11754,.T.);
#15625=ORIENTED_EDGE('',*,*,#11755,.T.);
#15626=ORIENTED_EDGE('',*,*,#11751,.F.);
#15627=ORIENTED_EDGE('',*,*,#11756,.F.);
#15628=ORIENTED_EDGE('',*,*,#11757,.T.);
#15629=ORIENTED_EDGE('',*,*,#11758,.T.);
#15630=ORIENTED_EDGE('',*,*,#11754,.F.);
#15631=ORIENTED_EDGE('',*,*,#11759,.F.);
#15632=ORIENTED_EDGE('',*,*,#11760,.T.);
#15633=ORIENTED_EDGE('',*,*,#11761,.T.);
#15634=ORIENTED_EDGE('',*,*,#11757,.F.);
#15635=ORIENTED_EDGE('',*,*,#11762,.F.);
#15636=ORIENTED_EDGE('',*,*,#11763,.T.);
#15637=ORIENTED_EDGE('',*,*,#11764,.T.);
#15638=ORIENTED_EDGE('',*,*,#11760,.F.);
#15639=ORIENTED_EDGE('',*,*,#11765,.F.);
#15640=ORIENTED_EDGE('',*,*,#11766,.T.);
#15641=ORIENTED_EDGE('',*,*,#11767,.T.);
#15642=ORIENTED_EDGE('',*,*,#11763,.F.);
#15643=ORIENTED_EDGE('',*,*,#11768,.F.);
#15644=ORIENTED_EDGE('',*,*,#11769,.T.);
#15645=ORIENTED_EDGE('',*,*,#11770,.T.);
#15646=ORIENTED_EDGE('',*,*,#11766,.F.);
#15647=ORIENTED_EDGE('',*,*,#11771,.F.);
#15648=ORIENTED_EDGE('',*,*,#11772,.T.);
#15649=ORIENTED_EDGE('',*,*,#11773,.T.);
#15650=ORIENTED_EDGE('',*,*,#11769,.F.);
#15651=ORIENTED_EDGE('',*,*,#11774,.F.);
#15652=ORIENTED_EDGE('',*,*,#11775,.T.);
#15653=ORIENTED_EDGE('',*,*,#11776,.T.);
#15654=ORIENTED_EDGE('',*,*,#11772,.F.);
#15655=ORIENTED_EDGE('',*,*,#11777,.F.);
#15656=ORIENTED_EDGE('',*,*,#11778,.T.);
#15657=ORIENTED_EDGE('',*,*,#11779,.T.);
#15658=ORIENTED_EDGE('',*,*,#11775,.F.);
#15659=ORIENTED_EDGE('',*,*,#11780,.F.);
#15660=ORIENTED_EDGE('',*,*,#11781,.T.);
#15661=ORIENTED_EDGE('',*,*,#11782,.T.);
#15662=ORIENTED_EDGE('',*,*,#11778,.F.);
#15663=ORIENTED_EDGE('',*,*,#11783,.F.);
#15664=ORIENTED_EDGE('',*,*,#11784,.T.);
#15665=ORIENTED_EDGE('',*,*,#11785,.T.);
#15666=ORIENTED_EDGE('',*,*,#11781,.F.);
#15667=ORIENTED_EDGE('',*,*,#11786,.F.);
#15668=ORIENTED_EDGE('',*,*,#11787,.F.);
#15669=ORIENTED_EDGE('',*,*,#11788,.F.);
#15670=ORIENTED_EDGE('',*,*,#11789,.F.);
#15671=ORIENTED_EDGE('',*,*,#11790,.T.);
#15672=ORIENTED_EDGE('',*,*,#11791,.T.);
#15673=ORIENTED_EDGE('',*,*,#11792,.T.);
#15674=ORIENTED_EDGE('',*,*,#11793,.T.);
#15675=ORIENTED_EDGE('',*,*,#11794,.T.);
#15676=ORIENTED_EDGE('',*,*,#11795,.T.);
#15677=ORIENTED_EDGE('',*,*,#11794,.F.);
#15678=ORIENTED_EDGE('',*,*,#11796,.T.);
#15679=ORIENTED_EDGE('',*,*,#11797,.T.);
#15680=ORIENTED_EDGE('',*,*,#11798,.T.);
#15681=ORIENTED_EDGE('',*,*,#11799,.T.);
#15682=ORIENTED_EDGE('',*,*,#11791,.F.);
#15683=ORIENTED_EDGE('',*,*,#11800,.T.);
#15684=ORIENTED_EDGE('',*,*,#11801,.T.);
#15685=ORIENTED_EDGE('',*,*,#11802,.T.);
#15686=ORIENTED_EDGE('',*,*,#11798,.F.);
#15687=ORIENTED_EDGE('',*,*,#11803,.T.);
#15688=ORIENTED_EDGE('',*,*,#11804,.T.);
#15689=ORIENTED_EDGE('',*,*,#11805,.T.);
#15690=ORIENTED_EDGE('',*,*,#11801,.F.);
#15691=ORIENTED_EDGE('',*,*,#11806,.T.);
#15692=ORIENTED_EDGE('',*,*,#11807,.T.);
#15693=ORIENTED_EDGE('',*,*,#11808,.T.);
#15694=ORIENTED_EDGE('',*,*,#11804,.F.);
#15695=ORIENTED_EDGE('',*,*,#11809,.T.);
#15696=ORIENTED_EDGE('',*,*,#11810,.T.);
#15697=ORIENTED_EDGE('',*,*,#11811,.T.);
#15698=ORIENTED_EDGE('',*,*,#11807,.F.);
#15699=ORIENTED_EDGE('',*,*,#11812,.T.);
#15700=ORIENTED_EDGE('',*,*,#11813,.T.);
#15701=ORIENTED_EDGE('',*,*,#11814,.T.);
#15702=ORIENTED_EDGE('',*,*,#11810,.F.);
#15703=ORIENTED_EDGE('',*,*,#11815,.T.);
#15704=ORIENTED_EDGE('',*,*,#11816,.T.);
#15705=ORIENTED_EDGE('',*,*,#11817,.T.);
#15706=ORIENTED_EDGE('',*,*,#11813,.F.);
#15707=ORIENTED_EDGE('',*,*,#11818,.T.);
#15708=ORIENTED_EDGE('',*,*,#11819,.T.);
#15709=ORIENTED_EDGE('',*,*,#11820,.T.);
#15710=ORIENTED_EDGE('',*,*,#11816,.F.);
#15711=ORIENTED_EDGE('',*,*,#11821,.T.);
#15712=ORIENTED_EDGE('',*,*,#11822,.T.);
#15713=ORIENTED_EDGE('',*,*,#11823,.T.);
#15714=ORIENTED_EDGE('',*,*,#11819,.F.);
#15715=ORIENTED_EDGE('',*,*,#11824,.T.);
#15716=ORIENTED_EDGE('',*,*,#11825,.T.);
#15717=ORIENTED_EDGE('',*,*,#11826,.T.);
#15718=ORIENTED_EDGE('',*,*,#11822,.F.);
#15719=ORIENTED_EDGE('',*,*,#11827,.T.);
#15720=ORIENTED_EDGE('',*,*,#11828,.T.);
#15721=ORIENTED_EDGE('',*,*,#11829,.T.);
#15722=ORIENTED_EDGE('',*,*,#11825,.F.);
#15723=ORIENTED_EDGE('',*,*,#11830,.T.);
#15724=ORIENTED_EDGE('',*,*,#11831,.T.);
#15725=ORIENTED_EDGE('',*,*,#11832,.T.);
#15726=ORIENTED_EDGE('',*,*,#11828,.F.);
#15727=ORIENTED_EDGE('',*,*,#11833,.T.);
#15728=ORIENTED_EDGE('',*,*,#11834,.T.);
#15729=ORIENTED_EDGE('',*,*,#11835,.T.);
#15730=ORIENTED_EDGE('',*,*,#11831,.F.);
#15731=ORIENTED_EDGE('',*,*,#11836,.T.);
#15732=ORIENTED_EDGE('',*,*,#11837,.F.);
#15733=ORIENTED_EDGE('',*,*,#11838,.T.);
#15734=ORIENTED_EDGE('',*,*,#11839,.F.);
#15735=ORIENTED_EDGE('',*,*,#11840,.T.);
#15736=ORIENTED_EDGE('',*,*,#11841,.T.);
#15737=ORIENTED_EDGE('',*,*,#11842,.T.);
#15738=ORIENTED_EDGE('',*,*,#11843,.F.);
#15739=ORIENTED_EDGE('',*,*,#11844,.F.);
#15740=ORIENTED_EDGE('',*,*,#11845,.T.);
#15741=ORIENTED_EDGE('',*,*,#11846,.T.);
#15742=ORIENTED_EDGE('',*,*,#11841,.F.);
#15743=ORIENTED_EDGE('',*,*,#11847,.F.);
#15744=ORIENTED_EDGE('',*,*,#11848,.T.);
#15745=ORIENTED_EDGE('',*,*,#11849,.T.);
#15746=ORIENTED_EDGE('',*,*,#11845,.F.);
#15747=ORIENTED_EDGE('',*,*,#11850,.F.);
#15748=ORIENTED_EDGE('',*,*,#11851,.T.);
#15749=ORIENTED_EDGE('',*,*,#11852,.T.);
#15750=ORIENTED_EDGE('',*,*,#11848,.F.);
#15751=ORIENTED_EDGE('',*,*,#11853,.F.);
#15752=ORIENTED_EDGE('',*,*,#11854,.T.);
#15753=ORIENTED_EDGE('',*,*,#11855,.T.);
#15754=ORIENTED_EDGE('',*,*,#11851,.F.);
#15755=ORIENTED_EDGE('',*,*,#11856,.F.);
#15756=ORIENTED_EDGE('',*,*,#11857,.T.);
#15757=ORIENTED_EDGE('',*,*,#11858,.T.);
#15758=ORIENTED_EDGE('',*,*,#11854,.F.);
#15759=ORIENTED_EDGE('',*,*,#11859,.F.);
#15760=ORIENTED_EDGE('',*,*,#11860,.T.);
#15761=ORIENTED_EDGE('',*,*,#11861,.T.);
#15762=ORIENTED_EDGE('',*,*,#11857,.F.);
#15763=ORIENTED_EDGE('',*,*,#11862,.F.);
#15764=ORIENTED_EDGE('',*,*,#11863,.T.);
#15765=ORIENTED_EDGE('',*,*,#11864,.T.);
#15766=ORIENTED_EDGE('',*,*,#11860,.F.);
#15767=ORIENTED_EDGE('',*,*,#11865,.F.);
#15768=ORIENTED_EDGE('',*,*,#11866,.T.);
#15769=ORIENTED_EDGE('',*,*,#11867,.T.);
#15770=ORIENTED_EDGE('',*,*,#11863,.F.);
#15771=ORIENTED_EDGE('',*,*,#11868,.F.);
#15772=ORIENTED_EDGE('',*,*,#11869,.T.);
#15773=ORIENTED_EDGE('',*,*,#11870,.T.);
#15774=ORIENTED_EDGE('',*,*,#11866,.F.);
#15775=ORIENTED_EDGE('',*,*,#11871,.F.);
#15776=ORIENTED_EDGE('',*,*,#11872,.T.);
#15777=ORIENTED_EDGE('',*,*,#11873,.T.);
#15778=ORIENTED_EDGE('',*,*,#11869,.F.);
#15779=ORIENTED_EDGE('',*,*,#11874,.F.);
#15780=ORIENTED_EDGE('',*,*,#11875,.T.);
#15781=ORIENTED_EDGE('',*,*,#11876,.T.);
#15782=ORIENTED_EDGE('',*,*,#11872,.F.);
#15783=ORIENTED_EDGE('',*,*,#11877,.F.);
#15784=ORIENTED_EDGE('',*,*,#11878,.T.);
#15785=ORIENTED_EDGE('',*,*,#11879,.T.);
#15786=ORIENTED_EDGE('',*,*,#11875,.F.);
#15787=ORIENTED_EDGE('',*,*,#11880,.F.);
#15788=ORIENTED_EDGE('',*,*,#11881,.T.);
#15789=ORIENTED_EDGE('',*,*,#11882,.T.);
#15790=ORIENTED_EDGE('',*,*,#11878,.F.);
#15791=ORIENTED_EDGE('',*,*,#11883,.F.);
#15792=ORIENTED_EDGE('',*,*,#11884,.F.);
#15793=ORIENTED_EDGE('',*,*,#11885,.F.);
#15794=ORIENTED_EDGE('',*,*,#11886,.F.);
#15795=ORIENTED_EDGE('',*,*,#11887,.T.);
#15796=ORIENTED_EDGE('',*,*,#11888,.T.);
#15797=ORIENTED_EDGE('',*,*,#11889,.T.);
#15798=ORIENTED_EDGE('',*,*,#11890,.T.);
#15799=ORIENTED_EDGE('',*,*,#11891,.T.);
#15800=ORIENTED_EDGE('',*,*,#11892,.T.);
#15801=ORIENTED_EDGE('',*,*,#11891,.F.);
#15802=ORIENTED_EDGE('',*,*,#11893,.T.);
#15803=ORIENTED_EDGE('',*,*,#11894,.T.);
#15804=ORIENTED_EDGE('',*,*,#11895,.T.);
#15805=ORIENTED_EDGE('',*,*,#11896,.T.);
#15806=ORIENTED_EDGE('',*,*,#11888,.F.);
#15807=ORIENTED_EDGE('',*,*,#11897,.T.);
#15808=ORIENTED_EDGE('',*,*,#11898,.T.);
#15809=ORIENTED_EDGE('',*,*,#11899,.T.);
#15810=ORIENTED_EDGE('',*,*,#11895,.F.);
#15811=ORIENTED_EDGE('',*,*,#11900,.T.);
#15812=ORIENTED_EDGE('',*,*,#11901,.T.);
#15813=ORIENTED_EDGE('',*,*,#11902,.T.);
#15814=ORIENTED_EDGE('',*,*,#11898,.F.);
#15815=ORIENTED_EDGE('',*,*,#11903,.T.);
#15816=ORIENTED_EDGE('',*,*,#11904,.T.);
#15817=ORIENTED_EDGE('',*,*,#11905,.T.);
#15818=ORIENTED_EDGE('',*,*,#11901,.F.);
#15819=ORIENTED_EDGE('',*,*,#11906,.T.);
#15820=ORIENTED_EDGE('',*,*,#11907,.T.);
#15821=ORIENTED_EDGE('',*,*,#11908,.T.);
#15822=ORIENTED_EDGE('',*,*,#11904,.F.);
#15823=ORIENTED_EDGE('',*,*,#11909,.T.);
#15824=ORIENTED_EDGE('',*,*,#11910,.T.);
#15825=ORIENTED_EDGE('',*,*,#11911,.T.);
#15826=ORIENTED_EDGE('',*,*,#11907,.F.);
#15827=ORIENTED_EDGE('',*,*,#11912,.T.);
#15828=ORIENTED_EDGE('',*,*,#11913,.T.);
#15829=ORIENTED_EDGE('',*,*,#11914,.T.);
#15830=ORIENTED_EDGE('',*,*,#11910,.F.);
#15831=ORIENTED_EDGE('',*,*,#11915,.T.);
#15832=ORIENTED_EDGE('',*,*,#11916,.T.);
#15833=ORIENTED_EDGE('',*,*,#11917,.T.);
#15834=ORIENTED_EDGE('',*,*,#11913,.F.);
#15835=ORIENTED_EDGE('',*,*,#11918,.T.);
#15836=ORIENTED_EDGE('',*,*,#11919,.T.);
#15837=ORIENTED_EDGE('',*,*,#11920,.T.);
#15838=ORIENTED_EDGE('',*,*,#11916,.F.);
#15839=ORIENTED_EDGE('',*,*,#11921,.T.);
#15840=ORIENTED_EDGE('',*,*,#11922,.T.);
#15841=ORIENTED_EDGE('',*,*,#11923,.T.);
#15842=ORIENTED_EDGE('',*,*,#11919,.F.);
#15843=ORIENTED_EDGE('',*,*,#11924,.T.);
#15844=ORIENTED_EDGE('',*,*,#11925,.T.);
#15845=ORIENTED_EDGE('',*,*,#11926,.T.);
#15846=ORIENTED_EDGE('',*,*,#11922,.F.);
#15847=ORIENTED_EDGE('',*,*,#11927,.T.);
#15848=ORIENTED_EDGE('',*,*,#11928,.T.);
#15849=ORIENTED_EDGE('',*,*,#11929,.T.);
#15850=ORIENTED_EDGE('',*,*,#11925,.F.);
#15851=ORIENTED_EDGE('',*,*,#11930,.T.);
#15852=ORIENTED_EDGE('',*,*,#11931,.T.);
#15853=ORIENTED_EDGE('',*,*,#11932,.T.);
#15854=ORIENTED_EDGE('',*,*,#11928,.F.);
#15855=ORIENTED_EDGE('',*,*,#11933,.T.);
#15856=ORIENTED_EDGE('',*,*,#11934,.F.);
#15857=ORIENTED_EDGE('',*,*,#11935,.T.);
#15858=ORIENTED_EDGE('',*,*,#11936,.F.);
#15859=ORIENTED_EDGE('',*,*,#11937,.T.);
#15860=ORIENTED_EDGE('',*,*,#11938,.T.);
#15861=ORIENTED_EDGE('',*,*,#11939,.T.);
#15862=ORIENTED_EDGE('',*,*,#11940,.F.);
#15863=ORIENTED_EDGE('',*,*,#11941,.F.);
#15864=ORIENTED_EDGE('',*,*,#11942,.T.);
#15865=ORIENTED_EDGE('',*,*,#11943,.T.);
#15866=ORIENTED_EDGE('',*,*,#11938,.F.);
#15867=ORIENTED_EDGE('',*,*,#11944,.F.);
#15868=ORIENTED_EDGE('',*,*,#11945,.T.);
#15869=ORIENTED_EDGE('',*,*,#11946,.T.);
#15870=ORIENTED_EDGE('',*,*,#11942,.F.);
#15871=ORIENTED_EDGE('',*,*,#11947,.F.);
#15872=ORIENTED_EDGE('',*,*,#11948,.T.);
#15873=ORIENTED_EDGE('',*,*,#11949,.T.);
#15874=ORIENTED_EDGE('',*,*,#11945,.F.);
#15875=ORIENTED_EDGE('',*,*,#11950,.F.);
#15876=ORIENTED_EDGE('',*,*,#11951,.T.);
#15877=ORIENTED_EDGE('',*,*,#11952,.T.);
#15878=ORIENTED_EDGE('',*,*,#11948,.F.);
#15879=ORIENTED_EDGE('',*,*,#11953,.F.);
#15880=ORIENTED_EDGE('',*,*,#11954,.T.);
#15881=ORIENTED_EDGE('',*,*,#11955,.T.);
#15882=ORIENTED_EDGE('',*,*,#11951,.F.);
#15883=ORIENTED_EDGE('',*,*,#11956,.F.);
#15884=ORIENTED_EDGE('',*,*,#11957,.T.);
#15885=ORIENTED_EDGE('',*,*,#11958,.T.);
#15886=ORIENTED_EDGE('',*,*,#11954,.F.);
#15887=ORIENTED_EDGE('',*,*,#11959,.F.);
#15888=ORIENTED_EDGE('',*,*,#11960,.T.);
#15889=ORIENTED_EDGE('',*,*,#11961,.T.);
#15890=ORIENTED_EDGE('',*,*,#11957,.F.);
#15891=ORIENTED_EDGE('',*,*,#11962,.F.);
#15892=ORIENTED_EDGE('',*,*,#11963,.T.);
#15893=ORIENTED_EDGE('',*,*,#11964,.T.);
#15894=ORIENTED_EDGE('',*,*,#11960,.F.);
#15895=ORIENTED_EDGE('',*,*,#11965,.F.);
#15896=ORIENTED_EDGE('',*,*,#11966,.T.);
#15897=ORIENTED_EDGE('',*,*,#11967,.T.);
#15898=ORIENTED_EDGE('',*,*,#11963,.F.);
#15899=ORIENTED_EDGE('',*,*,#11968,.F.);
#15900=ORIENTED_EDGE('',*,*,#11969,.T.);
#15901=ORIENTED_EDGE('',*,*,#11970,.T.);
#15902=ORIENTED_EDGE('',*,*,#11966,.F.);
#15903=ORIENTED_EDGE('',*,*,#11971,.F.);
#15904=ORIENTED_EDGE('',*,*,#11972,.T.);
#15905=ORIENTED_EDGE('',*,*,#11973,.T.);
#15906=ORIENTED_EDGE('',*,*,#11969,.F.);
#15907=ORIENTED_EDGE('',*,*,#11974,.F.);
#15908=ORIENTED_EDGE('',*,*,#11975,.T.);
#15909=ORIENTED_EDGE('',*,*,#11976,.T.);
#15910=ORIENTED_EDGE('',*,*,#11972,.F.);
#15911=ORIENTED_EDGE('',*,*,#11977,.F.);
#15912=ORIENTED_EDGE('',*,*,#11978,.T.);
#15913=ORIENTED_EDGE('',*,*,#11979,.T.);
#15914=ORIENTED_EDGE('',*,*,#11975,.F.);
#15915=ORIENTED_EDGE('',*,*,#11980,.F.);
#15916=ORIENTED_EDGE('',*,*,#11981,.F.);
#15917=ORIENTED_EDGE('',*,*,#11982,.F.);
#15918=ORIENTED_EDGE('',*,*,#11983,.F.);
#15919=ORIENTED_EDGE('',*,*,#11984,.T.);
#15920=ORIENTED_EDGE('',*,*,#11985,.T.);
#15921=ORIENTED_EDGE('',*,*,#11986,.T.);
#15922=ORIENTED_EDGE('',*,*,#11987,.T.);
#15923=ORIENTED_EDGE('',*,*,#11988,.T.);
#15924=ORIENTED_EDGE('',*,*,#11989,.T.);
#15925=ORIENTED_EDGE('',*,*,#11988,.F.);
#15926=ORIENTED_EDGE('',*,*,#11990,.T.);
#15927=ORIENTED_EDGE('',*,*,#11991,.T.);
#15928=ORIENTED_EDGE('',*,*,#11992,.T.);
#15929=ORIENTED_EDGE('',*,*,#11993,.T.);
#15930=ORIENTED_EDGE('',*,*,#11985,.F.);
#15931=ORIENTED_EDGE('',*,*,#11994,.T.);
#15932=ORIENTED_EDGE('',*,*,#11995,.T.);
#15933=ORIENTED_EDGE('',*,*,#11996,.T.);
#15934=ORIENTED_EDGE('',*,*,#11992,.F.);
#15935=ORIENTED_EDGE('',*,*,#11997,.T.);
#15936=ORIENTED_EDGE('',*,*,#11998,.T.);
#15937=ORIENTED_EDGE('',*,*,#11999,.T.);
#15938=ORIENTED_EDGE('',*,*,#11995,.F.);
#15939=ORIENTED_EDGE('',*,*,#12000,.T.);
#15940=ORIENTED_EDGE('',*,*,#12001,.T.);
#15941=ORIENTED_EDGE('',*,*,#12002,.T.);
#15942=ORIENTED_EDGE('',*,*,#11998,.F.);
#15943=ORIENTED_EDGE('',*,*,#12003,.T.);
#15944=ORIENTED_EDGE('',*,*,#12004,.T.);
#15945=ORIENTED_EDGE('',*,*,#12005,.T.);
#15946=ORIENTED_EDGE('',*,*,#12001,.F.);
#15947=ORIENTED_EDGE('',*,*,#12006,.T.);
#15948=ORIENTED_EDGE('',*,*,#12007,.T.);
#15949=ORIENTED_EDGE('',*,*,#12008,.T.);
#15950=ORIENTED_EDGE('',*,*,#12004,.F.);
#15951=ORIENTED_EDGE('',*,*,#12009,.T.);
#15952=ORIENTED_EDGE('',*,*,#12010,.T.);
#15953=ORIENTED_EDGE('',*,*,#12011,.T.);
#15954=ORIENTED_EDGE('',*,*,#12007,.F.);
#15955=ORIENTED_EDGE('',*,*,#12012,.T.);
#15956=ORIENTED_EDGE('',*,*,#12013,.T.);
#15957=ORIENTED_EDGE('',*,*,#12014,.T.);
#15958=ORIENTED_EDGE('',*,*,#12010,.F.);
#15959=ORIENTED_EDGE('',*,*,#12015,.T.);
#15960=ORIENTED_EDGE('',*,*,#12016,.T.);
#15961=ORIENTED_EDGE('',*,*,#12017,.T.);
#15962=ORIENTED_EDGE('',*,*,#12013,.F.);
#15963=ORIENTED_EDGE('',*,*,#12018,.T.);
#15964=ORIENTED_EDGE('',*,*,#12019,.T.);
#15965=ORIENTED_EDGE('',*,*,#12020,.T.);
#15966=ORIENTED_EDGE('',*,*,#12016,.F.);
#15967=ORIENTED_EDGE('',*,*,#12021,.T.);
#15968=ORIENTED_EDGE('',*,*,#12022,.T.);
#15969=ORIENTED_EDGE('',*,*,#12023,.T.);
#15970=ORIENTED_EDGE('',*,*,#12019,.F.);
#15971=ORIENTED_EDGE('',*,*,#12024,.T.);
#15972=ORIENTED_EDGE('',*,*,#12025,.T.);
#15973=ORIENTED_EDGE('',*,*,#12026,.T.);
#15974=ORIENTED_EDGE('',*,*,#12022,.F.);
#15975=ORIENTED_EDGE('',*,*,#12027,.T.);
#15976=ORIENTED_EDGE('',*,*,#12028,.T.);
#15977=ORIENTED_EDGE('',*,*,#12029,.T.);
#15978=ORIENTED_EDGE('',*,*,#12025,.F.);
#15979=ORIENTED_EDGE('',*,*,#12030,.T.);
#15980=ORIENTED_EDGE('',*,*,#12031,.F.);
#15981=ORIENTED_EDGE('',*,*,#12032,.T.);
#15982=ORIENTED_EDGE('',*,*,#12033,.F.);
#15983=ORIENTED_EDGE('',*,*,#12034,.T.);
#15984=ORIENTED_EDGE('',*,*,#12035,.T.);
#15985=ORIENTED_EDGE('',*,*,#12036,.T.);
#15986=ORIENTED_EDGE('',*,*,#12037,.F.);
#15987=ORIENTED_EDGE('',*,*,#12038,.F.);
#15988=ORIENTED_EDGE('',*,*,#12039,.T.);
#15989=ORIENTED_EDGE('',*,*,#12040,.T.);
#15990=ORIENTED_EDGE('',*,*,#12035,.F.);
#15991=ORIENTED_EDGE('',*,*,#12041,.F.);
#15992=ORIENTED_EDGE('',*,*,#12042,.T.);
#15993=ORIENTED_EDGE('',*,*,#12043,.T.);
#15994=ORIENTED_EDGE('',*,*,#12039,.F.);
#15995=ORIENTED_EDGE('',*,*,#12044,.F.);
#15996=ORIENTED_EDGE('',*,*,#12045,.T.);
#15997=ORIENTED_EDGE('',*,*,#12046,.T.);
#15998=ORIENTED_EDGE('',*,*,#12042,.F.);
#15999=ORIENTED_EDGE('',*,*,#12047,.F.);
#16000=ORIENTED_EDGE('',*,*,#12048,.T.);
#16001=ORIENTED_EDGE('',*,*,#12049,.T.);
#16002=ORIENTED_EDGE('',*,*,#12045,.F.);
#16003=ORIENTED_EDGE('',*,*,#12050,.F.);
#16004=ORIENTED_EDGE('',*,*,#12051,.T.);
#16005=ORIENTED_EDGE('',*,*,#12052,.T.);
#16006=ORIENTED_EDGE('',*,*,#12048,.F.);
#16007=ORIENTED_EDGE('',*,*,#12053,.F.);
#16008=ORIENTED_EDGE('',*,*,#12054,.T.);
#16009=ORIENTED_EDGE('',*,*,#12055,.T.);
#16010=ORIENTED_EDGE('',*,*,#12051,.F.);
#16011=ORIENTED_EDGE('',*,*,#12056,.F.);
#16012=ORIENTED_EDGE('',*,*,#12057,.T.);
#16013=ORIENTED_EDGE('',*,*,#12058,.T.);
#16014=ORIENTED_EDGE('',*,*,#12054,.F.);
#16015=ORIENTED_EDGE('',*,*,#12059,.F.);
#16016=ORIENTED_EDGE('',*,*,#12060,.T.);
#16017=ORIENTED_EDGE('',*,*,#12061,.T.);
#16018=ORIENTED_EDGE('',*,*,#12057,.F.);
#16019=ORIENTED_EDGE('',*,*,#12062,.F.);
#16020=ORIENTED_EDGE('',*,*,#12063,.T.);
#16021=ORIENTED_EDGE('',*,*,#12064,.T.);
#16022=ORIENTED_EDGE('',*,*,#12060,.F.);
#16023=ORIENTED_EDGE('',*,*,#12065,.F.);
#16024=ORIENTED_EDGE('',*,*,#12066,.T.);
#16025=ORIENTED_EDGE('',*,*,#12067,.T.);
#16026=ORIENTED_EDGE('',*,*,#12063,.F.);
#16027=ORIENTED_EDGE('',*,*,#12068,.F.);
#16028=ORIENTED_EDGE('',*,*,#12069,.T.);
#16029=ORIENTED_EDGE('',*,*,#12070,.T.);
#16030=ORIENTED_EDGE('',*,*,#12066,.F.);
#16031=ORIENTED_EDGE('',*,*,#12071,.F.);
#16032=ORIENTED_EDGE('',*,*,#12072,.T.);
#16033=ORIENTED_EDGE('',*,*,#12073,.T.);
#16034=ORIENTED_EDGE('',*,*,#12069,.F.);
#16035=ORIENTED_EDGE('',*,*,#12074,.F.);
#16036=ORIENTED_EDGE('',*,*,#12075,.T.);
#16037=ORIENTED_EDGE('',*,*,#12076,.T.);
#16038=ORIENTED_EDGE('',*,*,#12072,.F.);
#16039=ORIENTED_EDGE('',*,*,#12077,.F.);
#16040=ORIENTED_EDGE('',*,*,#12078,.F.);
#16041=ORIENTED_EDGE('',*,*,#12079,.F.);
#16042=ORIENTED_EDGE('',*,*,#12080,.F.);
#16043=ORIENTED_EDGE('',*,*,#12081,.T.);
#16044=ORIENTED_EDGE('',*,*,#12082,.T.);
#16045=ORIENTED_EDGE('',*,*,#12083,.T.);
#16046=ORIENTED_EDGE('',*,*,#12084,.T.);
#16047=ORIENTED_EDGE('',*,*,#12085,.T.);
#16048=ORIENTED_EDGE('',*,*,#12086,.T.);
#16049=ORIENTED_EDGE('',*,*,#12085,.F.);
#16050=ORIENTED_EDGE('',*,*,#12087,.T.);
#16051=ORIENTED_EDGE('',*,*,#12088,.T.);
#16052=ORIENTED_EDGE('',*,*,#12089,.T.);
#16053=ORIENTED_EDGE('',*,*,#12090,.T.);
#16054=ORIENTED_EDGE('',*,*,#12082,.F.);
#16055=ORIENTED_EDGE('',*,*,#12091,.T.);
#16056=ORIENTED_EDGE('',*,*,#12092,.T.);
#16057=ORIENTED_EDGE('',*,*,#12093,.T.);
#16058=ORIENTED_EDGE('',*,*,#12089,.F.);
#16059=ORIENTED_EDGE('',*,*,#12094,.T.);
#16060=ORIENTED_EDGE('',*,*,#12095,.T.);
#16061=ORIENTED_EDGE('',*,*,#12096,.T.);
#16062=ORIENTED_EDGE('',*,*,#12092,.F.);
#16063=ORIENTED_EDGE('',*,*,#12097,.T.);
#16064=ORIENTED_EDGE('',*,*,#12098,.T.);
#16065=ORIENTED_EDGE('',*,*,#12099,.T.);
#16066=ORIENTED_EDGE('',*,*,#12095,.F.);
#16067=ORIENTED_EDGE('',*,*,#12100,.T.);
#16068=ORIENTED_EDGE('',*,*,#12101,.T.);
#16069=ORIENTED_EDGE('',*,*,#12102,.T.);
#16070=ORIENTED_EDGE('',*,*,#12098,.F.);
#16071=ORIENTED_EDGE('',*,*,#12103,.T.);
#16072=ORIENTED_EDGE('',*,*,#12104,.T.);
#16073=ORIENTED_EDGE('',*,*,#12105,.T.);
#16074=ORIENTED_EDGE('',*,*,#12101,.F.);
#16075=ORIENTED_EDGE('',*,*,#12106,.T.);
#16076=ORIENTED_EDGE('',*,*,#12107,.T.);
#16077=ORIENTED_EDGE('',*,*,#12108,.T.);
#16078=ORIENTED_EDGE('',*,*,#12104,.F.);
#16079=ORIENTED_EDGE('',*,*,#12109,.T.);
#16080=ORIENTED_EDGE('',*,*,#12110,.T.);
#16081=ORIENTED_EDGE('',*,*,#12111,.T.);
#16082=ORIENTED_EDGE('',*,*,#12107,.F.);
#16083=ORIENTED_EDGE('',*,*,#12112,.T.);
#16084=ORIENTED_EDGE('',*,*,#12113,.T.);
#16085=ORIENTED_EDGE('',*,*,#12114,.T.);
#16086=ORIENTED_EDGE('',*,*,#12110,.F.);
#16087=ORIENTED_EDGE('',*,*,#12115,.T.);
#16088=ORIENTED_EDGE('',*,*,#12116,.T.);
#16089=ORIENTED_EDGE('',*,*,#12117,.T.);
#16090=ORIENTED_EDGE('',*,*,#12113,.F.);
#16091=ORIENTED_EDGE('',*,*,#12118,.T.);
#16092=ORIENTED_EDGE('',*,*,#12119,.T.);
#16093=ORIENTED_EDGE('',*,*,#12120,.T.);
#16094=ORIENTED_EDGE('',*,*,#12116,.F.);
#16095=ORIENTED_EDGE('',*,*,#12121,.T.);
#16096=ORIENTED_EDGE('',*,*,#12122,.T.);
#16097=ORIENTED_EDGE('',*,*,#12123,.T.);
#16098=ORIENTED_EDGE('',*,*,#12119,.F.);
#16099=ORIENTED_EDGE('',*,*,#12124,.T.);
#16100=ORIENTED_EDGE('',*,*,#12125,.T.);
#16101=ORIENTED_EDGE('',*,*,#12126,.T.);
#16102=ORIENTED_EDGE('',*,*,#12122,.F.);
#16103=ORIENTED_EDGE('',*,*,#12127,.T.);
#16104=ORIENTED_EDGE('',*,*,#12128,.F.);
#16105=ORIENTED_EDGE('',*,*,#12129,.T.);
#16106=ORIENTED_EDGE('',*,*,#12130,.F.);
#16107=ORIENTED_EDGE('',*,*,#12131,.T.);
#16108=ORIENTED_EDGE('',*,*,#12132,.T.);
#16109=ORIENTED_EDGE('',*,*,#12133,.T.);
#16110=ORIENTED_EDGE('',*,*,#12134,.F.);
#16111=ORIENTED_EDGE('',*,*,#12135,.F.);
#16112=ORIENTED_EDGE('',*,*,#12136,.T.);
#16113=ORIENTED_EDGE('',*,*,#12137,.T.);
#16114=ORIENTED_EDGE('',*,*,#12132,.F.);
#16115=ORIENTED_EDGE('',*,*,#12138,.F.);
#16116=ORIENTED_EDGE('',*,*,#12139,.T.);
#16117=ORIENTED_EDGE('',*,*,#12140,.T.);
#16118=ORIENTED_EDGE('',*,*,#12136,.F.);
#16119=ORIENTED_EDGE('',*,*,#12141,.F.);
#16120=ORIENTED_EDGE('',*,*,#12142,.T.);
#16121=ORIENTED_EDGE('',*,*,#12143,.T.);
#16122=ORIENTED_EDGE('',*,*,#12139,.F.);
#16123=ORIENTED_EDGE('',*,*,#12144,.F.);
#16124=ORIENTED_EDGE('',*,*,#12145,.T.);
#16125=ORIENTED_EDGE('',*,*,#12146,.T.);
#16126=ORIENTED_EDGE('',*,*,#12142,.F.);
#16127=ORIENTED_EDGE('',*,*,#12147,.F.);
#16128=ORIENTED_EDGE('',*,*,#12148,.T.);
#16129=ORIENTED_EDGE('',*,*,#12149,.T.);
#16130=ORIENTED_EDGE('',*,*,#12145,.F.);
#16131=ORIENTED_EDGE('',*,*,#12150,.F.);
#16132=ORIENTED_EDGE('',*,*,#12151,.T.);
#16133=ORIENTED_EDGE('',*,*,#12152,.T.);
#16134=ORIENTED_EDGE('',*,*,#12148,.F.);
#16135=ORIENTED_EDGE('',*,*,#12153,.F.);
#16136=ORIENTED_EDGE('',*,*,#12154,.T.);
#16137=ORIENTED_EDGE('',*,*,#12155,.T.);
#16138=ORIENTED_EDGE('',*,*,#12151,.F.);
#16139=ORIENTED_EDGE('',*,*,#12156,.F.);
#16140=ORIENTED_EDGE('',*,*,#12157,.T.);
#16141=ORIENTED_EDGE('',*,*,#12158,.T.);
#16142=ORIENTED_EDGE('',*,*,#12154,.F.);
#16143=ORIENTED_EDGE('',*,*,#12159,.F.);
#16144=ORIENTED_EDGE('',*,*,#12160,.T.);
#16145=ORIENTED_EDGE('',*,*,#12161,.T.);
#16146=ORIENTED_EDGE('',*,*,#12157,.F.);
#16147=ORIENTED_EDGE('',*,*,#12162,.F.);
#16148=ORIENTED_EDGE('',*,*,#12163,.T.);
#16149=ORIENTED_EDGE('',*,*,#12164,.T.);
#16150=ORIENTED_EDGE('',*,*,#12160,.F.);
#16151=ORIENTED_EDGE('',*,*,#12165,.F.);
#16152=ORIENTED_EDGE('',*,*,#12166,.T.);
#16153=ORIENTED_EDGE('',*,*,#12167,.T.);
#16154=ORIENTED_EDGE('',*,*,#12163,.F.);
#16155=ORIENTED_EDGE('',*,*,#12168,.F.);
#16156=ORIENTED_EDGE('',*,*,#12169,.T.);
#16157=ORIENTED_EDGE('',*,*,#12170,.T.);
#16158=ORIENTED_EDGE('',*,*,#12166,.F.);
#16159=ORIENTED_EDGE('',*,*,#12171,.F.);
#16160=ORIENTED_EDGE('',*,*,#12172,.T.);
#16161=ORIENTED_EDGE('',*,*,#12173,.T.);
#16162=ORIENTED_EDGE('',*,*,#12169,.F.);
#16163=ORIENTED_EDGE('',*,*,#12174,.F.);
#16164=ORIENTED_EDGE('',*,*,#12175,.F.);
#16165=ORIENTED_EDGE('',*,*,#12176,.F.);
#16166=ORIENTED_EDGE('',*,*,#12177,.F.);
#16167=ORIENTED_EDGE('',*,*,#12178,.T.);
#16168=ORIENTED_EDGE('',*,*,#12179,.T.);
#16169=ORIENTED_EDGE('',*,*,#12180,.T.);
#16170=ORIENTED_EDGE('',*,*,#12181,.T.);
#16171=ORIENTED_EDGE('',*,*,#12182,.T.);
#16172=ORIENTED_EDGE('',*,*,#12183,.T.);
#16173=ORIENTED_EDGE('',*,*,#12182,.F.);
#16174=ORIENTED_EDGE('',*,*,#12184,.T.);
#16175=ORIENTED_EDGE('',*,*,#12185,.T.);
#16176=ORIENTED_EDGE('',*,*,#12186,.T.);
#16177=ORIENTED_EDGE('',*,*,#12187,.T.);
#16178=ORIENTED_EDGE('',*,*,#12179,.F.);
#16179=ORIENTED_EDGE('',*,*,#12188,.T.);
#16180=ORIENTED_EDGE('',*,*,#12189,.T.);
#16181=ORIENTED_EDGE('',*,*,#12190,.T.);
#16182=ORIENTED_EDGE('',*,*,#12186,.F.);
#16183=ORIENTED_EDGE('',*,*,#12191,.T.);
#16184=ORIENTED_EDGE('',*,*,#12192,.T.);
#16185=ORIENTED_EDGE('',*,*,#12193,.T.);
#16186=ORIENTED_EDGE('',*,*,#12189,.F.);
#16187=ORIENTED_EDGE('',*,*,#12194,.T.);
#16188=ORIENTED_EDGE('',*,*,#12195,.T.);
#16189=ORIENTED_EDGE('',*,*,#12196,.T.);
#16190=ORIENTED_EDGE('',*,*,#12192,.F.);
#16191=ORIENTED_EDGE('',*,*,#12197,.T.);
#16192=ORIENTED_EDGE('',*,*,#12198,.T.);
#16193=ORIENTED_EDGE('',*,*,#12199,.T.);
#16194=ORIENTED_EDGE('',*,*,#12195,.F.);
#16195=ORIENTED_EDGE('',*,*,#12200,.T.);
#16196=ORIENTED_EDGE('',*,*,#12201,.T.);
#16197=ORIENTED_EDGE('',*,*,#12202,.T.);
#16198=ORIENTED_EDGE('',*,*,#12198,.F.);
#16199=ORIENTED_EDGE('',*,*,#12203,.T.);
#16200=ORIENTED_EDGE('',*,*,#12204,.T.);
#16201=ORIENTED_EDGE('',*,*,#12205,.T.);
#16202=ORIENTED_EDGE('',*,*,#12201,.F.);
#16203=ORIENTED_EDGE('',*,*,#12206,.T.);
#16204=ORIENTED_EDGE('',*,*,#12207,.T.);
#16205=ORIENTED_EDGE('',*,*,#12208,.T.);
#16206=ORIENTED_EDGE('',*,*,#12204,.F.);
#16207=ORIENTED_EDGE('',*,*,#12209,.T.);
#16208=ORIENTED_EDGE('',*,*,#12210,.T.);
#16209=ORIENTED_EDGE('',*,*,#12211,.T.);
#16210=ORIENTED_EDGE('',*,*,#12207,.F.);
#16211=ORIENTED_EDGE('',*,*,#12212,.T.);
#16212=ORIENTED_EDGE('',*,*,#12213,.T.);
#16213=ORIENTED_EDGE('',*,*,#12214,.T.);
#16214=ORIENTED_EDGE('',*,*,#12210,.F.);
#16215=ORIENTED_EDGE('',*,*,#12215,.T.);
#16216=ORIENTED_EDGE('',*,*,#12216,.T.);
#16217=ORIENTED_EDGE('',*,*,#12217,.T.);
#16218=ORIENTED_EDGE('',*,*,#12213,.F.);
#16219=ORIENTED_EDGE('',*,*,#12218,.T.);
#16220=ORIENTED_EDGE('',*,*,#12219,.T.);
#16221=ORIENTED_EDGE('',*,*,#12220,.T.);
#16222=ORIENTED_EDGE('',*,*,#12216,.F.);
#16223=ORIENTED_EDGE('',*,*,#12221,.T.);
#16224=ORIENTED_EDGE('',*,*,#12222,.T.);
#16225=ORIENTED_EDGE('',*,*,#12223,.T.);
#16226=ORIENTED_EDGE('',*,*,#12219,.F.);
#16227=ORIENTED_EDGE('',*,*,#12224,.T.);
#16228=ORIENTED_EDGE('',*,*,#12225,.F.);
#16229=ORIENTED_EDGE('',*,*,#12226,.T.);
#16230=ORIENTED_EDGE('',*,*,#12227,.F.);
#16231=ORIENTED_EDGE('',*,*,#12228,.T.);
#16232=ORIENTED_EDGE('',*,*,#12229,.T.);
#16233=ORIENTED_EDGE('',*,*,#12230,.T.);
#16234=ORIENTED_EDGE('',*,*,#12231,.F.);
#16235=ORIENTED_EDGE('',*,*,#12232,.F.);
#16236=ORIENTED_EDGE('',*,*,#12233,.T.);
#16237=ORIENTED_EDGE('',*,*,#12234,.T.);
#16238=ORIENTED_EDGE('',*,*,#12229,.F.);
#16239=ORIENTED_EDGE('',*,*,#12235,.F.);
#16240=ORIENTED_EDGE('',*,*,#12236,.T.);
#16241=ORIENTED_EDGE('',*,*,#12237,.T.);
#16242=ORIENTED_EDGE('',*,*,#12233,.F.);
#16243=ORIENTED_EDGE('',*,*,#12238,.F.);
#16244=ORIENTED_EDGE('',*,*,#12239,.T.);
#16245=ORIENTED_EDGE('',*,*,#12240,.T.);
#16246=ORIENTED_EDGE('',*,*,#12236,.F.);
#16247=ORIENTED_EDGE('',*,*,#12241,.F.);
#16248=ORIENTED_EDGE('',*,*,#12242,.T.);
#16249=ORIENTED_EDGE('',*,*,#12243,.T.);
#16250=ORIENTED_EDGE('',*,*,#12239,.F.);
#16251=ORIENTED_EDGE('',*,*,#12244,.F.);
#16252=ORIENTED_EDGE('',*,*,#12245,.T.);
#16253=ORIENTED_EDGE('',*,*,#12246,.T.);
#16254=ORIENTED_EDGE('',*,*,#12242,.F.);
#16255=ORIENTED_EDGE('',*,*,#12247,.F.);
#16256=ORIENTED_EDGE('',*,*,#12248,.T.);
#16257=ORIENTED_EDGE('',*,*,#12249,.T.);
#16258=ORIENTED_EDGE('',*,*,#12245,.F.);
#16259=ORIENTED_EDGE('',*,*,#12250,.F.);
#16260=ORIENTED_EDGE('',*,*,#12251,.T.);
#16261=ORIENTED_EDGE('',*,*,#12252,.T.);
#16262=ORIENTED_EDGE('',*,*,#12248,.F.);
#16263=ORIENTED_EDGE('',*,*,#12253,.F.);
#16264=ORIENTED_EDGE('',*,*,#12254,.T.);
#16265=ORIENTED_EDGE('',*,*,#12255,.T.);
#16266=ORIENTED_EDGE('',*,*,#12251,.F.);
#16267=ORIENTED_EDGE('',*,*,#12256,.F.);
#16268=ORIENTED_EDGE('',*,*,#12257,.T.);
#16269=ORIENTED_EDGE('',*,*,#12258,.T.);
#16270=ORIENTED_EDGE('',*,*,#12254,.F.);
#16271=ORIENTED_EDGE('',*,*,#12259,.F.);
#16272=ORIENTED_EDGE('',*,*,#12260,.T.);
#16273=ORIENTED_EDGE('',*,*,#12261,.T.);
#16274=ORIENTED_EDGE('',*,*,#12257,.F.);
#16275=ORIENTED_EDGE('',*,*,#12262,.F.);
#16276=ORIENTED_EDGE('',*,*,#12263,.T.);
#16277=ORIENTED_EDGE('',*,*,#12264,.T.);
#16278=ORIENTED_EDGE('',*,*,#12260,.F.);
#16279=ORIENTED_EDGE('',*,*,#12265,.F.);
#16280=ORIENTED_EDGE('',*,*,#12266,.T.);
#16281=ORIENTED_EDGE('',*,*,#12267,.T.);
#16282=ORIENTED_EDGE('',*,*,#12263,.F.);
#16283=ORIENTED_EDGE('',*,*,#12268,.F.);
#16284=ORIENTED_EDGE('',*,*,#12269,.T.);
#16285=ORIENTED_EDGE('',*,*,#12270,.T.);
#16286=ORIENTED_EDGE('',*,*,#12266,.F.);
#16287=ORIENTED_EDGE('',*,*,#12271,.F.);
#16288=ORIENTED_EDGE('',*,*,#12272,.F.);
#16289=ORIENTED_EDGE('',*,*,#12273,.F.);
#16290=ORIENTED_EDGE('',*,*,#12274,.F.);
#16291=ORIENTED_EDGE('',*,*,#12275,.T.);
#16292=ORIENTED_EDGE('',*,*,#12276,.T.);
#16293=ORIENTED_EDGE('',*,*,#12277,.T.);
#16294=ORIENTED_EDGE('',*,*,#12278,.T.);
#16295=ORIENTED_EDGE('',*,*,#12279,.T.);
#16296=ORIENTED_EDGE('',*,*,#12280,.T.);
#16297=ORIENTED_EDGE('',*,*,#12279,.F.);
#16298=ORIENTED_EDGE('',*,*,#12281,.T.);
#16299=ORIENTED_EDGE('',*,*,#12282,.T.);
#16300=ORIENTED_EDGE('',*,*,#12283,.T.);
#16301=ORIENTED_EDGE('',*,*,#12284,.T.);
#16302=ORIENTED_EDGE('',*,*,#12276,.F.);
#16303=ORIENTED_EDGE('',*,*,#12285,.T.);
#16304=ORIENTED_EDGE('',*,*,#12286,.T.);
#16305=ORIENTED_EDGE('',*,*,#12287,.T.);
#16306=ORIENTED_EDGE('',*,*,#12283,.F.);
#16307=ORIENTED_EDGE('',*,*,#12288,.T.);
#16308=ORIENTED_EDGE('',*,*,#12289,.T.);
#16309=ORIENTED_EDGE('',*,*,#12290,.T.);
#16310=ORIENTED_EDGE('',*,*,#12286,.F.);
#16311=ORIENTED_EDGE('',*,*,#12291,.T.);
#16312=ORIENTED_EDGE('',*,*,#12292,.T.);
#16313=ORIENTED_EDGE('',*,*,#12293,.T.);
#16314=ORIENTED_EDGE('',*,*,#12289,.F.);
#16315=ORIENTED_EDGE('',*,*,#12294,.T.);
#16316=ORIENTED_EDGE('',*,*,#12295,.T.);
#16317=ORIENTED_EDGE('',*,*,#12296,.T.);
#16318=ORIENTED_EDGE('',*,*,#12292,.F.);
#16319=ORIENTED_EDGE('',*,*,#12297,.T.);
#16320=ORIENTED_EDGE('',*,*,#12298,.T.);
#16321=ORIENTED_EDGE('',*,*,#12299,.T.);
#16322=ORIENTED_EDGE('',*,*,#12295,.F.);
#16323=ORIENTED_EDGE('',*,*,#12300,.T.);
#16324=ORIENTED_EDGE('',*,*,#12301,.T.);
#16325=ORIENTED_EDGE('',*,*,#12302,.T.);
#16326=ORIENTED_EDGE('',*,*,#12298,.F.);
#16327=ORIENTED_EDGE('',*,*,#12303,.T.);
#16328=ORIENTED_EDGE('',*,*,#12304,.T.);
#16329=ORIENTED_EDGE('',*,*,#12305,.T.);
#16330=ORIENTED_EDGE('',*,*,#12301,.F.);
#16331=ORIENTED_EDGE('',*,*,#12306,.T.);
#16332=ORIENTED_EDGE('',*,*,#12307,.T.);
#16333=ORIENTED_EDGE('',*,*,#12308,.T.);
#16334=ORIENTED_EDGE('',*,*,#12304,.F.);
#16335=ORIENTED_EDGE('',*,*,#12309,.T.);
#16336=ORIENTED_EDGE('',*,*,#12310,.T.);
#16337=ORIENTED_EDGE('',*,*,#12311,.T.);
#16338=ORIENTED_EDGE('',*,*,#12307,.F.);
#16339=ORIENTED_EDGE('',*,*,#12312,.T.);
#16340=ORIENTED_EDGE('',*,*,#12313,.T.);
#16341=ORIENTED_EDGE('',*,*,#12314,.T.);
#16342=ORIENTED_EDGE('',*,*,#12310,.F.);
#16343=ORIENTED_EDGE('',*,*,#12315,.T.);
#16344=ORIENTED_EDGE('',*,*,#12316,.T.);
#16345=ORIENTED_EDGE('',*,*,#12317,.T.);
#16346=ORIENTED_EDGE('',*,*,#12313,.F.);
#16347=ORIENTED_EDGE('',*,*,#12318,.T.);
#16348=ORIENTED_EDGE('',*,*,#12319,.T.);
#16349=ORIENTED_EDGE('',*,*,#12320,.T.);
#16350=ORIENTED_EDGE('',*,*,#12316,.F.);
#16351=ORIENTED_EDGE('',*,*,#12321,.T.);
#16352=ORIENTED_EDGE('',*,*,#12322,.F.);
#16353=ORIENTED_EDGE('',*,*,#12323,.T.);
#16354=ORIENTED_EDGE('',*,*,#12324,.F.);
#16355=ORIENTED_EDGE('',*,*,#12325,.T.);
#16356=ORIENTED_EDGE('',*,*,#12326,.T.);
#16357=ORIENTED_EDGE('',*,*,#12327,.T.);
#16358=ORIENTED_EDGE('',*,*,#12328,.F.);
#16359=ORIENTED_EDGE('',*,*,#12329,.F.);
#16360=ORIENTED_EDGE('',*,*,#12330,.T.);
#16361=ORIENTED_EDGE('',*,*,#12331,.T.);
#16362=ORIENTED_EDGE('',*,*,#12326,.F.);
#16363=ORIENTED_EDGE('',*,*,#12332,.F.);
#16364=ORIENTED_EDGE('',*,*,#12333,.T.);
#16365=ORIENTED_EDGE('',*,*,#12334,.T.);
#16366=ORIENTED_EDGE('',*,*,#12330,.F.);
#16367=ORIENTED_EDGE('',*,*,#12335,.F.);
#16368=ORIENTED_EDGE('',*,*,#12336,.T.);
#16369=ORIENTED_EDGE('',*,*,#12337,.T.);
#16370=ORIENTED_EDGE('',*,*,#12333,.F.);
#16371=ORIENTED_EDGE('',*,*,#12338,.F.);
#16372=ORIENTED_EDGE('',*,*,#12339,.T.);
#16373=ORIENTED_EDGE('',*,*,#12340,.T.);
#16374=ORIENTED_EDGE('',*,*,#12336,.F.);
#16375=ORIENTED_EDGE('',*,*,#12341,.F.);
#16376=ORIENTED_EDGE('',*,*,#12342,.T.);
#16377=ORIENTED_EDGE('',*,*,#12343,.T.);
#16378=ORIENTED_EDGE('',*,*,#12339,.F.);
#16379=ORIENTED_EDGE('',*,*,#12344,.F.);
#16380=ORIENTED_EDGE('',*,*,#12345,.T.);
#16381=ORIENTED_EDGE('',*,*,#12346,.T.);
#16382=ORIENTED_EDGE('',*,*,#12342,.F.);
#16383=ORIENTED_EDGE('',*,*,#12347,.F.);
#16384=ORIENTED_EDGE('',*,*,#12348,.T.);
#16385=ORIENTED_EDGE('',*,*,#12349,.T.);
#16386=ORIENTED_EDGE('',*,*,#12345,.F.);
#16387=ORIENTED_EDGE('',*,*,#12350,.F.);
#16388=ORIENTED_EDGE('',*,*,#12351,.T.);
#16389=ORIENTED_EDGE('',*,*,#12352,.T.);
#16390=ORIENTED_EDGE('',*,*,#12348,.F.);
#16391=ORIENTED_EDGE('',*,*,#12353,.F.);
#16392=ORIENTED_EDGE('',*,*,#12354,.T.);
#16393=ORIENTED_EDGE('',*,*,#12355,.T.);
#16394=ORIENTED_EDGE('',*,*,#12351,.F.);
#16395=ORIENTED_EDGE('',*,*,#12356,.F.);
#16396=ORIENTED_EDGE('',*,*,#12357,.T.);
#16397=ORIENTED_EDGE('',*,*,#12358,.T.);
#16398=ORIENTED_EDGE('',*,*,#12354,.F.);
#16399=ORIENTED_EDGE('',*,*,#12359,.F.);
#16400=ORIENTED_EDGE('',*,*,#12360,.T.);
#16401=ORIENTED_EDGE('',*,*,#12361,.T.);
#16402=ORIENTED_EDGE('',*,*,#12357,.F.);
#16403=ORIENTED_EDGE('',*,*,#12362,.F.);
#16404=ORIENTED_EDGE('',*,*,#12363,.T.);
#16405=ORIENTED_EDGE('',*,*,#12364,.T.);
#16406=ORIENTED_EDGE('',*,*,#12360,.F.);
#16407=ORIENTED_EDGE('',*,*,#12365,.F.);
#16408=ORIENTED_EDGE('',*,*,#12366,.T.);
#16409=ORIENTED_EDGE('',*,*,#12367,.T.);
#16410=ORIENTED_EDGE('',*,*,#12363,.F.);
#16411=ORIENTED_EDGE('',*,*,#12368,.F.);
#16412=ORIENTED_EDGE('',*,*,#12369,.F.);
#16413=ORIENTED_EDGE('',*,*,#12370,.F.);
#16414=ORIENTED_EDGE('',*,*,#12371,.F.);
#16415=ORIENTED_EDGE('',*,*,#12372,.T.);
#16416=ORIENTED_EDGE('',*,*,#12373,.F.);
#16417=ORIENTED_EDGE('',*,*,#12374,.T.);
#16418=ORIENTED_EDGE('',*,*,#12375,.F.);
#16419=ORIENTED_EDGE('',*,*,#12376,.F.);
#16420=ORIENTED_EDGE('',*,*,#12374,.F.);
#16421=ORIENTED_EDGE('',*,*,#12377,.F.);
#16422=ORIENTED_EDGE('',*,*,#12378,.F.);
#16423=ORIENTED_EDGE('',*,*,#12379,.F.);
#16424=ORIENTED_EDGE('',*,*,#12380,.T.);
#16425=ORIENTED_EDGE('',*,*,#12381,.F.);
#16426=ORIENTED_EDGE('',*,*,#12382,.F.);
#16427=ORIENTED_EDGE('',*,*,#12380,.F.);
#16428=ORIENTED_EDGE('',*,*,#12383,.F.);
#16429=ORIENTED_EDGE('',*,*,#12384,.F.);
#16430=ORIENTED_EDGE('',*,*,#12385,.T.);
#16431=ORIENTED_EDGE('',*,*,#12386,.F.);
#16432=ORIENTED_EDGE('',*,*,#12387,.F.);
#16433=ORIENTED_EDGE('',*,*,#12388,.F.);
#16434=ORIENTED_EDGE('',*,*,#12385,.F.);
#16435=ORIENTED_EDGE('',*,*,#12389,.F.);
#16436=ORIENTED_EDGE('',*,*,#12390,.F.);
#16437=ORIENTED_EDGE('',*,*,#12391,.F.);
#16438=ORIENTED_EDGE('',*,*,#12392,.T.);
#16439=ORIENTED_EDGE('',*,*,#12393,.F.);
#16440=ORIENTED_EDGE('',*,*,#12392,.F.);
#16441=ORIENTED_EDGE('',*,*,#12394,.F.);
#16442=ORIENTED_EDGE('',*,*,#12395,.F.);
#16443=ORIENTED_EDGE('',*,*,#12396,.T.);
#16444=ORIENTED_EDGE('',*,*,#12397,.F.);
#16445=ORIENTED_EDGE('',*,*,#12398,.F.);
#16446=ORIENTED_EDGE('',*,*,#12396,.F.);
#16447=ORIENTED_EDGE('',*,*,#12399,.F.);
#16448=ORIENTED_EDGE('',*,*,#12400,.F.);
#16449=ORIENTED_EDGE('',*,*,#12401,.F.);
#16450=ORIENTED_EDGE('',*,*,#12402,.T.);
#16451=ORIENTED_EDGE('',*,*,#12403,.F.);
#16452=ORIENTED_EDGE('',*,*,#12404,.F.);
#16453=ORIENTED_EDGE('',*,*,#12402,.F.);
#16454=ORIENTED_EDGE('',*,*,#12405,.F.);
#16455=ORIENTED_EDGE('',*,*,#12406,.F.);
#16456=ORIENTED_EDGE('',*,*,#12407,.T.);
#16457=ORIENTED_EDGE('',*,*,#12408,.F.);
#16458=ORIENTED_EDGE('',*,*,#12409,.F.);
#16459=ORIENTED_EDGE('',*,*,#12410,.F.);
#16460=ORIENTED_EDGE('',*,*,#12407,.F.);
#16461=ORIENTED_EDGE('',*,*,#12411,.F.);
#16462=ORIENTED_EDGE('',*,*,#12412,.F.);
#16463=ORIENTED_EDGE('',*,*,#12413,.F.);
#16464=ORIENTED_EDGE('',*,*,#12414,.T.);
#16465=ORIENTED_EDGE('',*,*,#12415,.F.);
#16466=ORIENTED_EDGE('',*,*,#12414,.F.);
#16467=ORIENTED_EDGE('',*,*,#12416,.F.);
#16468=ORIENTED_EDGE('',*,*,#12417,.F.);
#16469=ORIENTED_EDGE('',*,*,#12418,.T.);
#16470=ORIENTED_EDGE('',*,*,#12419,.F.);
#16471=ORIENTED_EDGE('',*,*,#12420,.F.);
#16472=ORIENTED_EDGE('',*,*,#12418,.F.);
#16473=ORIENTED_EDGE('',*,*,#12421,.F.);
#16474=ORIENTED_EDGE('',*,*,#12422,.F.);
#16475=ORIENTED_EDGE('',*,*,#12423,.F.);
#16476=ORIENTED_EDGE('',*,*,#12424,.T.);
#16477=ORIENTED_EDGE('',*,*,#12425,.F.);
#16478=ORIENTED_EDGE('',*,*,#12426,.F.);
#16479=ORIENTED_EDGE('',*,*,#12424,.F.);
#16480=ORIENTED_EDGE('',*,*,#12427,.F.);
#16481=ORIENTED_EDGE('',*,*,#12428,.F.);
#16482=ORIENTED_EDGE('',*,*,#12429,.T.);
#16483=ORIENTED_EDGE('',*,*,#12430,.F.);
#16484=ORIENTED_EDGE('',*,*,#12431,.F.);
#16485=ORIENTED_EDGE('',*,*,#12432,.F.);
#16486=ORIENTED_EDGE('',*,*,#12429,.F.);
#16487=ORIENTED_EDGE('',*,*,#12433,.F.);
#16488=ORIENTED_EDGE('',*,*,#12434,.F.);
#16489=ORIENTED_EDGE('',*,*,#12435,.F.);
#16490=ORIENTED_EDGE('',*,*,#12436,.T.);
#16491=ORIENTED_EDGE('',*,*,#12437,.F.);
#16492=ORIENTED_EDGE('',*,*,#12436,.F.);
#16493=ORIENTED_EDGE('',*,*,#12438,.F.);
#16494=ORIENTED_EDGE('',*,*,#12278,.F.);
#16495=ORIENTED_EDGE('',*,*,#12439,.T.);
#16496=ORIENTED_EDGE('',*,*,#12328,.T.);
#16497=ORIENTED_EDGE('',*,*,#12440,.T.);
#16498=ORIENTED_EDGE('',*,*,#12281,.F.);
#16499=ORIENTED_EDGE('',*,*,#12369,.T.);
#16500=ORIENTED_EDGE('',*,*,#12441,.T.);
#16501=ORIENTED_EDGE('',*,*,#12366,.F.);
#16502=ORIENTED_EDGE('',*,*,#12442,.F.);
#16503=ORIENTED_EDGE('',*,*,#12440,.F.);
#16504=ORIENTED_EDGE('',*,*,#12327,.F.);
#16505=ORIENTED_EDGE('',*,*,#12331,.F.);
#16506=ORIENTED_EDGE('',*,*,#12334,.F.);
#16507=ORIENTED_EDGE('',*,*,#12337,.F.);
#16508=ORIENTED_EDGE('',*,*,#12340,.F.);
#16509=ORIENTED_EDGE('',*,*,#12343,.F.);
#16510=ORIENTED_EDGE('',*,*,#12346,.F.);
#16511=ORIENTED_EDGE('',*,*,#12349,.F.);
#16512=ORIENTED_EDGE('',*,*,#12352,.F.);
#16513=ORIENTED_EDGE('',*,*,#12355,.F.);
#16514=ORIENTED_EDGE('',*,*,#12358,.F.);
#16515=ORIENTED_EDGE('',*,*,#12361,.F.);
#16516=ORIENTED_EDGE('',*,*,#12364,.F.);
#16517=ORIENTED_EDGE('',*,*,#12367,.F.);
#16518=ORIENTED_EDGE('',*,*,#12441,.F.);
#16519=ORIENTED_EDGE('',*,*,#12372,.F.);
#16520=ORIENTED_EDGE('',*,*,#12443,.F.);
#16521=ORIENTED_EDGE('',*,*,#12323,.F.);
#16522=ORIENTED_EDGE('',*,*,#12444,.F.);
#16523=ORIENTED_EDGE('',*,*,#12321,.F.);
#16524=ORIENTED_EDGE('',*,*,#12318,.F.);
#16525=ORIENTED_EDGE('',*,*,#12315,.F.);
#16526=ORIENTED_EDGE('',*,*,#12312,.F.);
#16527=ORIENTED_EDGE('',*,*,#12309,.F.);
#16528=ORIENTED_EDGE('',*,*,#12306,.F.);
#16529=ORIENTED_EDGE('',*,*,#12303,.F.);
#16530=ORIENTED_EDGE('',*,*,#12300,.F.);
#16531=ORIENTED_EDGE('',*,*,#12297,.F.);
#16532=ORIENTED_EDGE('',*,*,#12294,.F.);
#16533=ORIENTED_EDGE('',*,*,#12291,.F.);
#16534=ORIENTED_EDGE('',*,*,#12288,.F.);
#16535=ORIENTED_EDGE('',*,*,#12285,.F.);
#16536=ORIENTED_EDGE('',*,*,#12282,.F.);
#16537=ORIENTED_EDGE('',*,*,#12439,.F.);
#16538=ORIENTED_EDGE('',*,*,#12277,.F.);
#16539=ORIENTED_EDGE('',*,*,#12284,.F.);
#16540=ORIENTED_EDGE('',*,*,#12287,.F.);
#16541=ORIENTED_EDGE('',*,*,#12290,.F.);
#16542=ORIENTED_EDGE('',*,*,#12293,.F.);
#16543=ORIENTED_EDGE('',*,*,#12296,.F.);
#16544=ORIENTED_EDGE('',*,*,#12299,.F.);
#16545=ORIENTED_EDGE('',*,*,#12302,.F.);
#16546=ORIENTED_EDGE('',*,*,#12305,.F.);
#16547=ORIENTED_EDGE('',*,*,#12308,.F.);
#16548=ORIENTED_EDGE('',*,*,#12311,.F.);
#16549=ORIENTED_EDGE('',*,*,#12314,.F.);
#16550=ORIENTED_EDGE('',*,*,#12317,.F.);
#16551=ORIENTED_EDGE('',*,*,#12320,.F.);
#16552=ORIENTED_EDGE('',*,*,#12445,.F.);
#16553=ORIENTED_EDGE('',*,*,#12325,.F.);
#16554=ORIENTED_EDGE('',*,*,#12446,.F.);
#16555=ORIENTED_EDGE('',*,*,#12370,.T.);
#16556=ORIENTED_EDGE('',*,*,#12442,.T.);
#16557=ORIENTED_EDGE('',*,*,#12368,.T.);
#16558=ORIENTED_EDGE('',*,*,#12365,.T.);
#16559=ORIENTED_EDGE('',*,*,#12362,.T.);
#16560=ORIENTED_EDGE('',*,*,#12359,.T.);
#16561=ORIENTED_EDGE('',*,*,#12356,.T.);
#16562=ORIENTED_EDGE('',*,*,#12353,.T.);
#16563=ORIENTED_EDGE('',*,*,#12350,.T.);
#16564=ORIENTED_EDGE('',*,*,#12347,.T.);
#16565=ORIENTED_EDGE('',*,*,#12344,.T.);
#16566=ORIENTED_EDGE('',*,*,#12341,.T.);
#16567=ORIENTED_EDGE('',*,*,#12338,.T.);
#16568=ORIENTED_EDGE('',*,*,#12335,.T.);
#16569=ORIENTED_EDGE('',*,*,#12332,.T.);
#16570=ORIENTED_EDGE('',*,*,#12329,.T.);
#16571=ORIENTED_EDGE('',*,*,#12322,.T.);
#16572=ORIENTED_EDGE('',*,*,#12445,.T.);
#16573=ORIENTED_EDGE('',*,*,#12319,.F.);
#16574=ORIENTED_EDGE('',*,*,#12444,.T.);
#16575=ORIENTED_EDGE('',*,*,#12181,.F.);
#16576=ORIENTED_EDGE('',*,*,#12447,.T.);
#16577=ORIENTED_EDGE('',*,*,#12231,.T.);
#16578=ORIENTED_EDGE('',*,*,#12448,.T.);
#16579=ORIENTED_EDGE('',*,*,#12184,.F.);
#16580=ORIENTED_EDGE('',*,*,#12272,.T.);
#16581=ORIENTED_EDGE('',*,*,#12449,.T.);
#16582=ORIENTED_EDGE('',*,*,#12269,.F.);
#16583=ORIENTED_EDGE('',*,*,#12450,.F.);
#16584=ORIENTED_EDGE('',*,*,#12448,.F.);
#16585=ORIENTED_EDGE('',*,*,#12230,.F.);
#16586=ORIENTED_EDGE('',*,*,#12234,.F.);
#16587=ORIENTED_EDGE('',*,*,#12237,.F.);
#16588=ORIENTED_EDGE('',*,*,#12240,.F.);
#16589=ORIENTED_EDGE('',*,*,#12243,.F.);
#16590=ORIENTED_EDGE('',*,*,#12246,.F.);
#16591=ORIENTED_EDGE('',*,*,#12249,.F.);
#16592=ORIENTED_EDGE('',*,*,#12252,.F.);
#16593=ORIENTED_EDGE('',*,*,#12255,.F.);
#16594=ORIENTED_EDGE('',*,*,#12258,.F.);
#16595=ORIENTED_EDGE('',*,*,#12261,.F.);
#16596=ORIENTED_EDGE('',*,*,#12264,.F.);
#16597=ORIENTED_EDGE('',*,*,#12267,.F.);
#16598=ORIENTED_EDGE('',*,*,#12270,.F.);
#16599=ORIENTED_EDGE('',*,*,#12449,.F.);
#16600=ORIENTED_EDGE('',*,*,#12275,.F.);
#16601=ORIENTED_EDGE('',*,*,#12451,.F.);
#16602=ORIENTED_EDGE('',*,*,#12226,.F.);
#16603=ORIENTED_EDGE('',*,*,#12452,.F.);
#16604=ORIENTED_EDGE('',*,*,#12224,.F.);
#16605=ORIENTED_EDGE('',*,*,#12221,.F.);
#16606=ORIENTED_EDGE('',*,*,#12218,.F.);
#16607=ORIENTED_EDGE('',*,*,#12215,.F.);
#16608=ORIENTED_EDGE('',*,*,#12212,.F.);
#16609=ORIENTED_EDGE('',*,*,#12209,.F.);
#16610=ORIENTED_EDGE('',*,*,#12206,.F.);
#16611=ORIENTED_EDGE('',*,*,#12203,.F.);
#16612=ORIENTED_EDGE('',*,*,#12200,.F.);
#16613=ORIENTED_EDGE('',*,*,#12197,.F.);
#16614=ORIENTED_EDGE('',*,*,#12194,.F.);
#16615=ORIENTED_EDGE('',*,*,#12191,.F.);
#16616=ORIENTED_EDGE('',*,*,#12188,.F.);
#16617=ORIENTED_EDGE('',*,*,#12185,.F.);
#16618=ORIENTED_EDGE('',*,*,#12447,.F.);
#16619=ORIENTED_EDGE('',*,*,#12180,.F.);
#16620=ORIENTED_EDGE('',*,*,#12187,.F.);
#16621=ORIENTED_EDGE('',*,*,#12190,.F.);
#16622=ORIENTED_EDGE('',*,*,#12193,.F.);
#16623=ORIENTED_EDGE('',*,*,#12196,.F.);
#16624=ORIENTED_EDGE('',*,*,#12199,.F.);
#16625=ORIENTED_EDGE('',*,*,#12202,.F.);
#16626=ORIENTED_EDGE('',*,*,#12205,.F.);
#16627=ORIENTED_EDGE('',*,*,#12208,.F.);
#16628=ORIENTED_EDGE('',*,*,#12211,.F.);
#16629=ORIENTED_EDGE('',*,*,#12214,.F.);
#16630=ORIENTED_EDGE('',*,*,#12217,.F.);
#16631=ORIENTED_EDGE('',*,*,#12220,.F.);
#16632=ORIENTED_EDGE('',*,*,#12223,.F.);
#16633=ORIENTED_EDGE('',*,*,#12453,.F.);
#16634=ORIENTED_EDGE('',*,*,#12228,.F.);
#16635=ORIENTED_EDGE('',*,*,#12454,.F.);
#16636=ORIENTED_EDGE('',*,*,#12273,.T.);
#16637=ORIENTED_EDGE('',*,*,#12450,.T.);
#16638=ORIENTED_EDGE('',*,*,#12271,.T.);
#16639=ORIENTED_EDGE('',*,*,#12268,.T.);
#16640=ORIENTED_EDGE('',*,*,#12265,.T.);
#16641=ORIENTED_EDGE('',*,*,#12262,.T.);
#16642=ORIENTED_EDGE('',*,*,#12259,.T.);
#16643=ORIENTED_EDGE('',*,*,#12256,.T.);
#16644=ORIENTED_EDGE('',*,*,#12253,.T.);
#16645=ORIENTED_EDGE('',*,*,#12250,.T.);
#16646=ORIENTED_EDGE('',*,*,#12247,.T.);
#16647=ORIENTED_EDGE('',*,*,#12244,.T.);
#16648=ORIENTED_EDGE('',*,*,#12241,.T.);
#16649=ORIENTED_EDGE('',*,*,#12238,.T.);
#16650=ORIENTED_EDGE('',*,*,#12235,.T.);
#16651=ORIENTED_EDGE('',*,*,#12232,.T.);
#16652=ORIENTED_EDGE('',*,*,#12225,.T.);
#16653=ORIENTED_EDGE('',*,*,#12453,.T.);
#16654=ORIENTED_EDGE('',*,*,#12222,.F.);
#16655=ORIENTED_EDGE('',*,*,#12452,.T.);
#16656=ORIENTED_EDGE('',*,*,#12084,.F.);
#16657=ORIENTED_EDGE('',*,*,#12455,.T.);
#16658=ORIENTED_EDGE('',*,*,#12134,.T.);
#16659=ORIENTED_EDGE('',*,*,#12456,.T.);
#16660=ORIENTED_EDGE('',*,*,#12087,.F.);
#16661=ORIENTED_EDGE('',*,*,#12175,.T.);
#16662=ORIENTED_EDGE('',*,*,#12457,.T.);
#16663=ORIENTED_EDGE('',*,*,#12172,.F.);
#16664=ORIENTED_EDGE('',*,*,#12458,.F.);
#16665=ORIENTED_EDGE('',*,*,#12456,.F.);
#16666=ORIENTED_EDGE('',*,*,#12133,.F.);
#16667=ORIENTED_EDGE('',*,*,#12137,.F.);
#16668=ORIENTED_EDGE('',*,*,#12140,.F.);
#16669=ORIENTED_EDGE('',*,*,#12143,.F.);
#16670=ORIENTED_EDGE('',*,*,#12146,.F.);
#16671=ORIENTED_EDGE('',*,*,#12149,.F.);
#16672=ORIENTED_EDGE('',*,*,#12152,.F.);
#16673=ORIENTED_EDGE('',*,*,#12155,.F.);
#16674=ORIENTED_EDGE('',*,*,#12158,.F.);
#16675=ORIENTED_EDGE('',*,*,#12161,.F.);
#16676=ORIENTED_EDGE('',*,*,#12164,.F.);
#16677=ORIENTED_EDGE('',*,*,#12167,.F.);
#16678=ORIENTED_EDGE('',*,*,#12170,.F.);
#16679=ORIENTED_EDGE('',*,*,#12173,.F.);
#16680=ORIENTED_EDGE('',*,*,#12457,.F.);
#16681=ORIENTED_EDGE('',*,*,#12178,.F.);
#16682=ORIENTED_EDGE('',*,*,#12459,.F.);
#16683=ORIENTED_EDGE('',*,*,#12129,.F.);
#16684=ORIENTED_EDGE('',*,*,#12460,.F.);
#16685=ORIENTED_EDGE('',*,*,#12127,.F.);
#16686=ORIENTED_EDGE('',*,*,#12124,.F.);
#16687=ORIENTED_EDGE('',*,*,#12121,.F.);
#16688=ORIENTED_EDGE('',*,*,#12118,.F.);
#16689=ORIENTED_EDGE('',*,*,#12115,.F.);
#16690=ORIENTED_EDGE('',*,*,#12112,.F.);
#16691=ORIENTED_EDGE('',*,*,#12109,.F.);
#16692=ORIENTED_EDGE('',*,*,#12106,.F.);
#16693=ORIENTED_EDGE('',*,*,#12103,.F.);
#16694=ORIENTED_EDGE('',*,*,#12100,.F.);
#16695=ORIENTED_EDGE('',*,*,#12097,.F.);
#16696=ORIENTED_EDGE('',*,*,#12094,.F.);
#16697=ORIENTED_EDGE('',*,*,#12091,.F.);
#16698=ORIENTED_EDGE('',*,*,#12088,.F.);
#16699=ORIENTED_EDGE('',*,*,#12455,.F.);
#16700=ORIENTED_EDGE('',*,*,#12083,.F.);
#16701=ORIENTED_EDGE('',*,*,#12090,.F.);
#16702=ORIENTED_EDGE('',*,*,#12093,.F.);
#16703=ORIENTED_EDGE('',*,*,#12096,.F.);
#16704=ORIENTED_EDGE('',*,*,#12099,.F.);
#16705=ORIENTED_EDGE('',*,*,#12102,.F.);
#16706=ORIENTED_EDGE('',*,*,#12105,.F.);
#16707=ORIENTED_EDGE('',*,*,#12108,.F.);
#16708=ORIENTED_EDGE('',*,*,#12111,.F.);
#16709=ORIENTED_EDGE('',*,*,#12114,.F.);
#16710=ORIENTED_EDGE('',*,*,#12117,.F.);
#16711=ORIENTED_EDGE('',*,*,#12120,.F.);
#16712=ORIENTED_EDGE('',*,*,#12123,.F.);
#16713=ORIENTED_EDGE('',*,*,#12126,.F.);
#16714=ORIENTED_EDGE('',*,*,#12461,.F.);
#16715=ORIENTED_EDGE('',*,*,#12131,.F.);
#16716=ORIENTED_EDGE('',*,*,#12462,.F.);
#16717=ORIENTED_EDGE('',*,*,#12176,.T.);
#16718=ORIENTED_EDGE('',*,*,#12458,.T.);
#16719=ORIENTED_EDGE('',*,*,#12174,.T.);
#16720=ORIENTED_EDGE('',*,*,#12171,.T.);
#16721=ORIENTED_EDGE('',*,*,#12168,.T.);
#16722=ORIENTED_EDGE('',*,*,#12165,.T.);
#16723=ORIENTED_EDGE('',*,*,#12162,.T.);
#16724=ORIENTED_EDGE('',*,*,#12159,.T.);
#16725=ORIENTED_EDGE('',*,*,#12156,.T.);
#16726=ORIENTED_EDGE('',*,*,#12153,.T.);
#16727=ORIENTED_EDGE('',*,*,#12150,.T.);
#16728=ORIENTED_EDGE('',*,*,#12147,.T.);
#16729=ORIENTED_EDGE('',*,*,#12144,.T.);
#16730=ORIENTED_EDGE('',*,*,#12141,.T.);
#16731=ORIENTED_EDGE('',*,*,#12138,.T.);
#16732=ORIENTED_EDGE('',*,*,#12135,.T.);
#16733=ORIENTED_EDGE('',*,*,#12128,.T.);
#16734=ORIENTED_EDGE('',*,*,#12461,.T.);
#16735=ORIENTED_EDGE('',*,*,#12125,.F.);
#16736=ORIENTED_EDGE('',*,*,#12460,.T.);
#16737=ORIENTED_EDGE('',*,*,#11987,.F.);
#16738=ORIENTED_EDGE('',*,*,#12463,.T.);
#16739=ORIENTED_EDGE('',*,*,#12037,.T.);
#16740=ORIENTED_EDGE('',*,*,#12464,.T.);
#16741=ORIENTED_EDGE('',*,*,#11990,.F.);
#16742=ORIENTED_EDGE('',*,*,#12078,.T.);
#16743=ORIENTED_EDGE('',*,*,#12465,.T.);
#16744=ORIENTED_EDGE('',*,*,#12075,.F.);
#16745=ORIENTED_EDGE('',*,*,#12466,.F.);
#16746=ORIENTED_EDGE('',*,*,#12464,.F.);
#16747=ORIENTED_EDGE('',*,*,#12036,.F.);
#16748=ORIENTED_EDGE('',*,*,#12040,.F.);
#16749=ORIENTED_EDGE('',*,*,#12043,.F.);
#16750=ORIENTED_EDGE('',*,*,#12046,.F.);
#16751=ORIENTED_EDGE('',*,*,#12049,.F.);
#16752=ORIENTED_EDGE('',*,*,#12052,.F.);
#16753=ORIENTED_EDGE('',*,*,#12055,.F.);
#16754=ORIENTED_EDGE('',*,*,#12058,.F.);
#16755=ORIENTED_EDGE('',*,*,#12061,.F.);
#16756=ORIENTED_EDGE('',*,*,#12064,.F.);
#16757=ORIENTED_EDGE('',*,*,#12067,.F.);
#16758=ORIENTED_EDGE('',*,*,#12070,.F.);
#16759=ORIENTED_EDGE('',*,*,#12073,.F.);
#16760=ORIENTED_EDGE('',*,*,#12076,.F.);
#16761=ORIENTED_EDGE('',*,*,#12465,.F.);
#16762=ORIENTED_EDGE('',*,*,#12081,.F.);
#16763=ORIENTED_EDGE('',*,*,#12467,.F.);
#16764=ORIENTED_EDGE('',*,*,#12032,.F.);
#16765=ORIENTED_EDGE('',*,*,#12468,.F.);
#16766=ORIENTED_EDGE('',*,*,#12030,.F.);
#16767=ORIENTED_EDGE('',*,*,#12027,.F.);
#16768=ORIENTED_EDGE('',*,*,#12024,.F.);
#16769=ORIENTED_EDGE('',*,*,#12021,.F.);
#16770=ORIENTED_EDGE('',*,*,#12018,.F.);
#16771=ORIENTED_EDGE('',*,*,#12015,.F.);
#16772=ORIENTED_EDGE('',*,*,#12012,.F.);
#16773=ORIENTED_EDGE('',*,*,#12009,.F.);
#16774=ORIENTED_EDGE('',*,*,#12006,.F.);
#16775=ORIENTED_EDGE('',*,*,#12003,.F.);
#16776=ORIENTED_EDGE('',*,*,#12000,.F.);
#16777=ORIENTED_EDGE('',*,*,#11997,.F.);
#16778=ORIENTED_EDGE('',*,*,#11994,.F.);
#16779=ORIENTED_EDGE('',*,*,#11991,.F.);
#16780=ORIENTED_EDGE('',*,*,#12463,.F.);
#16781=ORIENTED_EDGE('',*,*,#11986,.F.);
#16782=ORIENTED_EDGE('',*,*,#11993,.F.);
#16783=ORIENTED_EDGE('',*,*,#11996,.F.);
#16784=ORIENTED_EDGE('',*,*,#11999,.F.);
#16785=ORIENTED_EDGE('',*,*,#12002,.F.);
#16786=ORIENTED_EDGE('',*,*,#12005,.F.);
#16787=ORIENTED_EDGE('',*,*,#12008,.F.);
#16788=ORIENTED_EDGE('',*,*,#12011,.F.);
#16789=ORIENTED_EDGE('',*,*,#12014,.F.);
#16790=ORIENTED_EDGE('',*,*,#12017,.F.);
#16791=ORIENTED_EDGE('',*,*,#12020,.F.);
#16792=ORIENTED_EDGE('',*,*,#12023,.F.);
#16793=ORIENTED_EDGE('',*,*,#12026,.F.);
#16794=ORIENTED_EDGE('',*,*,#12029,.F.);
#16795=ORIENTED_EDGE('',*,*,#12469,.F.);
#16796=ORIENTED_EDGE('',*,*,#12034,.F.);
#16797=ORIENTED_EDGE('',*,*,#12470,.F.);
#16798=ORIENTED_EDGE('',*,*,#12079,.T.);
#16799=ORIENTED_EDGE('',*,*,#12466,.T.);
#16800=ORIENTED_EDGE('',*,*,#12077,.T.);
#16801=ORIENTED_EDGE('',*,*,#12074,.T.);
#16802=ORIENTED_EDGE('',*,*,#12071,.T.);
#16803=ORIENTED_EDGE('',*,*,#12068,.T.);
#16804=ORIENTED_EDGE('',*,*,#12065,.T.);
#16805=ORIENTED_EDGE('',*,*,#12062,.T.);
#16806=ORIENTED_EDGE('',*,*,#12059,.T.);
#16807=ORIENTED_EDGE('',*,*,#12056,.T.);
#16808=ORIENTED_EDGE('',*,*,#12053,.T.);
#16809=ORIENTED_EDGE('',*,*,#12050,.T.);
#16810=ORIENTED_EDGE('',*,*,#12047,.T.);
#16811=ORIENTED_EDGE('',*,*,#12044,.T.);
#16812=ORIENTED_EDGE('',*,*,#12041,.T.);
#16813=ORIENTED_EDGE('',*,*,#12038,.T.);
#16814=ORIENTED_EDGE('',*,*,#12031,.T.);
#16815=ORIENTED_EDGE('',*,*,#12469,.T.);
#16816=ORIENTED_EDGE('',*,*,#12028,.F.);
#16817=ORIENTED_EDGE('',*,*,#12468,.T.);
#16818=ORIENTED_EDGE('',*,*,#11890,.F.);
#16819=ORIENTED_EDGE('',*,*,#12471,.T.);
#16820=ORIENTED_EDGE('',*,*,#11940,.T.);
#16821=ORIENTED_EDGE('',*,*,#12472,.T.);
#16822=ORIENTED_EDGE('',*,*,#11893,.F.);
#16823=ORIENTED_EDGE('',*,*,#11981,.T.);
#16824=ORIENTED_EDGE('',*,*,#12473,.T.);
#16825=ORIENTED_EDGE('',*,*,#11978,.F.);
#16826=ORIENTED_EDGE('',*,*,#12474,.F.);
#16827=ORIENTED_EDGE('',*,*,#12472,.F.);
#16828=ORIENTED_EDGE('',*,*,#11939,.F.);
#16829=ORIENTED_EDGE('',*,*,#11943,.F.);
#16830=ORIENTED_EDGE('',*,*,#11946,.F.);
#16831=ORIENTED_EDGE('',*,*,#11949,.F.);
#16832=ORIENTED_EDGE('',*,*,#11952,.F.);
#16833=ORIENTED_EDGE('',*,*,#11955,.F.);
#16834=ORIENTED_EDGE('',*,*,#11958,.F.);
#16835=ORIENTED_EDGE('',*,*,#11961,.F.);
#16836=ORIENTED_EDGE('',*,*,#11964,.F.);
#16837=ORIENTED_EDGE('',*,*,#11967,.F.);
#16838=ORIENTED_EDGE('',*,*,#11970,.F.);
#16839=ORIENTED_EDGE('',*,*,#11973,.F.);
#16840=ORIENTED_EDGE('',*,*,#11976,.F.);
#16841=ORIENTED_EDGE('',*,*,#11979,.F.);
#16842=ORIENTED_EDGE('',*,*,#12473,.F.);
#16843=ORIENTED_EDGE('',*,*,#11984,.F.);
#16844=ORIENTED_EDGE('',*,*,#12475,.F.);
#16845=ORIENTED_EDGE('',*,*,#11935,.F.);
#16846=ORIENTED_EDGE('',*,*,#12476,.F.);
#16847=ORIENTED_EDGE('',*,*,#11933,.F.);
#16848=ORIENTED_EDGE('',*,*,#11930,.F.);
#16849=ORIENTED_EDGE('',*,*,#11927,.F.);
#16850=ORIENTED_EDGE('',*,*,#11924,.F.);
#16851=ORIENTED_EDGE('',*,*,#11921,.F.);
#16852=ORIENTED_EDGE('',*,*,#11918,.F.);
#16853=ORIENTED_EDGE('',*,*,#11915,.F.);
#16854=ORIENTED_EDGE('',*,*,#11912,.F.);
#16855=ORIENTED_EDGE('',*,*,#11909,.F.);
#16856=ORIENTED_EDGE('',*,*,#11906,.F.);
#16857=ORIENTED_EDGE('',*,*,#11903,.F.);
#16858=ORIENTED_EDGE('',*,*,#11900,.F.);
#16859=ORIENTED_EDGE('',*,*,#11897,.F.);
#16860=ORIENTED_EDGE('',*,*,#11894,.F.);
#16861=ORIENTED_EDGE('',*,*,#12471,.F.);
#16862=ORIENTED_EDGE('',*,*,#11889,.F.);
#16863=ORIENTED_EDGE('',*,*,#11896,.F.);
#16864=ORIENTED_EDGE('',*,*,#11899,.F.);
#16865=ORIENTED_EDGE('',*,*,#11902,.F.);
#16866=ORIENTED_EDGE('',*,*,#11905,.F.);
#16867=ORIENTED_EDGE('',*,*,#11908,.F.);
#16868=ORIENTED_EDGE('',*,*,#11911,.F.);
#16869=ORIENTED_EDGE('',*,*,#11914,.F.);
#16870=ORIENTED_EDGE('',*,*,#11917,.F.);
#16871=ORIENTED_EDGE('',*,*,#11920,.F.);
#16872=ORIENTED_EDGE('',*,*,#11923,.F.);
#16873=ORIENTED_EDGE('',*,*,#11926,.F.);
#16874=ORIENTED_EDGE('',*,*,#11929,.F.);
#16875=ORIENTED_EDGE('',*,*,#11932,.F.);
#16876=ORIENTED_EDGE('',*,*,#12477,.F.);
#16877=ORIENTED_EDGE('',*,*,#11937,.F.);
#16878=ORIENTED_EDGE('',*,*,#12478,.F.);
#16879=ORIENTED_EDGE('',*,*,#11982,.T.);
#16880=ORIENTED_EDGE('',*,*,#12474,.T.);
#16881=ORIENTED_EDGE('',*,*,#11980,.T.);
#16882=ORIENTED_EDGE('',*,*,#11977,.T.);
#16883=ORIENTED_EDGE('',*,*,#11974,.T.);
#16884=ORIENTED_EDGE('',*,*,#11971,.T.);
#16885=ORIENTED_EDGE('',*,*,#11968,.T.);
#16886=ORIENTED_EDGE('',*,*,#11965,.T.);
#16887=ORIENTED_EDGE('',*,*,#11962,.T.);
#16888=ORIENTED_EDGE('',*,*,#11959,.T.);
#16889=ORIENTED_EDGE('',*,*,#11956,.T.);
#16890=ORIENTED_EDGE('',*,*,#11953,.T.);
#16891=ORIENTED_EDGE('',*,*,#11950,.T.);
#16892=ORIENTED_EDGE('',*,*,#11947,.T.);
#16893=ORIENTED_EDGE('',*,*,#11944,.T.);
#16894=ORIENTED_EDGE('',*,*,#11941,.T.);
#16895=ORIENTED_EDGE('',*,*,#11934,.T.);
#16896=ORIENTED_EDGE('',*,*,#12477,.T.);
#16897=ORIENTED_EDGE('',*,*,#11931,.F.);
#16898=ORIENTED_EDGE('',*,*,#12476,.T.);
#16899=ORIENTED_EDGE('',*,*,#11793,.F.);
#16900=ORIENTED_EDGE('',*,*,#12479,.T.);
#16901=ORIENTED_EDGE('',*,*,#11843,.T.);
#16902=ORIENTED_EDGE('',*,*,#12480,.T.);
#16903=ORIENTED_EDGE('',*,*,#11796,.F.);
#16904=ORIENTED_EDGE('',*,*,#11884,.T.);
#16905=ORIENTED_EDGE('',*,*,#12481,.T.);
#16906=ORIENTED_EDGE('',*,*,#11881,.F.);
#16907=ORIENTED_EDGE('',*,*,#12482,.F.);
#16908=ORIENTED_EDGE('',*,*,#12480,.F.);
#16909=ORIENTED_EDGE('',*,*,#11842,.F.);
#16910=ORIENTED_EDGE('',*,*,#11846,.F.);
#16911=ORIENTED_EDGE('',*,*,#11849,.F.);
#16912=ORIENTED_EDGE('',*,*,#11852,.F.);
#16913=ORIENTED_EDGE('',*,*,#11855,.F.);
#16914=ORIENTED_EDGE('',*,*,#11858,.F.);
#16915=ORIENTED_EDGE('',*,*,#11861,.F.);
#16916=ORIENTED_EDGE('',*,*,#11864,.F.);
#16917=ORIENTED_EDGE('',*,*,#11867,.F.);
#16918=ORIENTED_EDGE('',*,*,#11870,.F.);
#16919=ORIENTED_EDGE('',*,*,#11873,.F.);
#16920=ORIENTED_EDGE('',*,*,#11876,.F.);
#16921=ORIENTED_EDGE('',*,*,#11879,.F.);
#16922=ORIENTED_EDGE('',*,*,#11882,.F.);
#16923=ORIENTED_EDGE('',*,*,#12481,.F.);
#16924=ORIENTED_EDGE('',*,*,#11887,.F.);
#16925=ORIENTED_EDGE('',*,*,#12483,.F.);
#16926=ORIENTED_EDGE('',*,*,#11838,.F.);
#16927=ORIENTED_EDGE('',*,*,#12484,.F.);
#16928=ORIENTED_EDGE('',*,*,#11836,.F.);
#16929=ORIENTED_EDGE('',*,*,#11833,.F.);
#16930=ORIENTED_EDGE('',*,*,#11830,.F.);
#16931=ORIENTED_EDGE('',*,*,#11827,.F.);
#16932=ORIENTED_EDGE('',*,*,#11824,.F.);
#16933=ORIENTED_EDGE('',*,*,#11821,.F.);
#16934=ORIENTED_EDGE('',*,*,#11818,.F.);
#16935=ORIENTED_EDGE('',*,*,#11815,.F.);
#16936=ORIENTED_EDGE('',*,*,#11812,.F.);
#16937=ORIENTED_EDGE('',*,*,#11809,.F.);
#16938=ORIENTED_EDGE('',*,*,#11806,.F.);
#16939=ORIENTED_EDGE('',*,*,#11803,.F.);
#16940=ORIENTED_EDGE('',*,*,#11800,.F.);
#16941=ORIENTED_EDGE('',*,*,#11797,.F.);
#16942=ORIENTED_EDGE('',*,*,#12479,.F.);
#16943=ORIENTED_EDGE('',*,*,#11792,.F.);
#16944=ORIENTED_EDGE('',*,*,#11799,.F.);
#16945=ORIENTED_EDGE('',*,*,#11802,.F.);
#16946=ORIENTED_EDGE('',*,*,#11805,.F.);
#16947=ORIENTED_EDGE('',*,*,#11808,.F.);
#16948=ORIENTED_EDGE('',*,*,#11811,.F.);
#16949=ORIENTED_EDGE('',*,*,#11814,.F.);
#16950=ORIENTED_EDGE('',*,*,#11817,.F.);
#16951=ORIENTED_EDGE('',*,*,#11820,.F.);
#16952=ORIENTED_EDGE('',*,*,#11823,.F.);
#16953=ORIENTED_EDGE('',*,*,#11826,.F.);
#16954=ORIENTED_EDGE('',*,*,#11829,.F.);
#16955=ORIENTED_EDGE('',*,*,#11832,.F.);
#16956=ORIENTED_EDGE('',*,*,#11835,.F.);
#16957=ORIENTED_EDGE('',*,*,#12485,.F.);
#16958=ORIENTED_EDGE('',*,*,#11840,.F.);
#16959=ORIENTED_EDGE('',*,*,#12486,.F.);
#16960=ORIENTED_EDGE('',*,*,#11885,.T.);
#16961=ORIENTED_EDGE('',*,*,#12482,.T.);
#16962=ORIENTED_EDGE('',*,*,#11883,.T.);
#16963=ORIENTED_EDGE('',*,*,#11880,.T.);
#16964=ORIENTED_EDGE('',*,*,#11877,.T.);
#16965=ORIENTED_EDGE('',*,*,#11874,.T.);
#16966=ORIENTED_EDGE('',*,*,#11871,.T.);
#16967=ORIENTED_EDGE('',*,*,#11868,.T.);
#16968=ORIENTED_EDGE('',*,*,#11865,.T.);
#16969=ORIENTED_EDGE('',*,*,#11862,.T.);
#16970=ORIENTED_EDGE('',*,*,#11859,.T.);
#16971=ORIENTED_EDGE('',*,*,#11856,.T.);
#16972=ORIENTED_EDGE('',*,*,#11853,.T.);
#16973=ORIENTED_EDGE('',*,*,#11850,.T.);
#16974=ORIENTED_EDGE('',*,*,#11847,.T.);
#16975=ORIENTED_EDGE('',*,*,#11844,.T.);
#16976=ORIENTED_EDGE('',*,*,#11837,.T.);
#16977=ORIENTED_EDGE('',*,*,#12485,.T.);
#16978=ORIENTED_EDGE('',*,*,#11834,.F.);
#16979=ORIENTED_EDGE('',*,*,#12484,.T.);
#16980=ORIENTED_EDGE('',*,*,#11696,.F.);
#16981=ORIENTED_EDGE('',*,*,#12487,.T.);
#16982=ORIENTED_EDGE('',*,*,#11746,.T.);
#16983=ORIENTED_EDGE('',*,*,#12488,.T.);
#16984=ORIENTED_EDGE('',*,*,#11699,.F.);
#16985=ORIENTED_EDGE('',*,*,#11787,.T.);
#16986=ORIENTED_EDGE('',*,*,#12489,.T.);
#16987=ORIENTED_EDGE('',*,*,#11784,.F.);
#16988=ORIENTED_EDGE('',*,*,#12490,.F.);
#16989=ORIENTED_EDGE('',*,*,#12488,.F.);
#16990=ORIENTED_EDGE('',*,*,#11745,.F.);
#16991=ORIENTED_EDGE('',*,*,#11749,.F.);
#16992=ORIENTED_EDGE('',*,*,#11752,.F.);
#16993=ORIENTED_EDGE('',*,*,#11755,.F.);
#16994=ORIENTED_EDGE('',*,*,#11758,.F.);
#16995=ORIENTED_EDGE('',*,*,#11761,.F.);
#16996=ORIENTED_EDGE('',*,*,#11764,.F.);
#16997=ORIENTED_EDGE('',*,*,#11767,.F.);
#16998=ORIENTED_EDGE('',*,*,#11770,.F.);
#16999=ORIENTED_EDGE('',*,*,#11773,.F.);
#17000=ORIENTED_EDGE('',*,*,#11776,.F.);
#17001=ORIENTED_EDGE('',*,*,#11779,.F.);
#17002=ORIENTED_EDGE('',*,*,#11782,.F.);
#17003=ORIENTED_EDGE('',*,*,#11785,.F.);
#17004=ORIENTED_EDGE('',*,*,#12489,.F.);
#17005=ORIENTED_EDGE('',*,*,#11790,.F.);
#17006=ORIENTED_EDGE('',*,*,#12491,.F.);
#17007=ORIENTED_EDGE('',*,*,#11741,.F.);
#17008=ORIENTED_EDGE('',*,*,#12492,.F.);
#17009=ORIENTED_EDGE('',*,*,#11739,.F.);
#17010=ORIENTED_EDGE('',*,*,#11736,.F.);
#17011=ORIENTED_EDGE('',*,*,#11733,.F.);
#17012=ORIENTED_EDGE('',*,*,#11730,.F.);
#17013=ORIENTED_EDGE('',*,*,#11727,.F.);
#17014=ORIENTED_EDGE('',*,*,#11724,.F.);
#17015=ORIENTED_EDGE('',*,*,#11721,.F.);
#17016=ORIENTED_EDGE('',*,*,#11718,.F.);
#17017=ORIENTED_EDGE('',*,*,#11715,.F.);
#17018=ORIENTED_EDGE('',*,*,#11712,.F.);
#17019=ORIENTED_EDGE('',*,*,#11709,.F.);
#17020=ORIENTED_EDGE('',*,*,#11706,.F.);
#17021=ORIENTED_EDGE('',*,*,#11703,.F.);
#17022=ORIENTED_EDGE('',*,*,#11700,.F.);
#17023=ORIENTED_EDGE('',*,*,#12487,.F.);
#17024=ORIENTED_EDGE('',*,*,#11695,.F.);
#17025=ORIENTED_EDGE('',*,*,#11702,.F.);
#17026=ORIENTED_EDGE('',*,*,#11705,.F.);
#17027=ORIENTED_EDGE('',*,*,#11708,.F.);
#17028=ORIENTED_EDGE('',*,*,#11711,.F.);
#17029=ORIENTED_EDGE('',*,*,#11714,.F.);
#17030=ORIENTED_EDGE('',*,*,#11717,.F.);
#17031=ORIENTED_EDGE('',*,*,#11720,.F.);
#17032=ORIENTED_EDGE('',*,*,#11723,.F.);
#17033=ORIENTED_EDGE('',*,*,#11726,.F.);
#17034=ORIENTED_EDGE('',*,*,#11729,.F.);
#17035=ORIENTED_EDGE('',*,*,#11732,.F.);
#17036=ORIENTED_EDGE('',*,*,#11735,.F.);
#17037=ORIENTED_EDGE('',*,*,#11738,.F.);
#17038=ORIENTED_EDGE('',*,*,#12493,.F.);
#17039=ORIENTED_EDGE('',*,*,#11743,.F.);
#17040=ORIENTED_EDGE('',*,*,#12494,.F.);
#17041=ORIENTED_EDGE('',*,*,#11788,.T.);
#17042=ORIENTED_EDGE('',*,*,#12490,.T.);
#17043=ORIENTED_EDGE('',*,*,#11786,.T.);
#17044=ORIENTED_EDGE('',*,*,#11783,.T.);
#17045=ORIENTED_EDGE('',*,*,#11780,.T.);
#17046=ORIENTED_EDGE('',*,*,#11777,.T.);
#17047=ORIENTED_EDGE('',*,*,#11774,.T.);
#17048=ORIENTED_EDGE('',*,*,#11771,.T.);
#17049=ORIENTED_EDGE('',*,*,#11768,.T.);
#17050=ORIENTED_EDGE('',*,*,#11765,.T.);
#17051=ORIENTED_EDGE('',*,*,#11762,.T.);
#17052=ORIENTED_EDGE('',*,*,#11759,.T.);
#17053=ORIENTED_EDGE('',*,*,#11756,.T.);
#17054=ORIENTED_EDGE('',*,*,#11753,.T.);
#17055=ORIENTED_EDGE('',*,*,#11750,.T.);
#17056=ORIENTED_EDGE('',*,*,#11747,.T.);
#17057=ORIENTED_EDGE('',*,*,#11740,.T.);
#17058=ORIENTED_EDGE('',*,*,#12493,.T.);
#17059=ORIENTED_EDGE('',*,*,#11737,.F.);
#17060=ORIENTED_EDGE('',*,*,#12492,.T.);
#17061=ORIENTED_EDGE('',*,*,#11599,.F.);
#17062=ORIENTED_EDGE('',*,*,#12495,.T.);
#17063=ORIENTED_EDGE('',*,*,#11649,.T.);
#17064=ORIENTED_EDGE('',*,*,#12496,.T.);
#17065=ORIENTED_EDGE('',*,*,#11602,.F.);
#17066=ORIENTED_EDGE('',*,*,#11690,.T.);
#17067=ORIENTED_EDGE('',*,*,#12497,.T.);
#17068=ORIENTED_EDGE('',*,*,#11687,.F.);
#17069=ORIENTED_EDGE('',*,*,#12498,.F.);
#17070=ORIENTED_EDGE('',*,*,#12496,.F.);
#17071=ORIENTED_EDGE('',*,*,#11648,.F.);
#17072=ORIENTED_EDGE('',*,*,#11652,.F.);
#17073=ORIENTED_EDGE('',*,*,#11655,.F.);
#17074=ORIENTED_EDGE('',*,*,#11658,.F.);
#17075=ORIENTED_EDGE('',*,*,#11661,.F.);
#17076=ORIENTED_EDGE('',*,*,#11664,.F.);
#17077=ORIENTED_EDGE('',*,*,#11667,.F.);
#17078=ORIENTED_EDGE('',*,*,#11670,.F.);
#17079=ORIENTED_EDGE('',*,*,#11673,.F.);
#17080=ORIENTED_EDGE('',*,*,#11676,.F.);
#17081=ORIENTED_EDGE('',*,*,#11679,.F.);
#17082=ORIENTED_EDGE('',*,*,#11682,.F.);
#17083=ORIENTED_EDGE('',*,*,#11685,.F.);
#17084=ORIENTED_EDGE('',*,*,#11688,.F.);
#17085=ORIENTED_EDGE('',*,*,#12497,.F.);
#17086=ORIENTED_EDGE('',*,*,#11693,.F.);
#17087=ORIENTED_EDGE('',*,*,#12499,.F.);
#17088=ORIENTED_EDGE('',*,*,#11644,.F.);
#17089=ORIENTED_EDGE('',*,*,#12500,.F.);
#17090=ORIENTED_EDGE('',*,*,#11642,.F.);
#17091=ORIENTED_EDGE('',*,*,#11639,.F.);
#17092=ORIENTED_EDGE('',*,*,#11636,.F.);
#17093=ORIENTED_EDGE('',*,*,#11633,.F.);
#17094=ORIENTED_EDGE('',*,*,#11630,.F.);
#17095=ORIENTED_EDGE('',*,*,#11627,.F.);
#17096=ORIENTED_EDGE('',*,*,#11624,.F.);
#17097=ORIENTED_EDGE('',*,*,#11621,.F.);
#17098=ORIENTED_EDGE('',*,*,#11618,.F.);
#17099=ORIENTED_EDGE('',*,*,#11615,.F.);
#17100=ORIENTED_EDGE('',*,*,#11612,.F.);
#17101=ORIENTED_EDGE('',*,*,#11609,.F.);
#17102=ORIENTED_EDGE('',*,*,#11606,.F.);
#17103=ORIENTED_EDGE('',*,*,#11603,.F.);
#17104=ORIENTED_EDGE('',*,*,#12495,.F.);
#17105=ORIENTED_EDGE('',*,*,#11598,.F.);
#17106=ORIENTED_EDGE('',*,*,#11605,.F.);
#17107=ORIENTED_EDGE('',*,*,#11608,.F.);
#17108=ORIENTED_EDGE('',*,*,#11611,.F.);
#17109=ORIENTED_EDGE('',*,*,#11614,.F.);
#17110=ORIENTED_EDGE('',*,*,#11617,.F.);
#17111=ORIENTED_EDGE('',*,*,#11620,.F.);
#17112=ORIENTED_EDGE('',*,*,#11623,.F.);
#17113=ORIENTED_EDGE('',*,*,#11626,.F.);
#17114=ORIENTED_EDGE('',*,*,#11629,.F.);
#17115=ORIENTED_EDGE('',*,*,#11632,.F.);
#17116=ORIENTED_EDGE('',*,*,#11635,.F.);
#17117=ORIENTED_EDGE('',*,*,#11638,.F.);
#17118=ORIENTED_EDGE('',*,*,#11641,.F.);
#17119=ORIENTED_EDGE('',*,*,#12501,.F.);
#17120=ORIENTED_EDGE('',*,*,#11646,.F.);
#17121=ORIENTED_EDGE('',*,*,#12502,.F.);
#17122=ORIENTED_EDGE('',*,*,#11691,.T.);
#17123=ORIENTED_EDGE('',*,*,#12498,.T.);
#17124=ORIENTED_EDGE('',*,*,#11689,.T.);
#17125=ORIENTED_EDGE('',*,*,#11686,.T.);
#17126=ORIENTED_EDGE('',*,*,#11683,.T.);
#17127=ORIENTED_EDGE('',*,*,#11680,.T.);
#17128=ORIENTED_EDGE('',*,*,#11677,.T.);
#17129=ORIENTED_EDGE('',*,*,#11674,.T.);
#17130=ORIENTED_EDGE('',*,*,#11671,.T.);
#17131=ORIENTED_EDGE('',*,*,#11668,.T.);
#17132=ORIENTED_EDGE('',*,*,#11665,.T.);
#17133=ORIENTED_EDGE('',*,*,#11662,.T.);
#17134=ORIENTED_EDGE('',*,*,#11659,.T.);
#17135=ORIENTED_EDGE('',*,*,#11656,.T.);
#17136=ORIENTED_EDGE('',*,*,#11653,.T.);
#17137=ORIENTED_EDGE('',*,*,#11650,.T.);
#17138=ORIENTED_EDGE('',*,*,#11643,.T.);
#17139=ORIENTED_EDGE('',*,*,#12501,.T.);
#17140=ORIENTED_EDGE('',*,*,#11640,.F.);
#17141=ORIENTED_EDGE('',*,*,#12500,.T.);
#17142=ORIENTED_EDGE('',*,*,#12183,.F.);
#17143=ORIENTED_EDGE('',*,*,#12086,.F.);
#17144=ORIENTED_EDGE('',*,*,#12280,.F.);
#17145=ORIENTED_EDGE('',*,*,#11892,.F.);
#17146=ORIENTED_EDGE('',*,*,#11795,.F.);
#17147=ORIENTED_EDGE('',*,*,#11601,.F.);
#17148=ORIENTED_EDGE('',*,*,#11989,.F.);
#17149=ORIENTED_EDGE('',*,*,#11698,.F.);
#17150=ORIENTED_EDGE('',*,*,#12503,.F.);
#17151=ORIENTED_EDGE('',*,*,#12504,.T.);
#17152=ORIENTED_EDGE('',*,*,#12505,.F.);
#17153=ORIENTED_EDGE('',*,*,#12504,.F.);
#17154=ORIENTED_EDGE('',*,*,#12506,.F.);
#17155=ORIENTED_EDGE('',*,*,#12507,.T.);
#17156=ORIENTED_EDGE('',*,*,#12508,.F.);
#17157=ORIENTED_EDGE('',*,*,#12507,.F.);
#17158=ORIENTED_EDGE('',*,*,#12509,.F.);
#17159=ORIENTED_EDGE('',*,*,#12510,.T.);
#17160=ORIENTED_EDGE('',*,*,#12511,.F.);
#17161=ORIENTED_EDGE('',*,*,#12510,.F.);
#17162=ORIENTED_EDGE('',*,*,#12512,.F.);
#17163=ORIENTED_EDGE('',*,*,#12513,.T.);
#17164=ORIENTED_EDGE('',*,*,#12514,.F.);
#17165=ORIENTED_EDGE('',*,*,#12513,.F.);
#17166=ORIENTED_EDGE('',*,*,#12515,.F.);
#17167=ORIENTED_EDGE('',*,*,#12516,.T.);
#17168=ORIENTED_EDGE('',*,*,#12517,.T.);
#17169=ORIENTED_EDGE('',*,*,#12516,.F.);
#17170=ORIENTED_EDGE('',*,*,#12517,.F.);
#17171=ORIENTED_EDGE('',*,*,#12518,.F.);
#17172=ORIENTED_EDGE('',*,*,#12519,.F.);
#17173=ORIENTED_EDGE('',*,*,#12520,.T.);
#17174=ORIENTED_EDGE('',*,*,#12386,.T.);
#17175=ORIENTED_EDGE('',*,*,#12388,.T.);
#17176=ORIENTED_EDGE('',*,*,#12521,.T.);
#17177=ORIENTED_EDGE('',*,*,#12408,.T.);
#17178=ORIENTED_EDGE('',*,*,#12410,.T.);
#17179=ORIENTED_EDGE('',*,*,#12522,.T.);
#17180=ORIENTED_EDGE('',*,*,#12430,.T.);
#17181=ORIENTED_EDGE('',*,*,#12432,.T.);
#17182=ORIENTED_EDGE('',*,*,#12523,.T.);
#17183=ORIENTED_EDGE('',*,*,#12524,.F.);
#17184=ORIENTED_EDGE('',*,*,#12523,.F.);
#17185=ORIENTED_EDGE('',*,*,#12431,.T.);
#17186=ORIENTED_EDGE('',*,*,#12522,.F.);
#17187=ORIENTED_EDGE('',*,*,#12409,.T.);
#17188=ORIENTED_EDGE('',*,*,#12521,.F.);
#17189=ORIENTED_EDGE('',*,*,#12387,.T.);
#17190=ORIENTED_EDGE('',*,*,#12520,.F.);
#17191=ORIENTED_EDGE('',*,*,#12375,.T.);
#17192=ORIENTED_EDGE('',*,*,#12376,.T.);
#17193=ORIENTED_EDGE('',*,*,#12381,.T.);
#17194=ORIENTED_EDGE('',*,*,#12382,.T.);
#17195=ORIENTED_EDGE('',*,*,#12393,.T.);
#17196=ORIENTED_EDGE('',*,*,#12397,.T.);
#17197=ORIENTED_EDGE('',*,*,#12398,.T.);
#17198=ORIENTED_EDGE('',*,*,#12403,.T.);
#17199=ORIENTED_EDGE('',*,*,#12404,.T.);
#17200=ORIENTED_EDGE('',*,*,#12415,.T.);
#17201=ORIENTED_EDGE('',*,*,#12419,.T.);
#17202=ORIENTED_EDGE('',*,*,#12420,.T.);
#17203=ORIENTED_EDGE('',*,*,#12425,.T.);
#17204=ORIENTED_EDGE('',*,*,#12426,.T.);
#17205=ORIENTED_EDGE('',*,*,#12437,.T.);
#17206=ORIENTED_EDGE('',*,*,#12525,.F.);
#17207=ORIENTED_EDGE('',*,*,#12526,.T.);
#17208=ORIENTED_EDGE('',*,*,#12383,.T.);
#17209=ORIENTED_EDGE('',*,*,#12527,.T.);
#17210=ORIENTED_EDGE('',*,*,#12405,.T.);
#17211=ORIENTED_EDGE('',*,*,#12528,.T.);
#17212=ORIENTED_EDGE('',*,*,#12427,.T.);
#17213=ORIENTED_EDGE('',*,*,#12529,.T.);
#17214=ORIENTED_EDGE('',*,*,#12530,.F.);
#17215=ORIENTED_EDGE('',*,*,#12529,.F.);
#17216=ORIENTED_EDGE('',*,*,#12433,.T.);
#17217=ORIENTED_EDGE('',*,*,#12428,.T.);
#17218=ORIENTED_EDGE('',*,*,#12528,.F.);
#17219=ORIENTED_EDGE('',*,*,#12411,.T.);
#17220=ORIENTED_EDGE('',*,*,#12406,.T.);
#17221=ORIENTED_EDGE('',*,*,#12527,.F.);
#17222=ORIENTED_EDGE('',*,*,#12389,.T.);
#17223=ORIENTED_EDGE('',*,*,#12384,.T.);
#17224=ORIENTED_EDGE('',*,*,#12526,.F.);
#17225=ORIENTED_EDGE('',*,*,#12373,.T.);
#17226=ORIENTED_EDGE('',*,*,#12377,.T.);
#17227=ORIENTED_EDGE('',*,*,#12378,.T.);
#17228=ORIENTED_EDGE('',*,*,#12379,.T.);
#17229=ORIENTED_EDGE('',*,*,#12390,.T.);
#17230=ORIENTED_EDGE('',*,*,#12394,.T.);
#17231=ORIENTED_EDGE('',*,*,#12391,.T.);
#17232=ORIENTED_EDGE('',*,*,#12395,.T.);
#17233=ORIENTED_EDGE('',*,*,#12399,.T.);
#17234=ORIENTED_EDGE('',*,*,#12400,.T.);
#17235=ORIENTED_EDGE('',*,*,#12401,.T.);
#17236=ORIENTED_EDGE('',*,*,#12412,.T.);
#17237=ORIENTED_EDGE('',*,*,#12416,.T.);
#17238=ORIENTED_EDGE('',*,*,#12413,.T.);
#17239=ORIENTED_EDGE('',*,*,#12417,.T.);
#17240=ORIENTED_EDGE('',*,*,#12421,.T.);
#17241=ORIENTED_EDGE('',*,*,#12422,.T.);
#17242=ORIENTED_EDGE('',*,*,#12423,.T.);
#17243=ORIENTED_EDGE('',*,*,#12434,.T.);
#17244=ORIENTED_EDGE('',*,*,#12438,.T.);
#17245=ORIENTED_EDGE('',*,*,#12435,.T.);
#17246=ORIENTED_EDGE('',*,*,#12525,.T.);
#17247=ORIENTED_EDGE('',*,*,#12454,.T.);
#17248=ORIENTED_EDGE('',*,*,#12227,.T.);
#17249=ORIENTED_EDGE('',*,*,#12451,.T.);
#17250=ORIENTED_EDGE('',*,*,#12274,.T.);
#17251=ORIENTED_EDGE('',*,*,#12470,.T.);
#17252=ORIENTED_EDGE('',*,*,#12033,.T.);
#17253=ORIENTED_EDGE('',*,*,#12467,.T.);
#17254=ORIENTED_EDGE('',*,*,#12080,.T.);
#17255=ORIENTED_EDGE('',*,*,#12486,.T.);
#17256=ORIENTED_EDGE('',*,*,#11839,.T.);
#17257=ORIENTED_EDGE('',*,*,#12483,.T.);
#17258=ORIENTED_EDGE('',*,*,#11886,.T.);
#17259=ORIENTED_EDGE('',*,*,#12502,.T.);
#17260=ORIENTED_EDGE('',*,*,#11645,.T.);
#17261=ORIENTED_EDGE('',*,*,#12499,.T.);
#17262=ORIENTED_EDGE('',*,*,#11692,.T.);
#17263=ORIENTED_EDGE('',*,*,#12519,.T.);
#17264=ORIENTED_EDGE('',*,*,#12494,.T.);
#17265=ORIENTED_EDGE('',*,*,#11742,.T.);
#17266=ORIENTED_EDGE('',*,*,#12491,.T.);
#17267=ORIENTED_EDGE('',*,*,#11789,.T.);
#17268=ORIENTED_EDGE('',*,*,#12478,.T.);
#17269=ORIENTED_EDGE('',*,*,#11936,.T.);
#17270=ORIENTED_EDGE('',*,*,#12475,.T.);
#17271=ORIENTED_EDGE('',*,*,#11983,.T.);
#17272=ORIENTED_EDGE('',*,*,#12462,.T.);
#17273=ORIENTED_EDGE('',*,*,#12130,.T.);
#17274=ORIENTED_EDGE('',*,*,#12459,.T.);
#17275=ORIENTED_EDGE('',*,*,#12177,.T.);
#17276=ORIENTED_EDGE('',*,*,#12446,.T.);
#17277=ORIENTED_EDGE('',*,*,#12324,.T.);
#17278=ORIENTED_EDGE('',*,*,#12443,.T.);
#17279=ORIENTED_EDGE('',*,*,#12371,.T.);
#17280=ORIENTED_EDGE('',*,*,#12531,.T.);
#17281=ORIENTED_EDGE('',*,*,#12530,.T.);
#17282=ORIENTED_EDGE('',*,*,#12512,.T.);
#17283=ORIENTED_EDGE('',*,*,#12509,.T.);
#17284=ORIENTED_EDGE('',*,*,#12506,.T.);
#17285=ORIENTED_EDGE('',*,*,#12503,.T.);
#17286=ORIENTED_EDGE('',*,*,#12518,.T.);
#17287=ORIENTED_EDGE('',*,*,#12532,.T.);
#17288=ORIENTED_EDGE('',*,*,#12533,.T.);
#17289=ORIENTED_EDGE('',*,*,#12532,.F.);
#17290=ORIENTED_EDGE('',*,*,#12531,.F.);
#17291=ORIENTED_EDGE('',*,*,#12534,.T.);
#17292=ORIENTED_EDGE('',*,*,#12535,.T.);
#17293=ORIENTED_EDGE('',*,*,#12534,.F.);
#17294=ORIENTED_EDGE('',*,*,#12524,.T.);
#17295=ORIENTED_EDGE('',*,*,#12515,.T.);
#17296=ORIENTED_EDGE('',*,*,#12535,.F.);
#17297=ORIENTED_EDGE('',*,*,#12533,.F.);
#17298=ORIENTED_EDGE('',*,*,#12514,.T.);
#17299=ORIENTED_EDGE('',*,*,#12511,.T.);
#17300=ORIENTED_EDGE('',*,*,#12508,.T.);
#17301=ORIENTED_EDGE('',*,*,#12505,.T.);
#23078=CYLINDRICAL_SURFACE('',#25393,2.5175);
#23079=CYLINDRICAL_SURFACE('',#25397,2.5175);
#23080=CYLINDRICAL_SURFACE('',#25398,2.5175);
#23081=CYLINDRICAL_SURFACE('',#25399,2.5175);
#23082=CYLINDRICAL_SURFACE('',#25400,2.5175);
#23083=CYLINDRICAL_SURFACE('',#25401,2.5175);
#23084=CYLINDRICAL_SURFACE('',#25402,2.5175);
#23085=CYLINDRICAL_SURFACE('',#25403,2.5175);
#23086=CYLINDRICAL_SURFACE('',#25404,2.5175);
#23087=CYLINDRICAL_SURFACE('',#25405,2.5175);
#23088=CYLINDRICAL_SURFACE('',#25406,2.5175);
#23089=CYLINDRICAL_SURFACE('',#25407,2.5175);
#23090=CYLINDRICAL_SURFACE('',#25408,2.5175);
#23091=CYLINDRICAL_SURFACE('',#25409,2.5175);
#23092=CYLINDRICAL_SURFACE('',#25410,2.5175);
#23093=CYLINDRICAL_SURFACE('',#25412,3.0735);
#23094=CYLINDRICAL_SURFACE('',#25414,3.0735);
#23095=CYLINDRICAL_SURFACE('',#25415,3.0735);
#23096=CYLINDRICAL_SURFACE('',#25416,3.0735);
#23097=CYLINDRICAL_SURFACE('',#25417,3.0735);
#23098=CYLINDRICAL_SURFACE('',#25418,3.0735);
#23099=CYLINDRICAL_SURFACE('',#25419,3.0735);
#23100=CYLINDRICAL_SURFACE('',#25420,3.0735);
#23101=CYLINDRICAL_SURFACE('',#25421,3.0735);
#23102=CYLINDRICAL_SURFACE('',#25422,3.0735);
#23103=CYLINDRICAL_SURFACE('',#25423,3.0735);
#23104=CYLINDRICAL_SURFACE('',#25424,3.0735);
#23105=CYLINDRICAL_SURFACE('',#25425,3.0735);
#23106=CYLINDRICAL_SURFACE('',#25426,3.0735);
#23107=CYLINDRICAL_SURFACE('',#25427,3.0735);
#23108=CYLINDRICAL_SURFACE('',#25429,2.5175);
#23109=CYLINDRICAL_SURFACE('',#25433,2.5175);
#23110=CYLINDRICAL_SURFACE('',#25434,2.5175);
#23111=CYLINDRICAL_SURFACE('',#25435,2.5175);
#23112=CYLINDRICAL_SURFACE('',#25436,2.5175);
#23113=CYLINDRICAL_SURFACE('',#25437,2.5175);
#23114=CYLINDRICAL_SURFACE('',#25438,2.5175);
#23115=CYLINDRICAL_SURFACE('',#25439,2.5175);
#23116=CYLINDRICAL_SURFACE('',#25440,2.5175);
#23117=CYLINDRICAL_SURFACE('',#25441,2.5175);
#23118=CYLINDRICAL_SURFACE('',#25442,2.5175);
#23119=CYLINDRICAL_SURFACE('',#25443,2.5175);
#23120=CYLINDRICAL_SURFACE('',#25444,2.5175);
#23121=CYLINDRICAL_SURFACE('',#25445,2.5175);
#23122=CYLINDRICAL_SURFACE('',#25446,2.5175);
#23123=CYLINDRICAL_SURFACE('',#25448,3.0735);
#23124=CYLINDRICAL_SURFACE('',#25450,3.0735);
#23125=CYLINDRICAL_SURFACE('',#25451,3.0735);
#23126=CYLINDRICAL_SURFACE('',#25452,3.0735);
#23127=CYLINDRICAL_SURFACE('',#25453,3.0735);
#23128=CYLINDRICAL_SURFACE('',#25454,3.0735);
#23129=CYLINDRICAL_SURFACE('',#25455,3.0735);
#23130=CYLINDRICAL_SURFACE('',#25456,3.0735);
#23131=CYLINDRICAL_SURFACE('',#25457,3.0735);
#23132=CYLINDRICAL_SURFACE('',#25458,3.0735);
#23133=CYLINDRICAL_SURFACE('',#25459,3.0735);
#23134=CYLINDRICAL_SURFACE('',#25460,3.0735);
#23135=CYLINDRICAL_SURFACE('',#25461,3.0735);
#23136=CYLINDRICAL_SURFACE('',#25462,3.0735);
#23137=CYLINDRICAL_SURFACE('',#25463,3.0735);
#23138=CYLINDRICAL_SURFACE('',#25465,2.5175);
#23139=CYLINDRICAL_SURFACE('',#25469,2.5175);
#23140=CYLINDRICAL_SURFACE('',#25470,2.5175);
#23141=CYLINDRICAL_SURFACE('',#25471,2.5175);
#23142=CYLINDRICAL_SURFACE('',#25472,2.5175);
#23143=CYLINDRICAL_SURFACE('',#25473,2.5175);
#23144=CYLINDRICAL_SURFACE('',#25474,2.5175);
#23145=CYLINDRICAL_SURFACE('',#25475,2.5175);
#23146=CYLINDRICAL_SURFACE('',#25476,2.5175);
#23147=CYLINDRICAL_SURFACE('',#25477,2.5175);
#23148=CYLINDRICAL_SURFACE('',#25478,2.5175);
#23149=CYLINDRICAL_SURFACE('',#25479,2.5175);
#23150=CYLINDRICAL_SURFACE('',#25480,2.5175);
#23151=CYLINDRICAL_SURFACE('',#25481,2.5175);
#23152=CYLINDRICAL_SURFACE('',#25482,2.5175);
#23153=CYLINDRICAL_SURFACE('',#25484,3.0735);
#23154=CYLINDRICAL_SURFACE('',#25486,3.0735);
#23155=CYLINDRICAL_SURFACE('',#25487,3.0735);
#23156=CYLINDRICAL_SURFACE('',#25488,3.0735);
#23157=CYLINDRICAL_SURFACE('',#25489,3.0735);
#23158=CYLINDRICAL_SURFACE('',#25490,3.0735);
#23159=CYLINDRICAL_SURFACE('',#25491,3.0735);
#23160=CYLINDRICAL_SURFACE('',#25492,3.0735);
#23161=CYLINDRICAL_SURFACE('',#25493,3.0735);
#23162=CYLINDRICAL_SURFACE('',#25494,3.0735);
#23163=CYLINDRICAL_SURFACE('',#25495,3.0735);
#23164=CYLINDRICAL_SURFACE('',#25496,3.0735);
#23165=CYLINDRICAL_SURFACE('',#25497,3.0735);
#23166=CYLINDRICAL_SURFACE('',#25498,3.0735);
#23167=CYLINDRICAL_SURFACE('',#25499,3.0735);
#23168=CYLINDRICAL_SURFACE('',#25501,2.5175);
#23169=CYLINDRICAL_SURFACE('',#25505,2.5175);
#23170=CYLINDRICAL_SURFACE('',#25506,2.5175);
#23171=CYLINDRICAL_SURFACE('',#25507,2.5175);
#23172=CYLINDRICAL_SURFACE('',#25508,2.5175);
#23173=CYLINDRICAL_SURFACE('',#25509,2.5175);
#23174=CYLINDRICAL_SURFACE('',#25510,2.5175);
#23175=CYLINDRICAL_SURFACE('',#25511,2.5175);
#23176=CYLINDRICAL_SURFACE('',#25512,2.5175);
#23177=CYLINDRICAL_SURFACE('',#25513,2.5175);
#23178=CYLINDRICAL_SURFACE('',#25514,2.5175);
#23179=CYLINDRICAL_SURFACE('',#25515,2.5175);
#23180=CYLINDRICAL_SURFACE('',#25516,2.5175);
#23181=CYLINDRICAL_SURFACE('',#25517,2.5175);
#23182=CYLINDRICAL_SURFACE('',#25518,2.5175);
#23183=CYLINDRICAL_SURFACE('',#25520,3.0735);
#23184=CYLINDRICAL_SURFACE('',#25522,3.0735);
#23185=CYLINDRICAL_SURFACE('',#25523,3.0735);
#23186=CYLINDRICAL_SURFACE('',#25524,3.0735);
#23187=CYLINDRICAL_SURFACE('',#25525,3.0735);
#23188=CYLINDRICAL_SURFACE('',#25526,3.0735);
#23189=CYLINDRICAL_SURFACE('',#25527,3.0735);
#23190=CYLINDRICAL_SURFACE('',#25528,3.0735);
#23191=CYLINDRICAL_SURFACE('',#25529,3.0735);
#23192=CYLINDRICAL_SURFACE('',#25530,3.0735);
#23193=CYLINDRICAL_SURFACE('',#25531,3.0735);
#23194=CYLINDRICAL_SURFACE('',#25532,3.0735);
#23195=CYLINDRICAL_SURFACE('',#25533,3.0735);
#23196=CYLINDRICAL_SURFACE('',#25534,3.0735);
#23197=CYLINDRICAL_SURFACE('',#25535,3.0735);
#23198=CYLINDRICAL_SURFACE('',#25537,2.5175);
#23199=CYLINDRICAL_SURFACE('',#25541,2.5175);
#23200=CYLINDRICAL_SURFACE('',#25542,2.5175);
#23201=CYLINDRICAL_SURFACE('',#25543,2.5175);
#23202=CYLINDRICAL_SURFACE('',#25544,2.5175);
#23203=CYLINDRICAL_SURFACE('',#25545,2.5175);
#23204=CYLINDRICAL_SURFACE('',#25546,2.5175);
#23205=CYLINDRICAL_SURFACE('',#25547,2.5175);
#23206=CYLINDRICAL_SURFACE('',#25548,2.5175);
#23207=CYLINDRICAL_SURFACE('',#25549,2.5175);
#23208=CYLINDRICAL_SURFACE('',#25550,2.5175);
#23209=CYLINDRICAL_SURFACE('',#25551,2.5175);
#23210=CYLINDRICAL_SURFACE('',#25552,2.5175);
#23211=CYLINDRICAL_SURFACE('',#25553,2.5175);
#23212=CYLINDRICAL_SURFACE('',#25554,2.5175);
#23213=CYLINDRICAL_SURFACE('',#25556,3.0735);
#23214=CYLINDRICAL_SURFACE('',#25558,3.0735);
#23215=CYLINDRICAL_SURFACE('',#25559,3.0735);
#23216=CYLINDRICAL_SURFACE('',#25560,3.0735);
#23217=CYLINDRICAL_SURFACE('',#25561,3.0735);
#23218=CYLINDRICAL_SURFACE('',#25562,3.0735);
#23219=CYLINDRICAL_SURFACE('',#25563,3.0735);
#23220=CYLINDRICAL_SURFACE('',#25564,3.0735);
#23221=CYLINDRICAL_SURFACE('',#25565,3.0735);
#23222=CYLINDRICAL_SURFACE('',#25566,3.0735);
#23223=CYLINDRICAL_SURFACE('',#25567,3.0735);
#23224=CYLINDRICAL_SURFACE('',#25568,3.0735);
#23225=CYLINDRICAL_SURFACE('',#25569,3.0735);
#23226=CYLINDRICAL_SURFACE('',#25570,3.0735);
#23227=CYLINDRICAL_SURFACE('',#25571,3.0735);
#23228=CYLINDRICAL_SURFACE('',#25573,2.5175);
#23229=CYLINDRICAL_SURFACE('',#25577,2.5175);
#23230=CYLINDRICAL_SURFACE('',#25578,2.5175);
#23231=CYLINDRICAL_SURFACE('',#25579,2.5175);
#23232=CYLINDRICAL_SURFACE('',#25580,2.5175);
#23233=CYLINDRICAL_SURFACE('',#25581,2.5175);
#23234=CYLINDRICAL_SURFACE('',#25582,2.5175);
#23235=CYLINDRICAL_SURFACE('',#25583,2.5175);
#23236=CYLINDRICAL_SURFACE('',#25584,2.5175);
#23237=CYLINDRICAL_SURFACE('',#25585,2.5175);
#23238=CYLINDRICAL_SURFACE('',#25586,2.5175);
#23239=CYLINDRICAL_SURFACE('',#25587,2.5175);
#23240=CYLINDRICAL_SURFACE('',#25588,2.5175);
#23241=CYLINDRICAL_SURFACE('',#25589,2.5175);
#23242=CYLINDRICAL_SURFACE('',#25590,2.5175);
#23243=CYLINDRICAL_SURFACE('',#25592,3.0735);
#23244=CYLINDRICAL_SURFACE('',#25594,3.0735);
#23245=CYLINDRICAL_SURFACE('',#25595,3.0735);
#23246=CYLINDRICAL_SURFACE('',#25596,3.0735);
#23247=CYLINDRICAL_SURFACE('',#25597,3.0735);
#23248=CYLINDRICAL_SURFACE('',#25598,3.0735);
#23249=CYLINDRICAL_SURFACE('',#25599,3.0735);
#23250=CYLINDRICAL_SURFACE('',#25600,3.0735);
#23251=CYLINDRICAL_SURFACE('',#25601,3.0735);
#23252=CYLINDRICAL_SURFACE('',#25602,3.0735);
#23253=CYLINDRICAL_SURFACE('',#25603,3.0735);
#23254=CYLINDRICAL_SURFACE('',#25604,3.0735);
#23255=CYLINDRICAL_SURFACE('',#25605,3.0735);
#23256=CYLINDRICAL_SURFACE('',#25606,3.0735);
#23257=CYLINDRICAL_SURFACE('',#25607,3.0735);
#23258=CYLINDRICAL_SURFACE('',#25609,2.5175);
#23259=CYLINDRICAL_SURFACE('',#25613,2.5175);
#23260=CYLINDRICAL_SURFACE('',#25614,2.5175);
#23261=CYLINDRICAL_SURFACE('',#25615,2.5175);
#23262=CYLINDRICAL_SURFACE('',#25616,2.5175);
#23263=CYLINDRICAL_SURFACE('',#25617,2.5175);
#23264=CYLINDRICAL_SURFACE('',#25618,2.5175);
#23265=CYLINDRICAL_SURFACE('',#25619,2.5175);
#23266=CYLINDRICAL_SURFACE('',#25620,2.5175);
#23267=CYLINDRICAL_SURFACE('',#25621,2.5175);
#23268=CYLINDRICAL_SURFACE('',#25622,2.5175);
#23269=CYLINDRICAL_SURFACE('',#25623,2.5175);
#23270=CYLINDRICAL_SURFACE('',#25624,2.5175);
#23271=CYLINDRICAL_SURFACE('',#25625,2.5175);
#23272=CYLINDRICAL_SURFACE('',#25626,2.5175);
#23273=CYLINDRICAL_SURFACE('',#25628,3.0735);
#23274=CYLINDRICAL_SURFACE('',#25630,3.0735);
#23275=CYLINDRICAL_SURFACE('',#25631,3.0735);
#23276=CYLINDRICAL_SURFACE('',#25632,3.0735);
#23277=CYLINDRICAL_SURFACE('',#25633,3.0735);
#23278=CYLINDRICAL_SURFACE('',#25634,3.0735);
#23279=CYLINDRICAL_SURFACE('',#25635,3.0735);
#23280=CYLINDRICAL_SURFACE('',#25636,3.0735);
#23281=CYLINDRICAL_SURFACE('',#25637,3.0735);
#23282=CYLINDRICAL_SURFACE('',#25638,3.0735);
#23283=CYLINDRICAL_SURFACE('',#25639,3.0735);
#23284=CYLINDRICAL_SURFACE('',#25640,3.0735);
#23285=CYLINDRICAL_SURFACE('',#25641,3.0735);
#23286=CYLINDRICAL_SURFACE('',#25642,3.0735);
#23287=CYLINDRICAL_SURFACE('',#25643,3.0735);
#23288=CYLINDRICAL_SURFACE('',#25645,2.5175);
#23289=CYLINDRICAL_SURFACE('',#25649,2.5175);
#23290=CYLINDRICAL_SURFACE('',#25650,2.5175);
#23291=CYLINDRICAL_SURFACE('',#25651,2.5175);
#23292=CYLINDRICAL_SURFACE('',#25652,2.5175);
#23293=CYLINDRICAL_SURFACE('',#25653,2.5175);
#23294=CYLINDRICAL_SURFACE('',#25654,2.5175);
#23295=CYLINDRICAL_SURFACE('',#25655,2.5175);
#23296=CYLINDRICAL_SURFACE('',#25656,2.5175);
#23297=CYLINDRICAL_SURFACE('',#25657,2.5175);
#23298=CYLINDRICAL_SURFACE('',#25658,2.5175);
#23299=CYLINDRICAL_SURFACE('',#25659,2.5175);
#23300=CYLINDRICAL_SURFACE('',#25660,2.5175);
#23301=CYLINDRICAL_SURFACE('',#25661,2.5175);
#23302=CYLINDRICAL_SURFACE('',#25662,2.5175);
#23303=CYLINDRICAL_SURFACE('',#25664,3.0735);
#23304=CYLINDRICAL_SURFACE('',#25666,3.0735);
#23305=CYLINDRICAL_SURFACE('',#25667,3.0735);
#23306=CYLINDRICAL_SURFACE('',#25668,3.0735);
#23307=CYLINDRICAL_SURFACE('',#25669,3.0735);
#23308=CYLINDRICAL_SURFACE('',#25670,3.0735);
#23309=CYLINDRICAL_SURFACE('',#25671,3.0735);
#23310=CYLINDRICAL_SURFACE('',#25672,3.0735);
#23311=CYLINDRICAL_SURFACE('',#25673,3.0735);
#23312=CYLINDRICAL_SURFACE('',#25674,3.0735);
#23313=CYLINDRICAL_SURFACE('',#25675,3.0735);
#23314=CYLINDRICAL_SURFACE('',#25676,3.0735);
#23315=CYLINDRICAL_SURFACE('',#25677,3.0735);
#23316=CYLINDRICAL_SURFACE('',#25678,3.0735);
#23317=CYLINDRICAL_SURFACE('',#25679,3.0735);
#23318=CYLINDRICAL_SURFACE('',#25681,2.);
#23319=CYLINDRICAL_SURFACE('',#25682,2.);
#23320=CYLINDRICAL_SURFACE('',#25683,2.);
#23321=CYLINDRICAL_SURFACE('',#25684,2.);
#23322=CYLINDRICAL_SURFACE('',#25685,2.);
#23323=CYLINDRICAL_SURFACE('',#25686,2.);
#23324=CYLINDRICAL_SURFACE('',#25687,2.);
#23325=CYLINDRICAL_SURFACE('',#25688,2.);
#23326=CYLINDRICAL_SURFACE('',#25689,2.);
#23327=CYLINDRICAL_SURFACE('',#25690,2.);
#23328=CYLINDRICAL_SURFACE('',#25691,2.);
#23329=CYLINDRICAL_SURFACE('',#25692,2.);
#23330=CYLINDRICAL_SURFACE('',#25694,3.0735);
#23331=CYLINDRICAL_SURFACE('',#25695,2.5175);
#23332=CYLINDRICAL_SURFACE('',#25697,3.0735);
#23333=CYLINDRICAL_SURFACE('',#25698,2.5175);
#23334=CYLINDRICAL_SURFACE('',#25700,3.0735);
#23335=CYLINDRICAL_SURFACE('',#25701,2.5175);
#23336=CYLINDRICAL_SURFACE('',#25703,3.0735);
#23337=CYLINDRICAL_SURFACE('',#25704,2.5175);
#23338=CYLINDRICAL_SURFACE('',#25706,3.0735);
#23339=CYLINDRICAL_SURFACE('',#25707,2.5175);
#23340=CYLINDRICAL_SURFACE('',#25709,3.0735);
#23341=CYLINDRICAL_SURFACE('',#25710,2.5175);
#23342=CYLINDRICAL_SURFACE('',#25712,3.0735);
#23343=CYLINDRICAL_SURFACE('',#25713,2.5175);
#23344=CYLINDRICAL_SURFACE('',#25715,3.0735);
#23345=CYLINDRICAL_SURFACE('',#25716,2.5175);
#23346=CYLINDRICAL_SURFACE('',#25725,5.5);
#23347=CYLINDRICAL_SURFACE('',#25728,5.5);
#23348=CYLINDRICAL_SURFACE('',#25731,5.5);
#23349=CYLINDRICAL_SURFACE('',#25734,5.5);
#23350=CYLINDRICAL_SURFACE('',#25737,18.);
#23351=CYLINDRICAL_SURFACE('',#25742,90.);
#23352=CYLINDRICAL_SURFACE('',#25745,100.);
#23353=CYLINDRICAL_SURFACE('',#25751,17.);
#23354=CYLINDRICAL_SURFACE('',#25753,140.);
#23804=ADVANCED_FACE('',(#1698),#23078,.F.);
#23805=ADVANCED_FACE('',(#1699),#23079,.F.);
#23806=ADVANCED_FACE('',(#1700),#23080,.F.);
#23807=ADVANCED_FACE('',(#1701),#23081,.F.);
#23808=ADVANCED_FACE('',(#1702),#23082,.F.);
#23809=ADVANCED_FACE('',(#1703),#23083,.F.);
#23810=ADVANCED_FACE('',(#1704),#23084,.F.);
#23811=ADVANCED_FACE('',(#1705),#23085,.F.);
#23812=ADVANCED_FACE('',(#1706),#23086,.F.);
#23813=ADVANCED_FACE('',(#1707),#23087,.F.);
#23814=ADVANCED_FACE('',(#1708),#23088,.F.);
#23815=ADVANCED_FACE('',(#1709),#23089,.F.);
#23816=ADVANCED_FACE('',(#1710),#23090,.F.);
#23817=ADVANCED_FACE('',(#1711),#23091,.F.);
#23818=ADVANCED_FACE('',(#1712),#23092,.F.);
#23819=ADVANCED_FACE('',(#1713),#23093,.F.);
#23820=ADVANCED_FACE('',(#1714),#23094,.F.);
#23821=ADVANCED_FACE('',(#1715),#23095,.F.);
#23822=ADVANCED_FACE('',(#1716),#23096,.F.);
#23823=ADVANCED_FACE('',(#1717),#23097,.F.);
#23824=ADVANCED_FACE('',(#1718),#23098,.F.);
#23825=ADVANCED_FACE('',(#1719),#23099,.F.);
#23826=ADVANCED_FACE('',(#1720),#23100,.F.);
#23827=ADVANCED_FACE('',(#1721),#23101,.F.);
#23828=ADVANCED_FACE('',(#1722),#23102,.F.);
#23829=ADVANCED_FACE('',(#1723),#23103,.F.);
#23830=ADVANCED_FACE('',(#1724),#23104,.F.);
#23831=ADVANCED_FACE('',(#1725),#23105,.F.);
#23832=ADVANCED_FACE('',(#1726),#23106,.F.);
#23833=ADVANCED_FACE('',(#1727),#23107,.F.);
#23834=ADVANCED_FACE('',(#1728),#23108,.F.);
#23835=ADVANCED_FACE('',(#1729),#23109,.F.);
#23836=ADVANCED_FACE('',(#1730),#23110,.F.);
#23837=ADVANCED_FACE('',(#1731),#23111,.F.);
#23838=ADVANCED_FACE('',(#1732),#23112,.F.);
#23839=ADVANCED_FACE('',(#1733),#23113,.F.);
#23840=ADVANCED_FACE('',(#1734),#23114,.F.);
#23841=ADVANCED_FACE('',(#1735),#23115,.F.);
#23842=ADVANCED_FACE('',(#1736),#23116,.F.);
#23843=ADVANCED_FACE('',(#1737),#23117,.F.);
#23844=ADVANCED_FACE('',(#1738),#23118,.F.);
#23845=ADVANCED_FACE('',(#1739),#23119,.F.);
#23846=ADVANCED_FACE('',(#1740),#23120,.F.);
#23847=ADVANCED_FACE('',(#1741),#23121,.F.);
#23848=ADVANCED_FACE('',(#1742),#23122,.F.);
#23849=ADVANCED_FACE('',(#1743),#23123,.F.);
#23850=ADVANCED_FACE('',(#1744),#23124,.F.);
#23851=ADVANCED_FACE('',(#1745),#23125,.F.);
#23852=ADVANCED_FACE('',(#1746),#23126,.F.);
#23853=ADVANCED_FACE('',(#1747),#23127,.F.);
#23854=ADVANCED_FACE('',(#1748),#23128,.F.);
#23855=ADVANCED_FACE('',(#1749),#23129,.F.);
#23856=ADVANCED_FACE('',(#1750),#23130,.F.);
#23857=ADVANCED_FACE('',(#1751),#23131,.F.);
#23858=ADVANCED_FACE('',(#1752),#23132,.F.);
#23859=ADVANCED_FACE('',(#1753),#23133,.F.);
#23860=ADVANCED_FACE('',(#1754),#23134,.F.);
#23861=ADVANCED_FACE('',(#1755),#23135,.F.);
#23862=ADVANCED_FACE('',(#1756),#23136,.F.);
#23863=ADVANCED_FACE('',(#1757),#23137,.F.);
#23864=ADVANCED_FACE('',(#1758),#23138,.F.);
#23865=ADVANCED_FACE('',(#1759),#23139,.F.);
#23866=ADVANCED_FACE('',(#1760),#23140,.F.);
#23867=ADVANCED_FACE('',(#1761),#23141,.F.);
#23868=ADVANCED_FACE('',(#1762),#23142,.F.);
#23869=ADVANCED_FACE('',(#1763),#23143,.F.);
#23870=ADVANCED_FACE('',(#1764),#23144,.F.);
#23871=ADVANCED_FACE('',(#1765),#23145,.F.);
#23872=ADVANCED_FACE('',(#1766),#23146,.F.);
#23873=ADVANCED_FACE('',(#1767),#23147,.F.);
#23874=ADVANCED_FACE('',(#1768),#23148,.F.);
#23875=ADVANCED_FACE('',(#1769),#23149,.F.);
#23876=ADVANCED_FACE('',(#1770),#23150,.F.);
#23877=ADVANCED_FACE('',(#1771),#23151,.F.);
#23878=ADVANCED_FACE('',(#1772),#23152,.F.);
#23879=ADVANCED_FACE('',(#1773),#23153,.F.);
#23880=ADVANCED_FACE('',(#1774),#23154,.F.);
#23881=ADVANCED_FACE('',(#1775),#23155,.F.);
#23882=ADVANCED_FACE('',(#1776),#23156,.F.);
#23883=ADVANCED_FACE('',(#1777),#23157,.F.);
#23884=ADVANCED_FACE('',(#1778),#23158,.F.);
#23885=ADVANCED_FACE('',(#1779),#23159,.F.);
#23886=ADVANCED_FACE('',(#1780),#23160,.F.);
#23887=ADVANCED_FACE('',(#1781),#23161,.F.);
#23888=ADVANCED_FACE('',(#1782),#23162,.F.);
#23889=ADVANCED_FACE('',(#1783),#23163,.F.);
#23890=ADVANCED_FACE('',(#1784),#23164,.F.);
#23891=ADVANCED_FACE('',(#1785),#23165,.F.);
#23892=ADVANCED_FACE('',(#1786),#23166,.F.);
#23893=ADVANCED_FACE('',(#1787),#23167,.F.);
#23894=ADVANCED_FACE('',(#1788),#23168,.F.);
#23895=ADVANCED_FACE('',(#1789),#23169,.F.);
#23896=ADVANCED_FACE('',(#1790),#23170,.F.);
#23897=ADVANCED_FACE('',(#1791),#23171,.F.);
#23898=ADVANCED_FACE('',(#1792),#23172,.F.);
#23899=ADVANCED_FACE('',(#1793),#23173,.F.);
#23900=ADVANCED_FACE('',(#1794),#23174,.F.);
#23901=ADVANCED_FACE('',(#1795),#23175,.F.);
#23902=ADVANCED_FACE('',(#1796),#23176,.F.);
#23903=ADVANCED_FACE('',(#1797),#23177,.F.);
#23904=ADVANCED_FACE('',(#1798),#23178,.F.);
#23905=ADVANCED_FACE('',(#1799),#23179,.F.);
#23906=ADVANCED_FACE('',(#1800),#23180,.F.);
#23907=ADVANCED_FACE('',(#1801),#23181,.F.);
#23908=ADVANCED_FACE('',(#1802),#23182,.F.);
#23909=ADVANCED_FACE('',(#1803),#23183,.F.);
#23910=ADVANCED_FACE('',(#1804),#23184,.F.);
#23911=ADVANCED_FACE('',(#1805),#23185,.F.);
#23912=ADVANCED_FACE('',(#1806),#23186,.F.);
#23913=ADVANCED_FACE('',(#1807),#23187,.F.);
#23914=ADVANCED_FACE('',(#1808),#23188,.F.);
#23915=ADVANCED_FACE('',(#1809),#23189,.F.);
#23916=ADVANCED_FACE('',(#1810),#23190,.F.);
#23917=ADVANCED_FACE('',(#1811),#23191,.F.);
#23918=ADVANCED_FACE('',(#1812),#23192,.F.);
#23919=ADVANCED_FACE('',(#1813),#23193,.F.);
#23920=ADVANCED_FACE('',(#1814),#23194,.F.);
#23921=ADVANCED_FACE('',(#1815),#23195,.F.);
#23922=ADVANCED_FACE('',(#1816),#23196,.F.);
#23923=ADVANCED_FACE('',(#1817),#23197,.F.);
#23924=ADVANCED_FACE('',(#1818),#23198,.F.);
#23925=ADVANCED_FACE('',(#1819),#23199,.F.);
#23926=ADVANCED_FACE('',(#1820),#23200,.F.);
#23927=ADVANCED_FACE('',(#1821),#23201,.F.);
#23928=ADVANCED_FACE('',(#1822),#23202,.F.);
#23929=ADVANCED_FACE('',(#1823),#23203,.F.);
#23930=ADVANCED_FACE('',(#1824),#23204,.F.);
#23931=ADVANCED_FACE('',(#1825),#23205,.F.);
#23932=ADVANCED_FACE('',(#1826),#23206,.F.);
#23933=ADVANCED_FACE('',(#1827),#23207,.F.);
#23934=ADVANCED_FACE('',(#1828),#23208,.F.);
#23935=ADVANCED_FACE('',(#1829),#23209,.F.);
#23936=ADVANCED_FACE('',(#1830),#23210,.F.);
#23937=ADVANCED_FACE('',(#1831),#23211,.F.);
#23938=ADVANCED_FACE('',(#1832),#23212,.F.);
#23939=ADVANCED_FACE('',(#1833),#23213,.F.);
#23940=ADVANCED_FACE('',(#1834),#23214,.F.);
#23941=ADVANCED_FACE('',(#1835),#23215,.F.);
#23942=ADVANCED_FACE('',(#1836),#23216,.F.);
#23943=ADVANCED_FACE('',(#1837),#23217,.F.);
#23944=ADVANCED_FACE('',(#1838),#23218,.F.);
#23945=ADVANCED_FACE('',(#1839),#23219,.F.);
#23946=ADVANCED_FACE('',(#1840),#23220,.F.);
#23947=ADVANCED_FACE('',(#1841),#23221,.F.);
#23948=ADVANCED_FACE('',(#1842),#23222,.F.);
#23949=ADVANCED_FACE('',(#1843),#23223,.F.);
#23950=ADVANCED_FACE('',(#1844),#23224,.F.);
#23951=ADVANCED_FACE('',(#1845),#23225,.F.);
#23952=ADVANCED_FACE('',(#1846),#23226,.F.);
#23953=ADVANCED_FACE('',(#1847),#23227,.F.);
#23954=ADVANCED_FACE('',(#1848),#23228,.F.);
#23955=ADVANCED_FACE('',(#1849),#23229,.F.);
#23956=ADVANCED_FACE('',(#1850),#23230,.F.);
#23957=ADVANCED_FACE('',(#1851),#23231,.F.);
#23958=ADVANCED_FACE('',(#1852),#23232,.F.);
#23959=ADVANCED_FACE('',(#1853),#23233,.F.);
#23960=ADVANCED_FACE('',(#1854),#23234,.F.);
#23961=ADVANCED_FACE('',(#1855),#23235,.F.);
#23962=ADVANCED_FACE('',(#1856),#23236,.F.);
#23963=ADVANCED_FACE('',(#1857),#23237,.F.);
#23964=ADVANCED_FACE('',(#1858),#23238,.F.);
#23965=ADVANCED_FACE('',(#1859),#23239,.F.);
#23966=ADVANCED_FACE('',(#1860),#23240,.F.);
#23967=ADVANCED_FACE('',(#1861),#23241,.F.);
#23968=ADVANCED_FACE('',(#1862),#23242,.F.);
#23969=ADVANCED_FACE('',(#1863),#23243,.F.);
#23970=ADVANCED_FACE('',(#1864),#23244,.F.);
#23971=ADVANCED_FACE('',(#1865),#23245,.F.);
#23972=ADVANCED_FACE('',(#1866),#23246,.F.);
#23973=ADVANCED_FACE('',(#1867),#23247,.F.);
#23974=ADVANCED_FACE('',(#1868),#23248,.F.);
#23975=ADVANCED_FACE('',(#1869),#23249,.F.);
#23976=ADVANCED_FACE('',(#1870),#23250,.F.);
#23977=ADVANCED_FACE('',(#1871),#23251,.F.);
#23978=ADVANCED_FACE('',(#1872),#23252,.F.);
#23979=ADVANCED_FACE('',(#1873),#23253,.F.);
#23980=ADVANCED_FACE('',(#1874),#23254,.F.);
#23981=ADVANCED_FACE('',(#1875),#23255,.F.);
#23982=ADVANCED_FACE('',(#1876),#23256,.F.);
#23983=ADVANCED_FACE('',(#1877),#23257,.F.);
#23984=ADVANCED_FACE('',(#1878),#23258,.F.);
#23985=ADVANCED_FACE('',(#1879),#23259,.F.);
#23986=ADVANCED_FACE('',(#1880),#23260,.F.);
#23987=ADVANCED_FACE('',(#1881),#23261,.F.);
#23988=ADVANCED_FACE('',(#1882),#23262,.F.);
#23989=ADVANCED_FACE('',(#1883),#23263,.F.);
#23990=ADVANCED_FACE('',(#1884),#23264,.F.);
#23991=ADVANCED_FACE('',(#1885),#23265,.F.);
#23992=ADVANCED_FACE('',(#1886),#23266,.F.);
#23993=ADVANCED_FACE('',(#1887),#23267,.F.);
#23994=ADVANCED_FACE('',(#1888),#23268,.F.);
#23995=ADVANCED_FACE('',(#1889),#23269,.F.);
#23996=ADVANCED_FACE('',(#1890),#23270,.F.);
#23997=ADVANCED_FACE('',(#1891),#23271,.F.);
#23998=ADVANCED_FACE('',(#1892),#23272,.F.);
#23999=ADVANCED_FACE('',(#1893),#23273,.F.);
#24000=ADVANCED_FACE('',(#1894),#23274,.F.);
#24001=ADVANCED_FACE('',(#1895),#23275,.F.);
#24002=ADVANCED_FACE('',(#1896),#23276,.F.);
#24003=ADVANCED_FACE('',(#1897),#23277,.F.);
#24004=ADVANCED_FACE('',(#1898),#23278,.F.);
#24005=ADVANCED_FACE('',(#1899),#23279,.F.);
#24006=ADVANCED_FACE('',(#1900),#23280,.F.);
#24007=ADVANCED_FACE('',(#1901),#23281,.F.);
#24008=ADVANCED_FACE('',(#1902),#23282,.F.);
#24009=ADVANCED_FACE('',(#1903),#23283,.F.);
#24010=ADVANCED_FACE('',(#1904),#23284,.F.);
#24011=ADVANCED_FACE('',(#1905),#23285,.F.);
#24012=ADVANCED_FACE('',(#1906),#23286,.F.);
#24013=ADVANCED_FACE('',(#1907),#23287,.F.);
#24014=ADVANCED_FACE('',(#1908),#23288,.F.);
#24015=ADVANCED_FACE('',(#1909),#23289,.F.);
#24016=ADVANCED_FACE('',(#1910),#23290,.F.);
#24017=ADVANCED_FACE('',(#1911),#23291,.F.);
#24018=ADVANCED_FACE('',(#1912),#23292,.F.);
#24019=ADVANCED_FACE('',(#1913),#23293,.F.);
#24020=ADVANCED_FACE('',(#1914),#23294,.F.);
#24021=ADVANCED_FACE('',(#1915),#23295,.F.);
#24022=ADVANCED_FACE('',(#1916),#23296,.F.);
#24023=ADVANCED_FACE('',(#1917),#23297,.F.);
#24024=ADVANCED_FACE('',(#1918),#23298,.F.);
#24025=ADVANCED_FACE('',(#1919),#23299,.F.);
#24026=ADVANCED_FACE('',(#1920),#23300,.F.);
#24027=ADVANCED_FACE('',(#1921),#23301,.F.);
#24028=ADVANCED_FACE('',(#1922),#23302,.F.);
#24029=ADVANCED_FACE('',(#1923),#23303,.F.);
#24030=ADVANCED_FACE('',(#1924),#23304,.F.);
#24031=ADVANCED_FACE('',(#1925),#23305,.F.);
#24032=ADVANCED_FACE('',(#1926),#23306,.F.);
#24033=ADVANCED_FACE('',(#1927),#23307,.F.);
#24034=ADVANCED_FACE('',(#1928),#23308,.F.);
#24035=ADVANCED_FACE('',(#1929),#23309,.F.);
#24036=ADVANCED_FACE('',(#1930),#23310,.F.);
#24037=ADVANCED_FACE('',(#1931),#23311,.F.);
#24038=ADVANCED_FACE('',(#1932),#23312,.F.);
#24039=ADVANCED_FACE('',(#1933),#23313,.F.);
#24040=ADVANCED_FACE('',(#1934),#23314,.F.);
#24041=ADVANCED_FACE('',(#1935),#23315,.F.);
#24042=ADVANCED_FACE('',(#1936),#23316,.F.);
#24043=ADVANCED_FACE('',(#1937),#23317,.F.);
#24044=ADVANCED_FACE('',(#1938),#23318,.F.);
#24045=ADVANCED_FACE('',(#1939),#23319,.F.);
#24046=ADVANCED_FACE('',(#1940),#23320,.F.);
#24047=ADVANCED_FACE('',(#1941),#23321,.F.);
#24048=ADVANCED_FACE('',(#1942),#23322,.F.);
#24049=ADVANCED_FACE('',(#1943),#23323,.F.);
#24050=ADVANCED_FACE('',(#1944),#23324,.F.);
#24051=ADVANCED_FACE('',(#1945),#23325,.F.);
#24052=ADVANCED_FACE('',(#1946),#23326,.F.);
#24053=ADVANCED_FACE('',(#1947),#23327,.F.);
#24054=ADVANCED_FACE('',(#1948),#23328,.F.);
#24055=ADVANCED_FACE('',(#1949),#23329,.F.);
#24056=ADVANCED_FACE('',(#1950),#1480,.T.);
#24057=ADVANCED_FACE('',(#1951),#23330,.F.);
#24058=ADVANCED_FACE('',(#1952),#1318,.F.);
#24059=ADVANCED_FACE('',(#1953),#1319,.F.);
#24060=ADVANCED_FACE('',(#1954),#23331,.F.);
#24061=ADVANCED_FACE('',(#1955),#1481,.T.);
#24062=ADVANCED_FACE('',(#1956),#23332,.F.);
#24063=ADVANCED_FACE('',(#1957),#1320,.F.);
#24064=ADVANCED_FACE('',(#1958),#1321,.F.);
#24065=ADVANCED_FACE('',(#1959),#23333,.F.);
#24066=ADVANCED_FACE('',(#1960),#1482,.T.);
#24067=ADVANCED_FACE('',(#1961),#23334,.F.);
#24068=ADVANCED_FACE('',(#1962),#1322,.F.);
#24069=ADVANCED_FACE('',(#1963),#1323,.F.);
#24070=ADVANCED_FACE('',(#1964),#23335,.F.);
#24071=ADVANCED_FACE('',(#1965),#1483,.T.);
#24072=ADVANCED_FACE('',(#1966),#23336,.F.);
#24073=ADVANCED_FACE('',(#1967),#1324,.F.);
#24074=ADVANCED_FACE('',(#1968),#1325,.F.);
#24075=ADVANCED_FACE('',(#1969),#23337,.F.);
#24076=ADVANCED_FACE('',(#1970),#1484,.T.);
#24077=ADVANCED_FACE('',(#1971),#23338,.F.);
#24078=ADVANCED_FACE('',(#1972),#1326,.F.);
#24079=ADVANCED_FACE('',(#1973),#1327,.F.);
#24080=ADVANCED_FACE('',(#1974),#23339,.F.);
#24081=ADVANCED_FACE('',(#1975),#1485,.T.);
#24082=ADVANCED_FACE('',(#1976),#23340,.F.);
#24083=ADVANCED_FACE('',(#1977),#1328,.F.);
#24084=ADVANCED_FACE('',(#1978),#1329,.F.);
#24085=ADVANCED_FACE('',(#1979),#23341,.F.);
#24086=ADVANCED_FACE('',(#1980),#1486,.T.);
#24087=ADVANCED_FACE('',(#1981),#23342,.F.);
#24088=ADVANCED_FACE('',(#1982),#1330,.F.);
#24089=ADVANCED_FACE('',(#1983),#1331,.F.);
#24090=ADVANCED_FACE('',(#1984),#23343,.F.);
#24091=ADVANCED_FACE('',(#1985),#1487,.T.);
#24092=ADVANCED_FACE('',(#1986),#23344,.F.);
#24093=ADVANCED_FACE('',(#1987),#1332,.F.);
#24094=ADVANCED_FACE('',(#1988),#1333,.F.);
#24095=ADVANCED_FACE('',(#1989),#23345,.F.);
#24096=ADVANCED_FACE('',(#1990),#1488,.F.);
#24097=ADVANCED_FACE('',(#1991),#1489,.F.);
#24098=ADVANCED_FACE('',(#1992),#1490,.F.);
#24099=ADVANCED_FACE('',(#1993),#1491,.F.);
#24100=ADVANCED_FACE('',(#1994),#1492,.F.);
#24101=ADVANCED_FACE('',(#1995),#1493,.F.);
#24102=ADVANCED_FACE('',(#1996),#1494,.F.);
#24103=ADVANCED_FACE('',(#1997),#1495,.F.);
#24104=ADVANCED_FACE('',(#1998),#23346,.F.);
#24105=ADVANCED_FACE('',(#1999),#23347,.F.);
#24106=ADVANCED_FACE('',(#2000),#23348,.F.);
#24107=ADVANCED_FACE('',(#2001),#23349,.F.);
#24108=ADVANCED_FACE('',(#2002),#23350,.F.);
#24109=ADVANCED_FACE('',(#2003,#1203),#1496,.F.);
#24110=ADVANCED_FACE('',(#2004,#1204,#1205,#1206,#1207,#1208,#1209,#1210,
#1211,#1212),#23351,.F.);
#24111=ADVANCED_FACE('',(#2005,#1213,#1214,#1215,#1216,#1217,#1218,#1219,
#1220,#1221),#23352,.T.);
#24112=ADVANCED_FACE('',(#2006,#1222,#1223,#1224,#1225,#1226,#1227,#1228,
#1229,#1230),#1497,.T.);
#24113=ADVANCED_FACE('',(#2007,#1231,#1232,#1233,#1234,#1235),#1498,.T.);
#24114=ADVANCED_FACE('',(#2008),#23353,.F.);
#24115=ADVANCED_FACE('',(#2009),#23354,.T.);
#24116=ADVANCED_FACE('',(#2010,#1236),#1499,.T.);
#24117=ADVANCED_FACE('',(#2011,#1237,#1238,#1239,#1240,#1241),#1500,.F.);
#25150=CLOSED_SHELL('',(#23804,#23805,#23806,#23807,#23808,#23809,#23810,
#23811,#23812,#23813,#23814,#23815,#23816,#23817,#23818,#23819,#23820,#23821,
#23822,#23823,#23824,#23825,#23826,#23827,#23828,#23829,#23830,#23831,#23832,
#23833,#23834,#23835,#23836,#23837,#23838,#23839,#23840,#23841,#23842,#23843,
#23844,#23845,#23846,#23847,#23848,#23849,#23850,#23851,#23852,#23853,#23854,
#23855,#23856,#23857,#23858,#23859,#23860,#23861,#23862,#23863,#23864,#23865,
#23866,#23867,#23868,#23869,#23870,#23871,#23872,#23873,#23874,#23875,#23876,
#23877,#23878,#23879,#23880,#23881,#23882,#23883,#23884,#23885,#23886,#23887,
#23888,#23889,#23890,#23891,#23892,#23893,#23894,#23895,#23896,#23897,#23898,
#23899,#23900,#23901,#23902,#23903,#23904,#23905,#23906,#23907,#23908,#23909,
#23910,#23911,#23912,#23913,#23914,#23915,#23916,#23917,#23918,#23919,#23920,
#23921,#23922,#23923,#23924,#23925,#23926,#23927,#23928,#23929,#23930,#23931,
#23932,#23933,#23934,#23935,#23936,#23937,#23938,#23939,#23940,#23941,#23942,
#23943,#23944,#23945,#23946,#23947,#23948,#23949,#23950,#23951,#23952,#23953,
#23954,#23955,#23956,#23957,#23958,#23959,#23960,#23961,#23962,#23963,#23964,
#23965,#23966,#23967,#23968,#23969,#23970,#23971,#23972,#23973,#23974,#23975,
#23976,#23977,#23978,#23979,#23980,#23981,#23982,#23983,#23984,#23985,#23986,
#23987,#23988,#23989,#23990,#23991,#23992,#23993,#23994,#23995,#23996,#23997,
#23998,#23999,#24000,#24001,#24002,#24003,#24004,#24005,#24006,#24007,#24008,
#24009,#24010,#24011,#24012,#24013,#24014,#24015,#24016,#24017,#24018,#24019,
#24020,#24021,#24022,#24023,#24024,#24025,#24026,#24027,#24028,#24029,#24030,
#24031,#24032,#24033,#24034,#24035,#24036,#24037,#24038,#24039,#24040,#24041,
#24042,#24043,#24044,#24045,#24046,#24047,#24048,#24049,#24050,#24051,#24052,
#24053,#24054,#24055,#24056,#24057,#24058,#24059,#24060,#24061,#24062,#24063,
#24064,#24065,#24066,#24067,#24068,#24069,#24070,#24071,#24072,#24073,#24074,
#24075,#24076,#24077,#24078,#24079,#24080,#24081,#24082,#24083,#24084,#24085,
#24086,#24087,#24088,#24089,#24090,#24091,#24092,#24093,#24094,#24095,#24096,
#24097,#24098,#24099,#24100,#24101,#24102,#24103,#24104,#24105,#24106,#24107,
#24108,#24109,#24110,#24111,#24112,#24113,#24114,#24115,#24116,#24117));
#25392=AXIS2_PLACEMENT_3D('',#32406,#27336,#27337);
#25393=AXIS2_PLACEMENT_3D('',#32407,#27338,#27339);
#25394=AXIS2_PLACEMENT_3D('',#32417,#27341,#27342);
#25395=AXIS2_PLACEMENT_3D('',#32420,#27344,#27345);
#25396=AXIS2_PLACEMENT_3D('',#32422,#27346,#27347);
#25397=AXIS2_PLACEMENT_3D('',#32433,#27348,#27349);
#25398=AXIS2_PLACEMENT_3D('',#32484,#27351,#27352);
#25399=AXIS2_PLACEMENT_3D('',#32535,#27354,#27355);
#25400=AXIS2_PLACEMENT_3D('',#32583,#27357,#27358);
#25401=AXIS2_PLACEMENT_3D('',#32634,#27360,#27361);
#25402=AXIS2_PLACEMENT_3D('',#32685,#27363,#27364);
#25403=AXIS2_PLACEMENT_3D('',#32733,#27366,#27367);
#25404=AXIS2_PLACEMENT_3D('',#32784,#27369,#27370);
#25405=AXIS2_PLACEMENT_3D('',#32835,#27372,#27373);
#25406=AXIS2_PLACEMENT_3D('',#32883,#27375,#27376);
#25407=AXIS2_PLACEMENT_3D('',#32934,#27378,#27379);
#25408=AXIS2_PLACEMENT_3D('',#32985,#27381,#27382);
#25409=AXIS2_PLACEMENT_3D('',#33033,#27384,#27385);
#25410=AXIS2_PLACEMENT_3D('',#33084,#27387,#27388);
#25411=AXIS2_PLACEMENT_3D('',#33103,#27390,#27391);
#25412=AXIS2_PLACEMENT_3D('',#33123,#27392,#27393);
#25413=AXIS2_PLACEMENT_3D('',#33137,#27395,#27396);
#25414=AXIS2_PLACEMENT_3D('',#33147,#27397,#27398);
#25415=AXIS2_PLACEMENT_3D('',#33171,#27400,#27401);
#25416=AXIS2_PLACEMENT_3D('',#33196,#27403,#27404);
#25417=AXIS2_PLACEMENT_3D('',#33221,#27406,#27407);
#25418=AXIS2_PLACEMENT_3D('',#33245,#27409,#27410);
#25419=AXIS2_PLACEMENT_3D('',#33270,#27412,#27413);
#25420=AXIS2_PLACEMENT_3D('',#33295,#27415,#27416);
#25421=AXIS2_PLACEMENT_3D('',#33319,#27418,#27419);
#25422=AXIS2_PLACEMENT_3D('',#33344,#27421,#27422);
#25423=AXIS2_PLACEMENT_3D('',#33369,#27424,#27425);
#25424=AXIS2_PLACEMENT_3D('',#33393,#27427,#27428);
#25425=AXIS2_PLACEMENT_3D('',#33418,#27430,#27431);
#25426=AXIS2_PLACEMENT_3D('',#33443,#27433,#27434);
#25427=AXIS2_PLACEMENT_3D('',#33467,#27436,#27437);
#25428=AXIS2_PLACEMENT_3D('',#33478,#27439,#27440);
#25429=AXIS2_PLACEMENT_3D('',#33484,#27441,#27442);
#25430=AXIS2_PLACEMENT_3D('',#33494,#27444,#27445);
#25431=AXIS2_PLACEMENT_3D('',#33497,#27447,#27448);
#25432=AXIS2_PLACEMENT_3D('',#33499,#27449,#27450);
#25433=AXIS2_PLACEMENT_3D('',#33510,#27451,#27452);
#25434=AXIS2_PLACEMENT_3D('',#33561,#27454,#27455);
#25435=AXIS2_PLACEMENT_3D('',#33612,#27457,#27458);
#25436=AXIS2_PLACEMENT_3D('',#33660,#27460,#27461);
#25437=AXIS2_PLACEMENT_3D('',#33711,#27463,#27464);
#25438=AXIS2_PLACEMENT_3D('',#33762,#27466,#27467);
#25439=AXIS2_PLACEMENT_3D('',#33810,#27469,#27470);
#25440=AXIS2_PLACEMENT_3D('',#33861,#27472,#27473);
#25441=AXIS2_PLACEMENT_3D('',#33912,#27475,#27476);
#25442=AXIS2_PLACEMENT_3D('',#33960,#27478,#27479);
#25443=AXIS2_PLACEMENT_3D('',#34011,#27481,#27482);
#25444=AXIS2_PLACEMENT_3D('',#34062,#27484,#27485);
#25445=AXIS2_PLACEMENT_3D('',#34110,#27487,#27488);
#25446=AXIS2_PLACEMENT_3D('',#34161,#27490,#27491);
#25447=AXIS2_PLACEMENT_3D('',#34180,#27493,#27494);
#25448=AXIS2_PLACEMENT_3D('',#34200,#27495,#27496);
#25449=AXIS2_PLACEMENT_3D('',#34214,#27498,#27499);
#25450=AXIS2_PLACEMENT_3D('',#34224,#27500,#27501);
#25451=AXIS2_PLACEMENT_3D('',#34248,#27503,#27504);
#25452=AXIS2_PLACEMENT_3D('',#34273,#27506,#27507);
#25453=AXIS2_PLACEMENT_3D('',#34298,#27509,#27510);
#25454=AXIS2_PLACEMENT_3D('',#34322,#27512,#27513);
#25455=AXIS2_PLACEMENT_3D('',#34347,#27515,#27516);
#25456=AXIS2_PLACEMENT_3D('',#34372,#27518,#27519);
#25457=AXIS2_PLACEMENT_3D('',#34396,#27521,#27522);
#25458=AXIS2_PLACEMENT_3D('',#34421,#27524,#27525);
#25459=AXIS2_PLACEMENT_3D('',#34446,#27527,#27528);
#25460=AXIS2_PLACEMENT_3D('',#34470,#27530,#27531);
#25461=AXIS2_PLACEMENT_3D('',#34495,#27533,#27534);
#25462=AXIS2_PLACEMENT_3D('',#34520,#27536,#27537);
#25463=AXIS2_PLACEMENT_3D('',#34544,#27539,#27540);
#25464=AXIS2_PLACEMENT_3D('',#34555,#27542,#27543);
#25465=AXIS2_PLACEMENT_3D('',#34561,#27544,#27545);
#25466=AXIS2_PLACEMENT_3D('',#34571,#27547,#27548);
#25467=AXIS2_PLACEMENT_3D('',#34574,#27550,#27551);
#25468=AXIS2_PLACEMENT_3D('',#34576,#27552,#27553);
#25469=AXIS2_PLACEMENT_3D('',#34587,#27554,#27555);
#25470=AXIS2_PLACEMENT_3D('',#34638,#27557,#27558);
#25471=AXIS2_PLACEMENT_3D('',#34689,#27560,#27561);
#25472=AXIS2_PLACEMENT_3D('',#34737,#27563,#27564);
#25473=AXIS2_PLACEMENT_3D('',#34788,#27566,#27567);
#25474=AXIS2_PLACEMENT_3D('',#34839,#27569,#27570);
#25475=AXIS2_PLACEMENT_3D('',#34887,#27572,#27573);
#25476=AXIS2_PLACEMENT_3D('',#34938,#27575,#27576);
#25477=AXIS2_PLACEMENT_3D('',#34989,#27578,#27579);
#25478=AXIS2_PLACEMENT_3D('',#35037,#27581,#27582);
#25479=AXIS2_PLACEMENT_3D('',#35088,#27584,#27585);
#25480=AXIS2_PLACEMENT_3D('',#35139,#27587,#27588);
#25481=AXIS2_PLACEMENT_3D('',#35187,#27590,#27591);
#25482=AXIS2_PLACEMENT_3D('',#35238,#27593,#27594);
#25483=AXIS2_PLACEMENT_3D('',#35257,#27596,#27597);
#25484=AXIS2_PLACEMENT_3D('',#35277,#27598,#27599);
#25485=AXIS2_PLACEMENT_3D('',#35291,#27601,#27602);
#25486=AXIS2_PLACEMENT_3D('',#35301,#27603,#27604);
#25487=AXIS2_PLACEMENT_3D('',#35325,#27606,#27607);
#25488=AXIS2_PLACEMENT_3D('',#35350,#27609,#27610);
#25489=AXIS2_PLACEMENT_3D('',#35375,#27612,#27613);
#25490=AXIS2_PLACEMENT_3D('',#35399,#27615,#27616);
#25491=AXIS2_PLACEMENT_3D('',#35424,#27618,#27619);
#25492=AXIS2_PLACEMENT_3D('',#35449,#27621,#27622);
#25493=AXIS2_PLACEMENT_3D('',#35473,#27624,#27625);
#25494=AXIS2_PLACEMENT_3D('',#35498,#27627,#27628);
#25495=AXIS2_PLACEMENT_3D('',#35523,#27630,#27631);
#25496=AXIS2_PLACEMENT_3D('',#35547,#27633,#27634);
#25497=AXIS2_PLACEMENT_3D('',#35572,#27636,#27637);
#25498=AXIS2_PLACEMENT_3D('',#35597,#27639,#27640);
#25499=AXIS2_PLACEMENT_3D('',#35621,#27642,#27643);
#25500=AXIS2_PLACEMENT_3D('',#35632,#27645,#27646);
#25501=AXIS2_PLACEMENT_3D('',#35638,#27647,#27648);
#25502=AXIS2_PLACEMENT_3D('',#35648,#27650,#27651);
#25503=AXIS2_PLACEMENT_3D('',#35651,#27653,#27654);
#25504=AXIS2_PLACEMENT_3D('',#35653,#27655,#27656);
#25505=AXIS2_PLACEMENT_3D('',#35664,#27657,#27658);
#25506=AXIS2_PLACEMENT_3D('',#35715,#27660,#27661);
#25507=AXIS2_PLACEMENT_3D('',#35766,#27663,#27664);
#25508=AXIS2_PLACEMENT_3D('',#35814,#27666,#27667);
#25509=AXIS2_PLACEMENT_3D('',#35865,#27669,#27670);
#25510=AXIS2_PLACEMENT_3D('',#35916,#27672,#27673);
#25511=AXIS2_PLACEMENT_3D('',#35964,#27675,#27676);
#25512=AXIS2_PLACEMENT_3D('',#36015,#27678,#27679);
#25513=AXIS2_PLACEMENT_3D('',#36066,#27681,#27682);
#25514=AXIS2_PLACEMENT_3D('',#36114,#27684,#27685);
#25515=AXIS2_PLACEMENT_3D('',#36165,#27687,#27688);
#25516=AXIS2_PLACEMENT_3D('',#36216,#27690,#27691);
#25517=AXIS2_PLACEMENT_3D('',#36264,#27693,#27694);
#25518=AXIS2_PLACEMENT_3D('',#36315,#27696,#27697);
#25519=AXIS2_PLACEMENT_3D('',#36334,#27699,#27700);
#25520=AXIS2_PLACEMENT_3D('',#36354,#27701,#27702);
#25521=AXIS2_PLACEMENT_3D('',#36368,#27704,#27705);
#25522=AXIS2_PLACEMENT_3D('',#36378,#27706,#27707);
#25523=AXIS2_PLACEMENT_3D('',#36402,#27709,#27710);
#25524=AXIS2_PLACEMENT_3D('',#36427,#27712,#27713);
#25525=AXIS2_PLACEMENT_3D('',#36452,#27715,#27716);
#25526=AXIS2_PLACEMENT_3D('',#36476,#27718,#27719);
#25527=AXIS2_PLACEMENT_3D('',#36501,#27721,#27722);
#25528=AXIS2_PLACEMENT_3D('',#36526,#27724,#27725);
#25529=AXIS2_PLACEMENT_3D('',#36550,#27727,#27728);
#25530=AXIS2_PLACEMENT_3D('',#36575,#27730,#27731);
#25531=AXIS2_PLACEMENT_3D('',#36600,#27733,#27734);
#25532=AXIS2_PLACEMENT_3D('',#36624,#27736,#27737);
#25533=AXIS2_PLACEMENT_3D('',#36649,#27739,#27740);
#25534=AXIS2_PLACEMENT_3D('',#36674,#27742,#27743);
#25535=AXIS2_PLACEMENT_3D('',#36698,#27745,#27746);
#25536=AXIS2_PLACEMENT_3D('',#36709,#27748,#27749);
#25537=AXIS2_PLACEMENT_3D('',#36715,#27750,#27751);
#25538=AXIS2_PLACEMENT_3D('',#36725,#27753,#27754);
#25539=AXIS2_PLACEMENT_3D('',#36728,#27756,#27757);
#25540=AXIS2_PLACEMENT_3D('',#36730,#27758,#27759);
#25541=AXIS2_PLACEMENT_3D('',#36741,#27760,#27761);
#25542=AXIS2_PLACEMENT_3D('',#36792,#27763,#27764);
#25543=AXIS2_PLACEMENT_3D('',#36843,#27766,#27767);
#25544=AXIS2_PLACEMENT_3D('',#36891,#27769,#27770);
#25545=AXIS2_PLACEMENT_3D('',#36942,#27772,#27773);
#25546=AXIS2_PLACEMENT_3D('',#36993,#27775,#27776);
#25547=AXIS2_PLACEMENT_3D('',#37041,#27778,#27779);
#25548=AXIS2_PLACEMENT_3D('',#37092,#27781,#27782);
#25549=AXIS2_PLACEMENT_3D('',#37143,#27784,#27785);
#25550=AXIS2_PLACEMENT_3D('',#37191,#27787,#27788);
#25551=AXIS2_PLACEMENT_3D('',#37242,#27790,#27791);
#25552=AXIS2_PLACEMENT_3D('',#37293,#27793,#27794);
#25553=AXIS2_PLACEMENT_3D('',#37341,#27796,#27797);
#25554=AXIS2_PLACEMENT_3D('',#37392,#27799,#27800);
#25555=AXIS2_PLACEMENT_3D('',#37411,#27802,#27803);
#25556=AXIS2_PLACEMENT_3D('',#37431,#27804,#27805);
#25557=AXIS2_PLACEMENT_3D('',#37445,#27807,#27808);
#25558=AXIS2_PLACEMENT_3D('',#37455,#27809,#27810);
#25559=AXIS2_PLACEMENT_3D('',#37479,#27812,#27813);
#25560=AXIS2_PLACEMENT_3D('',#37504,#27815,#27816);
#25561=AXIS2_PLACEMENT_3D('',#37529,#27818,#27819);
#25562=AXIS2_PLACEMENT_3D('',#37553,#27821,#27822);
#25563=AXIS2_PLACEMENT_3D('',#37578,#27824,#27825);
#25564=AXIS2_PLACEMENT_3D('',#37603,#27827,#27828);
#25565=AXIS2_PLACEMENT_3D('',#37627,#27830,#27831);
#25566=AXIS2_PLACEMENT_3D('',#37652,#27833,#27834);
#25567=AXIS2_PLACEMENT_3D('',#37677,#27836,#27837);
#25568=AXIS2_PLACEMENT_3D('',#37701,#27839,#27840);
#25569=AXIS2_PLACEMENT_3D('',#37726,#27842,#27843);
#25570=AXIS2_PLACEMENT_3D('',#37751,#27845,#27846);
#25571=AXIS2_PLACEMENT_3D('',#37775,#27848,#27849);
#25572=AXIS2_PLACEMENT_3D('',#37786,#27851,#27852);
#25573=AXIS2_PLACEMENT_3D('',#37792,#27853,#27854);
#25574=AXIS2_PLACEMENT_3D('',#37802,#27856,#27857);
#25575=AXIS2_PLACEMENT_3D('',#37805,#27859,#27860);
#25576=AXIS2_PLACEMENT_3D('',#37807,#27861,#27862);
#25577=AXIS2_PLACEMENT_3D('',#37818,#27863,#27864);
#25578=AXIS2_PLACEMENT_3D('',#37869,#27866,#27867);
#25579=AXIS2_PLACEMENT_3D('',#37920,#27869,#27870);
#25580=AXIS2_PLACEMENT_3D('',#37968,#27872,#27873);
#25581=AXIS2_PLACEMENT_3D('',#38019,#27875,#27876);
#25582=AXIS2_PLACEMENT_3D('',#38070,#27878,#27879);
#25583=AXIS2_PLACEMENT_3D('',#38118,#27881,#27882);
#25584=AXIS2_PLACEMENT_3D('',#38169,#27884,#27885);
#25585=AXIS2_PLACEMENT_3D('',#38220,#27887,#27888);
#25586=AXIS2_PLACEMENT_3D('',#38268,#27890,#27891);
#25587=AXIS2_PLACEMENT_3D('',#38319,#27893,#27894);
#25588=AXIS2_PLACEMENT_3D('',#38370,#27896,#27897);
#25589=AXIS2_PLACEMENT_3D('',#38418,#27899,#27900);
#25590=AXIS2_PLACEMENT_3D('',#38469,#27902,#27903);
#25591=AXIS2_PLACEMENT_3D('',#38488,#27905,#27906);
#25592=AXIS2_PLACEMENT_3D('',#38508,#27907,#27908);
#25593=AXIS2_PLACEMENT_3D('',#38522,#27910,#27911);
#25594=AXIS2_PLACEMENT_3D('',#38532,#27912,#27913);
#25595=AXIS2_PLACEMENT_3D('',#38556,#27915,#27916);
#25596=AXIS2_PLACEMENT_3D('',#38581,#27918,#27919);
#25597=AXIS2_PLACEMENT_3D('',#38606,#27921,#27922);
#25598=AXIS2_PLACEMENT_3D('',#38630,#27924,#27925);
#25599=AXIS2_PLACEMENT_3D('',#38655,#27927,#27928);
#25600=AXIS2_PLACEMENT_3D('',#38680,#27930,#27931);
#25601=AXIS2_PLACEMENT_3D('',#38704,#27933,#27934);
#25602=AXIS2_PLACEMENT_3D('',#38729,#27936,#27937);
#25603=AXIS2_PLACEMENT_3D('',#38754,#27939,#27940);
#25604=AXIS2_PLACEMENT_3D('',#38778,#27942,#27943);
#25605=AXIS2_PLACEMENT_3D('',#38803,#27945,#27946);
#25606=AXIS2_PLACEMENT_3D('',#38828,#27948,#27949);
#25607=AXIS2_PLACEMENT_3D('',#38852,#27951,#27952);
#25608=AXIS2_PLACEMENT_3D('',#38863,#27954,#27955);
#25609=AXIS2_PLACEMENT_3D('',#38869,#27956,#27957);
#25610=AXIS2_PLACEMENT_3D('',#38879,#27959,#27960);
#25611=AXIS2_PLACEMENT_3D('',#38882,#27962,#27963);
#25612=AXIS2_PLACEMENT_3D('',#38884,#27964,#27965);
#25613=AXIS2_PLACEMENT_3D('',#38895,#27966,#27967);
#25614=AXIS2_PLACEMENT_3D('',#38946,#27969,#27970);
#25615=AXIS2_PLACEMENT_3D('',#38997,#27972,#27973);
#25616=AXIS2_PLACEMENT_3D('',#39045,#27975,#27976);
#25617=AXIS2_PLACEMENT_3D('',#39096,#27978,#27979);
#25618=AXIS2_PLACEMENT_3D('',#39147,#27981,#27982);
#25619=AXIS2_PLACEMENT_3D('',#39195,#27984,#27985);
#25620=AXIS2_PLACEMENT_3D('',#39246,#27987,#27988);
#25621=AXIS2_PLACEMENT_3D('',#39297,#27990,#27991);
#25622=AXIS2_PLACEMENT_3D('',#39345,#27993,#27994);
#25623=AXIS2_PLACEMENT_3D('',#39396,#27996,#27997);
#25624=AXIS2_PLACEMENT_3D('',#39447,#27999,#28000);
#25625=AXIS2_PLACEMENT_3D('',#39495,#28002,#28003);
#25626=AXIS2_PLACEMENT_3D('',#39546,#28005,#28006);
#25627=AXIS2_PLACEMENT_3D('',#39565,#28008,#28009);
#25628=AXIS2_PLACEMENT_3D('',#39585,#28010,#28011);
#25629=AXIS2_PLACEMENT_3D('',#39599,#28013,#28014);
#25630=AXIS2_PLACEMENT_3D('',#39609,#28015,#28016);
#25631=AXIS2_PLACEMENT_3D('',#39633,#28018,#28019);
#25632=AXIS2_PLACEMENT_3D('',#39658,#28021,#28022);
#25633=AXIS2_PLACEMENT_3D('',#39683,#28024,#28025);
#25634=AXIS2_PLACEMENT_3D('',#39707,#28027,#28028);
#25635=AXIS2_PLACEMENT_3D('',#39732,#28030,#28031);
#25636=AXIS2_PLACEMENT_3D('',#39757,#28033,#28034);
#25637=AXIS2_PLACEMENT_3D('',#39781,#28036,#28037);
#25638=AXIS2_PLACEMENT_3D('',#39806,#28039,#28040);
#25639=AXIS2_PLACEMENT_3D('',#39831,#28042,#28043);
#25640=AXIS2_PLACEMENT_3D('',#39855,#28045,#28046);
#25641=AXIS2_PLACEMENT_3D('',#39880,#28048,#28049);
#25642=AXIS2_PLACEMENT_3D('',#39905,#28051,#28052);
#25643=AXIS2_PLACEMENT_3D('',#39929,#28054,#28055);
#25644=AXIS2_PLACEMENT_3D('',#39940,#28057,#28058);
#25645=AXIS2_PLACEMENT_3D('',#39946,#28059,#28060);
#25646=AXIS2_PLACEMENT_3D('',#39956,#28062,#28063);
#25647=AXIS2_PLACEMENT_3D('',#39959,#28065,#28066);
#25648=AXIS2_PLACEMENT_3D('',#39961,#28067,#28068);
#25649=AXIS2_PLACEMENT_3D('',#39972,#28069,#28070);
#25650=AXIS2_PLACEMENT_3D('',#40023,#28072,#28073);
#25651=AXIS2_PLACEMENT_3D('',#40074,#28075,#28076);
#25652=AXIS2_PLACEMENT_3D('',#40122,#28078,#28079);
#25653=AXIS2_PLACEMENT_3D('',#40173,#28081,#28082);
#25654=AXIS2_PLACEMENT_3D('',#40224,#28084,#28085);
#25655=AXIS2_PLACEMENT_3D('',#40272,#28087,#28088);
#25656=AXIS2_PLACEMENT_3D('',#40323,#28090,#28091);
#25657=AXIS2_PLACEMENT_3D('',#40374,#28093,#28094);
#25658=AXIS2_PLACEMENT_3D('',#40422,#28096,#28097);
#25659=AXIS2_PLACEMENT_3D('',#40473,#28099,#28100);
#25660=AXIS2_PLACEMENT_3D('',#40524,#28102,#28103);
#25661=AXIS2_PLACEMENT_3D('',#40572,#28105,#28106);
#25662=AXIS2_PLACEMENT_3D('',#40623,#28108,#28109);
#25663=AXIS2_PLACEMENT_3D('',#40642,#28111,#28112);
#25664=AXIS2_PLACEMENT_3D('',#40662,#28113,#28114);
#25665=AXIS2_PLACEMENT_3D('',#40676,#28116,#28117);
#25666=AXIS2_PLACEMENT_3D('',#40686,#28118,#28119);
#25667=AXIS2_PLACEMENT_3D('',#40710,#28121,#28122);
#25668=AXIS2_PLACEMENT_3D('',#40735,#28124,#28125);
#25669=AXIS2_PLACEMENT_3D('',#40760,#28127,#28128);
#25670=AXIS2_PLACEMENT_3D('',#40784,#28130,#28131);
#25671=AXIS2_PLACEMENT_3D('',#40809,#28133,#28134);
#25672=AXIS2_PLACEMENT_3D('',#40834,#28136,#28137);
#25673=AXIS2_PLACEMENT_3D('',#40858,#28139,#28140);
#25674=AXIS2_PLACEMENT_3D('',#40883,#28142,#28143);
#25675=AXIS2_PLACEMENT_3D('',#40908,#28145,#28146);
#25676=AXIS2_PLACEMENT_3D('',#40932,#28148,#28149);
#25677=AXIS2_PLACEMENT_3D('',#40957,#28151,#28152);
#25678=AXIS2_PLACEMENT_3D('',#40982,#28154,#28155);
#25679=AXIS2_PLACEMENT_3D('',#41006,#28157,#28158);
#25680=AXIS2_PLACEMENT_3D('',#41017,#28160,#28161);
#25681=AXIS2_PLACEMENT_3D('',#41023,#28162,#28163);
#25682=AXIS2_PLACEMENT_3D('',#41102,#28165,#28166);
#25683=AXIS2_PLACEMENT_3D('',#41181,#28168,#28169);
#25684=AXIS2_PLACEMENT_3D('',#41265,#28171,#28172);
#25685=AXIS2_PLACEMENT_3D('',#41343,#28174,#28175);
#25686=AXIS2_PLACEMENT_3D('',#41422,#28177,#28178);
#25687=AXIS2_PLACEMENT_3D('',#41501,#28180,#28181);
#25688=AXIS2_PLACEMENT_3D('',#41585,#28183,#28184);
#25689=AXIS2_PLACEMENT_3D('',#41663,#28186,#28187);
#25690=AXIS2_PLACEMENT_3D('',#41742,#28189,#28190);
#25691=AXIS2_PLACEMENT_3D('',#41821,#28192,#28193);
#25692=AXIS2_PLACEMENT_3D('',#41905,#28195,#28196);
#25693=AXIS2_PLACEMENT_3D('',#41983,#28198,#28199);
#25694=AXIS2_PLACEMENT_3D('',#42175,#28200,#28201);
#25695=AXIS2_PLACEMENT_3D('',#43229,#28202,#28203);
#25696=AXIS2_PLACEMENT_3D('',#43230,#28204,#28205);
#25697=AXIS2_PLACEMENT_3D('',#43422,#28206,#28207);
#25698=AXIS2_PLACEMENT_3D('',#44476,#28208,#28209);
#25699=AXIS2_PLACEMENT_3D('',#44477,#28210,#28211);
#25700=AXIS2_PLACEMENT_3D('',#44669,#28212,#28213);
#25701=AXIS2_PLACEMENT_3D('',#45723,#28214,#28215);
#25702=AXIS2_PLACEMENT_3D('',#45724,#28216,#28217);
#25703=AXIS2_PLACEMENT_3D('',#45916,#28218,#28219);
#25704=AXIS2_PLACEMENT_3D('',#46970,#28220,#28221);
#25705=AXIS2_PLACEMENT_3D('',#46971,#28222,#28223);
#25706=AXIS2_PLACEMENT_3D('',#47163,#28224,#28225);
#25707=AXIS2_PLACEMENT_3D('',#48217,#28226,#28227);
#25708=AXIS2_PLACEMENT_3D('',#48218,#28228,#28229);
#25709=AXIS2_PLACEMENT_3D('',#48410,#28230,#28231);
#25710=AXIS2_PLACEMENT_3D('',#49464,#28232,#28233);
#25711=AXIS2_PLACEMENT_3D('',#49465,#28234,#28235);
#25712=AXIS2_PLACEMENT_3D('',#49657,#28236,#28237);
#25713=AXIS2_PLACEMENT_3D('',#50711,#28238,#28239);
#25714=AXIS2_PLACEMENT_3D('',#50712,#28240,#28241);
#25715=AXIS2_PLACEMENT_3D('',#50904,#28242,#28243);
#25716=AXIS2_PLACEMENT_3D('',#51958,#28244,#28245);
#25717=AXIS2_PLACEMENT_3D('',#51959,#28246,#28247);
#25718=AXIS2_PLACEMENT_3D('',#51960,#28248,#28249);
#25719=AXIS2_PLACEMENT_3D('',#51961,#28250,#28251);
#25720=AXIS2_PLACEMENT_3D('',#51962,#28252,#28253);
#25721=AXIS2_PLACEMENT_3D('',#51963,#28254,#28255);
#25722=AXIS2_PLACEMENT_3D('',#51964,#28256,#28257);
#25723=AXIS2_PLACEMENT_3D('',#51965,#28258,#28259);
#25724=AXIS2_PLACEMENT_3D('',#51966,#28260,#28261);
#25725=AXIS2_PLACEMENT_3D('',#51967,#28262,#28263);
#25726=AXIS2_PLACEMENT_3D('',#51969,#28264,#28265);
#25727=AXIS2_PLACEMENT_3D('',#51972,#28267,#28268);
#25728=AXIS2_PLACEMENT_3D('',#51973,#28269,#28270);
#25729=AXIS2_PLACEMENT_3D('',#51975,#28271,#28272);
#25730=AXIS2_PLACEMENT_3D('',#51978,#28274,#28275);
#25731=AXIS2_PLACEMENT_3D('',#51979,#28276,#28277);
#25732=AXIS2_PLACEMENT_3D('',#51981,#28278,#28279);
#25733=AXIS2_PLACEMENT_3D('',#51984,#28281,#28282);
#25734=AXIS2_PLACEMENT_3D('',#51985,#28283,#28284);
#25735=AXIS2_PLACEMENT_3D('',#51987,#28285,#28286);
#25736=AXIS2_PLACEMENT_3D('',#51990,#28288,#28289);
#25737=AXIS2_PLACEMENT_3D('',#51991,#28290,#28291);
#25738=AXIS2_PLACEMENT_3D('',#51993,#28292,#28293);
#25739=AXIS2_PLACEMENT_3D('',#51996,#28295,#28296);
#25740=AXIS2_PLACEMENT_3D('',#51997,#28297,#28298);
#25741=AXIS2_PLACEMENT_3D('',#51999,#28299,#28300);
#25742=AXIS2_PLACEMENT_3D('',#52000,#28301,#28302);
#25743=AXIS2_PLACEMENT_3D('',#52002,#28303,#28304);
#25744=AXIS2_PLACEMENT_3D('',#52008,#28309,#28310);
#25745=AXIS2_PLACEMENT_3D('',#52009,#28311,#28312);
#25746=AXIS2_PLACEMENT_3D('',#52011,#28313,#28314);
#25747=AXIS2_PLACEMENT_3D('',#52017,#28319,#28320);
#25748=AXIS2_PLACEMENT_3D('',#52018,#28321,#28322);
#25749=AXIS2_PLACEMENT_3D('',#52019,#28323,#28324);
#25750=AXIS2_PLACEMENT_3D('',#52021,#28325,#28326);
#25751=AXIS2_PLACEMENT_3D('',#52022,#28327,#28328);
#25752=AXIS2_PLACEMENT_3D('',#52025,#28330,#28331);
#25753=AXIS2_PLACEMENT_3D('',#52026,#28332,#28333);
#25754=AXIS2_PLACEMENT_3D('',#52029,#28335,#28336);
#25755=AXIS2_PLACEMENT_3D('',#52030,#28337,#28338);
#25756=AXIS2_PLACEMENT_3D('',#52031,#28339,#28340);
#27336=DIRECTION('axis',(0.,0.,1.));
#27337=DIRECTION('refdir',(1.,0.,0.));
#27338=DIRECTION('center_axis',(0.,0.,-1.));
#27339=DIRECTION('ref_axis',(1.,0.,0.));
#27340=DIRECTION('',(0.,0.,-1.));
#27341=DIRECTION('center_axis',(0.,0.,1.));
#27342=DIRECTION('ref_axis',(1.,0.,0.));
#27343=DIRECTION('',(0.,0.,-1.));
#27344=DIRECTION('center_axis',(0.,0.,1.));
#27345=DIRECTION('ref_axis',(1.,0.,0.));
#27346=DIRECTION('center_axis',(0.,0.,1.));
#27347=DIRECTION('ref_axis',(1.,0.,0.));
#27348=DIRECTION('center_axis',(0.,0.,-1.));
#27349=DIRECTION('ref_axis',(1.,0.,0.));
#27350=DIRECTION('',(0.,0.,-1.));
#27351=DIRECTION('center_axis',(0.,0.,-1.));
#27352=DIRECTION('ref_axis',(1.,0.,0.));
#27353=DIRECTION('',(0.,0.,-1.));
#27354=DIRECTION('center_axis',(0.,0.,-1.));
#27355=DIRECTION('ref_axis',(1.,0.,0.));
#27356=DIRECTION('',(0.,0.,-1.));
#27357=DIRECTION('center_axis',(0.,0.,-1.));
#27358=DIRECTION('ref_axis',(1.,0.,0.));
#27359=DIRECTION('',(0.,0.,-1.));
#27360=DIRECTION('center_axis',(0.,0.,-1.));
#27361=DIRECTION('ref_axis',(1.,0.,0.));
#27362=DIRECTION('',(0.,0.,-1.));
#27363=DIRECTION('center_axis',(0.,0.,-1.));
#27364=DIRECTION('ref_axis',(1.,0.,0.));
#27365=DIRECTION('',(0.,0.,-1.));
#27366=DIRECTION('center_axis',(0.,0.,-1.));
#27367=DIRECTION('ref_axis',(1.,0.,0.));
#27368=DIRECTION('',(0.,0.,-1.));
#27369=DIRECTION('center_axis',(0.,0.,-1.));
#27370=DIRECTION('ref_axis',(1.,0.,0.));
#27371=DIRECTION('',(0.,0.,-1.));
#27372=DIRECTION('center_axis',(0.,0.,-1.));
#27373=DIRECTION('ref_axis',(1.,0.,0.));
#27374=DIRECTION('',(0.,0.,-1.));
#27375=DIRECTION('center_axis',(0.,0.,-1.));
#27376=DIRECTION('ref_axis',(1.,0.,0.));
#27377=DIRECTION('',(0.,0.,-1.));
#27378=DIRECTION('center_axis',(0.,0.,-1.));
#27379=DIRECTION('ref_axis',(1.,0.,0.));
#27380=DIRECTION('',(0.,0.,-1.));
#27381=DIRECTION('center_axis',(0.,0.,-1.));
#27382=DIRECTION('ref_axis',(1.,0.,0.));
#27383=DIRECTION('',(0.,0.,-1.));
#27384=DIRECTION('center_axis',(0.,0.,-1.));
#27385=DIRECTION('ref_axis',(1.,0.,0.));
#27386=DIRECTION('',(0.,0.,-1.));
#27387=DIRECTION('center_axis',(0.,0.,-1.));
#27388=DIRECTION('ref_axis',(0.938009462242609,-0.346609648947243,0.));
#27389=DIRECTION('',(0.,0.,-1.));
#27390=DIRECTION('center_axis',(0.,0.,-1.));
#27391=DIRECTION('ref_axis',(1.,0.,0.));
#27392=DIRECTION('center_axis',(0.,0.,-1.));
#27393=DIRECTION('ref_axis',(1.,-9.39183297226423E-14,0.));
#27394=DIRECTION('',(1.22464679914735E-16,-1.15166757854366E-29,-1.));
#27395=DIRECTION('center_axis',(0.,0.,1.));
#27396=DIRECTION('ref_axis',(1.,-9.39183297226423E-14,0.));
#27397=DIRECTION('center_axis',(0.,0.,-1.));
#27398=DIRECTION('ref_axis',(1.,-9.39183297226423E-14,0.));
#27399=DIRECTION('',(1.22464679914735E-16,-1.15166757854366E-29,-1.));
#27400=DIRECTION('center_axis',(0.,0.,-1.));
#27401=DIRECTION('ref_axis',(1.,-9.39183297226423E-14,0.));
#27402=DIRECTION('',(1.22464679914735E-16,-1.15166757854366E-29,-1.));
#27403=DIRECTION('center_axis',(0.,0.,-1.));
#27404=DIRECTION('ref_axis',(1.,-9.39183297226423E-14,0.));
#27405=DIRECTION('',(1.22464679914735E-16,-1.15166757854366E-29,-1.));
#27406=DIRECTION('center_axis',(0.,0.,-1.));
#27407=DIRECTION('ref_axis',(1.,-9.39183297226423E-14,0.));
#27408=DIRECTION('',(1.22464679914735E-16,-1.15166757854366E-29,-1.));
#27409=DIRECTION('center_axis',(0.,0.,-1.));
#27410=DIRECTION('ref_axis',(1.,-9.39183297226423E-14,0.));
#27411=DIRECTION('',(1.22464679914735E-16,-1.15166757854366E-29,-1.));
#27412=DIRECTION('center_axis',(0.,0.,-1.));
#27413=DIRECTION('ref_axis',(1.,-9.39183297226423E-14,0.));
#27414=DIRECTION('',(1.22464679914735E-16,-1.15166757854366E-29,-1.));
#27415=DIRECTION('center_axis',(0.,0.,-1.));
#27416=DIRECTION('ref_axis',(1.,-9.39183297226423E-14,0.));
#27417=DIRECTION('',(1.22464679914735E-16,-1.15166757854366E-29,-1.));
#27418=DIRECTION('center_axis',(0.,0.,-1.));
#27419=DIRECTION('ref_axis',(1.,-9.39183297226423E-14,0.));
#27420=DIRECTION('',(1.22464679914735E-16,-1.15166757854366E-29,-1.));
#27421=DIRECTION('center_axis',(0.,0.,-1.));
#27422=DIRECTION('ref_axis',(1.,-9.39183297226423E-14,0.));
#27423=DIRECTION('',(1.22464679914735E-16,-1.15166757854366E-29,-1.));
#27424=DIRECTION('center_axis',(0.,0.,-1.));
#27425=DIRECTION('ref_axis',(1.,-9.39183297226423E-14,0.));
#27426=DIRECTION('',(1.22464679914735E-16,-1.15166757854366E-29,-1.));
#27427=DIRECTION('center_axis',(0.,0.,-1.));
#27428=DIRECTION('ref_axis',(1.,-9.39183297226423E-14,0.));
#27429=DIRECTION('',(1.22464679914735E-16,-1.15166757854366E-29,-1.));
#27430=DIRECTION('center_axis',(0.,0.,-1.));
#27431=DIRECTION('ref_axis',(1.,-9.39183297226423E-14,0.));
#27432=DIRECTION('',(1.22464679914735E-16,-1.15166757854366E-29,-1.));
#27433=DIRECTION('center_axis',(0.,0.,-1.));
#27434=DIRECTION('ref_axis',(1.,-9.39183297226423E-14,0.));
#27435=DIRECTION('',(1.22464679914735E-16,-1.15166757854366E-29,-1.));
#27436=DIRECTION('center_axis',(0.,0.,-1.));
#27437=DIRECTION('ref_axis',(-0.609165547211943,-0.793043085897591,0.));
#27438=DIRECTION('',(1.22464679914735E-16,-1.15166757854366E-29,-1.));
#27439=DIRECTION('center_axis',(0.,0.,-1.));
#27440=DIRECTION('ref_axis',(1.,-9.39183297226423E-14,0.));
#27441=DIRECTION('center_axis',(0.,0.,-1.));
#27442=DIRECTION('ref_axis',(1.,0.,0.));
#27443=DIRECTION('',(0.,0.,-1.));
#27444=DIRECTION('center_axis',(0.,0.,1.));
#27445=DIRECTION('ref_axis',(1.,0.,0.));
#27446=DIRECTION('',(0.,0.,-1.));
#27447=DIRECTION('center_axis',(0.,0.,1.));
#27448=DIRECTION('ref_axis',(1.,0.,0.));
#27449=DIRECTION('center_axis',(0.,0.,1.));
#27450=DIRECTION('ref_axis',(1.,0.,0.));
#27451=DIRECTION('center_axis',(0.,0.,-1.));
#27452=DIRECTION('ref_axis',(1.,0.,0.));
#27453=DIRECTION('',(0.,0.,-1.));
#27454=DIRECTION('center_axis',(0.,0.,-1.));
#27455=DIRECTION('ref_axis',(1.,0.,0.));
#27456=DIRECTION('',(0.,0.,-1.));
#27457=DIRECTION('center_axis',(0.,0.,-1.));
#27458=DIRECTION('ref_axis',(1.,0.,0.));
#27459=DIRECTION('',(0.,0.,-1.));
#27460=DIRECTION('center_axis',(0.,0.,-1.));
#27461=DIRECTION('ref_axis',(1.,0.,0.));
#27462=DIRECTION('',(0.,0.,-1.));
#27463=DIRECTION('center_axis',(0.,0.,-1.));
#27464=DIRECTION('ref_axis',(1.,0.,0.));
#27465=DIRECTION('',(0.,0.,-1.));
#27466=DIRECTION('center_axis',(0.,0.,-1.));
#27467=DIRECTION('ref_axis',(1.,0.,0.));
#27468=DIRECTION('',(0.,0.,-1.));
#27469=DIRECTION('center_axis',(0.,0.,-1.));
#27470=DIRECTION('ref_axis',(1.,0.,0.));
#27471=DIRECTION('',(0.,0.,-1.));
#27472=DIRECTION('center_axis',(0.,0.,-1.));
#27473=DIRECTION('ref_axis',(1.,0.,0.));
#27474=DIRECTION('',(0.,0.,-1.));
#27475=DIRECTION('center_axis',(0.,0.,-1.));
#27476=DIRECTION('ref_axis',(1.,0.,0.));
#27477=DIRECTION('',(0.,0.,-1.));
#27478=DIRECTION('center_axis',(0.,0.,-1.));
#27479=DIRECTION('ref_axis',(1.,0.,0.));
#27480=DIRECTION('',(0.,0.,-1.));
#27481=DIRECTION('center_axis',(0.,0.,-1.));
#27482=DIRECTION('ref_axis',(1.,0.,0.));
#27483=DIRECTION('',(0.,0.,-1.));
#27484=DIRECTION('center_axis',(0.,0.,-1.));
#27485=DIRECTION('ref_axis',(1.,0.,0.));
#27486=DIRECTION('',(0.,0.,-1.));
#27487=DIRECTION('center_axis',(0.,0.,-1.));
#27488=DIRECTION('ref_axis',(1.,0.,0.));
#27489=DIRECTION('',(0.,0.,-1.));
#27490=DIRECTION('center_axis',(0.,0.,-1.));
#27491=DIRECTION('ref_axis',(0.93800946033191,-0.346609654118057,0.));
#27492=DIRECTION('',(0.,0.,-1.));
#27493=DIRECTION('center_axis',(0.,0.,-1.));
#27494=DIRECTION('ref_axis',(1.,0.,0.));
#27495=DIRECTION('center_axis',(0.,0.,-1.));
#27496=DIRECTION('ref_axis',(1.,-9.10285349619456E-14,0.));
#27497=DIRECTION('',(1.22464679914735E-16,-1.11627779950486E-29,-1.));
#27498=DIRECTION('center_axis',(0.,0.,1.));
#27499=DIRECTION('ref_axis',(1.,-9.10285349619456E-14,0.));
#27500=DIRECTION('center_axis',(0.,0.,-1.));
#27501=DIRECTION('ref_axis',(1.,-9.10285349619456E-14,0.));
#27502=DIRECTION('',(1.22464679914735E-16,-1.11627779950486E-29,-1.));
#27503=DIRECTION('center_axis',(0.,0.,-1.));
#27504=DIRECTION('ref_axis',(1.,-9.10285349619456E-14,0.));
#27505=DIRECTION('',(1.22464679914735E-16,-1.11627779950486E-29,-1.));
#27506=DIRECTION('center_axis',(0.,0.,-1.));
#27507=DIRECTION('ref_axis',(1.,-9.10285349619456E-14,0.));
#27508=DIRECTION('',(1.22464679914735E-16,-1.11627779950486E-29,-1.));
#27509=DIRECTION('center_axis',(0.,0.,-1.));
#27510=DIRECTION('ref_axis',(1.,-9.10285349619456E-14,0.));
#27511=DIRECTION('',(1.22464679914735E-16,-1.11627779950486E-29,-1.));
#27512=DIRECTION('center_axis',(0.,0.,-1.));
#27513=DIRECTION('ref_axis',(1.,-9.10285349619456E-14,0.));
#27514=DIRECTION('',(1.22464679914735E-16,-1.11627779950486E-29,-1.));
#27515=DIRECTION('center_axis',(0.,0.,-1.));
#27516=DIRECTION('ref_axis',(1.,-9.10285349619456E-14,0.));
#27517=DIRECTION('',(1.22464679914735E-16,-1.11627779950486E-29,-1.));
#27518=DIRECTION('center_axis',(0.,0.,-1.));
#27519=DIRECTION('ref_axis',(1.,-9.10285349619456E-14,0.));
#27520=DIRECTION('',(1.22464679914735E-16,-1.11627779950486E-29,-1.));
#27521=DIRECTION('center_axis',(0.,0.,-1.));
#27522=DIRECTION('ref_axis',(1.,-9.10285349619456E-14,0.));
#27523=DIRECTION('',(1.22464679914735E-16,-1.11627779950486E-29,-1.));
#27524=DIRECTION('center_axis',(0.,0.,-1.));
#27525=DIRECTION('ref_axis',(1.,-9.10285349619456E-14,0.));
#27526=DIRECTION('',(1.22464679914735E-16,-1.11627779950486E-29,-1.));
#27527=DIRECTION('center_axis',(0.,0.,-1.));
#27528=DIRECTION('ref_axis',(1.,-9.10285349619456E-14,0.));
#27529=DIRECTION('',(1.22464679914735E-16,-1.11627779950486E-29,-1.));
#27530=DIRECTION('center_axis',(0.,0.,-1.));
#27531=DIRECTION('ref_axis',(1.,-9.10285349619456E-14,0.));
#27532=DIRECTION('',(1.22464679914735E-16,-1.11627779950486E-29,-1.));
#27533=DIRECTION('center_axis',(0.,0.,-1.));
#27534=DIRECTION('ref_axis',(1.,-9.10285349619456E-14,0.));
#27535=DIRECTION('',(1.22464679914735E-16,-1.11627779950486E-29,-1.));
#27536=DIRECTION('center_axis',(0.,0.,-1.));
#27537=DIRECTION('ref_axis',(1.,-9.10285349619456E-14,0.));
#27538=DIRECTION('',(1.22464679914735E-16,-1.11627779950486E-29,-1.));
#27539=DIRECTION('center_axis',(0.,0.,-1.));
#27540=DIRECTION('ref_axis',(-0.609165548712575,-0.793043084744901,0.));
#27541=DIRECTION('',(1.22464679914735E-16,-1.11627779950486E-29,-1.));
#27542=DIRECTION('center_axis',(0.,0.,-1.));
#27543=DIRECTION('ref_axis',(1.,-9.10285349619456E-14,0.));
#27544=DIRECTION('center_axis',(0.,0.,-1.));
#27545=DIRECTION('ref_axis',(1.,0.,0.));
#27546=DIRECTION('',(0.,0.,-1.));
#27547=DIRECTION('center_axis',(0.,0.,1.));
#27548=DIRECTION('ref_axis',(1.,0.,0.));
#27549=DIRECTION('',(0.,0.,-1.));
#27550=DIRECTION('center_axis',(0.,0.,1.));
#27551=DIRECTION('ref_axis',(1.,0.,0.));
#27552=DIRECTION('center_axis',(0.,0.,1.));
#27553=DIRECTION('ref_axis',(1.,0.,0.));
#27554=DIRECTION('center_axis',(0.,0.,-1.));
#27555=DIRECTION('ref_axis',(1.,0.,0.));
#27556=DIRECTION('',(0.,0.,-1.));
#27557=DIRECTION('center_axis',(0.,0.,-1.));
#27558=DIRECTION('ref_axis',(1.,0.,0.));
#27559=DIRECTION('',(0.,0.,-1.));
#27560=DIRECTION('center_axis',(0.,0.,-1.));
#27561=DIRECTION('ref_axis',(1.,0.,0.));
#27562=DIRECTION('',(0.,0.,-1.));
#27563=DIRECTION('center_axis',(0.,0.,-1.));
#27564=DIRECTION('ref_axis',(1.,0.,0.));
#27565=DIRECTION('',(0.,0.,-1.));
#27566=DIRECTION('center_axis',(0.,0.,-1.));
#27567=DIRECTION('ref_axis',(1.,0.,0.));
#27568=DIRECTION('',(0.,0.,-1.));
#27569=DIRECTION('center_axis',(0.,0.,-1.));
#27570=DIRECTION('ref_axis',(1.,0.,0.));
#27571=DIRECTION('',(0.,0.,-1.));
#27572=DIRECTION('center_axis',(0.,0.,-1.));
#27573=DIRECTION('ref_axis',(1.,0.,0.));
#27574=DIRECTION('',(0.,0.,-1.));
#27575=DIRECTION('center_axis',(0.,0.,-1.));
#27576=DIRECTION('ref_axis',(1.,0.,0.));
#27577=DIRECTION('',(0.,0.,-1.));
#27578=DIRECTION('center_axis',(0.,0.,-1.));
#27579=DIRECTION('ref_axis',(1.,0.,0.));
#27580=DIRECTION('',(0.,0.,-1.));
#27581=DIRECTION('center_axis',(0.,0.,-1.));
#27582=DIRECTION('ref_axis',(1.,0.,0.));
#27583=DIRECTION('',(0.,0.,-1.));
#27584=DIRECTION('center_axis',(0.,0.,-1.));
#27585=DIRECTION('ref_axis',(1.,0.,0.));
#27586=DIRECTION('',(0.,0.,-1.));
#27587=DIRECTION('center_axis',(0.,0.,-1.));
#27588=DIRECTION('ref_axis',(1.,0.,0.));
#27589=DIRECTION('',(0.,0.,-1.));
#27590=DIRECTION('center_axis',(0.,0.,-1.));
#27591=DIRECTION('ref_axis',(1.,0.,0.));
#27592=DIRECTION('',(0.,0.,-1.));
#27593=DIRECTION('center_axis',(0.,0.,-1.));
#27594=DIRECTION('ref_axis',(0.938009461339291,-0.34660965139184,0.));
#27595=DIRECTION('',(0.,0.,-1.));
#27596=DIRECTION('center_axis',(0.,0.,-1.));
#27597=DIRECTION('ref_axis',(1.,0.,0.));
#27598=DIRECTION('center_axis',(0.,0.,-1.));
#27599=DIRECTION('ref_axis',(1.,-1.09812200906474E-13,0.));
#27600=DIRECTION('',(1.22464679914735E-16,-1.34631136325705E-29,-1.));
#27601=DIRECTION('center_axis',(0.,0.,1.));
#27602=DIRECTION('ref_axis',(1.,-1.09812200906474E-13,0.));
#27603=DIRECTION('center_axis',(0.,0.,-1.));
#27604=DIRECTION('ref_axis',(1.,-1.09812200906474E-13,0.));
#27605=DIRECTION('',(1.22464679914735E-16,-1.34631136325705E-29,-1.));
#27606=DIRECTION('center_axis',(0.,0.,-1.));
#27607=DIRECTION('ref_axis',(1.,-1.09812200906474E-13,0.));
#27608=DIRECTION('',(1.22464679914735E-16,-1.34631136325705E-29,-1.));
#27609=DIRECTION('center_axis',(0.,0.,-1.));
#27610=DIRECTION('ref_axis',(1.,-1.09812200906474E-13,0.));
#27611=DIRECTION('',(1.22464679914735E-16,-1.34631136325705E-29,-1.));
#27612=DIRECTION('center_axis',(0.,0.,-1.));
#27613=DIRECTION('ref_axis',(1.,-1.09812200906474E-13,0.));
#27614=DIRECTION('',(1.22464679914735E-16,-1.34631136325705E-29,-1.));
#27615=DIRECTION('center_axis',(0.,0.,-1.));
#27616=DIRECTION('ref_axis',(1.,-1.09812200906474E-13,0.));
#27617=DIRECTION('',(1.22464679914735E-16,-1.34631136325705E-29,-1.));
#27618=DIRECTION('center_axis',(0.,0.,-1.));
#27619=DIRECTION('ref_axis',(1.,-1.09812200906474E-13,0.));
#27620=DIRECTION('',(1.22464679914735E-16,-1.34631136325705E-29,-1.));
#27621=DIRECTION('center_axis',(0.,0.,-1.));
#27622=DIRECTION('ref_axis',(1.,-1.09812200906474E-13,0.));
#27623=DIRECTION('',(1.22464679914735E-16,-1.34631136325705E-29,-1.));
#27624=DIRECTION('center_axis',(0.,0.,-1.));
#27625=DIRECTION('ref_axis',(1.,-1.09812200906474E-13,0.));
#27626=DIRECTION('',(1.22464679914735E-16,-1.34631136325705E-29,-1.));
#27627=DIRECTION('center_axis',(0.,0.,-1.));
#27628=DIRECTION('ref_axis',(1.,-1.09812200906474E-13,0.));
#27629=DIRECTION('',(1.22464679914735E-16,-1.34631136325705E-29,-1.));
#27630=DIRECTION('center_axis',(0.,0.,-1.));
#27631=DIRECTION('ref_axis',(1.,-1.09812200906474E-13,0.));
#27632=DIRECTION('',(1.22464679914735E-16,-1.34631136325705E-29,-1.));
#27633=DIRECTION('center_axis',(0.,0.,-1.));
#27634=DIRECTION('ref_axis',(1.,-1.09812200906474E-13,0.));
#27635=DIRECTION('',(1.22464679914735E-16,-1.34631136325705E-29,-1.));
#27636=DIRECTION('center_axis',(0.,0.,-1.));
#27637=DIRECTION('ref_axis',(1.,-1.09812200906474E-13,0.));
#27638=DIRECTION('',(1.22464679914735E-16,-1.34631136325705E-29,-1.));
#27639=DIRECTION('center_axis',(0.,0.,-1.));
#27640=DIRECTION('ref_axis',(1.,-1.09812200906474E-13,0.));
#27641=DIRECTION('',(1.22464679914735E-16,-1.34631136325705E-29,-1.));
#27642=DIRECTION('center_axis',(0.,0.,-1.));
#27643=DIRECTION('ref_axis',(-0.609165549363982,-0.793043084244531,0.));
#27644=DIRECTION('',(1.22464679914735E-16,-1.34631136325705E-29,-1.));
#27645=DIRECTION('center_axis',(0.,0.,-1.));
#27646=DIRECTION('ref_axis',(1.,-1.09812200906474E-13,0.));
#27647=DIRECTION('center_axis',(0.,0.,-1.));
#27648=DIRECTION('ref_axis',(1.,0.,0.));
#27649=DIRECTION('',(0.,0.,-1.));
#27650=DIRECTION('center_axis',(0.,0.,1.));
#27651=DIRECTION('ref_axis',(1.,0.,0.));
#27652=DIRECTION('',(0.,0.,-1.));
#27653=DIRECTION('center_axis',(0.,0.,1.));
#27654=DIRECTION('ref_axis',(1.,0.,0.));
#27655=DIRECTION('center_axis',(0.,0.,1.));
#27656=DIRECTION('ref_axis',(1.,0.,0.));
#27657=DIRECTION('center_axis',(0.,0.,-1.));
#27658=DIRECTION('ref_axis',(1.,0.,0.));
#27659=DIRECTION('',(0.,0.,-1.));
#27660=DIRECTION('center_axis',(0.,0.,-1.));
#27661=DIRECTION('ref_axis',(1.,0.,0.));
#27662=DIRECTION('',(0.,0.,-1.));
#27663=DIRECTION('center_axis',(0.,0.,-1.));
#27664=DIRECTION('ref_axis',(1.,0.,0.));
#27665=DIRECTION('',(0.,0.,-1.));
#27666=DIRECTION('center_axis',(0.,0.,-1.));
#27667=DIRECTION('ref_axis',(1.,0.,0.));
#27668=DIRECTION('',(0.,0.,-1.));
#27669=DIRECTION('center_axis',(0.,0.,-1.));
#27670=DIRECTION('ref_axis',(1.,0.,0.));
#27671=DIRECTION('',(0.,0.,-1.));
#27672=DIRECTION('center_axis',(0.,0.,-1.));
#27673=DIRECTION('ref_axis',(1.,0.,0.));
#27674=DIRECTION('',(0.,0.,-1.));
#27675=DIRECTION('center_axis',(0.,0.,-1.));
#27676=DIRECTION('ref_axis',(1.,0.,0.));
#27677=DIRECTION('',(0.,0.,-1.));
#27678=DIRECTION('center_axis',(0.,0.,-1.));
#27679=DIRECTION('ref_axis',(1.,0.,0.));
#27680=DIRECTION('',(0.,0.,-1.));
#27681=DIRECTION('center_axis',(0.,0.,-1.));
#27682=DIRECTION('ref_axis',(1.,0.,0.));
#27683=DIRECTION('',(0.,0.,-1.));
#27684=DIRECTION('center_axis',(0.,0.,-1.));
#27685=DIRECTION('ref_axis',(1.,0.,0.));
#27686=DIRECTION('',(0.,0.,-1.));
#27687=DIRECTION('center_axis',(0.,0.,-1.));
#27688=DIRECTION('ref_axis',(1.,0.,0.));
#27689=DIRECTION('',(0.,0.,-1.));
#27690=DIRECTION('center_axis',(0.,0.,-1.));
#27691=DIRECTION('ref_axis',(1.,0.,0.));
#27692=DIRECTION('',(0.,0.,-1.));
#27693=DIRECTION('center_axis',(0.,0.,-1.));
#27694=DIRECTION('ref_axis',(1.,0.,0.));
#27695=DIRECTION('',(0.,0.,-1.));
#27696=DIRECTION('center_axis',(0.,0.,-1.));
#27697=DIRECTION('ref_axis',(0.938009461339277,-0.346609651391878,0.));
#27698=DIRECTION('',(0.,0.,-1.));
#27699=DIRECTION('center_axis',(0.,0.,-1.));
#27700=DIRECTION('ref_axis',(1.,0.,0.));
#27701=DIRECTION('center_axis',(0.,0.,-1.));
#27702=DIRECTION('ref_axis',(1.,-9.39183297226423E-14,0.));
#27703=DIRECTION('',(1.22464679914735E-16,-1.15166757854366E-29,-1.));
#27704=DIRECTION('center_axis',(0.,0.,1.));
#27705=DIRECTION('ref_axis',(1.,-9.39183297226423E-14,0.));
#27706=DIRECTION('center_axis',(0.,0.,-1.));
#27707=DIRECTION('ref_axis',(1.,-9.39183297226423E-14,0.));
#27708=DIRECTION('',(1.22464679914735E-16,-1.15166757854366E-29,-1.));
#27709=DIRECTION('center_axis',(0.,0.,-1.));
#27710=DIRECTION('ref_axis',(1.,-9.39183297226423E-14,0.));
#27711=DIRECTION('',(1.22464679914735E-16,-1.15166757854366E-29,-1.));
#27712=DIRECTION('center_axis',(0.,0.,-1.));
#27713=DIRECTION('ref_axis',(1.,-9.39183297226423E-14,0.));
#27714=DIRECTION('',(1.22464679914735E-16,-1.15166757854366E-29,-1.));
#27715=DIRECTION('center_axis',(0.,0.,-1.));
#27716=DIRECTION('ref_axis',(1.,-9.39183297226423E-14,0.));
#27717=DIRECTION('',(1.22464679914735E-16,-1.15166757854366E-29,-1.));
#27718=DIRECTION('center_axis',(0.,0.,-1.));
#27719=DIRECTION('ref_axis',(1.,-9.39183297226423E-14,0.));
#27720=DIRECTION('',(1.22464679914735E-16,-1.15166757854366E-29,-1.));
#27721=DIRECTION('center_axis',(0.,0.,-1.));
#27722=DIRECTION('ref_axis',(1.,-9.39183297226423E-14,0.));
#27723=DIRECTION('',(1.22464679914735E-16,-1.15166757854366E-29,-1.));
#27724=DIRECTION('center_axis',(0.,0.,-1.));
#27725=DIRECTION('ref_axis',(1.,-9.39183297226423E-14,0.));
#27726=DIRECTION('',(1.22464679914735E-16,-1.15166757854366E-29,-1.));
#27727=DIRECTION('center_axis',(0.,0.,-1.));
#27728=DIRECTION('ref_axis',(1.,-9.39183297226423E-14,0.));
#27729=DIRECTION('',(1.22464679914735E-16,-1.15166757854366E-29,-1.));
#27730=DIRECTION('center_axis',(0.,0.,-1.));
#27731=DIRECTION('ref_axis',(1.,-9.39183297226423E-14,0.));
#27732=DIRECTION('',(1.22464679914735E-16,-1.15166757854366E-29,-1.));
#27733=DIRECTION('center_axis',(0.,0.,-1.));
#27734=DIRECTION('ref_axis',(1.,-9.39183297226423E-14,0.));
#27735=DIRECTION('',(1.22464679914735E-16,-1.15166757854366E-29,-1.));
#27736=DIRECTION('center_axis',(0.,0.,-1.));
#27737=DIRECTION('ref_axis',(1.,-9.39183297226423E-14,0.));
#27738=DIRECTION('',(1.22464679914735E-16,-1.15166757854366E-29,-1.));
#27739=DIRECTION('center_axis',(0.,0.,-1.));
#27740=DIRECTION('ref_axis',(1.,-9.39183297226423E-14,0.));
#27741=DIRECTION('',(1.22464679914735E-16,-1.15166757854366E-29,-1.));
#27742=DIRECTION('center_axis',(0.,0.,-1.));
#27743=DIRECTION('ref_axis',(1.,-9.39183297226423E-14,0.));
#27744=DIRECTION('',(1.22464679914735E-16,-1.15166757854366E-29,-1.));
#27745=DIRECTION('center_axis',(0.,0.,-1.));
#27746=DIRECTION('ref_axis',(-0.609165549364011,-0.793043084244508,0.));
#27747=DIRECTION('',(1.22464679914735E-16,-1.15166757854366E-29,-1.));
#27748=DIRECTION('center_axis',(0.,0.,-1.));
#27749=DIRECTION('ref_axis',(1.,-9.39183297226423E-14,0.));
#27750=DIRECTION('center_axis',(0.,0.,-1.));
#27751=DIRECTION('ref_axis',(1.,0.,0.));
#27752=DIRECTION('',(0.,0.,-1.));
#27753=DIRECTION('center_axis',(0.,0.,1.));
#27754=DIRECTION('ref_axis',(1.,0.,0.));
#27755=DIRECTION('',(0.,0.,-1.));
#27756=DIRECTION('center_axis',(0.,0.,1.));
#27757=DIRECTION('ref_axis',(1.,0.,0.));
#27758=DIRECTION('center_axis',(0.,0.,1.));
#27759=DIRECTION('ref_axis',(1.,0.,0.));
#27760=DIRECTION('center_axis',(0.,0.,-1.));
#27761=DIRECTION('ref_axis',(1.,0.,0.));
#27762=DIRECTION('',(0.,0.,-1.));
#27763=DIRECTION('center_axis',(0.,0.,-1.));
#27764=DIRECTION('ref_axis',(1.,0.,0.));
#27765=DIRECTION('',(0.,0.,-1.));
#27766=DIRECTION('center_axis',(0.,0.,-1.));
#27767=DIRECTION('ref_axis',(1.,0.,0.));
#27768=DIRECTION('',(0.,0.,-1.));
#27769=DIRECTION('center_axis',(0.,0.,-1.));
#27770=DIRECTION('ref_axis',(1.,0.,0.));
#27771=DIRECTION('',(0.,0.,-1.));
#27772=DIRECTION('center_axis',(0.,0.,-1.));
#27773=DIRECTION('ref_axis',(1.,0.,0.));
#27774=DIRECTION('',(0.,0.,-1.));
#27775=DIRECTION('center_axis',(0.,0.,-1.));
#27776=DIRECTION('ref_axis',(1.,0.,0.));
#27777=DIRECTION('',(0.,0.,-1.));
#27778=DIRECTION('center_axis',(0.,0.,-1.));
#27779=DIRECTION('ref_axis',(1.,0.,0.));
#27780=DIRECTION('',(0.,0.,-1.));
#27781=DIRECTION('center_axis',(0.,0.,-1.));
#27782=DIRECTION('ref_axis',(1.,0.,0.));
#27783=DIRECTION('',(0.,0.,-1.));
#27784=DIRECTION('center_axis',(0.,0.,-1.));
#27785=DIRECTION('ref_axis',(1.,0.,0.));
#27786=DIRECTION('',(0.,0.,-1.));
#27787=DIRECTION('center_axis',(0.,0.,-1.));
#27788=DIRECTION('ref_axis',(1.,0.,0.));
#27789=DIRECTION('',(0.,0.,-1.));
#27790=DIRECTION('center_axis',(0.,0.,-1.));
#27791=DIRECTION('ref_axis',(1.,0.,0.));
#27792=DIRECTION('',(0.,0.,-1.));
#27793=DIRECTION('center_axis',(0.,0.,-1.));
#27794=DIRECTION('ref_axis',(1.,0.,0.));
#27795=DIRECTION('',(0.,0.,-1.));
#27796=DIRECTION('center_axis',(0.,0.,-1.));
#27797=DIRECTION('ref_axis',(1.,0.,0.));
#27798=DIRECTION('',(0.,0.,-1.));
#27799=DIRECTION('center_axis',(0.,0.,-1.));
#27800=DIRECTION('ref_axis',(0.938009463044599,-0.346609646776865,0.));
#27801=DIRECTION('',(0.,0.,-1.));
#27802=DIRECTION('center_axis',(0.,0.,-1.));
#27803=DIRECTION('ref_axis',(1.,0.,0.));
#27804=DIRECTION('center_axis',(0.,0.,-1.));
#27805=DIRECTION('ref_axis',(1.,-7.51346637781136E-14,0.));
#27806=DIRECTION('',(1.22464679914735E-16,-9.21634014791456E-30,-1.));
#27807=DIRECTION('center_axis',(0.,0.,1.));
#27808=DIRECTION('ref_axis',(1.,-7.51346637781136E-14,0.));
#27809=DIRECTION('center_axis',(0.,0.,-1.));
#27810=DIRECTION('ref_axis',(1.,-7.51346637781136E-14,0.));
#27811=DIRECTION('',(1.22464679914735E-16,-9.21634014791456E-30,-1.));
#27812=DIRECTION('center_axis',(0.,0.,-1.));
#27813=DIRECTION('ref_axis',(1.,-7.51346637781136E-14,0.));
#27814=DIRECTION('',(1.22464679914735E-16,-9.21634014791456E-30,-1.));
#27815=DIRECTION('center_axis',(0.,0.,-1.));
#27816=DIRECTION('ref_axis',(1.,-7.51346637781136E-14,0.));
#27817=DIRECTION('',(1.22464679914735E-16,-9.21634014791456E-30,-1.));
#27818=DIRECTION('center_axis',(0.,0.,-1.));
#27819=DIRECTION('ref_axis',(1.,-7.51346637781136E-14,0.));
#27820=DIRECTION('',(1.22464679914735E-16,-9.21634014791456E-30,-1.));
#27821=DIRECTION('center_axis',(0.,0.,-1.));
#27822=DIRECTION('ref_axis',(1.,-7.51346637781136E-14,0.));
#27823=DIRECTION('',(1.22464679914735E-16,-9.21634014791456E-30,-1.));
#27824=DIRECTION('center_axis',(0.,0.,-1.));
#27825=DIRECTION('ref_axis',(1.,-7.51346637781136E-14,0.));
#27826=DIRECTION('',(1.22464679914735E-16,-9.21634014791456E-30,-1.));
#27827=DIRECTION('center_axis',(0.,0.,-1.));
#27828=DIRECTION('ref_axis',(1.,-7.51346637781136E-14,0.));
#27829=DIRECTION('',(1.22464679914735E-16,-9.21634014791456E-30,-1.));
#27830=DIRECTION('center_axis',(0.,0.,-1.));
#27831=DIRECTION('ref_axis',(1.,-7.51346637781136E-14,0.));
#27832=DIRECTION('',(1.22464679914735E-16,-9.21634014791456E-30,-1.));
#27833=DIRECTION('center_axis',(0.,0.,-1.));
#27834=DIRECTION('ref_axis',(1.,-7.51346637781136E-14,0.));
#27835=DIRECTION('',(1.22464679914735E-16,-9.21634014791456E-30,-1.));
#27836=DIRECTION('center_axis',(0.,0.,-1.));
#27837=DIRECTION('ref_axis',(1.,-7.51346637781136E-14,0.));
#27838=DIRECTION('',(1.22464679914735E-16,-9.21634014791456E-30,-1.));
#27839=DIRECTION('center_axis',(0.,0.,-1.));
#27840=DIRECTION('ref_axis',(1.,-7.51346637781136E-14,0.));
#27841=DIRECTION('',(1.22464679914735E-16,-9.21634014791456E-30,-1.));
#27842=DIRECTION('center_axis',(0.,0.,-1.));
#27843=DIRECTION('ref_axis',(1.,-7.51346637781136E-14,0.));
#27844=DIRECTION('',(1.22464679914735E-16,-9.21634014791456E-30,-1.));
#27845=DIRECTION('center_axis',(0.,0.,-1.));
#27846=DIRECTION('ref_axis',(1.,-7.51346637781136E-14,0.));
#27847=DIRECTION('',(1.22464679914735E-16,-9.21634014791456E-30,-1.));
#27848=DIRECTION('center_axis',(0.,0.,-1.));
#27849=DIRECTION('ref_axis',(-0.609165547992927,-0.793043085297689,0.));
#27850=DIRECTION('',(1.22464679914735E-16,-9.21634014791456E-30,-1.));
#27851=DIRECTION('center_axis',(0.,0.,-1.));
#27852=DIRECTION('ref_axis',(1.,-7.51346637781136E-14,0.));
#27853=DIRECTION('center_axis',(0.,0.,-1.));
#27854=DIRECTION('ref_axis',(1.,0.,0.));
#27855=DIRECTION('',(0.,0.,-1.));
#27856=DIRECTION('center_axis',(0.,0.,1.));
#27857=DIRECTION('ref_axis',(1.,0.,0.));
#27858=DIRECTION('',(0.,0.,-1.));
#27859=DIRECTION('center_axis',(0.,0.,1.));
#27860=DIRECTION('ref_axis',(1.,0.,0.));
#27861=DIRECTION('center_axis',(0.,0.,1.));
#27862=DIRECTION('ref_axis',(1.,0.,0.));
#27863=DIRECTION('center_axis',(0.,0.,-1.));
#27864=DIRECTION('ref_axis',(1.,0.,0.));
#27865=DIRECTION('',(0.,0.,-1.));
#27866=DIRECTION('center_axis',(0.,0.,-1.));
#27867=DIRECTION('ref_axis',(1.,0.,0.));
#27868=DIRECTION('',(0.,0.,-1.));
#27869=DIRECTION('center_axis',(0.,0.,-1.));
#27870=DIRECTION('ref_axis',(1.,0.,0.));
#27871=DIRECTION('',(0.,0.,-1.));
#27872=DIRECTION('center_axis',(0.,0.,-1.));
#27873=DIRECTION('ref_axis',(1.,0.,0.));
#27874=DIRECTION('',(0.,0.,-1.));
#27875=DIRECTION('center_axis',(0.,0.,-1.));
#27876=DIRECTION('ref_axis',(1.,0.,0.));
#27877=DIRECTION('',(0.,0.,-1.));
#27878=DIRECTION('center_axis',(0.,0.,-1.));
#27879=DIRECTION('ref_axis',(1.,0.,0.));
#27880=DIRECTION('',(0.,0.,-1.));
#27881=DIRECTION('center_axis',(0.,0.,-1.));
#27882=DIRECTION('ref_axis',(1.,0.,0.));
#27883=DIRECTION('',(0.,0.,-1.));
#27884=DIRECTION('center_axis',(0.,0.,-1.));
#27885=DIRECTION('ref_axis',(1.,0.,0.));
#27886=DIRECTION('',(0.,0.,-1.));
#27887=DIRECTION('center_axis',(0.,0.,-1.));
#27888=DIRECTION('ref_axis',(1.,0.,0.));
#27889=DIRECTION('',(0.,0.,-1.));
#27890=DIRECTION('center_axis',(0.,0.,-1.));
#27891=DIRECTION('ref_axis',(1.,0.,0.));
#27892=DIRECTION('',(0.,0.,-1.));
#27893=DIRECTION('center_axis',(0.,0.,-1.));
#27894=DIRECTION('ref_axis',(1.,0.,0.));
#27895=DIRECTION('',(0.,0.,-1.));
#27896=DIRECTION('center_axis',(0.,0.,-1.));
#27897=DIRECTION('ref_axis',(1.,0.,0.));
#27898=DIRECTION('',(0.,0.,-1.));
#27899=DIRECTION('center_axis',(0.,0.,-1.));
#27900=DIRECTION('ref_axis',(1.,0.,0.));
#27901=DIRECTION('',(0.,0.,-1.));
#27902=DIRECTION('center_axis',(0.,0.,-1.));
#27903=DIRECTION('ref_axis',(0.938009463044576,-0.346609646776926,0.));
#27904=DIRECTION('',(0.,0.,-1.));
#27905=DIRECTION('center_axis',(0.,0.,-1.));
#27906=DIRECTION('ref_axis',(1.,0.,0.));
#27907=DIRECTION('center_axis',(0.,0.,-1.));
#27908=DIRECTION('ref_axis',(1.,-9.39183297226423E-14,0.));
#27909=DIRECTION('',(1.22464679914735E-16,-1.15166757854366E-29,-1.));
#27910=DIRECTION('center_axis',(0.,0.,1.));
#27911=DIRECTION('ref_axis',(1.,-9.39183297226423E-14,0.));
#27912=DIRECTION('center_axis',(0.,0.,-1.));
#27913=DIRECTION('ref_axis',(1.,-9.39183297226423E-14,0.));
#27914=DIRECTION('',(1.22464679914735E-16,-1.15166757854366E-29,-1.));
#27915=DIRECTION('center_axis',(0.,0.,-1.));
#27916=DIRECTION('ref_axis',(1.,-9.39183297226423E-14,0.));
#27917=DIRECTION('',(1.22464679914735E-16,-1.15166757854366E-29,-1.));
#27918=DIRECTION('center_axis',(0.,0.,-1.));
#27919=DIRECTION('ref_axis',(1.,-9.39183297226423E-14,0.));
#27920=DIRECTION('',(1.22464679914735E-16,-1.15166757854366E-29,-1.));
#27921=DIRECTION('center_axis',(0.,0.,-1.));
#27922=DIRECTION('ref_axis',(1.,-9.39183297226423E-14,0.));
#27923=DIRECTION('',(1.22464679914735E-16,-1.15166757854366E-29,-1.));
#27924=DIRECTION('center_axis',(0.,0.,-1.));
#27925=DIRECTION('ref_axis',(1.,-9.39183297226423E-14,0.));
#27926=DIRECTION('',(1.22464679914735E-16,-1.15166757854366E-29,-1.));
#27927=DIRECTION('center_axis',(0.,0.,-1.));
#27928=DIRECTION('ref_axis',(1.,-9.39183297226423E-14,0.));
#27929=DIRECTION('',(1.22464679914735E-16,-1.15166757854366E-29,-1.));
#27930=DIRECTION('center_axis',(0.,0.,-1.));
#27931=DIRECTION('ref_axis',(1.,-9.39183297226423E-14,0.));
#27932=DIRECTION('',(1.22464679914735E-16,-1.15166757854366E-29,-1.));
#27933=DIRECTION('center_axis',(0.,0.,-1.));
#27934=DIRECTION('ref_axis',(1.,-9.39183297226423E-14,0.));
#27935=DIRECTION('',(1.22464679914735E-16,-1.15166757854366E-29,-1.));
#27936=DIRECTION('center_axis',(0.,0.,-1.));
#27937=DIRECTION('ref_axis',(1.,-9.39183297226423E-14,0.));
#27938=DIRECTION('',(1.22464679914735E-16,-1.15166757854366E-29,-1.));
#27939=DIRECTION('center_axis',(0.,0.,-1.));
#27940=DIRECTION('ref_axis',(1.,-9.39183297226423E-14,0.));
#27941=DIRECTION('',(1.22464679914735E-16,-1.15166757854366E-29,-1.));
#27942=DIRECTION('center_axis',(0.,0.,-1.));
#27943=DIRECTION('ref_axis',(1.,-9.39183297226423E-14,0.));
#27944=DIRECTION('',(1.22464679914735E-16,-1.15166757854366E-29,-1.));
#27945=DIRECTION('center_axis',(0.,0.,-1.));
#27946=DIRECTION('ref_axis',(1.,-9.39183297226423E-14,0.));
#27947=DIRECTION('',(1.22464679914735E-16,-1.15166757854366E-29,-1.));
#27948=DIRECTION('center_axis',(0.,0.,-1.));
#27949=DIRECTION('ref_axis',(1.,-9.39183297226423E-14,0.));
#27950=DIRECTION('',(1.22464679914735E-16,-1.15166757854366E-29,-1.));
#27951=DIRECTION('center_axis',(0.,0.,-1.));
#27952=DIRECTION('ref_axis',(-0.609165547992994,-0.793043085297637,0.));
#27953=DIRECTION('',(1.22464679914735E-16,-1.15166757854366E-29,-1.));
#27954=DIRECTION('center_axis',(0.,0.,-1.));
#27955=DIRECTION('ref_axis',(1.,-9.39183297226423E-14,0.));
#27956=DIRECTION('center_axis',(0.,0.,-1.));
#27957=DIRECTION('ref_axis',(1.,0.,0.));
#27958=DIRECTION('',(0.,0.,-1.));
#27959=DIRECTION('center_axis',(0.,0.,1.));
#27960=DIRECTION('ref_axis',(1.,0.,0.));
#27961=DIRECTION('',(0.,0.,-1.));
#27962=DIRECTION('center_axis',(0.,0.,1.));
#27963=DIRECTION('ref_axis',(1.,0.,0.));
#27964=DIRECTION('center_axis',(0.,0.,1.));
#27965=DIRECTION('ref_axis',(1.,0.,0.));
#27966=DIRECTION('center_axis',(0.,0.,-1.));
#27967=DIRECTION('ref_axis',(1.,0.,0.));
#27968=DIRECTION('',(0.,0.,-1.));
#27969=DIRECTION('center_axis',(0.,0.,-1.));
#27970=DIRECTION('ref_axis',(1.,0.,0.));
#27971=DIRECTION('',(0.,0.,-1.));
#27972=DIRECTION('center_axis',(0.,0.,-1.));
#27973=DIRECTION('ref_axis',(1.,0.,0.));
#27974=DIRECTION('',(0.,0.,-1.));
#27975=DIRECTION('center_axis',(0.,0.,-1.));
#27976=DIRECTION('ref_axis',(1.,0.,0.));
#27977=DIRECTION('',(0.,0.,-1.));
#27978=DIRECTION('center_axis',(0.,0.,-1.));
#27979=DIRECTION('ref_axis',(1.,0.,0.));
#27980=DIRECTION('',(0.,0.,-1.));
#27981=DIRECTION('center_axis',(0.,0.,-1.));
#27982=DIRECTION('ref_axis',(1.,0.,0.));
#27983=DIRECTION('',(0.,0.,-1.));
#27984=DIRECTION('center_axis',(0.,0.,-1.));
#27985=DIRECTION('ref_axis',(1.,0.,0.));
#27986=DIRECTION('',(0.,0.,-1.));
#27987=DIRECTION('center_axis',(0.,0.,-1.));
#27988=DIRECTION('ref_axis',(1.,0.,0.));
#27989=DIRECTION('',(0.,0.,-1.));
#27990=DIRECTION('center_axis',(0.,0.,-1.));
#27991=DIRECTION('ref_axis',(1.,0.,0.));
#27992=DIRECTION('',(0.,0.,-1.));
#27993=DIRECTION('center_axis',(0.,0.,-1.));
#27994=DIRECTION('ref_axis',(1.,0.,0.));
#27995=DIRECTION('',(0.,0.,-1.));
#27996=DIRECTION('center_axis',(0.,0.,-1.));
#27997=DIRECTION('ref_axis',(1.,0.,0.));
#27998=DIRECTION('',(0.,0.,-1.));
#27999=DIRECTION('center_axis',(0.,0.,-1.));
#28000=DIRECTION('ref_axis',(1.,0.,0.));
#28001=DIRECTION('',(0.,0.,-1.));
#28002=DIRECTION('center_axis',(0.,0.,-1.));
#28003=DIRECTION('ref_axis',(1.,0.,0.));
#28004=DIRECTION('',(0.,0.,-1.));
#28005=DIRECTION('center_axis',(0.,0.,-1.));
#28006=DIRECTION('ref_axis',(0.938009460331926,-0.346609654118015,0.));
#28007=DIRECTION('',(0.,0.,-1.));
#28008=DIRECTION('center_axis',(0.,0.,-1.));
#28009=DIRECTION('ref_axis',(1.,0.,0.));
#28010=DIRECTION('center_axis',(0.,0.,-1.));
#28011=DIRECTION('ref_axis',(1.,-8.66938428209003E-14,0.));
#28012=DIRECTION('',(1.22464679914735E-16,-1.06319313094666E-29,-1.));
#28013=DIRECTION('center_axis',(0.,0.,1.));
#28014=DIRECTION('ref_axis',(1.,-8.66938428209003E-14,0.));
#28015=DIRECTION('center_axis',(0.,0.,-1.));
#28016=DIRECTION('ref_axis',(1.,-8.66938428209003E-14,0.));
#28017=DIRECTION('',(1.22464679914735E-16,-1.06319313094666E-29,-1.));
#28018=DIRECTION('center_axis',(0.,0.,-1.));
#28019=DIRECTION('ref_axis',(1.,-8.66938428209003E-14,0.));
#28020=DIRECTION('',(1.22464679914735E-16,-1.06319313094666E-29,-1.));
#28021=DIRECTION('center_axis',(0.,0.,-1.));
#28022=DIRECTION('ref_axis',(1.,-8.66938428209003E-14,0.));
#28023=DIRECTION('',(1.22464679914735E-16,-1.06319313094666E-29,-1.));
#28024=DIRECTION('center_axis',(0.,0.,-1.));
#28025=DIRECTION('ref_axis',(1.,-8.66938428209003E-14,0.));
#28026=DIRECTION('',(1.22464679914735E-16,-1.06319313094666E-29,-1.));
#28027=DIRECTION('center_axis',(0.,0.,-1.));
#28028=DIRECTION('ref_axis',(1.,-8.66938428209003E-14,0.));
#28029=DIRECTION('',(1.22464679914735E-16,-1.06319313094666E-29,-1.));
#28030=DIRECTION('center_axis',(0.,0.,-1.));
#28031=DIRECTION('ref_axis',(1.,-8.66938428209003E-14,0.));
#28032=DIRECTION('',(1.22464679914735E-16,-1.06319313094666E-29,-1.));
#28033=DIRECTION('center_axis',(0.,0.,-1.));
#28034=DIRECTION('ref_axis',(1.,-8.66938428209003E-14,0.));
#28035=DIRECTION('',(1.22464679914735E-16,-1.06319313094666E-29,-1.));
#28036=DIRECTION('center_axis',(0.,0.,-1.));
#28037=DIRECTION('ref_axis',(1.,-8.66938428209003E-14,0.));
#28038=DIRECTION('',(1.22464679914735E-16,-1.06319313094666E-29,-1.));
#28039=DIRECTION('center_axis',(0.,0.,-1.));
#28040=DIRECTION('ref_axis',(1.,-8.66938428209003E-14,0.));
#28041=DIRECTION('',(1.22464679914735E-16,-1.06319313094666E-29,-1.));
#28042=DIRECTION('center_axis',(0.,0.,-1.));
#28043=DIRECTION('ref_axis',(1.,-8.66938428209003E-14,0.));
#28044=DIRECTION('',(1.22464679914735E-16,-1.06319313094666E-29,-1.));
#28045=DIRECTION('center_axis',(0.,0.,-1.));
#28046=DIRECTION('ref_axis',(1.,-8.66938428209003E-14,0.));
#28047=DIRECTION('',(1.22464679914735E-16,-1.06319313094666E-29,-1.));
#28048=DIRECTION('center_axis',(0.,0.,-1.));
#28049=DIRECTION('ref_axis',(1.,-8.66938428209003E-14,0.));
#28050=DIRECTION('',(1.22464679914735E-16,-1.06319313094666E-29,-1.));
#28051=DIRECTION('center_axis',(0.,0.,-1.));
#28052=DIRECTION('ref_axis',(1.,-8.66938428209003E-14,0.));
#28053=DIRECTION('',(1.22464679914735E-16,-1.06319313094666E-29,-1.));
#28054=DIRECTION('center_axis',(0.,0.,-1.));
#28055=DIRECTION('ref_axis',(-0.60916554871253,-0.793043084744935,0.));
#28056=DIRECTION('',(1.22464679914735E-16,-1.06319313094666E-29,-1.));
#28057=DIRECTION('center_axis',(0.,0.,-1.));
#28058=DIRECTION('ref_axis',(1.,-8.66938428209003E-14,0.));
#28059=DIRECTION('center_axis',(0.,0.,-1.));
#28060=DIRECTION('ref_axis',(1.,0.,0.));
#28061=DIRECTION('',(0.,0.,-1.));
#28062=DIRECTION('center_axis',(0.,0.,1.));
#28063=DIRECTION('ref_axis',(1.,0.,0.));
#28064=DIRECTION('',(0.,0.,-1.));
#28065=DIRECTION('center_axis',(0.,0.,1.));
#28066=DIRECTION('ref_axis',(1.,0.,0.));
#28067=DIRECTION('center_axis',(0.,0.,1.));
#28068=DIRECTION('ref_axis',(1.,0.,0.));
#28069=DIRECTION('center_axis',(0.,0.,-1.));
#28070=DIRECTION('ref_axis',(1.,0.,0.));
#28071=DIRECTION('',(0.,0.,-1.));
#28072=DIRECTION('center_axis',(0.,0.,-1.));
#28073=DIRECTION('ref_axis',(1.,0.,0.));
#28074=DIRECTION('',(0.,0.,-1.));
#28075=DIRECTION('center_axis',(0.,0.,-1.));
#28076=DIRECTION('ref_axis',(1.,0.,0.));
#28077=DIRECTION('',(0.,0.,-1.));
#28078=DIRECTION('center_axis',(0.,0.,-1.));
#28079=DIRECTION('ref_axis',(1.,0.,0.));
#28080=DIRECTION('',(0.,0.,-1.));
#28081=DIRECTION('center_axis',(0.,0.,-1.));
#28082=DIRECTION('ref_axis',(1.,0.,0.));
#28083=DIRECTION('',(0.,0.,-1.));
#28084=DIRECTION('center_axis',(0.,0.,-1.));
#28085=DIRECTION('ref_axis',(1.,0.,0.));
#28086=DIRECTION('',(0.,0.,-1.));
#28087=DIRECTION('center_axis',(0.,0.,-1.));
#28088=DIRECTION('ref_axis',(1.,0.,0.));
#28089=DIRECTION('',(0.,0.,-1.));
#28090=DIRECTION('center_axis',(0.,0.,-1.));
#28091=DIRECTION('ref_axis',(1.,0.,0.));
#28092=DIRECTION('',(0.,0.,-1.));
#28093=DIRECTION('center_axis',(0.,0.,-1.));
#28094=DIRECTION('ref_axis',(1.,0.,0.));
#28095=DIRECTION('',(0.,0.,-1.));
#28096=DIRECTION('center_axis',(0.,0.,-1.));
#28097=DIRECTION('ref_axis',(1.,0.,0.));
#28098=DIRECTION('',(0.,0.,-1.));
#28099=DIRECTION('center_axis',(0.,0.,-1.));
#28100=DIRECTION('ref_axis',(1.,0.,0.));
#28101=DIRECTION('',(0.,0.,-1.));
#28102=DIRECTION('center_axis',(0.,0.,-1.));
#28103=DIRECTION('ref_axis',(1.,0.,0.));
#28104=DIRECTION('',(0.,0.,-1.));
#28105=DIRECTION('center_axis',(0.,0.,-1.));
#28106=DIRECTION('ref_axis',(1.,0.,0.));
#28107=DIRECTION('',(0.,0.,-1.));
#28108=DIRECTION('center_axis',(0.,0.,-1.));
#28109=DIRECTION('ref_axis',(0.938009462242626,-0.346609648947198,0.));
#28110=DIRECTION('',(0.,0.,-1.));
#28111=DIRECTION('center_axis',(0.,0.,-1.));
#28112=DIRECTION('ref_axis',(1.,0.,0.));
#28113=DIRECTION('center_axis',(0.,0.,-1.));
#28114=DIRECTION('ref_axis',(1.,-9.82530218636872E-14,0.));
#28115=DIRECTION('',(1.22464679914735E-16,-1.20475224710186E-29,-1.));
#28116=DIRECTION('center_axis',(0.,0.,1.));
#28117=DIRECTION('ref_axis',(1.,-9.82530218636872E-14,0.));
#28118=DIRECTION('center_axis',(0.,0.,-1.));
#28119=DIRECTION('ref_axis',(1.,-9.82530218636872E-14,0.));
#28120=DIRECTION('',(1.22464679914735E-16,-1.20475224710186E-29,-1.));
#28121=DIRECTION('center_axis',(0.,0.,-1.));
#28122=DIRECTION('ref_axis',(1.,-9.82530218636872E-14,0.));
#28123=DIRECTION('',(1.22464679914735E-16,-1.20475224710186E-29,-1.));
#28124=DIRECTION('center_axis',(0.,0.,-1.));
#28125=DIRECTION('ref_axis',(1.,-9.82530218636872E-14,0.));
#28126=DIRECTION('',(1.22464679914735E-16,-1.20475224710186E-29,-1.));
#28127=DIRECTION('center_axis',(0.,0.,-1.));
#28128=DIRECTION('ref_axis',(1.,-9.82530218636872E-14,0.));
#28129=DIRECTION('',(1.22464679914735E-16,-1.20475224710186E-29,-1.));
#28130=DIRECTION('center_axis',(0.,0.,-1.));
#28131=DIRECTION('ref_axis',(1.,-9.82530218636872E-14,0.));
#28132=DIRECTION('',(1.22464679914735E-16,-1.20475224710186E-29,-1.));
#28133=DIRECTION('center_axis',(0.,0.,-1.));
#28134=DIRECTION('ref_axis',(1.,-9.82530218636872E-14,0.));
#28135=DIRECTION('',(1.22464679914735E-16,-1.20475224710186E-29,-1.));
#28136=DIRECTION('center_axis',(0.,0.,-1.));
#28137=DIRECTION('ref_axis',(1.,-9.82530218636872E-14,0.));
#28138=DIRECTION('',(1.22464679914735E-16,-1.20475224710186E-29,-1.));
#28139=DIRECTION('center_axis',(0.,0.,-1.));
#28140=DIRECTION('ref_axis',(1.,-9.82530218636872E-14,0.));
#28141=DIRECTION('',(1.22464679914735E-16,-1.20475224710186E-29,-1.));
#28142=DIRECTION('center_axis',(0.,0.,-1.));
#28143=DIRECTION('ref_axis',(1.,-9.82530218636872E-14,0.));
#28144=DIRECTION('',(1.22464679914735E-16,-1.20475224710186E-29,-1.));
#28145=DIRECTION('center_axis',(0.,0.,-1.));
#28146=DIRECTION('ref_axis',(1.,-9.82530218636872E-14,0.));
#28147=DIRECTION('',(1.22464679914735E-16,-1.20475224710186E-29,-1.));
#28148=DIRECTION('center_axis',(0.,0.,-1.));
#28149=DIRECTION('ref_axis',(1.,-9.82530218636872E-14,0.));
#28150=DIRECTION('',(1.22464679914735E-16,-1.20475224710186E-29,-1.));
#28151=DIRECTION('center_axis',(0.,0.,-1.));
#28152=DIRECTION('ref_axis',(1.,-9.82530218636872E-14,0.));
#28153=DIRECTION('',(1.22464679914735E-16,-1.20475224710186E-29,-1.));
#28154=DIRECTION('center_axis',(0.,0.,-1.));
#28155=DIRECTION('ref_axis',(1.,-9.82530218636872E-14,0.));
#28156=DIRECTION('',(1.22464679914735E-16,-1.20475224710186E-29,-1.));
#28157=DIRECTION('center_axis',(0.,0.,-1.));
#28158=DIRECTION('ref_axis',(-0.609165547211898,-0.793043085897626,0.));
#28159=DIRECTION('',(1.22464679914735E-16,-1.20475224710186E-29,-1.));
#28160=DIRECTION('center_axis',(0.,0.,-1.));
#28161=DIRECTION('ref_axis',(1.,-9.82530218636872E-14,0.));
#28162=DIRECTION('center_axis',(0.,1.,0.));
#28163=DIRECTION('ref_axis',(0.,0.,-1.));
#28164=DIRECTION('',(0.,1.,0.));
#28165=DIRECTION('center_axis',(0.,-1.,0.));
#28166=DIRECTION('ref_axis',(0.,0.,1.));
#28167=DIRECTION('',(0.,-1.,0.));
#28168=DIRECTION('center_axis',(1.,0.,0.));
#28169=DIRECTION('ref_axis',(0.,-1.,0.));
#28170=DIRECTION('',(1.,0.,0.));
#28171=DIRECTION('center_axis',(-1.,0.,0.));
#28172=DIRECTION('ref_axis',(0.,1.,0.));
#28173=DIRECTION('',(-1.,0.,0.));
#28174=DIRECTION('center_axis',(0.,1.,0.));
#28175=DIRECTION('ref_axis',(0.,0.,-1.));
#28176=DIRECTION('',(0.,1.,0.));
#28177=DIRECTION('center_axis',(0.,-1.,0.));
#28178=DIRECTION('ref_axis',(0.,0.,1.));
#28179=DIRECTION('',(0.,-1.,0.));
#28180=DIRECTION('center_axis',(1.,0.,0.));
#28181=DIRECTION('ref_axis',(0.,-1.,0.));
#28182=DIRECTION('',(1.,0.,0.));
#28183=DIRECTION('center_axis',(-1.,0.,0.));
#28184=DIRECTION('ref_axis',(0.,1.,0.));
#28185=DIRECTION('',(-1.,0.,0.));
#28186=DIRECTION('center_axis',(0.,1.,0.));
#28187=DIRECTION('ref_axis',(0.,0.,-1.));
#28188=DIRECTION('',(0.,1.,0.));
#28189=DIRECTION('center_axis',(0.,-1.,0.));
#28190=DIRECTION('ref_axis',(0.,0.,1.));
#28191=DIRECTION('',(0.,-1.,0.));
#28192=DIRECTION('center_axis',(1.,0.,0.));
#28193=DIRECTION('ref_axis',(0.,-1.,0.));
#28194=DIRECTION('',(1.,0.,0.));
#28195=DIRECTION('center_axis',(-1.,0.,0.));
#28196=DIRECTION('ref_axis',(0.,1.,0.));
#28197=DIRECTION('',(-1.,0.,0.));
#28198=DIRECTION('center_axis',(0.,0.,1.));
#28199=DIRECTION('ref_axis',(1.,0.,0.));
#28200=DIRECTION('center_axis',(0.,0.,-1.));
#28201=DIRECTION('ref_axis',(1.,-9.82530218636872E-14,0.));
#28202=DIRECTION('center_axis',(0.,0.,-1.));
#28203=DIRECTION('ref_axis',(1.,0.,0.));
#28204=DIRECTION('center_axis',(0.,0.,1.));
#28205=DIRECTION('ref_axis',(1.,0.,0.));
#28206=DIRECTION('center_axis',(0.,0.,-1.));
#28207=DIRECTION('ref_axis',(1.,-8.66938428209003E-14,0.));
#28208=DIRECTION('center_axis',(0.,0.,-1.));
#28209=DIRECTION('ref_axis',(1.,0.,0.));
#28210=DIRECTION('center_axis',(0.,0.,1.));
#28211=DIRECTION('ref_axis',(1.,0.,0.));
#28212=DIRECTION('center_axis',(0.,0.,-1.));
#28213=DIRECTION('ref_axis',(1.,-9.39183297226423E-14,0.));
#28214=DIRECTION('center_axis',(0.,0.,-1.));
#28215=DIRECTION('ref_axis',(1.,0.,0.));
#28216=DIRECTION('center_axis',(0.,0.,1.));
#28217=DIRECTION('ref_axis',(1.,0.,0.));
#28218=DIRECTION('center_axis',(0.,0.,-1.));
#28219=DIRECTION('ref_axis',(1.,-7.51346637781136E-14,0.));
#28220=DIRECTION('center_axis',(0.,0.,-1.));
#28221=DIRECTION('ref_axis',(1.,0.,0.));
#28222=DIRECTION('center_axis',(0.,0.,1.));
#28223=DIRECTION('ref_axis',(1.,0.,0.));
#28224=DIRECTION('center_axis',(0.,0.,-1.));
#28225=DIRECTION('ref_axis',(1.,-9.39183297226423E-14,0.));
#28226=DIRECTION('center_axis',(0.,0.,-1.));
#28227=DIRECTION('ref_axis',(1.,0.,0.));
#28228=DIRECTION('center_axis',(0.,0.,1.));
#28229=DIRECTION('ref_axis',(1.,0.,0.));
#28230=DIRECTION('center_axis',(0.,0.,-1.));
#28231=DIRECTION('ref_axis',(1.,-1.09812200906474E-13,0.));
#28232=DIRECTION('center_axis',(0.,0.,-1.));
#28233=DIRECTION('ref_axis',(1.,0.,0.));
#28234=DIRECTION('center_axis',(0.,0.,1.));
#28235=DIRECTION('ref_axis',(1.,0.,0.));
#28236=DIRECTION('center_axis',(0.,0.,-1.));
#28237=DIRECTION('ref_axis',(1.,-9.10285349619456E-14,0.));
#28238=DIRECTION('center_axis',(0.,0.,-1.));
#28239=DIRECTION('ref_axis',(1.,0.,0.));
#28240=DIRECTION('center_axis',(0.,0.,1.));
#28241=DIRECTION('ref_axis',(1.,0.,0.));
#28242=DIRECTION('center_axis',(0.,0.,-1.));
#28243=DIRECTION('ref_axis',(1.,-9.39183297226423E-14,0.));
#28244=DIRECTION('center_axis',(0.,0.,-1.));
#28245=DIRECTION('ref_axis',(1.,0.,0.));
#28246=DIRECTION('center_axis',(0.,0.,-1.));
#28247=DIRECTION('ref_axis',(1.,0.,0.));
#28248=DIRECTION('center_axis',(0.,0.,-1.));
#28249=DIRECTION('ref_axis',(1.,0.,0.));
#28250=DIRECTION('center_axis',(0.,0.,-1.));
#28251=DIRECTION('ref_axis',(1.,0.,0.));
#28252=DIRECTION('center_axis',(0.,0.,-1.));
#28253=DIRECTION('ref_axis',(1.,0.,0.));
#28254=DIRECTION('center_axis',(0.,0.,-1.));
#28255=DIRECTION('ref_axis',(1.,0.,0.));
#28256=DIRECTION('center_axis',(0.,0.,-1.));
#28257=DIRECTION('ref_axis',(1.,0.,0.));
#28258=DIRECTION('center_axis',(0.,0.,-1.));
#28259=DIRECTION('ref_axis',(1.,0.,0.));
#28260=DIRECTION('center_axis',(0.,0.,-1.));
#28261=DIRECTION('ref_axis',(1.,0.,0.));
#28262=DIRECTION('center_axis',(0.,0.,-1.));
#28263=DIRECTION('ref_axis',(1.,0.,0.));
#28264=DIRECTION('center_axis',(0.,0.,-1.));
#28265=DIRECTION('ref_axis',(1.,0.,0.));
#28266=DIRECTION('',(0.,0.,-1.));
#28267=DIRECTION('center_axis',(0.,0.,1.));
#28268=DIRECTION('ref_axis',(1.,0.,0.));
#28269=DIRECTION('center_axis',(0.,0.,-1.));
#28270=DIRECTION('ref_axis',(1.,0.,0.));
#28271=DIRECTION('center_axis',(0.,0.,-1.));
#28272=DIRECTION('ref_axis',(1.,0.,0.));
#28273=DIRECTION('',(0.,0.,-1.));
#28274=DIRECTION('center_axis',(0.,0.,1.));
#28275=DIRECTION('ref_axis',(1.,0.,0.));
#28276=DIRECTION('center_axis',(0.,0.,-1.));
#28277=DIRECTION('ref_axis',(1.,0.,0.));
#28278=DIRECTION('center_axis',(0.,0.,-1.));
#28279=DIRECTION('ref_axis',(1.,0.,0.));
#28280=DIRECTION('',(0.,0.,-1.));
#28281=DIRECTION('center_axis',(0.,0.,1.));
#28282=DIRECTION('ref_axis',(1.,0.,0.));
#28283=DIRECTION('center_axis',(0.,0.,-1.));
#28284=DIRECTION('ref_axis',(1.,0.,0.));
#28285=DIRECTION('center_axis',(0.,0.,-1.));
#28286=DIRECTION('ref_axis',(1.,0.,0.));
#28287=DIRECTION('',(0.,0.,-1.));
#28288=DIRECTION('center_axis',(0.,0.,1.));
#28289=DIRECTION('ref_axis',(1.,0.,0.));
#28290=DIRECTION('center_axis',(0.,0.,-1.));
#28291=DIRECTION('ref_axis',(1.,0.,0.));
#28292=DIRECTION('center_axis',(0.,0.,-1.));
#28293=DIRECTION('ref_axis',(1.,0.,0.));
#28294=DIRECTION('',(0.,0.,-1.));
#28295=DIRECTION('center_axis',(0.,0.,-1.));
#28296=DIRECTION('ref_axis',(1.,0.,0.));
#28297=DIRECTION('center_axis',(0.,0.,-1.));
#28298=DIRECTION('ref_axis',(1.,0.,0.));
#28299=DIRECTION('center_axis',(0.,0.,1.));
#28300=DIRECTION('ref_axis',(1.,0.,0.));
#28301=DIRECTION('center_axis',(0.,0.,1.));
#28302=DIRECTION('ref_axis',(1.,0.,0.));
#28303=DIRECTION('center_axis',(0.,0.,-1.));
#28304=DIRECTION('ref_axis',(1.,0.,0.));
#28305=DIRECTION('',(0.,0.,-1.));
#28306=DIRECTION('',(0.,0.,-1.));
#28307=DIRECTION('',(0.,0.,-1.));
#28308=DIRECTION('',(0.,0.,-1.));
#28309=DIRECTION('center_axis',(0.,0.,1.));
#28310=DIRECTION('ref_axis',(1.,0.,0.));
#28311=DIRECTION('center_axis',(0.,0.,1.));
#28312=DIRECTION('ref_axis',(1.,0.,0.));
#28313=DIRECTION('center_axis',(0.,0.,1.));
#28314=DIRECTION('ref_axis',(1.,0.,0.));
#28315=DIRECTION('',(0.,0.,-1.));
#28316=DIRECTION('',(0.,0.,-1.));
#28317=DIRECTION('',(0.,0.,-1.));
#28318=DIRECTION('',(0.,0.,-1.));
#28319=DIRECTION('center_axis',(0.,0.,-1.));
#28320=DIRECTION('ref_axis',(1.,0.,0.));
#28321=DIRECTION('center_axis',(0.,0.,1.));
#28322=DIRECTION('ref_axis',(1.,0.,0.));
#28323=DIRECTION('center_axis',(0.,0.,1.));
#28324=DIRECTION('ref_axis',(1.,0.,0.));
#28325=DIRECTION('center_axis',(0.,0.,-1.));
#28326=DIRECTION('ref_axis',(1.,0.,0.));
#28327=DIRECTION('center_axis',(0.,0.,1.));
#28328=DIRECTION('ref_axis',(1.,0.,0.));
#28329=DIRECTION('',(0.,0.,-1.));
#28330=DIRECTION('center_axis',(0.,0.,-1.));
#28331=DIRECTION('ref_axis',(1.,0.,0.));
#28332=DIRECTION('center_axis',(0.,0.,1.));
#28333=DIRECTION('ref_axis',(1.,0.,0.));
#28334=DIRECTION('',(0.,0.,-1.));
#28335=DIRECTION('center_axis',(0.,0.,-1.));
#28336=DIRECTION('ref_axis',(1.,0.,0.));
#28337=DIRECTION('center_axis',(0.,0.,1.));
#28338=DIRECTION('ref_axis',(1.,0.,0.));
#28339=DIRECTION('center_axis',(0.,0.,1.));
#28340=DIRECTION('ref_axis',(1.,0.,0.));
#32406=CARTESIAN_POINT('',(0.,0.,0.));
#32407=CARTESIAN_POINT('Origin',(-87.7685555885722,36.3549260746835,114.));
#32408=CARTESIAN_POINT('',(-90.2820657582583,36.3551835591638,107.387416697508));
#32409=CARTESIAN_POINT('',(-90.2841460151391,36.3513531397369,107.112583302492));
#32410=CARTESIAN_POINT('',(-90.2860555885722,36.3549260746835,114.));
#32411=CARTESIAN_POINT('',(-89.6820215852369,37.990913278059,107.));
#32412=CARTESIAN_POINT('Ctrl Pts',(-90.2841460151391,36.3513531397369,107.112583302492));
#32413=CARTESIAN_POINT('Ctrl Pts',(-90.2790007066056,36.9439878981613,107.075055534995));
#32414=CARTESIAN_POINT('Ctrl Pts',(-90.0677774166561,37.5397296349884,107.037527767497));
#32415=CARTESIAN_POINT('Ctrl Pts',(-89.6820215852368,37.9909132780591,107.));
#32416=CARTESIAN_POINT('',(-90.2860555885722,36.3549260746835,107.));
#32417=CARTESIAN_POINT('Origin',(-87.7685555885722,36.3549260746835,107.));
#32418=CARTESIAN_POINT('',(-90.2860555885722,36.3549260746835,106.));
#32419=CARTESIAN_POINT('',(-90.2860555885722,36.3549260746835,114.));
#32420=CARTESIAN_POINT('Origin',(-87.7685555885722,36.3549260746835,106.));
#32421=CARTESIAN_POINT('',(-85.8514453951333,37.9934539829853,107.));
#32422=CARTESIAN_POINT('Origin',(-87.7685555885722,36.3549260746835,107.));
#32423=CARTESIAN_POINT('Ctrl Pts',(-85.8514365495282,37.9934601500707,107.));
#32424=CARTESIAN_POINT('Ctrl Pts',(-86.3742571255242,38.6021753146346,107.050946273303));
#32425=CARTESIAN_POINT('Ctrl Pts',(-87.2139815880401,38.9423514879707,107.101892546605));
#32426=CARTESIAN_POINT('Ctrl Pts',(-88.0126524090168,38.8645886693614,107.152838819908));
#32427=CARTESIAN_POINT('Ctrl Pts',(-88.8380243712328,38.7842260863082,107.205488327639));
#32428=CARTESIAN_POINT('Ctrl Pts',(-89.6195517979231,38.2575123321297,107.25813783537));
#32429=CARTESIAN_POINT('Ctrl Pts',(-90.0034364012539,37.5227256169419,107.3107873431));
#32430=CARTESIAN_POINT('Ctrl Pts',(-90.1896795438024,37.1662409188007,107.336330461236));
#32431=CARTESIAN_POINT('Ctrl Pts',(-90.2823277522487,36.7607811758956,107.361873579372));
#32432=CARTESIAN_POINT('Ctrl Pts',(-90.2820657582583,36.3551835591638,107.387416697508));
#32433=CARTESIAN_POINT('Origin',(-87.7685555885722,36.3549260746835,114.));
#32434=CARTESIAN_POINT('',(-90.2873602755412,36.3528305926337,108.387416697508));
#32435=CARTESIAN_POINT('',(-90.2899626058712,36.3555923892882,108.112583302492));
#32436=CARTESIAN_POINT('',(-90.2860555885722,36.3549260746835,114.));
#32437=CARTESIAN_POINT('Ctrl Pts',(-90.2899626058712,36.3555923892882,108.112583302492));
#32438=CARTESIAN_POINT('Ctrl Pts',(-90.2900904417905,36.392049525674,108.110268755777));
#32439=CARTESIAN_POINT('Ctrl Pts',(-90.2893674908555,36.4285014253324,108.107954209062));
#32440=CARTESIAN_POINT('Ctrl Pts',(-90.2877778743739,36.4649154267611,108.105639662347));
#32441=CARTESIAN_POINT('Ctrl Pts',(-90.2516185155238,37.2932327976625,108.052990154616));
#32442=CARTESIAN_POINT('Ctrl Pts',(-89.7670151124418,38.1019402561809,108.000340646886));
#32443=CARTESIAN_POINT('Ctrl Pts',(-89.053640710259,38.5245019232063,107.947691139155));
#32444=CARTESIAN_POINT('Ctrl Pts',(-88.3402663080762,38.9470635902317,107.895041631424));
#32445=CARTESIAN_POINT('Ctrl Pts',(-87.3981209067927,38.9834794657641,107.842392123693));
#32446=CARTESIAN_POINT('Ctrl Pts',(-86.6543416914832,38.6170777740084,107.789742615962));
#32447=CARTESIAN_POINT('Ctrl Pts',(-85.9105624761737,38.2506760822528,107.737093108232));
#32448=CARTESIAN_POINT('Ctrl Pts',(-85.3651494468382,37.481456823209,107.684443600501));
#32449=CARTESIAN_POINT('Ctrl Pts',(-85.2652957945526,36.6584694678107,107.63179409277));
#32450=CARTESIAN_POINT('Ctrl Pts',(-85.1654421422671,35.8354821124124,107.579144585039));
#32451=CARTESIAN_POINT('Ctrl Pts',(-85.5111478670314,34.9587266606595,107.526495077308));
#32452=CARTESIAN_POINT('Ctrl Pts',(-86.145817826788,34.4249747642233,107.473845569577));
#32453=CARTESIAN_POINT('Ctrl Pts',(-86.7804877865446,33.891222867787,107.421196061847));
#32454=CARTESIAN_POINT('Ctrl Pts',(-87.7041219812935,33.7004745266674,107.368546554116));
#32455=CARTESIAN_POINT('Ctrl Pts',(-88.4977390142088,33.940628476657,107.315897046385));
#32456=CARTESIAN_POINT('Ctrl Pts',(-89.291356047124,34.1807824266467,107.263247538654));
#32457=CARTESIAN_POINT('Ctrl Pts',(-89.9549559182057,34.8518386677455,107.210598030923));
#32458=CARTESIAN_POINT('Ctrl Pts',(-90.1879211493143,35.6461245790433,107.157948523192));
#32459=CARTESIAN_POINT('Ctrl Pts',(-90.2548323106925,35.8742555861396,107.142826782959));
#32460=CARTESIAN_POINT('Ctrl Pts',(-90.2862193071108,36.1125521273703,107.127705042726));
#32461=CARTESIAN_POINT('Ctrl Pts',(-90.2841460151391,36.3513531397369,107.112583302492));
#32462=CARTESIAN_POINT('Ctrl Pts',(-90.2820657582583,36.3551835591638,107.387416697508));
#32463=CARTESIAN_POINT('Ctrl Pts',(-90.2817877299011,35.9247628501715,107.414523087103));
#32464=CARTESIAN_POINT('Ctrl Pts',(-90.1768790488432,35.4941868748242,107.441629476698));
#32465=CARTESIAN_POINT('Ctrl Pts',(-89.968158017258,35.1218194639909,107.468735866293));
#32466=CARTESIAN_POINT('Ctrl Pts',(-89.5627532499601,34.3985597024246,107.521385374024));
#32467=CARTESIAN_POINT('Ctrl Pts',(-88.765701935393,33.8948998554888,107.574034881755));
#32468=CARTESIAN_POINT('Ctrl Pts',(-87.9384522457069,33.8390488807469,107.626684389485));
#32469=CARTESIAN_POINT('Ctrl Pts',(-87.1112025560208,33.7831979060051,107.679333897216));
#32470=CARTESIAN_POINT('Ctrl Pts',(-86.2537544912156,34.1751558034572,107.731983404947));
#32471=CARTESIAN_POINT('Ctrl Pts',(-85.754762161375,34.8372915889621,107.784632912678));
#32472=CARTESIAN_POINT('Ctrl Pts',(-85.2557698315344,35.499427374467,107.837282420409));
#32473=CARTESIAN_POINT('Ctrl Pts',(-85.1152332366584,36.4317410480246,107.889931928139));
#32474=CARTESIAN_POINT('Ctrl Pts',(-85.3968901882336,37.2115545845095,107.94258143587));
#32475=CARTESIAN_POINT('Ctrl Pts',(-85.6785471398087,37.9913681209943,107.995230943601));
#32476=CARTESIAN_POINT('Ctrl Pts',(-86.3823976378351,38.6186815204063,108.047880451332));
#32477=CARTESIAN_POINT('Ctrl Pts',(-87.1893483010309,38.8091253099958,108.100529959063));
#32478=CARTESIAN_POINT('Ctrl Pts',(-87.9962989642267,38.9995690995853,108.153179466794));
#32479=CARTESIAN_POINT('Ctrl Pts',(-88.906349792592,38.7531432793523,108.205828974524));
#32480=CARTESIAN_POINT('Ctrl Pts',(-89.5069496277807,38.1815546745416,108.258478482255));
#32481=CARTESIAN_POINT('Ctrl Pts',(-89.9972376612814,37.7149493966099,108.30145788734));
#32482=CARTESIAN_POINT('Ctrl Pts',(-90.2813088913625,37.0316570454253,108.344437292424));
#32483=CARTESIAN_POINT('Ctrl Pts',(-90.2873602755412,36.3528305926337,108.387416697508));
#32484=CARTESIAN_POINT('Origin',(-87.7685555885722,36.3549260746835,114.));
#32485=CARTESIAN_POINT('',(-90.2882104573874,36.3567838325376,109.387416697508));
#32486=CARTESIAN_POINT('',(-90.2831163782917,36.3564540169858,109.112583302492));
#32487=CARTESIAN_POINT('',(-90.2860555885722,36.3549260746835,114.));
#32488=CARTESIAN_POINT('Ctrl Pts',(-90.2831163782917,36.3564540169858,109.112583302492));
#32489=CARTESIAN_POINT('Ctrl Pts',(-90.2848726336429,36.6697453384204,109.092832468829));
#32490=CARTESIAN_POINT('Ctrl Pts',(-90.2305754403938,36.982449840124,109.073081635165));
#32491=CARTESIAN_POINT('Ctrl Pts',(-90.1174358665212,37.2721760255534,109.053330801502));
#32492=CARTESIAN_POINT('Ctrl Pts',(-89.8158413631797,38.0444948703993,109.000681293771));
#32493=CARTESIAN_POINT('Ctrl Pts',(-89.0961200626589,38.6535325956426,108.94803178604));
#32494=CARTESIAN_POINT('Ctrl Pts',(-88.2845464797145,38.8231922589131,108.89538227831));
#32495=CARTESIAN_POINT('Ctrl Pts',(-87.47297289677,38.9928519221836,108.842732770579));
#32496=CARTESIAN_POINT('Ctrl Pts',(-86.5695470314019,38.7231335234814,108.790083262848));
#32497=CARTESIAN_POINT('Ctrl Pts',(-85.9838236566503,38.1363076402997,108.737433755117));
#32498=CARTESIAN_POINT('Ctrl Pts',(-85.3981002818987,37.549481757118,108.684784247386));
#32499=CARTESIAN_POINT('Ctrl Pts',(-85.1300793977636,36.6455483894568,108.632134739655));
#32500=CARTESIAN_POINT('Ctrl Pts',(-85.3012633835703,35.8342964195734,108.579485231925));
#32501=CARTESIAN_POINT('Ctrl Pts',(-85.472447369377,35.02304444969,108.526835724194));
#32502=CARTESIAN_POINT('Ctrl Pts',(-86.0828362251256,34.3044738775844,108.474186216463));
#32503=CARTESIAN_POINT('Ctrl Pts',(-86.8557211165975,34.0043286221669,108.421536708732));
#32504=CARTESIAN_POINT('Ctrl Pts',(-87.6286060080694,33.7041833667494,108.368887201001));
#32505=CARTESIAN_POINT('Ctrl Pts',(-88.5639869352647,33.8224634280202,108.316237693271));
#32506=CARTESIAN_POINT('Ctrl Pts',(-89.2378197415534,34.3055671002978,108.26358818554));
#32507=CARTESIAN_POINT('Ctrl Pts',(-89.8820299060469,34.7674328528715,108.213253224524));
#32508=CARTESIAN_POINT('Ctrl Pts',(-90.2871825297673,35.5627509543319,108.162918263508));
#32509=CARTESIAN_POINT('Ctrl Pts',(-90.2899626058712,36.3555923892882,108.112583302492));
#32510=CARTESIAN_POINT('Ctrl Pts',(-90.2873602755412,36.3528305926337,108.387416697508));
#32511=CARTESIAN_POINT('Ctrl Pts',(-90.2887217998816,36.2000988024933,108.397086800155));
#32512=CARTESIAN_POINT('Ctrl Pts',(-90.2760093365286,36.0475930861384,108.406756902801));
#32513=CARTESIAN_POINT('Ctrl Pts',(-90.248405070806,35.8978323082241,108.416427005448));
#32514=CARTESIAN_POINT('Ctrl Pts',(-90.0981118366304,35.0824499361056,108.469076513179));
#32515=CARTESIAN_POINT('Ctrl Pts',(-89.506376526267,34.3484365812571,108.521726020909));
#32516=CARTESIAN_POINT('Ctrl Pts',(-88.7414548919972,34.0285444819078,108.57437552864));
#32517=CARTESIAN_POINT('Ctrl Pts',(-87.9765332577274,33.7086523825585,108.627025036371));
#32518=CARTESIAN_POINT('Ctrl Pts',(-87.0384252995513,33.8028815387084,108.679674544102));
#32519=CARTESIAN_POINT('Ctrl Pts',(-86.3524072420719,34.2685153510835,108.732324051833));
#32520=CARTESIAN_POINT('Ctrl Pts',(-85.6663891845924,34.7341491634585,108.784973559563));
#32521=CARTESIAN_POINT('Ctrl Pts',(-85.2324610278097,35.5711876320587,108.837623067294));
#32522=CARTESIAN_POINT('Ctrl Pts',(-85.2473378688992,36.4001717283435,108.890272575025));
#32523=CARTESIAN_POINT('Ctrl Pts',(-85.2622147099887,37.2291558246283,108.942922082756));
#32524=CARTESIAN_POINT('Ctrl Pts',(-85.7258965489504,38.0500855485976,108.995571590487));
#32525=CARTESIAN_POINT('Ctrl Pts',(-86.4281800972607,38.4908050723096,109.048221098218));
#32526=CARTESIAN_POINT('Ctrl Pts',(-87.130463645571,38.9315245960216,109.100870605948));
#32527=CARTESIAN_POINT('Ctrl Pts',(-88.0713489032298,38.9920339194763,109.153520113679));
#32528=CARTESIAN_POINT('Ctrl Pts',(-88.824299933075,38.6449019741468,109.20616962141));
#32529=CARTESIAN_POINT('Ctrl Pts',(-89.5772509629203,38.2977700288173,109.258819129141));
#32530=CARTESIAN_POINT('Ctrl Pts',(-90.142267764952,37.5429968147038,109.311468636872));
#32531=CARTESIAN_POINT('Ctrl Pts',(-90.2632085219966,36.7227473329821,109.364118144603));
#32532=CARTESIAN_POINT('Ctrl Pts',(-90.2810481609466,36.6017545844628,109.371884328904));
#32533=CARTESIAN_POINT('Ctrl Pts',(-90.2892254201477,36.4793371777813,109.379650513206));
#32534=CARTESIAN_POINT('Ctrl Pts',(-90.2882104573874,36.3567838325376,109.387416697508));
#32535=CARTESIAN_POINT('Origin',(-87.7685555885722,36.3549260746835,114.));
#32536=CARTESIAN_POINT('',(-90.2821395661149,36.3552114620833,110.387416697508));
#32537=CARTESIAN_POINT('',(-90.284691711587,36.3528024297121,110.112583302492));
#32538=CARTESIAN_POINT('',(-90.2860555885722,36.3549260746835,114.));
#32539=CARTESIAN_POINT('Ctrl Pts',(-90.284691711587,36.3528024297121,110.112583302492));
#32540=CARTESIAN_POINT('Ctrl Pts',(-90.2798922469406,36.9417394945665,110.07539618188));
#32541=CARTESIAN_POINT('Ctrl Pts',(-90.0733337455156,37.5337101378598,110.038209061269));
#32542=CARTESIAN_POINT('Ctrl Pts',(-89.6956382082861,37.9812527577399,110.001021940657));
#32543=CARTESIAN_POINT('Ctrl Pts',(-89.1608970457506,38.6148833867763,109.948372432926));
#32544=CARTESIAN_POINT('Ctrl Pts',(-88.2831136976804,38.9590097330537,109.895722925195));
#32545=CARTESIAN_POINT('Ctrl Pts',(-87.4602178940962,38.8576273644157,109.843073417464));
#32546=CARTESIAN_POINT('Ctrl Pts',(-86.6373220905121,38.7562449957777,109.790423909734));
#32547=CARTESIAN_POINT('Ctrl Pts',(-85.869313831414,38.2093539122244,109.737774402003));
#32548=CARTESIAN_POINT('Ctrl Pts',(-85.5043579873302,37.4648788415031,109.685124894272));
#32549=CARTESIAN_POINT('Ctrl Pts',(-85.1394021432465,36.7204037707817,109.632475386541));
#32550=CARTESIAN_POINT('Ctrl Pts',(-85.177498714177,35.7783447128923,109.57982587881));
#32551=CARTESIAN_POINT('Ctrl Pts',(-85.6013771882749,35.0657698746485,109.52717637108));
#32552=CARTESIAN_POINT('Ctrl Pts',(-86.0252556623728,34.3531950364047,109.474526863349));
#32553=CARTESIAN_POINT('Ctrl Pts',(-86.8349160396379,33.8701044178065,109.421877355618));
#32554=CARTESIAN_POINT('Ctrl Pts',(-87.6633111224845,33.8354996839412,109.369227847887));
#32555=CARTESIAN_POINT('Ctrl Pts',(-88.491706205331,33.8008949500758,109.316578340156));
#32556=CARTESIAN_POINT('Ctrl Pts',(-89.338835993759,34.2147761009433,109.263928832425));
#32557=CARTESIAN_POINT('Ctrl Pts',(-89.8206670348919,34.8895166586012,109.211279324695));
#32558=CARTESIAN_POINT('Ctrl Pts',(-90.1217449188274,35.3111363592072,109.178380650627));
#32559=CARTESIAN_POINT('Ctrl Pts',(-90.2801910095015,35.8346092560125,109.145481976559));
#32560=CARTESIAN_POINT('Ctrl Pts',(-90.2831163782917,36.3564540169858,109.112583302492));
#32561=CARTESIAN_POINT('Ctrl Pts',(-90.2882104573874,36.3567838325376,109.387416697508));
#32562=CARTESIAN_POINT('Ctrl Pts',(-90.2823446550742,35.6485078995844,109.432300020937));
#32563=CARTESIAN_POINT('Ctrl Pts',(-89.9694528690476,34.935691533327,109.477183344366));
#32564=CARTESIAN_POINT('Ctrl Pts',(-89.4402911475608,34.4671003638404,109.522066667795));
#32565=CARTESIAN_POINT('Ctrl Pts',(-88.8195683040227,33.9174286257501,109.574716175526));
#32566=CARTESIAN_POINT('Ctrl Pts',(-87.9012579048889,33.7038108988991,109.627365683257));
#32567=CARTESIAN_POINT('Ctrl Pts',(-87.1016619950835,33.9230875413012,109.680015190987));
#32568=CARTESIAN_POINT('Ctrl Pts',(-86.3020660852782,34.1423641837033,109.732664698718));
#32569=CARTESIAN_POINT('Ctrl Pts',(-85.6211846648011,34.7945351953585,109.785314206449));
#32570=CARTESIAN_POINT('Ctrl Pts',(-85.3676849764274,35.5839487607172,109.83796371418));
#32571=CARTESIAN_POINT('Ctrl Pts',(-85.1141852880536,36.3733623260759,109.890613221911));
#32572=CARTESIAN_POINT('Ctrl Pts',(-85.2880673317831,37.3000184451381,109.943262729642));
#32573=CARTESIAN_POINT('Ctrl Pts',(-85.8105043249304,37.9438316601752,109.995912237372));
#32574=CARTESIAN_POINT('Ctrl Pts',(-86.3329413180777,38.5876448752124,110.048561745103));
#32575=CARTESIAN_POINT('Ctrl Pts',(-87.2039332606428,38.9486151862244,110.101211252834));
#32576=CARTESIAN_POINT('Ctrl Pts',(-88.0286292016189,38.8631021907732,110.153860760565));
#32577=CARTESIAN_POINT('Ctrl Pts',(-88.8533251425949,38.777589195322,110.206510268296));
#32578=CARTESIAN_POINT('Ctrl Pts',(-89.6317250819818,38.2455928934076,110.259159776027));
#32579=CARTESIAN_POINT('Ctrl Pts',(-90.0109532436846,37.5082857190933,110.311809283757));
#32580=CARTESIAN_POINT('Ctrl Pts',(-90.1924836559242,37.1553486516045,110.337011755008));
#32581=CARTESIAN_POINT('Ctrl Pts',(-90.2825485383685,36.7553670064009,110.362214226258));
#32582=CARTESIAN_POINT('Ctrl Pts',(-90.2821395661149,36.3552114620833,110.387416697508));
#32583=CARTESIAN_POINT('Origin',(-87.7685555885722,36.3549260746835,114.));
#32584=CARTESIAN_POINT('',(-90.2872022523859,36.3527998634328,111.387416697508));
#32585=CARTESIAN_POINT('',(-90.2900214059965,36.35548699916,111.112583302492));
#32586=CARTESIAN_POINT('',(-90.2860555885722,36.3549260746835,114.));
#32587=CARTESIAN_POINT('Ctrl Pts',(-90.2900214059965,36.35548699916,111.112583302492));
#32588=CARTESIAN_POINT('Ctrl Pts',(-90.2901161298337,36.3865769482408,111.110609402663));
#32589=CARTESIAN_POINT('Ctrl Pts',(-90.289590328231,36.4176636198089,111.108635502833));
#32590=CARTESIAN_POINT('Ctrl Pts',(-90.2884340218591,36.4487268212695,111.106661603004));
#32591=CARTESIAN_POINT('Ctrl Pts',(-90.2575920508711,37.2772705199817,111.054012095273));
#32592=CARTESIAN_POINT('Ctrl Pts',(-89.7781836309555,38.089116640287,111.001362587543));
#32593=CARTESIAN_POINT('Ctrl Pts',(-89.0675412790233,38.5162270890477,110.948713079812));
#32594=CARTESIAN_POINT('Ctrl Pts',(-88.3568989270911,38.9433375378084,110.896063572081));
#32595=CARTESIAN_POINT('Ctrl Pts',(-87.4150226431423,38.9857123150244,110.84341406435));
#32596=CARTESIAN_POINT('Ctrl Pts',(-86.6688977175355,38.6241414600135,110.790764556619));
#32597=CARTESIAN_POINT('Ctrl Pts',(-85.9227727919286,38.2625706050026,110.738115048888));
#32598=CARTESIAN_POINT('Ctrl Pts',(-85.3723992246636,37.4970541177647,110.685465541158));
#32599=CARTESIAN_POINT('Ctrl Pts',(-85.2672805031015,36.6746272563465,110.632816033427));
#32600=CARTESIAN_POINT('Ctrl Pts',(-85.1621617815393,35.8522003949283,110.580166525696));
#32601=CARTESIAN_POINT('Ctrl Pts',(-85.50229790568,34.9728631593298,110.527517017965));
#32602=CARTESIAN_POINT('Ctrl Pts',(-86.1334933358886,34.4352497141681,110.474867510234));
#32603=CARTESIAN_POINT('Ctrl Pts',(-86.7646887660972,33.8976362690064,110.422218002503));
#32604=CARTESIAN_POINT('Ctrl Pts',(-87.6869435023737,33.7017466142814,110.369568494773));
#32605=CARTESIAN_POINT('Ctrl Pts',(-88.4821673848742,33.9363843445116,110.316918987042));
#32606=CARTESIAN_POINT('Ctrl Pts',(-89.2773912673748,34.1710220747418,110.264269479311));
#32607=CARTESIAN_POINT('Ctrl Pts',(-89.9455842960992,34.8361871899272,110.21161997158));
#32608=CARTESIAN_POINT('Ctrl Pts',(-90.183831321961,35.6303372034176,110.158970463849));
#32609=CARTESIAN_POINT('Ctrl Pts',(-90.25380097415,35.8635673981236,110.14350807673));
#32610=CARTESIAN_POINT('Ctrl Pts',(-90.2866873267115,36.1079226773738,110.128045689611));
#32611=CARTESIAN_POINT('Ctrl Pts',(-90.284691711587,36.3528024297121,110.112583302492));
#32612=CARTESIAN_POINT('Ctrl Pts',(-90.2821395661149,36.3552114620833,110.387416697508));
#32613=CARTESIAN_POINT('Ctrl Pts',(-90.2816941702547,35.9194175387913,110.414863733989));
#32614=CARTESIAN_POINT('Ctrl Pts',(-90.1739418475738,35.4834173616642,110.442310770469));
#32615=CARTESIAN_POINT('Ctrl Pts',(-89.9601635310367,35.1077531359413,110.46975780695));
#32616=CARTESIAN_POINT('Ctrl Pts',(-89.5500892726676,34.3871457738176,110.522407314681));
#32617=CARTESIAN_POINT('Ctrl Pts',(-88.7498843719111,33.8885490962844,110.575056822411));
#32618=CARTESIAN_POINT('Ctrl Pts',(-87.9223095518277,33.8379943251671,110.627706330142));
#32619=CARTESIAN_POINT('Ctrl Pts',(-87.0947347317443,33.7874395540498,110.680355837873));
#32620=CARTESIAN_POINT('Ctrl Pts',(-86.2397899923339,34.1849266893484,110.733005345604));
#32621=CARTESIAN_POINT('Ctrl Pts',(-85.7450515302878,34.8502609827235,110.785654853335));
#32622=CARTESIAN_POINT('Ctrl Pts',(-85.2503130682416,35.5155952760986,110.838304361066));
#32623=CARTESIAN_POINT('Ctrl Pts',(-85.1157808835598,36.4487767275502,110.890953868796));
#32624=CARTESIAN_POINT('Ctrl Pts',(-85.4024430963309,37.2267617168094,110.943603376527));
#32625=CARTESIAN_POINT('Ctrl Pts',(-85.689105309102,38.0047467060685,110.996252884258));
#32626=CARTESIAN_POINT('Ctrl Pts',(-86.3969619193261,38.6275352331353,111.048902391989));
#32627=CARTESIAN_POINT('Ctrl Pts',(-87.205116897016,38.8127955898771,111.10155189972));
#32628=CARTESIAN_POINT('Ctrl Pts',(-88.0132718747059,38.9980559466188,111.154201407451));
#32629=CARTESIAN_POINT('Ctrl Pts',(-88.9217252198616,38.7457881330357,111.206850915181));
#32630=CARTESIAN_POINT('Ctrl Pts',(-89.5186434231292,38.1703539262337,111.259500422912));
#32631=CARTESIAN_POINT('Ctrl Pts',(-90.0020639151804,37.7043324749317,111.302139181111));
#32632=CARTESIAN_POINT('Ctrl Pts',(-90.2811565836147,37.0263545637827,111.344777939309));
#32633=CARTESIAN_POINT('Ctrl Pts',(-90.2872022523859,36.3527998634328,111.387416697508));
#32634=CARTESIAN_POINT('Origin',(-87.7685555885722,36.3549260746835,114.));
#32635=CARTESIAN_POINT('',(-90.2883544400146,36.356729971742,112.387416697508));
#32636=CARTESIAN_POINT('',(-90.2832192959692,36.3565168099065,112.112583302492));
#32637=CARTESIAN_POINT('',(-90.2860555885722,36.3549260746835,114.));
#32638=CARTESIAN_POINT('Ctrl Pts',(-90.2832192959692,36.3565168099065,112.112583302492));
#32639=CARTESIAN_POINT('Ctrl Pts',(-90.2850210486953,36.6643730370269,112.093173115714));
#32640=CARTESIAN_POINT('Ctrl Pts',(-90.2326348324987,36.9716374824648,112.073762928937));
#32641=CARTESIAN_POINT('Ctrl Pts',(-90.1232771295477,37.2570748224305,112.054352742159));
#32642=CARTESIAN_POINT('Ctrl Pts',(-89.8266478753891,38.0313144322456,112.001703234428));
#32643=CARTESIAN_POINT('Ctrl Pts',(-89.1108519400598,38.6449615091715,111.949053726697));
#32644=CARTESIAN_POINT('Ctrl Pts',(-88.3003845258671,38.8198284824987,111.896404218966));
#32645=CARTESIAN_POINT('Ctrl Pts',(-87.4899171116743,38.9946954558259,111.843754711236));
#32646=CARTESIAN_POINT('Ctrl Pts',(-86.584778218618,38.7307823255544,111.791105203505));
#32647=CARTESIAN_POINT('Ctrl Pts',(-85.9952987995873,38.1477300960177,111.738455695774));
#32648=CARTESIAN_POINT('Ctrl Pts',(-85.4058193805567,37.564677866481,111.685806188043));
#32649=CARTESIAN_POINT('Ctrl Pts',(-85.1319994355516,36.6624865376791,111.633156680312));
#32650=CARTESIAN_POINT('Ctrl Pts',(-85.2979710727125,35.8501508290649,111.580507172582));
#32651=CARTESIAN_POINT('Ctrl Pts',(-85.4639427098734,35.0378151204507,111.527857664851));
#32652=CARTESIAN_POINT('Ctrl Pts',(-86.0697059292002,34.3153350320242,111.47520815712));
#32653=CARTESIAN_POINT('Ctrl Pts',(-86.840647186937,34.0102359252646,111.422558649389));
#32654=CARTESIAN_POINT('Ctrl Pts',(-87.6115884446739,33.7051368185049,111.369909141658));
#32655=CARTESIAN_POINT('Ctrl Pts',(-88.5477077408209,33.8174186934119,111.317259633927));
#32656=CARTESIAN_POINT('Ctrl Pts',(-89.2246296278641,34.2961802694251,111.264610126197));
#32657=CARTESIAN_POINT('Ctrl Pts',(-89.876172816134,34.7569924393774,111.213934518295));
#32658=CARTESIAN_POINT('Ctrl Pts',(-90.2875895763982,35.5573198146224,111.163258910394));
#32659=CARTESIAN_POINT('Ctrl Pts',(-90.2900214059965,36.35548699916,111.112583302492));
#32660=CARTESIAN_POINT('Ctrl Pts',(-90.2872022523859,36.3527998634328,111.387416697508));
#32661=CARTESIAN_POINT('Ctrl Pts',(-90.2886216576026,36.1946623452147,111.39742744704));
#32662=CARTESIAN_POINT('Ctrl Pts',(-90.2749901963085,36.036768642733,111.407438196572));
#32663=CARTESIAN_POINT('Ctrl Pts',(-90.2454185361615,35.8819190433356,111.417448946105));
#32664=CARTESIAN_POINT('Ctrl Pts',(-90.0898923845469,35.0675189672606,111.470098453835));
#32665=CARTESIAN_POINT('Ctrl Pts',(-89.493457019938,34.3373194151317,111.522747961566));
#32666=CARTESIAN_POINT('Ctrl Pts',(-88.7264973449979,34.0223452499004,111.575397469297));
#32667=CARTESIAN_POINT('Ctrl Pts',(-87.9595376700576,33.7073710846691,111.628046977028));
#32668=CARTESIAN_POINT('Ctrl Pts',(-87.0220536847861,33.8076223063356,111.680696484759));
#32669=CARTESIAN_POINT('Ctrl Pts',(-86.3390394977637,34.277651548058,111.733345992489));
#32670=CARTESIAN_POINT('Ctrl Pts',(-85.6560253107413,34.7476807897803,111.78599550022));
#32671=CARTESIAN_POINT('Ctrl Pts',(-85.2274809219679,35.5874880515586,111.838645007951));
#32672=CARTESIAN_POINT('Ctrl Pts',(-85.2476804132995,36.4163594820577,111.891294515682));
#32673=CARTESIAN_POINT('Ctrl Pts',(-85.267879904631,37.2452309125568,111.943944023413));
#32674=CARTESIAN_POINT('Ctrl Pts',(-85.7368232760675,38.0631665117766,111.996593531144));
#32675=CARTESIAN_POINT('Ctrl Pts',(-86.4419221813022,38.4993676140041,112.049243038874));
#32676=CARTESIAN_POINT('Ctrl Pts',(-87.147021086537,38.9355687162316,112.101892546605));
#32677=CARTESIAN_POINT('Ctrl Pts',(-88.08827552557,38.9900353214667,112.154542054336));
#32678=CARTESIAN_POINT('Ctrl Pts',(-88.8389821119455,38.6380758224897,112.207191562067));
#32679=CARTESIAN_POINT('Ctrl Pts',(-89.589688698321,38.2861163235126,112.259841069798));
#32680=CARTESIAN_POINT('Ctrl Pts',(-90.149847432039,37.5277307203235,112.312490577529));
#32681=CARTESIAN_POINT('Ctrl Pts',(-90.2655188693974,36.7067215935002,112.365140085259));
#32682=CARTESIAN_POINT('Ctrl Pts',(-90.2818328412294,36.5909287921421,112.372565622676));
#32683=CARTESIAN_POINT('Ctrl Pts',(-90.2893053017908,36.4738903160605,112.379991160092));
#32684=CARTESIAN_POINT('Ctrl Pts',(-90.2883544400146,36.356729971742,112.387416697508));
#32685=CARTESIAN_POINT('Origin',(-87.7685555885722,36.3549260746835,114.));
#32686=CARTESIAN_POINT('',(-90.282160762018,36.3552974008428,113.387416697508));
#32687=CARTESIAN_POINT('',(-90.2845474745906,36.3528324580843,113.112583302492));
#32688=CARTESIAN_POINT('',(-90.2860555885722,36.3549260746835,114.));
#32689=CARTESIAN_POINT('Ctrl Pts',(-90.2845474745906,36.3528324580843,113.112583302492));
#32690=CARTESIAN_POINT('Ctrl Pts',(-90.2798793876854,36.9364594673067,113.075736828766));
#32691=CARTESIAN_POINT('Ctrl Pts',(-90.0774217774617,37.5230086335642,113.03889035504));
#32692=CARTESIAN_POINT('Ctrl Pts',(-89.7060411231664,37.9688454350711,113.002043881314));
#32693=CARTESIAN_POINT('Ctrl Pts',(-89.1753795251323,38.6058965760332,112.949394373583));
#32694=CARTESIAN_POINT('Ctrl Pts',(-88.29982390578,38.9556520813125,112.896744865852));
#32695=CARTESIAN_POINT('Ctrl Pts',(-87.4762940907326,38.859555611257,112.844095358121));
#32696=CARTESIAN_POINT('Ctrl Pts',(-86.6527642756852,38.7634591412015,112.791445850391));
#32697=CARTESIAN_POINT('Ctrl Pts',(-85.8812602649427,38.2215106958113,112.73879634266));
#32698=CARTESIAN_POINT('Ctrl Pts',(-85.5115316696583,37.4793943614956,112.686146834929));
#32699=CARTESIAN_POINT('Ctrl Pts',(-85.141803074374,36.7372780271799,112.633497327198));
#32700=CARTESIAN_POINT('Ctrl Pts',(-85.1738498945477,35.7949938039387,112.580847819467));
#32701=CARTESIAN_POINT('Ctrl Pts',(-85.5931441915838,35.0797119152388,112.528198311736));
#32702=CARTESIAN_POINT('Ctrl Pts',(-86.0124384886199,34.3644300265389,112.475548804006));
#32703=CARTESIAN_POINT('Ctrl Pts',(-86.8189802625183,33.8761504723801,112.422899296275));
#32704=CARTESIAN_POINT('Ctrl Pts',(-87.6471360650118,33.8362273634649,112.370249788544));
#32705=CARTESIAN_POINT('Ctrl Pts',(-88.4752918675053,33.7963042545498,112.317600280813));
#32706=CARTESIAN_POINT('Ctrl Pts',(-89.325061698594,34.2047375908782,112.264950773082));
#32707=CARTESIAN_POINT('Ctrl Pts',(-89.8112153276443,34.8763703303946,112.212301265351));
#32708=CARTESIAN_POINT('Ctrl Pts',(-90.1181396884788,35.3003935958269,112.179061944398));
#32709=CARTESIAN_POINT('Ctrl Pts',(-90.2801338523397,35.8293229164172,112.145822623445));
#32710=CARTESIAN_POINT('Ctrl Pts',(-90.2832192959692,36.3565168099065,112.112583302492));
#32711=CARTESIAN_POINT('Ctrl Pts',(-90.2883544400146,36.356729971742,112.387416697508));
#32712=CARTESIAN_POINT('Ctrl Pts',(-90.2825633783946,35.6431848589072,112.432640667823));
#32713=CARTESIAN_POINT('Ctrl Pts',(-89.9643334791074,34.925119395463,112.477864638137));
#32714=CARTESIAN_POINT('Ctrl Pts',(-89.4281349618304,34.4564050669767,112.523088608452));
#32715=CARTESIAN_POINT('Ctrl Pts',(-88.8038954759064,33.9107303177339,112.575738116183));
#32716=CARTESIAN_POINT('Ctrl Pts',(-87.88423236306,33.7030134697058,112.628387623914));
#32717=CARTESIAN_POINT('Ctrl Pts',(-87.0860609103553,33.9274197972347,112.681037131644));
#32718=CARTESIAN_POINT('Ctrl Pts',(-86.2878894576506,34.1518261247636,112.733686639375));
#32719=CARTESIAN_POINT('Ctrl Pts',(-85.6112096650878,34.8083556278495,112.786336147106));
#32720=CARTESIAN_POINT('Ctrl Pts',(-85.3627840264822,35.5993806399895,112.838985654837));
#32721=CARTESIAN_POINT('Ctrl Pts',(-85.1143583878767,36.3904056521295,112.891635162568));
#32722=CARTESIAN_POINT('Ctrl Pts',(-85.2941869032285,37.3159261733237,112.944284670298));
#32723=CARTESIAN_POINT('Ctrl Pts',(-85.8207470497215,37.9563715495058,112.996934178029));
#32724=CARTESIAN_POINT('Ctrl Pts',(-86.3473071962145,38.5968169256878,113.04958368576));
#32725=CARTESIAN_POINT('Ctrl Pts',(-87.2205989738487,38.9521871568577,113.102233193491));
#32726=CARTESIAN_POINT('Ctrl Pts',(-88.044728835218,38.8613805527632,113.154882701222));
#32727=CARTESIAN_POINT('Ctrl Pts',(-88.8688586965873,38.7705739486686,113.207532208953));
#32728=CARTESIAN_POINT('Ctrl Pts',(-89.6438266416916,38.2335905093095,113.260181716683));
#32729=CARTESIAN_POINT('Ctrl Pts',(-90.0183127374104,37.4938635111128,113.312831224414));
#32730=CARTESIAN_POINT('Ctrl Pts',(-90.1951502415015,37.1445542108066,113.337693048779));
#32731=CARTESIAN_POINT('Ctrl Pts',(-90.2826859490201,36.7500359601435,113.362554873143));
#32732=CARTESIAN_POINT('Ctrl Pts',(-90.282160762018,36.3552974008428,113.387416697508));
#32733=CARTESIAN_POINT('Origin',(-87.7685555885722,36.3549260746835,114.));
#32734=CARTESIAN_POINT('',(-90.2870431970936,36.3527727133248,114.387416697508));
#32735=CARTESIAN_POINT('',(-90.2900699264125,36.3553920695694,114.112583302492));
#32736=CARTESIAN_POINT('',(-90.2860555885722,36.3549260746835,114.));
#32737=CARTESIAN_POINT('Ctrl Pts',(-90.2900699264125,36.3553920695694,114.112583302492));
#32738=CARTESIAN_POINT('Ctrl Pts',(-90.2901360139808,36.3811153253261,114.110950049548));
#32739=CARTESIAN_POINT('Ctrl Pts',(-90.2897760704703,36.4068366869338,114.109316796605));
#32740=CARTESIAN_POINT('Ctrl Pts',(-90.2889843694534,36.4325447522138,114.107683543661));
#32741=CARTESIAN_POINT('Ctrl Pts',(-90.263463112031,37.2612694068783,114.05503403593));
#32742=CARTESIAN_POINT('Ctrl Pts',(-89.7892774376809,38.0761770717666,114.002384528199));
#32743=CARTESIAN_POINT('Ctrl Pts',(-89.0813922110172,38.5078417491499,113.949735020469));
#32744=CARTESIAN_POINT('Ctrl Pts',(-88.3735069843535,38.9395064265332,113.897085512738));
#32745=CARTESIAN_POINT('Ctrl Pts',(-87.4319222053761,38.9879281164113,113.844436005007));
#32746=CARTESIAN_POINT('Ctrl Pts',(-86.6834910151311,38.6311555820177,113.791786497276));
#32747=CARTESIAN_POINT('Ctrl Pts',(-85.9350598248862,38.274383047624,113.739136989545));
#32748=CARTESIAN_POINT('Ctrl Pts',(-85.3797822233737,37.5124162889586,113.686487481814));
#32749=CARTESIAN_POINT('Ctrl Pts',(-85.2693848672369,36.6906813489767,113.633837974084));
#32750=CARTESIAN_POINT('Ctrl Pts',(-85.1589875111001,35.8689464089947,113.581188466353));
#32751=CARTESIAN_POINT('Ctrl Pts',(-85.493470400339,34.9874432876963,113.528538958622));
#32752=CARTESIAN_POINT('Ctrl Pts',(-86.1212008035358,34.4457880202692,113.475889450891));
#32753=CARTESIAN_POINT('Ctrl Pts',(-86.7489312067326,33.904132752842,113.42323994316));
#32754=CARTESIAN_POINT('Ctrl Pts',(-87.6699091238872,33.7023253392863,113.37059043543));
#32755=CARTESIAN_POINT('Ctrl Pts',(-88.4666232213963,33.9318521016899,113.317940927699));
#32756=CARTESIAN_POINT('Ctrl Pts',(-89.2633373189054,34.1613788640935,113.265291419968));
#32757=CARTESIAN_POINT('Ctrl Pts',(-89.9357875967688,34.8222398024565,113.212641912237));
#32758=CARTESIAN_POINT('Ctrl Pts',(-90.1791289473426,35.6148436599604,113.159992404506));
#32759=CARTESIAN_POINT('Ctrl Pts',(-90.2521691675388,35.8527479871284,113.144189370502));
#32760=CARTESIAN_POINT('Ctrl Pts',(-90.2865495640347,36.1025214638383,113.128386336497));
#32761=CARTESIAN_POINT('Ctrl Pts',(-90.2845474745906,36.3528324580843,113.112583302492));
#32762=CARTESIAN_POINT('Ctrl Pts',(-90.282160762018,36.3552974008428,113.387416697508));
#32763=CARTESIAN_POINT('Ctrl Pts',(-90.2815737684849,35.9141041103816,113.415204380874));
#32764=CARTESIAN_POINT('Ctrl Pts',(-90.1709794034964,35.4726356061123,113.44299206424));
#32765=CARTESIAN_POINT('Ctrl Pts',(-89.9521102560219,35.0937065350684,113.470779747607));
#32766=CARTESIAN_POINT('Ctrl Pts',(-89.5374174325816,34.3757471142548,113.523429255338));
#32767=CARTESIAN_POINT('Ctrl Pts',(-88.7340275393681,33.8822988296621,113.576078763068));
#32768=CARTESIAN_POINT('Ctrl Pts',(-87.9061451674701,33.8370589573346,113.628728270799));
#32769=CARTESIAN_POINT('Ctrl Pts',(-87.078262795572,33.7918190850072,113.68137777853));
#32770=CARTESIAN_POINT('Ctrl Pts',(-86.2258879449895,34.194787624945,113.734027286261));
#32771=CARTESIAN_POINT('Ctrl Pts',(-85.7354317923295,34.8632849174344,113.786676793992));
#32772=CARTESIAN_POINT('Ctrl Pts',(-85.2449756396694,35.5317822099238,113.839326301722));
#32773=CARTESIAN_POINT('Ctrl Pts',(-85.1164381849319,36.4658082549647,113.891975809453));
#32774=CARTESIAN_POINT('Ctrl Pts',(-85.4080899285771,37.2419365485969,113.944625317184));
#32775=CARTESIAN_POINT('Ctrl Pts',(-85.6997416722223,38.0180648422291,113.997274824915));
#32776=CARTESIAN_POINT('Ctrl Pts',(-86.4115826142503,38.6362953844525,114.049924332646));
#32777=CARTESIAN_POINT('Ctrl Pts',(-87.2209104884245,38.8163627602663,114.102573840377));
#32778=CARTESIAN_POINT('Ctrl Pts',(-88.0302383625986,38.99643013608,114.155223348107));
#32779=CARTESIAN_POINT('Ctrl Pts',(-88.937053168919,38.7383343454839,114.207872855838));
#32780=CARTESIAN_POINT('Ctrl Pts',(-89.530264204703,38.1590791903305,114.260522363569));
#32781=CARTESIAN_POINT('Ctrl Pts',(-90.0068442812343,37.6937111349145,114.302820474882));
#32782=CARTESIAN_POINT('Ctrl Pts',(-90.2810131308354,37.0210551986511,114.345118586195));
#32783=CARTESIAN_POINT('Ctrl Pts',(-90.2870431970936,36.3527727133248,114.387416697508));
#32784=CARTESIAN_POINT('Origin',(-87.7685555885722,36.3549260746835,114.));
#32785=CARTESIAN_POINT('',(-90.2884952448755,36.3566728106054,115.387416697508));
#32786=CARTESIAN_POINT('',(-90.283326517746,36.3565773825716,115.112583302492));
#32787=CARTESIAN_POINT('',(-90.2860555885722,36.3549260746835,114.));
#32788=CARTESIAN_POINT('Ctrl Pts',(-90.283326517746,36.3565773825716,115.112583302492));
#32789=CARTESIAN_POINT('Ctrl Pts',(-90.2851690825839,36.6589983336067,115.0935137626));
#32790=CARTESIAN_POINT('Ctrl Pts',(-90.2346569267751,36.9608245377031,115.074444222708));
#32791=CARTESIAN_POINT('Ctrl Pts',(-90.1290212830441,37.2419365615535,115.055374682816));
#32792=CARTESIAN_POINT('Ctrl Pts',(-89.8373695351387,38.0180648665217,115.002725175085));
#32793=CARTESIAN_POINT('Ctrl Pts',(-89.1255285827133,38.6362954177748,114.950075667354));
#32794=CARTESIAN_POINT('Ctrl Pts',(-88.316200696718,38.8163627962183,114.897426159623));
#32795=CARTESIAN_POINT('Ctrl Pts',(-87.5068728107227,38.9964301746617,114.844776651893));
#32796=CARTESIAN_POINT('Ctrl Pts',(-86.6000579911575,38.7383343802956,114.792127144162));
#32797=CARTESIAN_POINT('Ctrl Pts',(-86.0068469467092,38.1590792166814,114.739477636431));
#32798=CARTESIAN_POINT('Ctrl Pts',(-85.413635902261,37.5798240530672,114.6868281287));
#32799=CARTESIAN_POINT('Ctrl Pts',(-85.1340286329297,36.6794095202049,114.634178620969));
#32800=CARTESIAN_POINT('Ctrl Pts',(-85.2947808423313,35.8660248541325,114.581529113238));
#32801=CARTESIAN_POINT('Ctrl Pts',(-85.455533051733,35.0526401880602,114.528879605508));
#32802=CARTESIAN_POINT('Ctrl Pts',(-86.0566447398676,34.3262853887778,114.476230097777));
#32803=CARTESIAN_POINT('Ctrl Pts',(-86.8256110639121,34.0162423589988,114.423580590046));
#32804=CARTESIAN_POINT('Ctrl Pts',(-87.5945773879567,33.7061993292197,114.370931082315));
#32805=CARTESIAN_POINT('Ctrl Pts',(-88.5313983479111,33.812468068944,114.318281574584));
#32806=CARTESIAN_POINT('Ctrl Pts',(-89.2113804076409,34.2868732610265,114.265632066854));
#32807=CARTESIAN_POINT('Ctrl Pts',(-89.8702685816242,34.7465618164327,114.214615812066));
#32808=CARTESIAN_POINT('Ctrl Pts',(-90.2880056165118,35.5519009907723,114.163599557279));
#32809=CARTESIAN_POINT('Ctrl Pts',(-90.2900699264125,36.3553920695694,114.112583302492));
#32810=CARTESIAN_POINT('Ctrl Pts',(-90.2870431970936,36.3527727133248,114.387416697508));
#32811=CARTESIAN_POINT('Ctrl Pts',(-90.2885189037937,36.1892274222949,114.397768093926));
#32812=CARTESIAN_POINT('Ctrl Pts',(-90.2739357189781,36.0259440582166,114.408119490344));
#32813=CARTESIAN_POINT('Ctrl Pts',(-90.2423302986814,35.8660248612744,114.418470886762));
#32814=CARTESIAN_POINT('Ctrl Pts',(-90.081578091628,35.0526402070823,114.471120394492));
#32815=CARTESIAN_POINT('Ctrl Pts',(-89.4804664122735,34.3262854184089,114.523769902223));
#32816=CARTESIAN_POINT('Ctrl Pts',(-88.7115000994606,34.016242393158,114.576419409954));
#32817=CARTESIAN_POINT('Ctrl Pts',(-87.9425337866477,33.7061993679072,114.629068917685));
#32818=CARTESIAN_POINT('Ctrl Pts',(-87.0057128403764,33.8124681060789,114.681718425416));
#32819=CARTESIAN_POINT('Ctrl Pts',(-86.3257307905782,34.2868732912319,114.734367933146));
#32820=CARTESIAN_POINT('Ctrl Pts',(-85.6457487407801,34.7612784763849,114.787017440877));
#32821=CARTESIAN_POINT('Ctrl Pts',(-85.2226055874552,35.6038201085191,114.839666948608));
#32822=CARTESIAN_POINT('Ctrl Pts',(-85.2481268445046,36.4325447510792,114.892316456339));
#32823=CARTESIAN_POINT('Ctrl Pts',(-85.2736481015539,37.2612693936393,114.94496596407));
#32824=CARTESIAN_POINT('Ctrl Pts',(-85.7478337689776,38.0761770466252,114.997615471801));
#32825=CARTESIAN_POINT('Ctrl Pts',(-86.4557189853018,38.5078417177038,115.050264979531));
#32826=CARTESIAN_POINT('Ctrl Pts',(-87.1636042016259,38.9395063887825,115.102914487262));
#32827=CARTESIAN_POINT('Ctrl Pts',(-88.1051889668506,38.9879280779537,115.155563994993));
#32828=CARTESIAN_POINT('Ctrl Pts',(-88.853620146164,38.6311555487714,115.208213502724));
#32829=CARTESIAN_POINT('Ctrl Pts',(-89.6020513254776,38.2743830195891,115.260863010455));
#32830=CARTESIAN_POINT('Ctrl Pts',(-90.1573289188799,37.5124162720532,115.313512518185));
#32831=CARTESIAN_POINT('Ctrl Pts',(-90.2677262734045,36.6906813440736,115.366162025916));
#32832=CARTESIAN_POINT('Ctrl Pts',(-90.2825821230674,36.5801028740972,115.373246916447));
#32833=CARTESIAN_POINT('Ctrl Pts',(-90.2893819483098,36.468442104034,115.380331806977));
#32834=CARTESIAN_POINT('Ctrl Pts',(-90.2884952448755,36.3566728106054,115.387416697508));
#32835=CARTESIAN_POINT('Origin',(-87.7685555885722,36.3549260746835,114.));
#32836=CARTESIAN_POINT('',(-90.2821875011782,36.3553827988861,116.387416697508));
#32837=CARTESIAN_POINT('',(-90.2844059463112,36.3528657341098,116.112583302492));
#32838=CARTESIAN_POINT('',(-90.2860555885722,36.3549260746835,114.));
#32839=CARTESIAN_POINT('Ctrl Pts',(-90.2844059463112,36.3528657341098,116.112583302492));
#32840=CARTESIAN_POINT('Ctrl Pts',(-90.2798733875279,36.9311794857661,116.076077475652));
#32841=CARTESIAN_POINT('Ctrl Pts',(-90.0814675469238,37.5123030648938,116.039571648811));
#32842=CARTESIAN_POINT('Ctrl Pts',(-89.7163641558721,37.9563715728973,116.003065821971));
#32843=CARTESIAN_POINT('Ctrl Pts',(-89.1898040016879,38.5968169584335,115.95041631424));
#32844=CARTESIAN_POINT('Ctrl Pts',(-88.3165122112982,38.9521871947936,115.897766806509));
#32845=CARTESIAN_POINT('Ctrl Pts',(-87.4923823378917,38.8613805893724,115.845117298778));
#32846=CARTESIAN_POINT('Ctrl Pts',(-86.6682524644853,38.7705739839512,115.792467791047));
#32847=CARTESIAN_POINT('Ctrl Pts',(-85.8932845080619,38.2335905367486,115.739818283317));
#32848=CARTESIAN_POINT('Ctrl Pts',(-85.5187984068737,37.4938635277473,115.687168775586));
#32849=CARTESIAN_POINT('Ctrl Pts',(-85.1443123056855,36.754136518746,115.634519267855));
#32850=CARTESIAN_POINT('Ctrl Pts',(-85.1703080597325,35.811665947946,115.581869760124));
#32851=CARTESIAN_POINT('Ctrl Pts',(-85.58500088923,35.0937065166461,115.529220252393));
#32852=CARTESIAN_POINT('Ctrl Pts',(-85.9996937187276,34.3757470853462,115.476570744662));
#32853=CARTESIAN_POINT('Ctrl Pts',(-86.8030836236757,33.8822987935465,115.423921236932));
#32854=CARTESIAN_POINT('Ctrl Pts',(-87.6309660076658,33.8370589205585,115.371271729201));
#32855=CARTESIAN_POINT('Ctrl Pts',(-88.4588483916559,33.7918190475706,115.31862222147));
#32856=CARTESIAN_POINT('Ctrl Pts',(-89.3112232546881,34.1947875933945,115.265972713739));
#32857=CARTESIAN_POINT('Ctrl Pts',(-89.8016794145115,34.8632848956482,115.213323206008));
#32858=CARTESIAN_POINT('Ctrl Pts',(-90.1144933947941,35.2896538946663,115.17974323817));
#32859=CARTESIAN_POINT('Ctrl Pts',(-90.2800819052201,35.8240377477917,115.146163270331));
#32860=CARTESIAN_POINT('Ctrl Pts',(-90.283326517746,36.3565773825716,115.112583302492));
#32861=CARTESIAN_POINT('Ctrl Pts',(-90.2884952448755,36.3566728106054,115.387416697508));
#32862=CARTESIAN_POINT('Ctrl Pts',(-90.2827926440549,35.6378578835658,115.432981314708));
#32863=CARTESIAN_POINT('Ctrl Pts',(-89.9591688972838,34.9145543409096,115.478545931909));
#32864=CARTESIAN_POINT('Ctrl Pts',(-89.4159103495481,34.4457880481547,115.524110549109));
#32865=CARTESIAN_POINT('Ctrl Pts',(-88.7881799555201,33.9041327886388,115.57676005684));
#32866=CARTESIAN_POINT('Ctrl Pts',(-87.8672020518174,33.7023253780303,115.62940956457));
#32867=CARTESIAN_POINT('Ctrl Pts',(-87.0704879659451,33.9318521370812,115.682059072301));
#32868=CARTESIAN_POINT('Ctrl Pts',(-86.2737738800728,34.161378896132,115.734708580032));
#32869=CARTESIAN_POINT('Ctrl Pts',(-85.601323612031,34.8222398248422,115.787358087763));
#32870=CARTESIAN_POINT('Ctrl Pts',(-85.3579822650111,35.6148436707692,115.840007595494));
#32871=CARTESIAN_POINT('Ctrl Pts',(-85.1146409179913,36.4074475166962,115.892657103225));
#32872=CARTESIAN_POINT('Ctrl Pts',(-85.3004084919934,37.33179427984,115.945306610955));
#32873=CARTESIAN_POINT('Ctrl Pts',(-85.8310700822764,37.9688454114975,115.997956118686));
#32874=CARTESIAN_POINT('Ctrl Pts',(-86.3617316725594,38.6058965431549,116.050605626417));
#32875=CARTESIAN_POINT('Ctrl Pts',(-87.2372872791233,38.955652043326,116.103255134148));
#32876=CARTESIAN_POINT('Ctrl Pts',(-88.0608170821422,38.8595555746744,116.155904641879));
#32877=CARTESIAN_POINT('Ctrl Pts',(-88.8843468851612,38.7634591060228,116.20855414961));
#32878=CARTESIAN_POINT('Ctrl Pts',(-89.6558508846352,38.2215106685486,116.26120365734));
#32879=CARTESIAN_POINT('Ctrl Pts',(-90.0255794745196,37.4793943450724,116.313853165071));
#32880=CARTESIAN_POINT('Ctrl Pts',(-90.197778242606,37.1337583294227,116.33837434255));
#32881=CARTESIAN_POINT('Ctrl Pts',(-90.2828250094709,36.7447024542471,116.362895520029));
#32882=CARTESIAN_POINT('Ctrl Pts',(-90.2821875011782,36.3553827988861,116.387416697508));
#32883=CARTESIAN_POINT('Origin',(-87.7685555885722,36.3549260746835,114.));
#32884=CARTESIAN_POINT('',(-90.286883306508,36.3527492243956,117.387416697508));
#32885=CARTESIAN_POINT('',(-90.2901099846489,36.3552960960066,117.112583302492));
#32886=CARTESIAN_POINT('',(-90.2860555885722,36.3549260746835,114.));
#32887=CARTESIAN_POINT('Ctrl Pts',(-90.2901099846489,36.3552960960066,117.112583302492));
#32888=CARTESIAN_POINT('Ctrl Pts',(-90.290152157795,36.3756533940165,117.111290696434));
#32889=CARTESIAN_POINT('Ctrl Pts',(-90.2899267214508,36.3960097343219,117.109998090376));
#32890=CARTESIAN_POINT('Ctrl Pts',(-90.289430800665,36.4163594829559,117.108705484318));
#32891=CARTESIAN_POINT('Ctrl Pts',(-90.269231309038,37.2452309255615,117.056055976587));
#32892=CARTESIAN_POINT('Ctrl Pts',(-89.8002879307519,38.063166536728,117.003406468856));
#32893=CARTESIAN_POINT('Ctrl Pts',(-89.0951890152183,38.4993676453264,116.950756961126));
#32894=CARTESIAN_POINT('Ctrl Pts',(-88.3900900996848,38.9355687539247,116.898107453395));
#32895=CARTESIAN_POINT('Ctrl Pts',(-87.4488356469037,38.9900353599551,116.845457945664));
#32896=CARTESIAN_POINT('Ctrl Pts',(-86.6981290495635,38.638075855837,116.792808437933));
#32897=CARTESIAN_POINT('Ctrl Pts',(-85.9474224522232,38.286116351719,116.740158930202));
#32898=CARTESIAN_POINT('Ctrl Pts',(-85.3872637103238,37.5277307374526,116.687509422471));
#32899=CARTESIAN_POINT('Ctrl Pts',(-85.2715922712763,36.7067215986376,116.634859914741));
#32900=CARTESIAN_POINT('Ctrl Pts',(-85.1559208322288,35.8857124598225,116.58221040701));
#32901=CARTESIAN_POINT('Ctrl Pts',(-85.4847366960332,35.0020797964589,116.529560899279));
#32902=CARTESIAN_POINT('Ctrl Pts',(-86.108976191075,34.4564050392462,116.476911391548));
#32903=CARTESIAN_POINT('Ctrl Pts',(-86.7332156861168,33.9107302820335,116.424261883817));
#32904=CARTESIAN_POINT('Ctrl Pts',(-87.6528788123959,33.7030134309718,116.371612376086));
#32905=CARTESIAN_POINT('Ctrl Pts',(-88.4510502767586,33.9274197617787,116.318962868356));
#32906=CARTESIAN_POINT('Ctrl Pts',(-89.2492217411213,34.1518260925856,116.266313360625));
#32907=CARTESIAN_POINT('Ctrl Pts',(-89.9259015435676,34.808355605261,116.213663852894));
#32908=CARTESIAN_POINT('Ctrl Pts',(-90.1743271858014,35.5993806289549,116.161014345163));
#32909=CARTESIAN_POINT('Ctrl Pts',(-90.2505008190614,35.8419290612044,116.144870664273));
#32910=CARTESIAN_POINT('Ctrl Pts',(-90.2864103436622,36.0971226522707,116.128726983382));
#32911=CARTESIAN_POINT('Ctrl Pts',(-90.2844059463112,36.3528657341098,116.112583302492));
#32912=CARTESIAN_POINT('Ctrl Pts',(-90.2821875011782,36.3553827988861,116.387416697508));
#32913=CARTESIAN_POINT('Ctrl Pts',(-90.2814562131392,35.9087928319514,116.41554502776));
#32914=CARTESIAN_POINT('Ctrl Pts',(-90.1679775627328,35.461855770756,116.443673358012));
#32915=CARTESIAN_POINT('Ctrl Pts',(-89.943966953787,35.0797119338654,116.471801688264));
#32916=CARTESIAN_POINT('Ctrl Pts',(-89.5246726628754,34.3644300556127,116.524451195994));
#32917=CARTESIAN_POINT('Ctrl Pts',(-88.7181309007576,33.8761505085855,116.577100703725));
#32918=CARTESIAN_POINT('Ctrl Pts',(-87.8899751103602,33.8362274002532,116.629750211456));
#32919=CARTESIAN_POINT('Ctrl Pts',(-87.0618193199627,33.7963042919208,116.682399719187));
#32920=CARTESIAN_POINT('Ctrl Pts',(-86.2120495012857,34.2047376222833,116.735049226918));
#32921=CARTESIAN_POINT('Ctrl Pts',(-85.725895879336,34.8763703519896,116.787698734649));
#32922=CARTESIAN_POINT('Ctrl Pts',(-85.2397422573863,35.548003081696,116.840348242379));
#32923=CARTESIAN_POINT('Ctrl Pts',(-85.1172048321637,36.4828352107461,116.89299775011));
#32924=CARTESIAN_POINT('Ctrl Pts',(-85.4138340819895,37.2570748092528,116.945647257841));
#32925=CARTESIAN_POINT('Ctrl Pts',(-85.7104633318153,38.0313144077595,116.998296765572));
#32926=CARTESIAN_POINT('Ctrl Pts',(-86.4262592566894,38.6449614757227,117.050946273303));
#32927=CARTESIAN_POINT('Ctrl Pts',(-87.2367266590444,38.8198284464961,117.103595781033));
#32928=CARTESIAN_POINT('Ctrl Pts',(-88.0471940613994,38.9946954172694,117.156245288764));
#32929=CARTESIAN_POINT('Ctrl Pts',(-88.9523329412353,38.730782290853,117.208894796495));
#32930=CARTESIAN_POINT('Ctrl Pts',(-89.5418123516562,38.1477300698326,117.261544304226));
#32931=CARTESIAN_POINT('Ctrl Pts',(-90.0115804930765,37.6830838864755,117.303501768653));
#32932=CARTESIAN_POINT('Ctrl Pts',(-90.2808789705167,37.0157581916285,117.345459233081));
#32933=CARTESIAN_POINT('Ctrl Pts',(-90.286883306508,36.3527492243956,117.387416697508));
#32934=CARTESIAN_POINT('Origin',(-87.7685555885722,36.3549260746835,114.));
#32935=CARTESIAN_POINT('',(-90.2886325747468,36.3566124302836,118.387416697508));
#32936=CARTESIAN_POINT('',(-90.2834379459911,36.3566354806138,118.112583302492));
#32937=CARTESIAN_POINT('',(-90.2860555885722,36.3549260746835,114.));
#32938=CARTESIAN_POINT('Ctrl Pts',(-90.2834379459911,36.3566354806138,118.112583302492));
#32939=CARTESIAN_POINT('Ctrl Pts',(-90.2853166571071,36.653621048985,118.093854409486));
#32940=CARTESIAN_POINT('Ctrl Pts',(-90.2366418321613,36.9500108449635,118.075125516479));
#32941=CARTESIAN_POINT('Ctrl Pts',(-90.1346681153728,37.2267617295443,118.056396623473));
#32942=CARTESIAN_POINT('Ctrl Pts',(-89.8480058984144,38.0047467301666,118.003747115742));
#32943=CARTESIAN_POINT('Ctrl Pts',(-89.1401492778511,38.6275352663295,117.951097608011));
#32944=CARTESIAN_POINT('Ctrl Pts',(-88.3319942883572,38.812795625777,117.89844810028));
#32945=CARTESIAN_POINT('Ctrl Pts',(-87.5238392988634,38.9980559852244,117.845798592549));
#32946=CARTESIAN_POINT('Ctrl Pts',(-86.6153859404389,38.7457881679563,117.793149084819));
#32947=CARTESIAN_POINT('Ctrl Pts',(-86.0184677284529,38.1703539527493,117.740499577088));
#32948=CARTESIAN_POINT('Ctrl Pts',(-85.4215495164669,37.5949197375422,117.687850069357));
#32949=CARTESIAN_POINT('Ctrl Pts',(-85.1361664509194,36.696319124396,117.635200561626));
#32950=CARTESIAN_POINT('Ctrl Pts',(-85.291692604806,35.8819190364259,117.582551053895));
#32951=CARTESIAN_POINT('Ctrl Pts',(-85.4472187586926,35.0675189484558,117.529901546165));
#32952=CARTESIAN_POINT('Ctrl Pts',(-86.0436541320133,34.3373193856618,117.477252038434));
#32953=CARTESIAN_POINT('Ctrl Pts',(-86.8106138181558,34.0223452158303,117.424602530703));
#32954=CARTESIAN_POINT('Ctrl Pts',(-87.5775735042984,33.7073710459988,117.371953022972));
#32955=CARTESIAN_POINT('Ctrl Pts',(-88.5150575032628,33.8076222691299,117.319303515241));
#32956=CARTESIAN_POINT('Ctrl Pts',(-89.1980717002612,34.2776515177178,117.26665400751));
#32957=CARTESIAN_POINT('Ctrl Pts',(-89.8643171120078,34.7361410068596,117.215297105838));
#32958=CARTESIAN_POINT('Ctrl Pts',(-90.2884343912986,35.5464744556199,117.163940204165));
#32959=CARTESIAN_POINT('Ctrl Pts',(-90.2901099846489,36.3552960960066,117.112583302492));
#32960=CARTESIAN_POINT('Ctrl Pts',(-90.286883306508,36.3527492243956,117.387416697508));
#32961=CARTESIAN_POINT('Ctrl Pts',(-90.288413394689,36.1837942914657,117.398108740811));
#32962=CARTESIAN_POINT('Ctrl Pts',(-90.2728455288958,36.0151196808007,117.408800784115));
#32963=CARTESIAN_POINT('Ctrl Pts',(-90.2391400683468,35.8501508364386,117.419492827418));
#32964=CARTESIAN_POINT('Ctrl Pts',(-90.0731684336104,35.0378151396894,117.472142335149));
#32965=CARTESIAN_POINT('Ctrl Pts',(-89.4674052231316,34.3153350618152,117.52479184288));
#32966=CARTESIAN_POINT('Ctrl Pts',(-88.6964639766552,34.0102359595115,117.577441350611));
#32967=CARTESIAN_POINT('Ctrl Pts',(-87.9255227301789,33.7051368572078,117.630090858342));
#32968=CARTESIAN_POINT('Ctrl Pts',(-86.9894034477049,33.8174187304746,117.682740366072));
#32969=CARTESIAN_POINT('Ctrl Pts',(-86.3124815705486,34.2961802994946,117.735389873803));
#32970=CARTESIAN_POINT('Ctrl Pts',(-85.6355596933923,34.7749418685146,117.788039381534));
#32971=CARTESIAN_POINT('Ctrl Pts',(-85.2178352215536,35.620183133288,117.840688889265));
#32972=CARTESIAN_POINT('Ctrl Pts',(-85.2486771920908,36.4487268198985,117.893338396996));
#32973=CARTESIAN_POINT('Ctrl Pts',(-85.279519162628,37.277270506509,117.945987904727));
#32974=CARTESIAN_POINT('Ctrl Pts',(-85.7589275755411,38.0891166149566,117.998637412457));
#32975=CARTESIAN_POINT('Ctrl Pts',(-86.4695699170935,38.5162270574792,118.051286920188));
#32976=CARTESIAN_POINT('Ctrl Pts',(-87.1802122586458,38.9433375000017,118.103936427919));
#32977=CARTESIAN_POINT('Ctrl Pts',(-88.1220885288374,38.9857122765992,118.15658593565));
#32978=CARTESIAN_POINT('Ctrl Pts',(-88.8682134435465,38.6241414268697,118.209235443381));
#32979=CARTESIAN_POINT('Ctrl Pts',(-89.6143383582556,38.2625705771402,118.261884951112));
#32980=CARTESIAN_POINT('Ctrl Pts',(-90.1647119174822,37.4970541010838,118.314534458842));
#32981=CARTESIAN_POINT('Ctrl Pts',(-90.2698306375093,36.674627251678,118.367183966573));
#32982=CARTESIAN_POINT('Ctrl Pts',(-90.283296029496,36.5692768449678,118.373928210218));
#32983=CARTESIAN_POINT('Ctrl Pts',(-90.2894553061913,36.4629926050629,118.380672453863));
#32984=CARTESIAN_POINT('Ctrl Pts',(-90.2886325747468,36.3566124302836,118.387416697508));
#32985=CARTESIAN_POINT('Origin',(-87.7685555885722,36.3549260746835,114.));
#32986=CARTESIAN_POINT('',(-90.282219751568,36.3554675197253,119.387416697508));
#32987=CARTESIAN_POINT('',(-90.2842673072634,36.3529021929646,119.112583302492));
#32988=CARTESIAN_POINT('',(-90.2860555885722,36.3549260746835,114.));
#32989=CARTESIAN_POINT('Ctrl Pts',(-90.2842673072634,36.3529021929646,119.112583302492));
#32990=CARTESIAN_POINT('Ctrl Pts',(-90.2798740930897,36.9258994299071,119.076418122537));
#32991=CARTESIAN_POINT('Ctrl Pts',(-90.0854711696263,37.5015935291692,119.040252942582));
#32992=CARTESIAN_POINT('Ctrl Pts',(-89.7266068808129,37.9438316833838,119.004087762628));
#32993=CARTESIAN_POINT('Ctrl Pts',(-89.2041698800348,38.5876449078244,118.951438254897));
#32994=CARTESIAN_POINT('Ctrl Pts',(-88.3331779247476,38.9486152241081,118.898788747166));
#32995=CARTESIAN_POINT('Ctrl Pts',(-87.508481971726,38.8631022274075,118.846139239435));
#32996=CARTESIAN_POINT('Ctrl Pts',(-86.6837860187044,38.7775892307069,118.793489731704));
#32997=CARTESIAN_POINT('Ctrl Pts',(-85.9053860679484,38.245592921022,118.740840223974));
#32998=CARTESIAN_POINT('Ctrl Pts',(-85.526157900707,37.5082857359385,118.688190716243));
#32999=CARTESIAN_POINT('Ctrl Pts',(-85.1469297334656,36.770978550855,118.635541208512));
#33000=CARTESIAN_POINT('Ctrl Pts',(-85.1668733497388,35.828360490373,118.582891700781));
#33001=CARTESIAN_POINT('Ctrl Pts',(-85.5769476140976,35.1077531177242,118.53024219305));
#33002=CARTESIAN_POINT('Ctrl Pts',(-85.9870218784565,34.3871457450755,118.477592685319));
#33003=CARTESIAN_POINT('Ctrl Pts',(-86.787226790901,33.8885490602601,118.424943177589));
#33004=CARTESIAN_POINT('Ctrl Pts',(-87.614801623072,33.8379942884047,118.372293669858));
#33005=CARTESIAN_POINT('Ctrl Pts',(-88.4423764552431,33.7874395165493,118.319644162127));
#33006=CARTESIAN_POINT('Ctrl Pts',(-89.2973212071407,34.1849266576539,118.266994654396));
#33007=CARTESIAN_POINT('Ctrl Pts',(-89.7920596764127,34.8502609607471,118.214345146665));
#33008=CARTESIAN_POINT('Ctrl Pts',(-90.1108059236012,35.2789173628837,118.180424531941));
#33009=CARTESIAN_POINT('Ctrl Pts',(-90.2800353404061,35.8187535545449,118.146503917216));
#33010=CARTESIAN_POINT('Ctrl Pts',(-90.2834379459911,36.3566354806138,118.112583302492));
#33011=CARTESIAN_POINT('Ctrl Pts',(-90.2886325747468,36.3566124302836,118.387416697508));
#33012=CARTESIAN_POINT('Ctrl Pts',(-90.2830325836699,35.6325267842361,118.433321961594));
#33013=CARTESIAN_POINT('Ctrl Pts',(-89.9539590026799,34.9039965145798,118.47922722568));
#33014=CARTESIAN_POINT('Ctrl Pts',(-89.4036178173749,34.4352497422075,118.525132489766));
#33015=CARTESIAN_POINT('Ctrl Pts',(-88.7724223963857,33.897636304898,118.577781997497));
#33016=CARTESIAN_POINT('Ctrl Pts',(-87.8501676735797,33.7017466530343,118.630431505227));
#33017=CARTESIAN_POINT('Ctrl Pts',(-87.0549438026942,33.9363843798368,118.683081012958));
#33018=CARTESIAN_POINT('Ctrl Pts',(-86.2597199318087,34.1710221066394,118.735730520689));
#33019=CARTESIAN_POINT('Ctrl Pts',(-85.5915269128436,34.8361872121083,118.78838002842));
#33020=CARTESIAN_POINT('Ctrl Pts',(-85.3532798904614,35.6303372139996,118.841029536151));
#33021=CARTESIAN_POINT('Ctrl Pts',(-85.1150328680792,36.4244872158909,118.893679043881));
#33022=CARTESIAN_POINT('Ctrl Pts',(-85.3067318422799,37.3476221142046,118.946328551612));
#33023=CARTESIAN_POINT('Ctrl Pts',(-85.8414729970048,37.9812527339857,118.998978059343));
#33024=CARTESIAN_POINT('Ctrl Pts',(-86.3762141517297,38.6148833537668,119.051627567074));
#33025=CARTESIAN_POINT('Ctrl Pts',(-87.2539974869788,38.9590096950153,119.104277074805));
#33026=CARTESIAN_POINT('Ctrl Pts',(-88.0768932785437,38.8576273278598,119.156926582536));
#33027=CARTESIAN_POINT('Ctrl Pts',(-88.8997890701086,38.7562449607043,119.209576090266));
#33028=CARTESIAN_POINT('Ctrl Pts',(-89.6677973179892,38.2093538851449,119.262225597997));
#33029=CARTESIAN_POINT('Ctrl Pts',(-90.0327531567428,37.4648788252948,119.314875105728));
#33030=CARTESIAN_POINT('Ctrl Pts',(-90.2003677500134,37.1229610612634,119.339055636321));
#33031=CARTESIAN_POINT('Ctrl Pts',(-90.2829655843985,36.7393664592534,119.363236166915));
#33032=CARTESIAN_POINT('Ctrl Pts',(-90.282219751568,36.3554675197253,119.387416697508));
#33033=CARTESIAN_POINT('Origin',(-87.7685555885722,36.3549260746835,114.));
#33034=CARTESIAN_POINT('',(-90.2867225490468,36.352727843524,120.387416697508));
#33035=CARTESIAN_POINT('',(-90.2901412986672,36.3551993258176,120.112583302492));
#33036=CARTESIAN_POINT('',(-90.2860555885722,36.3549260746835,114.));
#33037=CARTESIAN_POINT('Ctrl Pts',(-90.2901412986672,36.3551993258176,120.112583302492));
#33038=CARTESIAN_POINT('Ctrl Pts',(-90.2901645977928,36.3701912646894,120.11163134332));
#33039=CARTESIAN_POINT('Ctrl Pts',(-90.2900423341944,36.3851828134258,120.110679384147));
#33040=CARTESIAN_POINT('Ctrl Pts',(-90.2897733450593,36.4001717289872,120.109727424975));
#33041=CARTESIAN_POINT('Ctrl Pts',(-90.2748965037429,37.2291558373634,120.057077917244));
#33042=CARTESIAN_POINT('Ctrl Pts',(-89.8112146580294,38.0500855733585,120.004428409513));
#33043=CARTESIAN_POINT('Ctrl Pts',(-89.1089310994663,38.4908051035161,119.951778901782));
#33044=CARTESIAN_POINT('Ctrl Pts',(-88.4066475409033,38.9315246336736,119.899129394052));
#33045=CARTESIAN_POINT('Ctrl Pts',(-87.4657622694907,38.9920339579935,119.846479886321));
#33046=CARTESIAN_POINT('Ctrl Pts',(-86.7128112286454,38.6449020075891,119.79383037859));
#33047=CARTESIAN_POINT('Ctrl Pts',(-85.9598601878,38.2977700571847,119.741180870859));
#33048=CARTESIAN_POINT('Ctrl Pts',(-85.3948433775217,37.542996832056,119.688531363128));
#33049=CARTESIAN_POINT('Ctrl Pts',(-85.2739026187123,36.722747338356,119.635881855397));
#33050=CARTESIAN_POINT('Ctrl Pts',(-85.1529618599029,35.902497844656,119.583232347667));
#33051=CARTESIAN_POINT('Ctrl Pts',(-85.4760971525623,35.0167720823848,119.530582839936));
#33052=CARTESIAN_POINT('Ctrl Pts',(-86.0968200051661,34.467100336265,119.477933332205));
#33053=CARTESIAN_POINT('Ctrl Pts',(-86.71754285777,33.9174285901452,119.425283824474));
#33054=CARTESIAN_POINT('Ctrl Pts',(-87.6358532703183,33.7038108601768,119.372634316743));
#33055=CARTESIAN_POINT('Ctrl Pts',(-88.4354491918029,33.9230875057825,119.319984809013));
#33056=CARTESIAN_POINT('Ctrl Pts',(-89.2350451132875,34.1423641513883,119.267335301282));
#33057=CARTESIAN_POINT('Ctrl Pts',(-89.9159265437086,34.7945351725681,119.214685793551));
#33058=CARTESIAN_POINT('Ctrl Pts',(-90.1694262357844,35.5839487494568,119.16203628582));
#33059=CARTESIAN_POINT('Ctrl Pts',(-90.2487958670574,35.8311106454198,119.145551958044));
#33060=CARTESIAN_POINT('Ctrl Pts',(-90.2862697632866,36.0917262695954,119.129067630268));
#33061=CARTESIAN_POINT('Ctrl Pts',(-90.2842673072634,36.3529021929646,119.112583302492));
#33062=CARTESIAN_POINT('Ctrl Pts',(-90.282219751568,36.3554675197253,119.387416697508));
#33063=CARTESIAN_POINT('Ctrl Pts',(-90.2813416443767,35.9034836358174,119.415885674645));
#33064=CARTESIAN_POINT('Ctrl Pts',(-90.1649362220051,35.4510778926663,119.444354651783));
#33065=CARTESIAN_POINT('Ctrl Pts',(-89.9357339572164,35.0657698934732,119.472823628921));
#33066=CARTESIAN_POINT('Ctrl Pts',(-89.5118554893097,34.3531950656423,119.525473136651));
#33067=CARTESIAN_POINT('Ctrl Pts',(-88.7021951238695,33.8701044541211,119.578122644382));
#33068=CARTESIAN_POINT('Ctrl Pts',(-87.8738000531233,33.8354997207509,119.630772152113));
#33069=CARTESIAN_POINT('Ctrl Pts',(-87.0454049823771,33.8008949873808,119.683421659844));
#33070=CARTESIAN_POINT('Ctrl Pts',(-86.1982752063249,34.2147761321616,119.736071167575));
#33071=CARTESIAN_POINT('Ctrl Pts',(-85.7164441722275,34.8895166799831,119.788720675305));
#33072=CARTESIAN_POINT('Ctrl Pts',(-85.2346131381301,35.5642572278047,119.841370183036));
#33073=CARTESIAN_POINT('Ctrl Pts',(-85.1180808459875,36.499857178667,119.894019690767));
#33074=CARTESIAN_POINT('Ctrl Pts',(-85.419675344928,37.272176012196,119.946669198498));
#33075=CARTESIAN_POINT('Ctrl Pts',(-85.7212698438684,38.044494845725,119.999318706229));
#33076=CARTESIAN_POINT('Ctrl Pts',(-86.4409911338919,38.6535325619209,120.05196821396));
#33077=CARTESIAN_POINT('Ctrl Pts',(-87.2525647049724,38.8231922227827,120.10461772169));
#33078=CARTESIAN_POINT('Ctrl Pts',(-88.0641382760528,38.9928518836446,120.157267229421));
#33079=CARTESIAN_POINT('Ctrl Pts',(-88.9675641281902,38.7231334891725,120.209916737152));
#33080=CARTESIAN_POINT('Ctrl Pts',(-89.5532874944098,38.1363076144321,120.262566244883));
#33081=CARTESIAN_POINT('Ctrl Pts',(-90.0162726867219,37.6724509439633,120.304183062425));
#33082=CARTESIAN_POINT('Ctrl Pts',(-90.2807536717285,37.0104618326376,120.345799879966));
#33083=CARTESIAN_POINT('Ctrl Pts',(-90.2867225490468,36.352727843524,120.387416697508));
#33084=CARTESIAN_POINT('Origin',(-87.7685555885722,36.3549260746835,114.));
#33085=CARTESIAN_POINT('',(-90.2887581529621,36.3565049378502,121.387416697508));
#33086=CARTESIAN_POINT('',(-90.2835503128821,36.3566878611388,121.112583302492));
#33087=CARTESIAN_POINT('',(-90.2860555885722,36.3549260746835,114.));
#33088=CARTESIAN_POINT('',(-85.855089591907,37.9909132780583,122.));
#33089=CARTESIAN_POINT('Ctrl Pts',(-90.2887581529621,36.3565049378502,121.387416697508));
#33090=CARTESIAN_POINT('Ctrl Pts',(-90.2833000777792,35.6272821077594,121.43366260848));
#33091=CARTESIAN_POINT('Ctrl Pts',(-89.9487703120527,34.8938081203929,121.479908519451));
#33092=CARTESIAN_POINT('Ctrl Pts',(-89.3912933146495,34.4249748138373,121.526154430423));
#33093=CARTESIAN_POINT('Ctrl Pts',(-88.7566233758821,33.8912229149252,121.578803938153));
#33094=CARTESIAN_POINT('Ctrl Pts',(-87.8329892401945,33.7004745205997,121.631453445884));
#33095=CARTESIAN_POINT('Ctrl Pts',(-87.0393721722715,33.9406285050808,121.684102953615));
#33096=CARTESIAN_POINT('Ctrl Pts',(-86.2457551043485,34.1807824895619,121.736752461346));
#33097=CARTESIAN_POINT('Ctrl Pts',(-85.5821551041903,34.8518388528496,121.789401969077));
#33098=CARTESIAN_POINT('Ctrl Pts',(-85.3491898794995,35.6461247484183,121.842051476807));
#33099=CARTESIAN_POINT('Ctrl Pts',(-85.1162246548087,36.4404106439871,121.894700984538));
#33100=CARTESIAN_POINT('Ctrl Pts',(-85.3138942055855,37.3579260718368,121.947350492269));
#33101=CARTESIAN_POINT('Ctrl Pts',(-85.855089591907,37.9909132780583,122.));
#33102=CARTESIAN_POINT('',(-89.6856658064524,37.9934539967174,122.));
#33103=CARTESIAN_POINT('Origin',(-87.7685555885722,36.3549260746835,122.));
#33104=CARTESIAN_POINT('Ctrl Pts',(-89.6856746522266,37.9934601639126,122.));
#33105=CARTESIAN_POINT('Ctrl Pts',(-89.1628540835289,38.6021752894523,121.949053726697));
#33106=CARTESIAN_POINT('Ctrl Pts',(-88.3231296031605,38.9423515356051,121.898107453395));
#33107=CARTESIAN_POINT('Ctrl Pts',(-87.5244587668031,38.8645887304742,121.847161180092));
#33108=CARTESIAN_POINT('Ctrl Pts',(-86.6990867886923,38.7842261613498,121.794511672361));
#33109=CARTESIAN_POINT('Ctrl Pts',(-85.9175593487471,38.2575123577278,121.74186216463));
#33110=CARTESIAN_POINT('Ctrl Pts',(-85.5336747406072,37.5227256222368,121.6892126569));
#33111=CARTESIAN_POINT('Ctrl Pts',(-85.1497901324673,36.7879388867457,121.636563149169));
#33112=CARTESIAN_POINT('Ctrl Pts',(-85.1635483561328,35.8450792193857,121.583913641438));
#33113=CARTESIAN_POINT('Ctrl Pts',(-85.5689531296241,35.1218194524428,121.531264133707));
#33114=CARTESIAN_POINT('Ctrl Pts',(-85.9743579031154,34.3985596854999,121.478614625976));
#33115=CARTESIAN_POINT('Ctrl Pts',(-86.7714092264326,33.8948998189741,121.425965118245));
#33116=CARTESIAN_POINT('Ctrl Pts',(-87.5986589277565,33.8390488405726,121.373315610515));
#33117=CARTESIAN_POINT('Ctrl Pts',(-88.4259086290804,33.7831978621711,121.320666102784));
#33118=CARTESIAN_POINT('Ctrl Pts',(-89.2833567084111,34.1751557718939,121.268016595053));
#33119=CARTESIAN_POINT('Ctrl Pts',(-89.7823490459092,34.837291568606,121.215367087322));
#33120=CARTESIAN_POINT('Ctrl Pts',(-90.1070644659248,35.2681713380526,121.181105825712));
#33121=CARTESIAN_POINT('Ctrl Pts',(-90.2799862325785,35.8134621316163,121.146844564102));
#33122=CARTESIAN_POINT('Ctrl Pts',(-90.2835503128821,36.3566878611388,121.112583302492));
#33123=CARTESIAN_POINT('Origin',(-87.7685555885722,36.3549260746835,124.208423447177));
#33124=CARTESIAN_POINT('',(-90.8468254863551,36.3557395475489,107.791576552823));
#33125=CARTESIAN_POINT('',(-90.837184588187,36.355240425647,107.708423447177));
#33126=CARTESIAN_POINT('',(-90.8420555885722,36.3549260746838,124.208423447177));
#33127=CARTESIAN_POINT('',(-86.9747563060399,33.3857031209377,107.));
#33128=CARTESIAN_POINT('Ctrl Pts',(-90.8371845881871,36.355240425647,107.708423447177));
#33129=CARTESIAN_POINT('Ctrl Pts',(-90.8375044446039,36.8504159072854,107.682880329042));
#33130=CARTESIAN_POINT('Ctrl Pts',(-90.4912521582202,38.3657324511424,107.604687703175));
#33131=CARTESIAN_POINT('Ctrl Pts',(-88.1200899510646,39.9637873692998,107.473845569578));
#33132=CARTESIAN_POINT('Ctrl Pts',(-84.9365305796935,38.6233314502058,107.315897046385));
#33133=CARTESIAN_POINT('Ctrl Pts',(-84.3257621873457,35.2211429743639,107.157948523192));
#33134=CARTESIAN_POINT('Ctrl Pts',(-85.9925177162683,33.6482971733151,107.052649507731));
#33135=CARTESIAN_POINT('Ctrl Pts',(-86.97475630604,33.3857031209377,107.));
#33136=CARTESIAN_POINT('',(-88.5623548711056,33.385703120938,107.));
#33137=CARTESIAN_POINT('Origin',(-87.7685555885722,36.3549260746835,107.));
#33138=CARTESIAN_POINT('Ctrl Pts',(-90.8468254863551,36.3557395475489,107.791576552823));
#33139=CARTESIAN_POINT('Ctrl Pts',(-90.8469815553513,36.4002483891304,107.789262006108));
#33140=CARTESIAN_POINT('Ctrl Pts',(-90.826021840379,37.4570579042178,107.734297951662));
#33141=CARTESIAN_POINT('Ctrl Pts',(-89.6167529221334,39.4750891176184,107.626684389485));
#33142=CARTESIAN_POINT('Ctrl Pts',(-86.1660869151683,39.6084645219268,107.468735866293));
#33143=CARTESIAN_POINT('Ctrl Pts',(-84.1684778438722,36.7911512436696,107.310787343101));
#33144=CARTESIAN_POINT('Ctrl Pts',(-85.4209928151755,33.6146075800065,107.154542054336));
#33145=CARTESIAN_POINT('Ctrl Pts',(-87.6173026093478,33.1297337487181,107.050946273303));
#33146=CARTESIAN_POINT('Ctrl Pts',(-88.5642689721409,33.3806144275731,107.));
#33147=CARTESIAN_POINT('Origin',(-87.7685555885722,36.3549260746835,124.208423447177));
#33148=CARTESIAN_POINT('',(-90.8384672418802,36.3567914691884,108.791576552823));
#33149=CARTESIAN_POINT('',(-90.8436484209055,36.3523677969953,108.708423447177));
#33150=CARTESIAN_POINT('',(-90.8420555885722,36.3549260746838,124.208423447177));
#33151=CARTESIAN_POINT('Ctrl Pts',(-90.8436484209055,36.3523677969953,108.708423447177));
#33152=CARTESIAN_POINT('Ctrl Pts',(-90.8362605641932,37.1811158020221,108.665444042093));
#33153=CARTESIAN_POINT('Ctrl Pts',(-90.0646115445956,39.0372061661879,108.569815129278));
#33154=CARTESIAN_POINT('Ctrl Pts',(-86.9355577907939,39.8844991017031,108.421536708732));
#33155=CARTESIAN_POINT('Ctrl Pts',(-84.3576616569105,37.5869248418109,108.26358818554));
#33156=CARTESIAN_POINT('Ctrl Pts',(-84.8723856581236,34.1722681478534,108.105639662347));
#33157=CARTESIAN_POINT('Ctrl Pts',(-88.0128424134507,32.7366980213559,107.947691139155));
#33158=CARTESIAN_POINT('Ctrl Pts',(-90.4599970867152,34.2830646424737,107.815285734098));
#33159=CARTESIAN_POINT('Ctrl Pts',(-90.8368451561489,35.8297595719873,107.735529836772));
#33160=CARTESIAN_POINT('Ctrl Pts',(-90.8371845881871,36.355240425647,107.708423447177));
#33161=CARTESIAN_POINT('Ctrl Pts',(-90.8384672418802,36.3567914691884,108.791576552823));
#33162=CARTESIAN_POINT('Ctrl Pts',(-90.8406113732891,36.7392744389716,108.771825719159));
#33163=CARTESIAN_POINT('Ctrl Pts',(-90.5976169530331,38.1387104789577,108.699425377765));
#33164=CARTESIAN_POINT('Ctrl Pts',(-88.5106433716724,39.9047352467602,108.57437552864));
#33165=CARTESIAN_POINT('Ctrl Pts',(-85.2017900681466,38.9168748712948,108.416427005448));
#33166=CARTESIAN_POINT('Ctrl Pts',(-84.2201469451404,35.6061628091222,108.258478482255));
#33167=CARTESIAN_POINT('Ctrl Pts',(-86.4557340134341,32.9743534903137,108.100529959063));
#33168=CARTESIAN_POINT('Ctrl Pts',(-89.8314223830532,33.4012134097122,107.944895982585));
#33169=CARTESIAN_POINT('Ctrl Pts',(-90.8434314192628,35.3877958929954,107.841911513838));
#33170=CARTESIAN_POINT('Ctrl Pts',(-90.8468254863551,36.3557395475489,107.791576552823));
#33171=CARTESIAN_POINT('Origin',(-87.7685555885722,36.3549260746835,124.208423447177));
#33172=CARTESIAN_POINT('',(-90.8403904938695,36.3523334141797,109.791576552823));
#33173=CARTESIAN_POINT('',(-90.8446863688317,36.3571941258315,109.708423447177));
#33174=CARTESIAN_POINT('',(-90.8420555885722,36.3549260746838,124.208423447177));
#33175=CARTESIAN_POINT('Ctrl Pts',(-90.8446863688317,36.3571941258315,109.708423447177));
#33176=CARTESIAN_POINT('Ctrl Pts',(-90.8459254901998,36.5068138702629,109.700657262876));
#33177=CARTESIAN_POINT('Ctrl Pts',(-90.7682625972272,37.6694638143677,109.640241570843));
#33178=CARTESIAN_POINT('Ctrl Pts',(-89.2869055754696,39.648322843942,109.52717637108));
#33179=CARTESIAN_POINT('Ctrl Pts',(-85.8408549227417,39.4267036912455,109.369227847887));
#33180=CARTESIAN_POINT('Ctrl Pts',(-84.1425914088798,36.4199976257601,109.211279324695));
#33181=CARTESIAN_POINT('Ctrl Pts',(-85.7318802150827,33.3542922832663,109.053330801502));
#33182=CARTESIAN_POINT('Ctrl Pts',(-89.1677588360808,33.0091721504837,108.89538227831));
#33183=CARTESIAN_POINT('Ctrl Pts',(-90.7452905864005,34.9660088512056,108.780413160201));
#33184=CARTESIAN_POINT('Ctrl Pts',(-90.8453106433724,36.1659045767385,108.718093549824));
#33185=CARTESIAN_POINT('Ctrl Pts',(-90.8436484209055,36.3523677969953,108.708423447177));
#33186=CARTESIAN_POINT('Ctrl Pts',(-90.8403904938695,36.3523334141797,109.791576552823));
#33187=CARTESIAN_POINT('Ctrl Pts',(-90.8345310481531,37.0713395984218,109.754389432211));
#33188=CARTESIAN_POINT('Ctrl Pts',(-90.2253200935287,38.8172614473035,109.664552803868));
#33189=CARTESIAN_POINT('Ctrl Pts',(-87.325110594749,39.9542601161072,109.522066667795));
#33190=CARTESIAN_POINT('Ctrl Pts',(-84.512232678954,37.9512375795022,109.364118144602));
#33191=CARTESIAN_POINT('Ctrl Pts',(-84.6517637344715,34.5008878105768,109.20616962141));
#33192=CARTESIAN_POINT('Ctrl Pts',(-87.6171951182148,32.7315384366804,109.048221098217));
#33193=CARTESIAN_POINT('Ctrl Pts',(-90.331884593125,34.0578509090687,108.910023408688));
#33194=CARTESIAN_POINT('Ctrl Pts',(-90.8348957936273,35.7196951939743,108.82447522689));
#33195=CARTESIAN_POINT('Ctrl Pts',(-90.8384672418802,36.3567914691884,108.791576552823));
#33196=CARTESIAN_POINT('Origin',(-87.7685555885722,36.3549260746835,124.208423447177));
#33197=CARTESIAN_POINT('',(-90.8468972727246,36.3556108815869,110.791576552823));
#33198=CARTESIAN_POINT('',(-90.8372746968057,36.3552744910384,110.708423447177));
#33199=CARTESIAN_POINT('',(-90.8420555885722,36.3549260746838,124.208423447177));
#33200=CARTESIAN_POINT('Ctrl Pts',(-90.8372746968057,36.3552744910384,110.708423447177));
#33201=CARTESIAN_POINT('Ctrl Pts',(-90.8377739922262,36.8438059966829,110.683220975927));
#33202=CARTESIAN_POINT('Ctrl Pts',(-90.4981129378111,38.3522539474203,110.605368996946));
#33203=CARTESIAN_POINT('Ctrl Pts',(-88.1425881647719,39.9621339138956,110.474867510234));
#33204=CARTESIAN_POINT('Ctrl Pts',(-84.952526116541,38.6400577459963,110.316918987042));
#33205=CARTESIAN_POINT('Ctrl Pts',(-84.3156723392984,35.2461221965173,110.158970463849));
#33206=CARTESIAN_POINT('Ctrl Pts',(-86.8094428010696,32.8575053889834,110.001021940657));
#33207=CARTESIAN_POINT('Ctrl Pts',(-90.0074378666204,33.6014242611079,109.850839601766));
#33208=CARTESIAN_POINT('Ctrl Pts',(-90.8375250804865,35.4924926045081,109.753306770606));
#33209=CARTESIAN_POINT('Ctrl Pts',(-90.8446863688317,36.3571941258315,109.708423447177));
#33210=CARTESIAN_POINT('Ctrl Pts',(-90.8468972727246,36.3556108815869,110.791576552823));
#33211=CARTESIAN_POINT('Ctrl Pts',(-90.8470129167021,36.3935671709611,110.789602652993));
#33212=CARTESIAN_POINT('Ctrl Pts',(-90.8292489756467,37.4438146379521,110.734979245433));
#33213=CARTESIAN_POINT('Ctrl Pts',(-89.6367303689711,39.4632652024454,110.627706330142));
#33214=CARTESIAN_POINT('Ctrl Pts',(-86.1870500209474,39.6184654540127,110.46975780695));
#33215=CARTESIAN_POINT('Ctrl Pts',(-84.1712726716061,36.8147138073089,110.311809283757));
#33216=CARTESIAN_POINT('Ctrl Pts',(-85.417042337004,33.594086605388,110.153860760565));
#33217=CARTESIAN_POINT('Ctrl Pts',(-88.7948575488562,32.8766285869604,109.995912237372));
#33218=CARTESIAN_POINT('Ctrl Pts',(-90.665968377309,34.7392604855723,109.875150834792));
#33219=CARTESIAN_POINT('Ctrl Pts',(-90.8428268486203,36.0533709836683,109.807038939942));
#33220=CARTESIAN_POINT('Ctrl Pts',(-90.8403904938695,36.3523334141797,109.791576552823));
#33221=CARTESIAN_POINT('Origin',(-87.7685555885722,36.3549260746835,124.208423447177));
#33222=CARTESIAN_POINT('',(-90.8385928893407,36.3568681301786,111.791576552823));
#33223=CARTESIAN_POINT('',(-90.8434554977008,36.3523302811269,111.708423447177));
#33224=CARTESIAN_POINT('',(-90.8420555885722,36.3549260746838,124.208423447177));
#33225=CARTESIAN_POINT('Ctrl Pts',(-90.8434554977008,36.3523302811269,111.708423447177));
#33226=CARTESIAN_POINT('Ctrl Pts',(-90.8360746186667,37.174642245983,111.665784688979));
#33227=CARTESIAN_POINT('Ctrl Pts',(-90.0746147106792,39.0243970272075,111.570496423049));
#33228=CARTESIAN_POINT('Ctrl Pts',(-86.9582295306161,39.8897839838954,111.422558649389));
#33229=CARTESIAN_POINT('Ctrl Pts',(-84.3656607621669,37.6087823498066,111.264610126197));
#33230=CARTESIAN_POINT('Ctrl Pts',(-84.858393238377,34.1909473654533,111.106661603004));
#33231=CARTESIAN_POINT('Ctrl Pts',(-87.9896814090755,32.7351260621679,110.948713079812));
#33232=CARTESIAN_POINT('Ctrl Pts',(-90.4528392552173,34.269885868269,110.815967027869));
#33233=CARTESIAN_POINT('Ctrl Pts',(-90.8367309334783,35.8232337270908,110.735870483658));
#33234=CARTESIAN_POINT('Ctrl Pts',(-90.8372746968057,36.3552744910384,110.708423447177));
#33235=CARTESIAN_POINT('Ctrl Pts',(-90.8385928893406,36.3568681301786,111.791576552823));
#33236=CARTESIAN_POINT('Ctrl Pts',(-90.8407925664026,36.7327156432091,111.772166366045));
#33237=CARTESIAN_POINT('Ctrl Pts',(-90.6033582589985,38.1253552741901,111.700106671536));
#33238=CARTESIAN_POINT('Ctrl Pts',(-88.5334211413281,39.8998985469101,111.575397469297));
#33239=CARTESIAN_POINT('Ctrl Pts',(-85.2182937675741,38.9333003273795,111.417448946105));
#33240=CARTESIAN_POINT('Ctrl Pts',(-84.21541122421,35.6289685906495,111.259500422912));
#33241=CARTESIAN_POINT('Ctrl Pts',(-86.4340566120166,32.9828404256698,111.10155189972));
#33242=CARTESIAN_POINT('Ctrl Pts',(-89.8198041109555,33.3889404587613,110.945577276356));
#33243=CARTESIAN_POINT('Ctrl Pts',(-90.8439283637791,35.3811652642377,110.842252160724));
#33244=CARTESIAN_POINT('Ctrl Pts',(-90.8468972727246,36.3556108815869,110.791576552823));
#33245=CARTESIAN_POINT('Origin',(-87.7685555885722,36.3549260746835,124.208423447177));
#33246=CARTESIAN_POINT('',(-90.8402144015523,36.3523700744382,112.791576552823));
#33247=CARTESIAN_POINT('',(-90.8448621506013,36.3571283696629,112.708423447177));
#33248=CARTESIAN_POINT('',(-90.8420555885722,36.3549260746838,124.208423447177));
#33249=CARTESIAN_POINT('Ctrl Pts',(-90.8448621506013,36.3571283696629,112.708423447177));
#33250=CARTESIAN_POINT('Ctrl Pts',(-90.8460230140249,36.5001640472249,112.700997909761));
#33251=CARTESIAN_POINT('Ctrl Pts',(-90.7722166884106,37.6561661169679,112.640922864614));
#33252=CARTESIAN_POINT('Ctrl Pts',(-89.3080212269955,39.6385055706828,112.528198311736));
#33253=CARTESIAN_POINT('Ctrl Pts',(-85.8606184245708,39.4390182485099,112.370249788544));
#33254=CARTESIAN_POINT('Ctrl Pts',(-84.1430842214608,36.4432783507515,112.212301265351));
#33255=CARTESIAN_POINT('Ctrl Pts',(-85.7126546431824,33.3674321313963,112.054352742159));
#33256=CARTESIAN_POINT('Ctrl Pts',(-89.1462479246903,33.0002558098966,111.896404218967));
#33257=CARTESIAN_POINT('Ctrl Pts',(-90.7410210066454,34.9526930047544,111.781094453973));
#33258=CARTESIAN_POINT('Ctrl Pts',(-90.8451883842683,36.1592674560054,111.71843419671));
#33259=CARTESIAN_POINT('Ctrl Pts',(-90.8434554977008,36.3523302811269,111.708423447177));
#33260=CARTESIAN_POINT('Ctrl Pts',(-90.8402144015524,36.3523700744382,112.791576552823));
#33261=CARTESIAN_POINT('Ctrl Pts',(-90.8345153488798,37.064893455906,112.754730079097));
#33262=CARTESIAN_POINT('Ctrl Pts',(-90.2341640589546,38.8041985290923,112.66523409764));
#33263=CARTESIAN_POINT('Ctrl Pts',(-87.3482310510782,39.957033294882,112.523088608452));
#33264=CARTESIAN_POINT('Ctrl Pts',(-84.5225497279198,37.9721134773169,112.365140085259));
#33265=CARTESIAN_POINT('Ctrl Pts',(-84.6399231958095,34.5209390263157,112.207191562067));
#33266=CARTESIAN_POINT('Ctrl Pts',(-87.5939325011642,32.7325848538746,112.049243038874));
#33267=CARTESIAN_POINT('Ctrl Pts',(-90.3237945448813,34.0446656332115,111.91070470246));
#33268=CARTESIAN_POINT('Ctrl Pts',(-90.8348260130765,35.7132413450188,111.824815873776));
#33269=CARTESIAN_POINT('Ctrl Pts',(-90.8385928893406,36.3568681301786,111.791576552823));
#33270=CARTESIAN_POINT('Origin',(-87.7685555885722,36.3549260746835,124.208423447177));
#33271=CARTESIAN_POINT('',(-90.8469565090695,36.3554949864144,113.791576552823));
#33272=CARTESIAN_POINT('',(-90.8373005739091,36.3553794097185,113.708423447177));
#33273=CARTESIAN_POINT('',(-90.8420555885722,36.3549260746838,124.208423447177));
#33274=CARTESIAN_POINT('Ctrl Pts',(-90.8373005739091,36.3553794097185,113.708423447178));
#33275=CARTESIAN_POINT('Ctrl Pts',(-90.8379417505728,36.8372975674189,113.683561622813));
#33276=CARTESIAN_POINT('Ctrl Pts',(-90.5047600111548,38.338927938775,113.606050290717));
#33277=CARTESIAN_POINT('Ctrl Pts',(-88.16574233066,39.9596578886113,113.475889450891));
#33278=CARTESIAN_POINT('Ctrl Pts',(-84.9672569937481,38.6580923607057,113.317940927699));
#33279=CARTESIAN_POINT('Ctrl Pts',(-84.3086238951178,35.2683160089,113.159992404506));
#33280=CARTESIAN_POINT('Ctrl Pts',(-86.7870056338769,32.863735955989,113.002043881314));
#33281=CARTESIAN_POINT('Ctrl Pts',(-89.99697594205,33.5887459138352,112.851520895538));
#33282=CARTESIAN_POINT('Ctrl Pts',(-90.8377921097319,35.485993948889,112.753647417492));
#33283=CARTESIAN_POINT('Ctrl Pts',(-90.8448621506013,36.3571283696629,112.708423447177));
#33284=CARTESIAN_POINT('Ctrl Pts',(-90.8469565090695,36.3554949864144,113.791576552823));
#33285=CARTESIAN_POINT('Ctrl Pts',(-90.8470371923431,36.38689932666,113.789943299879));
#33286=CARTESIAN_POINT('Ctrl Pts',(-90.8324320241331,37.4305764646951,113.735660539204));
#33287=CARTESIAN_POINT('Ctrl Pts',(-89.6566504974584,39.4512055771937,113.628728270799));
#33288=CARTESIAN_POINT('Ctrl Pts',(-86.2080378044846,39.6285530216908,113.470779747607));
#33289=CARTESIAN_POINT('Ctrl Pts',(-84.1742991253402,36.8378024761994,113.312831224414));
#33290=CARTESIAN_POINT('Ctrl Pts',(-85.3993634670394,33.6092425834755,113.154882701222));
#33291=CARTESIAN_POINT('Ctrl Pts',(-88.7725022496111,32.8701104060413,112.996934178029));
#33292=CARTESIAN_POINT('Ctrl Pts',(-90.6608461669204,34.7259096736242,112.875832128563));
#33293=CARTESIAN_POINT('Ctrl Pts',(-90.8426586605023,36.0467768904004,112.807379586827));
#33294=CARTESIAN_POINT('Ctrl Pts',(-90.8402144015524,36.3523700744382,112.791576552823));
#33295=CARTESIAN_POINT('Origin',(-87.7685555885722,36.3549260746835,124.208423447177));
#33296=CARTESIAN_POINT('',(-90.8387237914782,36.3569420805603,114.791576552823));
#33297=CARTESIAN_POINT('',(-90.8432613144075,36.3522971348084,114.708423447177));
#33298=CARTESIAN_POINT('',(-90.8420555885722,36.3549260746838,124.208423447177));
#33299=CARTESIAN_POINT('Ctrl Pts',(-90.8432613144075,36.3522971348084,114.708423447177));
#33300=CARTESIAN_POINT('Ctrl Pts',(-90.8358994837641,37.1681724947489,114.666125335864));
#33301=CARTESIAN_POINT('Ctrl Pts',(-90.0845448816577,39.0115735013954,114.571177716821));
#33302=CARTESIAN_POINT('Ctrl Pts',(-86.9809435523238,39.8949142157357,114.423580590046));
#33303=CARTESIAN_POINT('Ctrl Pts',(-84.373781921353,37.630606484029,114.265632066854));
#33304=CARTESIAN_POINT('Ctrl Pts',(-84.8445583270759,34.2096781232347,114.107683543661));
#33305=CARTESIAN_POINT('Ctrl Pts',(-87.9664341204409,32.7337808352518,113.949735020469));
#33306=CARTESIAN_POINT('Ctrl Pts',(-90.445741881575,34.256590833291,113.816648321641));
#33307=CARTESIAN_POINT('Ctrl Pts',(-90.8365839404934,35.8167468066471,113.736211130544));
#33308=CARTESIAN_POINT('Ctrl Pts',(-90.8373005739091,36.3553794097185,113.708423447178));
#33309=CARTESIAN_POINT('Ctrl Pts',(-90.8387237914782,36.3569420805603,114.791576552823));
#33310=CARTESIAN_POINT('Ctrl Pts',(-90.8409732941709,36.7261539149222,114.772507012931));
#33311=CARTESIAN_POINT('Ctrl Pts',(-90.6090448889861,38.1119999363053,114.700787965308));
#33312=CARTESIAN_POINT('Ctrl Pts',(-88.5561676363232,39.8949142674411,114.576419409954));
#33313=CARTESIAN_POINT('Ctrl Pts',(-85.2349020777131,38.9496224017201,114.418470886762));
#33314=CARTESIAN_POINT('Ctrl Pts',(-84.2108230998106,35.6517982903965,114.260522363569));
#33315=CARTESIAN_POINT('Ctrl Pts',(-86.412431965926,32.9914787564211,114.102573840377));
#33316=CARTESIAN_POINT('Ctrl Pts',(-89.8081172142279,33.3766699586493,113.946258570128));
#33317=CARTESIAN_POINT('Ctrl Pts',(-90.8444362880251,35.3745496713466,113.84259280761));
#33318=CARTESIAN_POINT('Ctrl Pts',(-90.8469565090695,36.3554949864144,113.791576552823));
#33319=CARTESIAN_POINT('Origin',(-87.7685555885722,36.3549260746835,124.208423447177));
#33320=CARTESIAN_POINT('',(-90.8400416161831,36.3524106996081,115.791576552823));
#33321=CARTESIAN_POINT('',(-90.845034052782,36.3570585842589,115.708423447177));
#33322=CARTESIAN_POINT('',(-90.8420555885722,36.3549260746838,124.208423447177));
#33323=CARTESIAN_POINT('Ctrl Pts',(-90.845034052782,36.3570585842589,115.708423447177));
#33324=CARTESIAN_POINT('Ctrl Pts',(-90.8461165882359,36.4935125756602,115.701338556647));
#33325=CARTESIAN_POINT('Ctrl Pts',(-90.7761238734907,37.6428715883725,115.641604158386));
#33326=CARTESIAN_POINT('Ctrl Pts',(-89.3290733498657,39.6285529738767,115.529220252393));
#33327=CARTESIAN_POINT('Ctrl Pts',(-85.8804607072626,39.4512055319686,115.371271729201));
#33328=CARTESIAN_POINT('Ctrl Pts',(-84.143726269733,36.466555675223,115.213323206008));
#33329=CARTESIAN_POINT('Ctrl Pts',(-85.6935143313946,33.3806946547291,115.055374682816));
#33330=CARTESIAN_POINT('Ctrl Pts',(-89.1246791914122,32.9914788055483,114.897426159624));
#33331=CARTESIAN_POINT('Ctrl Pts',(-90.7367041935985,34.939373215214,114.781775747744));
#33332=CARTESIAN_POINT('Ctrl Pts',(-90.8450629368673,36.1526322085003,114.718774843595));
#33333=CARTESIAN_POINT('Ctrl Pts',(-90.8432613144075,36.3522971348084,114.708423447177));
#33334=CARTESIAN_POINT('Ctrl Pts',(-90.8400416161831,36.3524106996081,115.791576552823));
#33335=CARTESIAN_POINT('Ctrl Pts',(-90.8345080235632,37.058447369207,115.755070725982));
#33336=CARTESIAN_POINT('Ctrl Pts',(-90.242941846011,38.7911234504317,115.665915391411));
#33337=CARTESIAN_POINT('Ctrl Pts',(-87.3713688406819,39.959657941262,115.524110549109));
#33338=CARTESIAN_POINT('Ctrl Pts',(-84.5330006014756,37.9929227377143,115.366162025916));
#33339=CARTESIAN_POINT('Ctrl Pts',(-84.6282116641132,34.5410657772132,115.208213502724));
#33340=CARTESIAN_POINT('Ctrl Pts',(-87.5706770538148,32.7337807823612,115.050264979531));
#33341=CARTESIAN_POINT('Ctrl Pts',(-90.3156406263894,34.0314891348168,114.911385996231));
#33342=CARTESIAN_POINT('Ctrl Pts',(-90.8347625932267,35.7067889256462,114.825156520661));
#33343=CARTESIAN_POINT('Ctrl Pts',(-90.8387237914782,36.3569420805603,114.791576552823));
#33344=CARTESIAN_POINT('Origin',(-87.7685555885722,36.3549260746835,124.208423447177));
#33345=CARTESIAN_POINT('',(-90.8470054143286,36.355377816704,116.791576552823));
#33346=CARTESIAN_POINT('',(-90.8373332185204,36.3554836682631,116.708423447177));
#33347=CARTESIAN_POINT('',(-90.8420555885722,36.3549260746838,124.208423447177));
#33348=CARTESIAN_POINT('Ctrl Pts',(-90.8373332185204,36.3554836682631,116.708423447177));
#33349=CARTESIAN_POINT('Ctrl Pts',(-90.8381115230835,36.8307861352947,116.683902269698));
#33350=CARTESIAN_POINT('Ctrl Pts',(-90.5113487431761,38.3255987424985,116.606731584489));
#33351=CARTESIAN_POINT('Ctrl Pts',(-88.1888801199258,39.9570332422698,116.476911391548));
#33352=CARTESIAN_POINT('Ctrl Pts',(-84.9821033690532,38.6760320151288,116.318962868356));
#33353=CARTESIAN_POINT('Ctrl Pts',(-84.3017180995052,35.2905546250324,116.161014345163));
#33354=CARTESIAN_POINT('Ctrl Pts',(-86.7646089421984,32.8701104569402,116.003065821971));
#33355=CARTESIAN_POINT('Ctrl Pts',(-89.9864431986579,33.5760883377251,115.852202189309));
#33356=CARTESIAN_POINT('Ctrl Pts',(-90.8380720096351,35.4794904896189,115.753988064378));
#33357=CARTESIAN_POINT('Ctrl Pts',(-90.845034052782,36.3570585842589,115.708423447177));
#33358=CARTESIAN_POINT('Ctrl Pts',(-90.8470054143286,36.355377816704,116.791576552823));
#33359=CARTESIAN_POINT('Ctrl Pts',(-90.8470569015836,36.3802311058533,116.790283946765));
#33360=CARTESIAN_POINT('Ctrl Pts',(-90.8355714137741,37.4173420438333,116.736341832976));
#33361=CARTESIAN_POINT('Ctrl Pts',(-89.6764927804399,39.4390182935569,116.629750211456));
#33362=CARTESIAN_POINT('Ctrl Pts',(-86.2290899276622,39.6385056186423,116.471801688264));
#33363=CARTESIAN_POINT('Ctrl Pts',(-84.1774737689002,36.8608712367781,116.313853165071));
#33364=CARTESIAN_POINT('Ctrl Pts',(-85.3817822782182,33.6245117640691,116.155904641879));
#33365=CARTESIAN_POINT('Ctrl Pts',(-88.7501055576055,32.8637359049969,115.997956118686));
#33366=CARTESIAN_POINT('Ctrl Pts',(-90.6556717462417,34.7125578096458,115.876513422334));
#33367=CARTESIAN_POINT('Ctrl Pts',(-90.8424886927505,36.0401857295852,115.807720233713));
#33368=CARTESIAN_POINT('Ctrl Pts',(-90.8400416161831,36.3524106996081,115.791576552823));
#33369=CARTESIAN_POINT('Origin',(-87.7685555885722,36.3549260746835,124.208423447177));
#33370=CARTESIAN_POINT('',(-90.8388598290993,36.3570130097889,117.791576552823));
#33371=CARTESIAN_POINT('',(-90.8430661113431,36.3522684582546,117.708423447177));
#33372=CARTESIAN_POINT('',(-90.8420555885722,36.3549260746838,124.208423447177));
#33373=CARTESIAN_POINT('Ctrl Pts',(-90.8430661113431,36.3522684582546,117.708423447177));
#33374=CARTESIAN_POINT('Ctrl Pts',(-90.8357356935995,37.1617056224215,117.66646598275));
#33375=CARTESIAN_POINT('Ctrl Pts',(-90.0944057462884,38.9987324296382,117.571859010592));
#33376=CARTESIAN_POINT('Ctrl Pts',(-87.0036900469868,39.8998984951319,117.424602530703));
#33377=CARTESIAN_POINT('Ctrl Pts',(-84.3820430458739,37.6523780223793,117.26665400751));
#33378=CARTESIAN_POINT('Ctrl Pts',(-84.8308439711031,34.228497328871,117.108705484318));
#33379=CARTESIAN_POINT('Ctrl Pts',(-87.9431786734311,32.7325849067827,116.950756961125));
#33380=CARTESIAN_POINT('Ctrl Pts',(-90.4385841834224,34.2433008167291,116.817329615412));
#33381=CARTESIAN_POINT('Ctrl Pts',(-90.8364404225768,35.8102625110144,116.736551777429));
#33382=CARTESIAN_POINT('Ctrl Pts',(-90.8373332185204,36.3554836682631,116.708423447177));
#33383=CARTESIAN_POINT('Ctrl Pts',(-90.8388598290993,36.3570130097889,117.791576552823));
#33384=CARTESIAN_POINT('Ctrl Pts',(-90.8411534611211,36.7195890353653,117.772847659816));
#33385=CARTESIAN_POINT('Ctrl Pts',(-90.6146771194904,38.0986443635484,117.701469259079));
#33386=CARTESIAN_POINT('Ctrl Pts',(-88.5788816583627,39.8897840355259,117.577441350611));
#33387=CARTESIAN_POINT('Ctrl Pts',(-85.2516148494836,38.9658374976431,117.419492827418));
#33388=CARTESIAN_POINT('Ctrl Pts',(-84.2063816594615,35.6746569798619,117.261544304226));
#33389=CARTESIAN_POINT('Ctrl Pts',(-86.3908632323328,33.0002557608977,117.103595781033));
#33390=CARTESIAN_POINT('Ctrl Pts',(-89.7963570069237,33.3644272205121,116.946939863899));
#33391=CARTESIAN_POINT('Ctrl Pts',(-90.8449597594478,35.3679246640809,116.842933454495));
#33392=CARTESIAN_POINT('Ctrl Pts',(-90.8470054143286,36.355377816704,116.791576552823));
#33393=CARTESIAN_POINT('Origin',(-87.7685555885722,36.3549260746835,124.208423447177));
#33394=CARTESIAN_POINT('',(-90.8398723581442,36.3524552105476,118.791576552823));
#33395=CARTESIAN_POINT('',(-90.8452017125077,36.3569848687002,118.708423447177));
#33396=CARTESIAN_POINT('',(-90.8420555885722,36.3549260746838,124.208423447177));
#33397=CARTESIAN_POINT('Ctrl Pts',(-90.8452017125077,36.3569848687002,118.708423447177));
#33398=CARTESIAN_POINT('Ctrl Pts',(-90.8462061475006,36.4868595329243,118.701679203533));
#33399=CARTESIAN_POINT('Ctrl Pts',(-90.7799843510519,37.6295802855217,118.642285452157));
#33400=CARTESIAN_POINT('Ctrl Pts',(-89.3500611330962,39.6184654063458,118.53024219305));
#33401=CARTESIAN_POINT('Ctrl Pts',(-85.9003808354589,39.4632651570443,118.372293669858));
#33402=CARTESIAN_POINT('Ctrl Pts',(-84.144517768422,36.4898283971866,118.214345146665));
#33403=CARTESIAN_POINT('Ctrl Pts',(-85.6744595728268,33.3940798045978,118.056396623473));
#33404=CARTESIAN_POINT('Ctrl Pts',(-89.1030545456374,32.9828404749231,117.89844810028));
#33405=CARTESIAN_POINT('Ctrl Pts',(-90.7323386857844,34.9260508120483,117.782457041515));
#33406=CARTESIAN_POINT('Ctrl Pts',(-90.8449341256527,36.1459991488762,117.719115490481));
#33407=CARTESIAN_POINT('Ctrl Pts',(-90.8430661113431,36.3522684582546,117.708423447177));
#33408=CARTESIAN_POINT('Ctrl Pts',(-90.8398723581442,36.3524552105476,118.791576552823));
#33409=CARTESIAN_POINT('Ctrl Pts',(-90.8345088849513,37.052001191776,118.755411372868));
#33410=CARTESIAN_POINT('Ctrl Pts',(-90.2516536622113,38.7780365130427,118.666596685182));
#33411=CARTESIAN_POINT('Ctrl Pts',(-87.394523006908,39.962133966582,118.525132489766));
#33412=CARTESIAN_POINT('Ctrl Pts',(-84.5435848754497,38.0136644637222,118.367183966573));
#33413=CARTESIAN_POINT('Ctrl Pts',(-84.6166296078616,34.5612673131065,118.209235443381));
#33414=CARTESIAN_POINT('Ctrl Pts',(-87.5474297648405,32.7351260092969,118.051286920188));
#33415=CARTESIAN_POINT('Ctrl Pts',(-90.3074225693738,34.0183219665893,117.912067290002));
#33416=CARTESIAN_POINT('Ctrl Pts',(-90.8347057443862,35.7003376970687,117.825497167547));
#33417=CARTESIAN_POINT('Ctrl Pts',(-90.8388598290993,36.3570130097889,117.791576552823));
#33418=CARTESIAN_POINT('Origin',(-87.7685555885722,36.3549260746835,124.208423447177));
#33419=CARTESIAN_POINT('',(-90.8470436441738,36.3552596744299,119.791576552823));
#33420=CARTESIAN_POINT('',(-90.8373725915384,36.3555871000405,119.708423447177));
#33421=CARTESIAN_POINT('',(-90.8420555885722,36.3549260746838,124.208423447177));
#33422=CARTESIAN_POINT('Ctrl Pts',(-90.8373725915384,36.3555871000405,119.708423447177));
#33423=CARTESIAN_POINT('Ctrl Pts',(-90.8382831445492,36.8242716643461,119.684242916584));
#33424=CARTESIAN_POINT('Ctrl Pts',(-90.5178793708824,38.3122665852445,119.60741287826));
#33425=CARTESIAN_POINT('Ctrl Pts',(-88.2120005759172,39.9542600635284,119.477933332205));
#33426=CARTESIAN_POINT('Ctrl Pts',(-84.9970646304694,38.6938759803182,119.319984809012));
#33427=CARTESIAN_POINT('Ctrl Pts',(-84.2949552395589,35.3128371203772,119.16203628582));
#33428=CARTESIAN_POINT('Ctrl Pts',(-86.7422536432798,32.8766286377651,119.004087762628));
#33429=CARTESIAN_POINT('Ctrl Pts',(-89.9758394835887,33.5634519078074,118.85288348308));
#33430=CARTESIAN_POINT('Ctrl Pts',(-90.8383649408792,35.4729819955614,118.754328711263));
#33431=CARTESIAN_POINT('Ctrl Pts',(-90.8452017125077,36.3569848687002,118.708423447177));
#33432=CARTESIAN_POINT('Ctrl Pts',(-90.8470436441738,36.3552596744299,119.791576552823));
#33433=CARTESIAN_POINT('Ctrl Pts',(-90.847072089005,36.3735626432968,119.79062459365));
#33434=CARTESIAN_POINT('Ctrl Pts',(-90.8386674461304,37.4041115135856,119.737023126747));
#33435=CARTESIAN_POINT('Ctrl Pts',(-89.6962562825846,39.4267037361566,119.630772152113));
#33436=CARTESIAN_POINT('Ctrl Pts',(-86.2502055794825,39.6483228920224,119.47282362892));
#33437=CARTESIAN_POINT('Ctrl Pts',(-84.1807964437643,36.8839191095796,119.314875105728));
#33438=CARTESIAN_POINT('Ctrl Pts',(-85.3642995086962,33.6398935322125,119.156926582536));
#33439=CARTESIAN_POINT('Ctrl Pts',(-88.727668390087,32.8575053379033,118.998978059343));
#33440=CARTESIAN_POINT('Ctrl Pts',(-90.650444889663,34.6992050189384,118.877194716105));
#33441=CARTESIAN_POINT('Ctrl Pts',(-90.8423170646337,36.0335975340926,118.808060880599));
#33442=CARTESIAN_POINT('Ctrl Pts',(-90.8398723581442,36.3524552105476,118.791576552823));
#33443=CARTESIAN_POINT('Origin',(-87.7685555885722,36.3549260746835,124.208423447177));
#33444=CARTESIAN_POINT('',(-90.8389970126702,36.3570769587632,120.791576552823));
#33445=CARTESIAN_POINT('',(-90.84286984995,36.3522423553315,120.708423447177));
#33446=CARTESIAN_POINT('',(-90.8420555885722,36.3549260746838,124.208423447177));
#33447=CARTESIAN_POINT('Ctrl Pts',(-90.84286984995,36.3522423553315,120.708423447177));
#33448=CARTESIAN_POINT('Ctrl Pts',(-90.8355827220701,37.1552395412463,120.666806629636));
#33449=CARTESIAN_POINT('Ctrl Pts',(-90.1041979681009,38.9858767921816,120.572540304363));
#33450=CARTESIAN_POINT('Ctrl Pts',(-87.0264678163487,39.9047351945452,120.42562447136));
#33451=CARTESIAN_POINT('Ctrl Pts',(-84.3904439217461,37.6740967587225,120.267675948167));
#33452=CARTESIAN_POINT('Ctrl Pts',(-84.8172506743583,34.2474038701722,120.109727424975));
#33453=CARTESIAN_POINT('Ctrl Pts',(-87.9199160567175,32.7315384896552,119.951778901782));
#33454=CARTESIAN_POINT('Ctrl Pts',(-90.431365923944,34.2300160043642,119.818010909183));
#33455=CARTESIAN_POINT('Ctrl Pts',(-90.8363005508424,35.8037807575614,119.736892424315));
#33456=CARTESIAN_POINT('Ctrl Pts',(-90.8373725915384,36.3555871000405,119.708423447177));
#33457=CARTESIAN_POINT('Ctrl Pts',(-90.8389970126702,36.3570769587632,120.791576552823));
#33458=CARTESIAN_POINT('Ctrl Pts',(-90.8413323422268,36.7130204263635,120.773188306702));
#33459=CARTESIAN_POINT('Ctrl Pts',(-90.6202675433234,38.0853011148081,120.70215055285));
#33460=CARTESIAN_POINT('Ctrl Pts',(-88.601553399534,39.8844991555637,120.578463291268));
#33461=CARTESIAN_POINT('Ctrl Pts',(-85.2684357075705,38.981949277713,120.420514768075));
#33462=CARTESIAN_POINT('Ctrl Pts',(-84.202084988714,35.697541610575,120.262566244883));
#33463=CARTESIAN_POINT('Ctrl Pts',(-86.3693523204529,33.0091721012914,120.10461772169));
#33464=CARTESIAN_POINT('Ctrl Pts',(-89.7845228766894,33.3522121930534,119.94762115767));
#33465=CARTESIAN_POINT('Ctrl Pts',(-90.8454989056133,35.3612899231855,119.843274101381));
#33466=CARTESIAN_POINT('Ctrl Pts',(-90.8470436441738,36.3552596744299,119.791576552823));
#33467=CARTESIAN_POINT('Origin',(-87.7685555885722,36.3549260746835,124.208423447177));
#33468=CARTESIAN_POINT('',(-90.8388342008425,36.3519111454271,121.791576552823));
#33469=CARTESIAN_POINT('',(-90.8453550251769,36.3568536361305,121.708423447177));
#33470=CARTESIAN_POINT('',(-90.8420555885722,36.3549260746838,124.208423447177));
#33471=CARTESIAN_POINT('',(-88.5623548711056,33.385703120938,122.));
#33472=CARTESIAN_POINT('Ctrl Pts',(-88.5623548711056,33.385703120938,122.));
#33473=CARTESIAN_POINT('Ctrl Pts',(-89.5445934608772,33.6482971733158,121.947350492269));
#33474=CARTESIAN_POINT('Ctrl Pts',(-90.6442900920727,34.6860341601982,121.877876009877));
#33475=CARTESIAN_POINT('Ctrl Pts',(-90.8411753710437,36.0264353653473,121.808401527484));
#33476=CARTESIAN_POINT('Ctrl Pts',(-90.8388342008425,36.3519111454271,121.791576552823));
#33477=CARTESIAN_POINT('',(-86.9728468550288,33.380626780384,122.));
#33478=CARTESIAN_POINT('Origin',(-87.7685555885722,36.3549260746835,122.));
#33479=CARTESIAN_POINT('Ctrl Pts',(-86.972842220194,33.3806144585182,122.));
#33480=CARTESIAN_POINT('Ctrl Pts',(-87.9198086173169,33.1297337454483,121.949053726697));
#33481=CARTESIAN_POINT('Ctrl Pts',(-89.9803571320055,33.5846360429098,121.851861542423));
#33482=CARTESIAN_POINT('Ctrl Pts',(-90.8386915121384,35.4665790111915,121.754669358149));
#33483=CARTESIAN_POINT('Ctrl Pts',(-90.8453550251768,36.3568536361305,121.708423447177));
#33484=CARTESIAN_POINT('Origin',(87.7685555885722,-36.3549260746835,114.));
#33485=CARTESIAN_POINT('',(85.2550452373729,-36.354668632511,107.387416697508));
#33486=CARTESIAN_POINT('',(85.2529645136107,-36.3584982898635,107.112583302492));
#33487=CARTESIAN_POINT('',(85.2510555885723,-36.3549260746835,114.));
#33488=CARTESIAN_POINT('',(85.8550895919076,-34.7189388713081,107.));
#33489=CARTESIAN_POINT('Ctrl Pts',(85.2529645136107,-36.3584982898635,107.112583302492));
#33490=CARTESIAN_POINT('Ctrl Pts',(85.2581100669596,-35.7658638142766,107.075055534995));
#33491=CARTESIAN_POINT('Ctrl Pts',(85.4693337604884,-35.1701225143786,107.037527767497));
#33492=CARTESIAN_POINT('Ctrl Pts',(85.8550895919077,-34.718938871308,107.));
#33493=CARTESIAN_POINT('',(85.2510555885723,-36.3549260746835,107.));
#33494=CARTESIAN_POINT('Origin',(87.7685555885722,-36.3549260746835,107.));
#33495=CARTESIAN_POINT('',(85.2510555885723,-36.3549260746835,106.));
#33496=CARTESIAN_POINT('',(85.2510555885723,-36.3549260746835,114.));
#33497=CARTESIAN_POINT('Origin',(87.7685555885722,-36.3549260746835,106.));
#33498=CARTESIAN_POINT('',(89.6856659018966,-34.7163980987228,107.));
#33499=CARTESIAN_POINT('Origin',(87.7685555885722,-36.3549260746835,107.));
#33500=CARTESIAN_POINT('Ctrl Pts',(89.685674748321,-34.7163919311049,107.));
#33501=CARTESIAN_POINT('Ctrl Pts',(89.1628542081215,-34.1076769579869,107.050946273303));
#33502=CARTESIAN_POINT('Ctrl Pts',(88.3231296580498,-33.7675004276397,107.101892546605));
#33503=CARTESIAN_POINT('Ctrl Pts',(87.5244587616235,-33.8452631801865,107.152838819908));
#33504=CARTESIAN_POINT('Ctrl Pts',(86.6990867214356,-33.9256256949687,107.205488327639));
#33505=CARTESIAN_POINT('Ctrl Pts',(85.9175592297027,-34.4523396916042,107.25813783537));
#33506=CARTESIAN_POINT('Ctrl Pts',(85.5336746027685,-35.1871265063861,107.3107873431));
#33507=CARTESIAN_POINT('Ctrl Pts',(85.3474314487688,-35.5436112528458,107.336330461236));
#33508=CARTESIAN_POINT('Ctrl Pts',(85.2547832386249,-35.9490710104433,107.361873579372));
#33509=CARTESIAN_POINT('Ctrl Pts',(85.2550452373729,-36.354668632511,107.387416697508));
#33510=CARTESIAN_POINT('Origin',(87.7685555885722,-36.3549260746835,114.));
#33511=CARTESIAN_POINT('',(85.2497507212102,-36.3570215567107,108.387416697508));
#33512=CARTESIAN_POINT('',(85.2471487745657,-36.3542597485476,108.112583302492));
#33513=CARTESIAN_POINT('',(85.2510555885723,-36.3549260746835,114.));
#33514=CARTESIAN_POINT('Ctrl Pts',(85.2471487745657,-36.3542597485476,108.112583302492));
#33515=CARTESIAN_POINT('Ctrl Pts',(85.2470209387648,-36.3178026153987,108.110268755777));
#33516=CARTESIAN_POINT('Ctrl Pts',(85.2477438897639,-36.2813507190277,108.107954209062));
#33517=CARTESIAN_POINT('Ctrl Pts',(85.2493335062549,-36.2449367209381,108.105639662347));
#33518=CARTESIAN_POINT('Ctrl Pts',(85.2854928653183,-35.4166194259904,108.052990154616));
#33519=CARTESIAN_POINT('Ctrl Pts',(85.7700962403271,-34.6079120701247,108.000340646886));
#33520=CARTESIAN_POINT('Ctrl Pts',(86.483470577241,-34.1853504230939,107.947691139155));
#33521=CARTESIAN_POINT('Ctrl Pts',(87.1968449141549,-33.762788776063,107.895041631424));
#33522=CARTESIAN_POINT('Ctrl Pts',(88.1389902129737,-33.726372837867,107.842392123693));
#33523=CARTESIAN_POINT('Ctrl Pts',(88.882769382702,-34.0927745244804,107.789742615962));
#33524=CARTESIAN_POINT('Ctrl Pts',(89.6265485524304,-34.4591762110938,107.737093108232));
#33525=CARTESIAN_POINT('Ctrl Pts',(90.1719615930681,-35.2283955225168,107.684443600501));
#33526=CARTESIAN_POINT('Ctrl Pts',(90.2718152031542,-36.0513827690257,107.63179409277));
#33527=CARTESIAN_POINT('Ctrl Pts',(90.3716688132402,-36.8743700155345,107.579144585039));
#33528=CARTESIAN_POINT('Ctrl Pts',(90.0259629927746,-37.7511251971291,107.526495077308));
#33529=CARTESIAN_POINT('Ctrl Pts',(89.3912931505371,-38.2848771074855,107.473845569577));
#33530=CARTESIAN_POINT('Ctrl Pts',(88.7566233082995,-38.8186290178419,107.421196061847));
#33531=CARTESIAN_POINT('Ctrl Pts',(87.83298944429,-39.0093776569599,107.368546554116));
#33532=CARTESIAN_POINT('Ctrl Pts',(87.0393722154312,-38.7692235139292,107.315897046385));
#33533=CARTESIAN_POINT('Ctrl Pts',(86.2457549865724,-38.5290693708984,107.263247538654));
#33534=CARTESIAN_POINT('Ctrl Pts',(85.5821543928644,-37.8580124457189,107.210598030923));
#33535=CARTESIAN_POINT('Ctrl Pts',(85.3491891976178,-37.0637266223766,107.157948523192));
#33536=CARTESIAN_POINT('Ctrl Pts',(85.2822780465398,-36.8355956405425,107.142826782959));
#33537=CARTESIAN_POINT('Ctrl Pts',(85.2508911229913,-36.5972991882612,107.127705042726));
#33538=CARTESIAN_POINT('Ctrl Pts',(85.2529645136107,-36.3584982898635,107.112583302492));
#33539=CARTESIAN_POINT('Ctrl Pts',(85.2550452373729,-36.354668632511,107.387416697508));
#33540=CARTESIAN_POINT('Ctrl Pts',(85.2553232707789,-36.7850893471658,107.414523087103));
#33541=CARTESIAN_POINT('Ctrl Pts',(85.360231964155,-37.2156653176389,107.441629476698));
#33542=CARTESIAN_POINT('Ctrl Pts',(85.568953011386,-37.5880327420653,107.468735866293));
#33543=CARTESIAN_POINT('Ctrl Pts',(85.9743578090732,-38.3112925300341,107.521385374024));
#33544=CARTESIAN_POINT('Ctrl Pts',(86.771409166583,-38.8149524730431,107.574034881755));
#33545=CARTESIAN_POINT('Ctrl Pts',(87.5986589133747,-38.8708034657323,107.626684389485));
#33546=CARTESIAN_POINT('Ctrl Pts',(88.4259086601662,-38.9266544584215,107.679333897216));
#33547=CARTESIAN_POINT('Ctrl Pts',(89.2833567962396,-38.534696500791,107.731983404947));
#33548=CARTESIAN_POINT('Ctrl Pts',(89.7823491636544,-37.8725606603013,107.784632912678));
#33549=CARTESIAN_POINT('Ctrl Pts',(90.2813415310692,-37.2104248198116,107.837282420409));
#33550=CARTESIAN_POINT('Ctrl Pts',(90.4218781298253,-36.2781110964627,107.889931928139));
#33551=CARTESIAN_POINT('Ctrl Pts',(90.1402211568184,-35.4982975081166,107.94258143587));
#33552=CARTESIAN_POINT('Ctrl Pts',(89.8585641838115,-34.7184839197706,107.995230943601));
#33553=CARTESIAN_POINT('Ctrl Pts',(89.1547136390417,-34.0911704664274,108.047880451332));
#33554=CARTESIAN_POINT('Ctrl Pts',(88.3477629187951,-33.9007266610526,108.100529959063));
#33555=CARTESIAN_POINT('Ctrl Pts',(87.5408121985486,-33.7102828556778,108.153179466794));
#33556=CARTESIAN_POINT('Ctrl Pts',(86.6307613028254,-33.9567086982715,108.205828974524));
#33557=CARTESIAN_POINT('Ctrl Pts',(86.0301614241252,-34.5282973451729,108.258478482255));
#33558=CARTESIAN_POINT('Ctrl Pts',(85.5398733551047,-34.9949026574645,108.30145788734));
#33559=CARTESIAN_POINT('Ctrl Pts',(85.255802105395,-35.6781950561571,108.344437292424));
#33560=CARTESIAN_POINT('Ctrl Pts',(85.2497507212102,-36.3570215567107,108.387416697508));
#33561=CARTESIAN_POINT('Origin',(87.7685555885722,-36.3549260746835,114.));
#33562=CARTESIAN_POINT('',(85.2489005391845,-36.3530683166817,109.387416697508));
#33563=CARTESIAN_POINT('',(85.2539950043281,-36.3533981322694,109.112583302492));
#33564=CARTESIAN_POINT('',(85.2510555885723,-36.3549260746835,114.));
#33565=CARTESIAN_POINT('Ctrl Pts',(85.2539950043281,-36.3533981322694,109.112583302492));
#33566=CARTESIAN_POINT('Ctrl Pts',(85.2522387491172,-36.0401068363841,109.092832468829));
#33567=CARTESIAN_POINT('Ctrl Pts',(85.3065359379297,-35.7274023602209,109.073081635165));
#33568=CARTESIAN_POINT('Ctrl Pts',(85.4196755025654,-35.4376761985452,109.053330801502));
#33569=CARTESIAN_POINT('Ctrl Pts',(85.7212699812842,-34.6653574170195,109.000681293771));
#33570=CARTESIAN_POINT('Ctrl Pts',(86.4409912230722,-34.056319742401,108.94803178604));
#33571=CARTESIAN_POINT('Ctrl Pts',(87.2525647396359,-33.8866600926086,108.89538227831));
#33572=CARTESIAN_POINT('Ctrl Pts',(88.0641382561996,-33.7170004428162,108.842732770579));
#33573=CARTESIAN_POINT('Ctrl Pts',(88.9675640475391,-33.98671881785,108.790083262848));
#33574=CARTESIAN_POINT('Ctrl Pts',(89.5532873745519,-34.5735446538035,108.737433755117));
#33575=CARTESIAN_POINT('Ctrl Pts',(90.1390107015647,-35.160370489757,108.684784247386));
#33576=CARTESIAN_POINT('Ctrl Pts',(90.4070315642508,-36.0643037866303,108.632134739655));
#33577=CARTESIAN_POINT('Ctrl Pts',(90.2358475921449,-36.8755556888539,108.579485231925));
#33578=CARTESIAN_POINT('Ctrl Pts',(90.0646636200388,-37.6868075910774,108.526835724194));
#33579=CARTESIAN_POINT('Ctrl Pts',(89.4542748131408,-38.4053780986513,108.474186216463));
#33580=CARTESIAN_POINT('Ctrl Pts',(88.6813899854773,-38.7055233320582,108.421536708732));
#33581=CARTESIAN_POINT('Ctrl Pts',(87.9085051578137,-39.0056685654652,108.368887201001));
#33582=CARTESIAN_POINT('Ctrl Pts',(86.9731243093848,-38.8873885247051,108.316237693271));
#33583=CARTESIAN_POINT('Ctrl Pts',(86.2992915567292,-38.4042848873103,108.26358818554));
#33584=CARTESIAN_POINT('Ctrl Pts',(85.655081443511,-37.9424191680858,108.213253224524));
#33585=CARTESIAN_POINT('Ctrl Pts',(85.2499288480938,-37.1471011131107,108.162918263508));
#33586=CARTESIAN_POINT('Ctrl Pts',(85.2471487745657,-36.3542597485476,108.112583302492));
#33587=CARTESIAN_POINT('Ctrl Pts',(85.2497507212102,-36.3570215567107,108.387416697508));
#33588=CARTESIAN_POINT('Ctrl Pts',(85.2483891968683,-36.5097533575973,108.397086800155));
#33589=CARTESIAN_POINT('Ctrl Pts',(85.2611016612133,-36.6622590847112,108.406756902801));
#33590=CARTESIAN_POINT('Ctrl Pts',(85.2887059289636,-36.8120198732506,108.416427005448));
#33591=CARTESIAN_POINT('Ctrl Pts',(85.4389991741796,-37.6274023032177,108.469076513178));
#33592=CARTESIAN_POINT('Ctrl Pts',(86.0307345262888,-38.3614157119429,108.521726020909));
#33593=CARTESIAN_POINT('Ctrl Pts',(86.7956562152289,-38.6813078345256,108.57437552864));
#33594=CARTESIAN_POINT('Ctrl Pts',(87.560577904169,-39.0011999571083,108.627025036371));
#33595=CARTESIAN_POINT('Ctrl Pts',(88.4986859299399,-38.9069707935486,108.679674544102));
#33596=CARTESIAN_POINT('Ctrl Pts',(89.1847040366692,-38.4413369476427,108.732324051833));
#33597=CARTESIAN_POINT('Ctrl Pts',(89.8707221433986,-37.9757031017368,108.784973559563));
#33598=CARTESIAN_POINT('Ctrl Pts',(90.3046503310864,-37.1386645734846,108.837623067294));
#33599=CARTESIAN_POINT('Ctrl Pts',(90.2897734888853,-36.3096804178693,108.890272575025));
#33600=CARTESIAN_POINT('Ctrl Pts',(90.2748966466842,-35.480696262254,108.942922082756));
#33601=CARTESIAN_POINT('Ctrl Pts',(89.8112147745942,-34.6597664792756,108.995571590487));
#33602=CARTESIAN_POINT('Ctrl Pts',(89.1089311759761,-34.2190469239351,109.048221098218));
#33603=CARTESIAN_POINT('Ctrl Pts',(88.406647577358,-33.7783273685947,109.100870605948));
#33604=CARTESIAN_POINT('Ctrl Pts',(87.4657622522118,-33.7178180408923,109.153520113679));
#33605=CARTESIAN_POINT('Ctrl Pts',(86.71281116839,-34.0649500111222,109.20616962141));
#33606=CARTESIAN_POINT('Ctrl Pts',(85.9598600845683,-34.4120819813521,109.258819129141));
#33607=CARTESIAN_POINT('Ctrl Pts',(85.3948432420709,-35.1668552495144,109.311468636872));
#33608=CARTESIAN_POINT('Ctrl Pts',(85.2739024763654,-35.9871047900117,109.364118144602));
#33609=CARTESIAN_POINT('Ctrl Pts',(85.2560628361378,-36.1080975472008,109.371884328904));
#33610=CARTESIAN_POINT('Ctrl Pts',(85.2478855763512,-36.2305149626551,109.379650513206));
#33611=CARTESIAN_POINT('Ctrl Pts',(85.2489005391845,-36.3530683166817,109.387416697508));
#33612=CARTESIAN_POINT('Origin',(87.7685555885722,-36.3549260746835,114.));
#33613=CARTESIAN_POINT('',(85.2549714308827,-36.3546406872631,110.387416697508));
#33614=CARTESIAN_POINT('',(85.2524196711837,-36.3570497194806,110.112583302492));
#33615=CARTESIAN_POINT('',(85.2510555885723,-36.3549260746835,114.));
#33616=CARTESIAN_POINT('Ctrl Pts',(85.2524196711837,-36.3570497194806,110.112583302492));
#33617=CARTESIAN_POINT('Ctrl Pts',(85.2572191354379,-35.768112702753,110.07539618188));
#33618=CARTESIAN_POINT('Ctrl Pts',(85.4637776199823,-35.1761421078341,110.038209061269));
#33619=CARTESIAN_POINT('Ctrl Pts',(85.8414731263454,-34.7285995245313,110.001021940657));
#33620=CARTESIAN_POINT('Ctrl Pts',(86.3762142451804,-34.094968947281,109.948372432926));
#33621=CARTESIAN_POINT('Ctrl Pts',(87.2539975215157,-33.7508426291429,109.895722925195));
#33622=CARTESIAN_POINT('Ctrl Pts',(88.07689325785,-33.8522249894879,109.843073417464));
#33623=CARTESIAN_POINT('Ctrl Pts',(88.8997889941843,-33.9536073498329,109.790423909734));
#33624=CARTESIAN_POINT('Ctrl Pts',(89.6677971905177,-34.500498388661,109.737774402003));
#33625=CARTESIAN_POINT('Ctrl Pts',(90.0327530047769,-35.2449733985566,109.685124894272));
#33626=CARTESIAN_POINT('Ctrl Pts',(90.3977088190361,-35.9894484084521,109.632475386541));
#33627=CARTESIAN_POINT('Ctrl Pts',(90.3596122512212,-36.9315073894151,109.57982587881));
#33628=CARTESIAN_POINT('Ctrl Pts',(89.9357338117621,-37.6440821693962,109.52717637108));
#33629=CARTESIAN_POINT('Ctrl Pts',(89.511855372303,-38.3566569493773,109.474526863349));
#33630=CARTESIAN_POINT('Ctrl Pts',(88.7021950611999,-38.8397475283767,109.421877355618));
#33631=CARTESIAN_POINT('Ctrl Pts',(87.8738000460567,-38.8743522594697,109.369227847887));
#33632=CARTESIAN_POINT('Ctrl Pts',(87.0454050309135,-38.9089569905627,109.316578340156));
#33633=CARTESIAN_POINT('Ctrl Pts',(86.1982753117304,-38.4950758737495,109.263928832425));
#33634=CARTESIAN_POINT('Ctrl Pts',(85.7164443099636,-37.8203353711265,109.211279324695));
#33635=CARTESIAN_POINT('Ctrl Pts',(85.4153664506265,-37.3987157049098,109.178380650627));
#33636=CARTESIAN_POINT('Ctrl Pts',(85.2569203728846,-36.8752428506858,109.14548197656));
#33637=CARTESIAN_POINT('Ctrl Pts',(85.2539950043281,-36.3533981322694,109.112583302492));
#33638=CARTESIAN_POINT('Ctrl Pts',(85.2489005391845,-36.3530683166817,109.387416697508));
#33639=CARTESIAN_POINT('Ctrl Pts',(85.254766341919,-37.0613443003947,109.432300020937));
#33640=CARTESIAN_POINT('Ctrl Pts',(85.567658150359,-37.7741607177567,109.477183344366));
#33641=CARTESIAN_POINT('Ctrl Pts',(86.0968199097674,-38.2427519208318,109.522066667795));
#33642=CARTESIAN_POINT('Ctrl Pts',(86.7175427977887,-38.7924236983225,109.574716175526));
#33643=CARTESIAN_POINT('Ctrl Pts',(87.635853262745,-39.0060414404716,109.627365683257));
#33644=CARTESIAN_POINT('Ctrl Pts',(88.4354492298588,-38.7867647823512,109.680015190987));
#33645=CARTESIAN_POINT('Ctrl Pts',(89.2350451969726,-38.5674881242308,109.732664698718));
#33646=CARTESIAN_POINT('Ctrl Pts',(89.915926666244,-37.9153170658409,109.785314206449));
#33647=CARTESIAN_POINT('Ctrl Pts',(90.169426372785,-37.1259034439069,109.83796371418));
#33648=CARTESIAN_POINT('Ctrl Pts',(90.4229260793259,-36.3364898219729,109.890613221911));
#33649=CARTESIAN_POINT('Ctrl Pts',(90.2490440231364,-35.4098336364947,109.943262729642));
#33650=CARTESIAN_POINT('Ctrl Pts',(89.7266069925469,-34.7660203753152,109.995912237372));
#33651=CARTESIAN_POINT('Ctrl Pts',(89.2041699619573,-34.1222071141356,110.048561745103));
#33652=CARTESIAN_POINT('Ctrl Pts',(88.3331779569678,-33.7612367772546,110.101211252834));
#33653=CARTESIAN_POINT('Ctrl Pts',(87.5084819568861,-33.8467497788348,110.153860760565));
#33654=CARTESIAN_POINT('Ctrl Pts',(86.6837859568044,-33.9322627804151,110.206510268296));
#33655=CARTESIAN_POINT('Ctrl Pts',(85.9053859616305,-34.4642591204566,110.259159776027));
#33656=CARTESIAN_POINT('Ctrl Pts',(85.5261577727488,-35.201566347613,110.311809283757));
#33657=CARTESIAN_POINT('Ctrl Pts',(85.3446273474991,-35.5545034403965,110.337011755008));
#33658=CARTESIAN_POINT('Ctrl Pts',(85.2545624585998,-35.9544851142665,110.362214226258));
#33659=CARTESIAN_POINT('Ctrl Pts',(85.2549714308827,-36.3546406872631,110.387416697508));
#33660=CARTESIAN_POINT('Origin',(87.7685555885722,-36.3549260746835,114.));
#33661=CARTESIAN_POINT('',(85.2499087442488,-36.3570522860866,111.387416697508));
#33662=CARTESIAN_POINT('',(85.2470899772098,-36.354365150253,111.112583302492));
#33663=CARTESIAN_POINT('',(85.2510555885723,-36.3549260746835,114.));
#33664=CARTESIAN_POINT('Ctrl Pts',(85.2470899772098,-36.354365150253,111.112583302492));
#33665=CARTESIAN_POINT('Ctrl Pts',(85.2469952533804,-36.323275203713,111.110609402663));
#33666=CARTESIAN_POINT('Ctrl Pts',(85.2475210549401,-36.2921885346853,111.108635502833));
#33667=CARTESIAN_POINT('Ctrl Pts',(85.2486773612175,-36.2611253357633,111.106661603004));
#33668=CARTESIAN_POINT('Ctrl Pts',(85.279519329685,-35.4325817047621,111.054012095273));
#33669=CARTESIAN_POINT('Ctrl Pts',(85.7589277104219,-34.6207356508032,111.001362587543));
#33670=CARTESIAN_POINT('Ctrl Pts',(86.4695700042782,-34.1936252369474,110.948713079812));
#33671=CARTESIAN_POINT('Ctrl Pts',(87.1802122981346,-33.7665148230915,110.896063572081));
#33672=CARTESIAN_POINT('Ctrl Pts',(88.1220885051104,-33.7241400493387,110.84341406435));
#33673=CARTESIAN_POINT('Ctrl Pts',(88.8682133697417,-34.0857108748008,110.790764556619));
#33674=CARTESIAN_POINT('Ctrl Pts',(89.614338234373,-34.4472817002629,110.738115048888));
#33675=CARTESIAN_POINT('Ctrl Pts',(90.1647117566598,-35.2127981249399,110.685465541158));
#33676=CARTESIAN_POINT('Ctrl Pts',(90.2698304696313,-36.0352249191472,110.632816033427));
#33677=CARTESIAN_POINT('Ctrl Pts',(90.3749491826028,-36.8576517133544,110.580166525696));
#33678=CARTESIAN_POINT('Ctrl Pts',(90.0348130862591,-37.7369888770919,110.527517017965));
#33679=CARTESIAN_POINT('Ctrl Pts',(89.4036177076337,-38.2746022783177,110.474867510234));
#33680=CARTESIAN_POINT('Ctrl Pts',(88.7724223290083,-38.8122156795435,110.422218002503));
#33681=CARTESIAN_POINT('Ctrl Pts',(87.8501676681012,-39.0081053182576,110.369568494773));
#33682=CARTESIAN_POINT('Ctrl Pts',(87.0549438505888,-38.7734676072038,110.316918987042));
#33683=CARTESIAN_POINT('Ctrl Pts',(86.2597200330764,-38.5388298961499,110.264269479311));
#33684=CARTESIAN_POINT('Ctrl Pts',(85.5915270589586,-37.8736648353281,110.21161997158));
#33685=CARTESIAN_POINT('Ctrl Pts',(85.3532800525671,-37.079514886736,110.158970463849));
#33686=CARTESIAN_POINT('Ctrl Pts',(85.2833104060962,-36.8462847110897,110.14350807673));
#33687=CARTESIAN_POINT('Ctrl Pts',(85.2504240562223,-36.6019294518078,110.128045689611));
#33688=CARTESIAN_POINT('Ctrl Pts',(85.2524196711837,-36.3570497194806,110.112583302492));
#33689=CARTESIAN_POINT('Ctrl Pts',(85.2549714308827,-36.3546406872631,110.387416697508));
#33690=CARTESIAN_POINT('Ctrl Pts',(85.2554168267748,-36.7904346417883,110.414863733989));
#33691=CARTESIAN_POINT('Ctrl Pts',(85.3631691571782,-37.2264348501634,110.442310770469));
#33692=CARTESIAN_POINT('Ctrl Pts',(85.5769474890366,-37.60209910281,110.46975780695));
#33693=CARTESIAN_POINT('Ctrl Pts',(85.9870217767954,-38.3227065165792,110.522407314681));
#33694=CARTESIAN_POINT('Ctrl Pts',(86.7872267349022,-38.8213032298464,110.575056822411));
#33695=CARTESIAN_POINT('Ctrl Pts',(87.6148016142974,-38.8718580045868,110.627706330142));
#33696=CARTESIAN_POINT('Ctrl Pts',(88.4423764936926,-38.9224127793273,110.680355837873));
#33697=CARTESIAN_POINT('Ctrl Pts',(89.2973212943763,-38.5249256155411,110.733005345604));
#33698=CARTESIAN_POINT('Ctrl Pts',(89.79205979188,-37.8595912744819,110.785654853335));
#33699=CARTESIAN_POINT('Ctrl Pts',(90.2867982893837,-37.1942569334227,110.838304361066));
#33700=CARTESIAN_POINT('Ctrl Pts',(90.4213304837074,-36.2610754150906,110.890953868796));
#33701=CARTESIAN_POINT('Ctrl Pts',(90.1346682503914,-35.4830903700737,110.943603376527));
#33702=CARTESIAN_POINT('Ctrl Pts',(89.8480060170754,-34.7051053250569,110.996252884258));
#33703=CARTESIAN_POINT('Ctrl Pts',(89.1401493561197,-34.0823167533554,111.048902391989));
#33704=CARTESIAN_POINT('Ctrl Pts',(88.3319943205098,-33.8970563833361,111.10155189972));
#33705=CARTESIAN_POINT('Ctrl Pts',(87.5238392849,-33.7117960133168,111.15420140745));
#33706=CARTESIAN_POINT('Ctrl Pts',(86.615385874636,-33.9640638449797,111.206850915181));
#33707=CARTESIAN_POINT('Ctrl Pts',(86.0184676285876,-34.5394980930228,111.259500422912));
#33708=CARTESIAN_POINT('Ctrl Pts',(85.53504710189,-35.0055195777242,111.302139181111));
#33709=CARTESIAN_POINT('Ctrl Pts',(85.2559544134533,-35.6834975374635,111.344777939309));
#33710=CARTESIAN_POINT('Ctrl Pts',(85.2499087442488,-36.3570522860866,111.387416697508));
#33711=CARTESIAN_POINT('Origin',(87.7685555885722,-36.3549260746835,114.));
#33712=CARTESIAN_POINT('',(85.2487565565375,-36.3531221774957,112.387416697508));
#33713=CARTESIAN_POINT('',(85.2538920866812,-36.3533353395906,112.112583302492));
#33714=CARTESIAN_POINT('',(85.2510555885723,-36.3549260746835,114.));
#33715=CARTESIAN_POINT('Ctrl Pts',(85.2538920866812,-36.3533353395906,112.112583302492));
#33716=CARTESIAN_POINT('Ctrl Pts',(85.2520903341024,-36.0454791376291,112.093173115714));
#33717=CARTESIAN_POINT('Ctrl Pts',(85.3044765460178,-35.7382147173017,112.073762928937));
#33718=CARTESIAN_POINT('Ctrl Pts',(85.4138342400317,-35.4527774006629,112.054352742159));
#33719=CARTESIAN_POINT('Ctrl Pts',(85.7104634699489,-34.6785378541209,112.001703234428));
#33720=CARTESIAN_POINT('Ctrl Pts',(86.4262593467811,-34.0648908273442,111.949053726697));
#33721=CARTESIAN_POINT('Ctrl Pts',(87.2367266947401,-33.8900238683076,111.896404218967));
#33722=CARTESIAN_POINT('Ctrl Pts',(88.047194042699,-33.7151569092711,111.843754711236));
#33723=CARTESIAN_POINT('Ctrl Pts',(88.9523328617846,-33.9790700179748,111.791105203505));
#33724=CARTESIAN_POINT('Ctrl Pts',(89.5418122326413,-34.5621221998627,111.738455695774));
#33725=CARTESIAN_POINT('Ctrl Pts',(90.1312916034979,-35.1451743817506,111.685806188043));
#33726=CARTESIAN_POINT('Ctrl Pts',(90.4051115261256,-36.0473656368227,111.633156680312));
#33727=CARTESIAN_POINT('Ctrl Pts',(90.2391399025284,-36.8597012790504,111.580507172582));
#33728=CARTESIAN_POINT('Ctrl Pts',(90.0731682789312,-37.672036921278,111.527857664851));
#33729=CARTESIAN_POINT('Ctrl Pts',(89.4674051091091,-38.3945169506613,111.47520815712));
#33730=CARTESIAN_POINT('Ctrl Pts',(88.696463914376,-38.6996160324873,111.422558649389));
#33731=CARTESIAN_POINT('Ctrl Pts',(87.9255227196427,-39.0047151143134,111.369909141658));
#33732=CARTESIAN_POINT('Ctrl Pts',(86.9894034999983,-38.8924332485823,111.317259633928));
#33733=CARTESIAN_POINT('Ctrl Pts',(86.3124816682752,-38.4136717116951,111.264610126197));
#33734=CARTESIAN_POINT('Ctrl Pts',(85.6609385332515,-37.9528595794017,111.213934518295));
#33735=CARTESIAN_POINT('Ctrl Pts',(85.2495218066094,-37.152532269562,111.163258910394));
#33736=CARTESIAN_POINT('Ctrl Pts',(85.2470899772098,-36.354365150253,111.112583302492));
#33737=CARTESIAN_POINT('Ctrl Pts',(85.2499087442488,-36.3570522860866,111.387416697508));
#33738=CARTESIAN_POINT('Ctrl Pts',(85.2484893389303,-36.5151898156383,111.39742744704));
#33739=CARTESIAN_POINT('Ctrl Pts',(85.2621208012014,-36.6730835294362,111.407438196572));
#33740=CARTESIAN_POINT('Ctrl Pts',(85.2916924634678,-36.8279331399315,111.417448946105));
#33741=CARTESIAN_POINT('Ctrl Pts',(85.4472186262289,-37.6423332743741,111.470098453835));
#33742=CARTESIAN_POINT('Ctrl Pts',(86.0436540335839,-38.372532878836,111.522747961566));
#33743=CARTESIAN_POINT('Ctrl Pts',(86.8106137634916,-38.6875070666412,111.575397469297));
#33744=CARTESIAN_POINT('Ctrl Pts',(87.5775734933993,-39.0024812544465,111.628046977028));
#33745=CARTESIAN_POINT('Ctrl Pts',(88.5150575458597,-38.9022300255951,111.680696484759));
#33746=CARTESIAN_POINT('Ctrl Pts',(89.1980717818333,-38.432200750186,111.73334599249));
#33747=CARTESIAN_POINT('Ctrl Pts',(89.8810860178069,-37.9621714747769,111.78599550022));
#33748=CARTESIAN_POINT('Ctrl Pts',(90.3096304372937,-37.1223641528102,111.838645007951));
#33749=CARTESIAN_POINT('Ctrl Pts',(90.2894309445145,-36.2934926629065,111.891294515682));
#33750=CARTESIAN_POINT('Ctrl Pts',(90.2692314517352,-35.4646211730027,111.943944023413));
#33751=CARTESIAN_POINT('Ctrl Pts',(89.80028804669,-34.6466855151619,111.996593531144));
#33752=CARTESIAN_POINT('Ctrl Pts',(89.0951890909213,-34.2104843816722,112.049243038874));
#33753=CARTESIAN_POINT('Ctrl Pts',(88.3900901351525,-33.7742832481825,112.101892546605));
#33754=CARTESIAN_POINT('Ctrl Pts',(87.4488356286603,-33.7198166390438,112.154542054336));
#33755=CARTESIAN_POINT('Ctrl Pts',(86.6981289884821,-34.0717761632455,112.207191562067));
#33756=CARTESIAN_POINT('Ctrl Pts',(85.9474223483039,-34.4237356874472,112.259841069798));
#33757=CARTESIAN_POINT('Ctrl Pts',(85.3872635744398,-35.1821213449894,112.312490577529));
#33758=CARTESIAN_POINT('Ctrl Pts',(85.2715921287914,-36.0031305306539,112.365140085259));
#33759=CARTESIAN_POINT('Ctrl Pts',(85.2552781557902,-36.1189233403108,112.372565622676));
#33760=CARTESIAN_POINT('Ctrl Pts',(85.2478056946932,-36.2359618247805,112.379991160092));
#33761=CARTESIAN_POINT('Ctrl Pts',(85.2487565565375,-36.3531221774957,112.387416697508));
#33762=CARTESIAN_POINT('Origin',(87.7685555885722,-36.3549260746835,114.));
#33763=CARTESIAN_POINT('',(85.254950234978,-36.3545547484977,113.387416697508));
#33764=CARTESIAN_POINT('',(85.2525639081684,-36.3570196911117,113.112583302492));
#33765=CARTESIAN_POINT('',(85.2510555885723,-36.3549260746835,114.));
#33766=CARTESIAN_POINT('Ctrl Pts',(85.2525639081684,-36.3570196911117,113.112583302492));
#33767=CARTESIAN_POINT('Ctrl Pts',(85.2572319946921,-35.773392729585,113.075736828766));
#33768=CARTESIAN_POINT('Ctrl Pts',(85.4596895883703,-35.1868436112621,113.03889035504));
#33769=CARTESIAN_POINT('Ctrl Pts',(85.8310702123153,-34.7410068461903,113.002043881314));
#33770=CARTESIAN_POINT('Ctrl Pts',(86.3617317669821,-34.10395575729,112.949394373583));
#33771=CARTESIAN_POINT('Ctrl Pts',(87.2372873147814,-33.7542002805938,112.896744865852));
#33772=CARTESIAN_POINT('Ctrl Pts',(88.0608170625274,-33.850296742796,112.844095358121));
#33773=CARTESIAN_POINT('Ctrl Pts',(88.8843468102735,-33.9463932049982,112.791445850391));
#33774=CARTESIAN_POINT('Ctrl Pts',(89.6558507579663,-34.4883416060987,112.73879634266));
#33775=CARTESIAN_POINT('Ctrl Pts',(90.0255793230353,-35.2304578797664,112.686146834929));
#33776=CARTESIAN_POINT('Ctrl Pts',(90.3953078881044,-35.9725741534341,112.633497327198));
#33777=CARTESIAN_POINT('Ctrl Pts',(90.3632610705496,-36.914858299669,112.580847819467));
#33778=CARTESIAN_POINT('Ctrl Pts',(89.9439668077795,-37.6301401299139,112.528198311736));
#33779=CARTESIAN_POINT('Ctrl Pts',(89.5246725450094,-38.3454219601589,112.475548804006));
#33780=CARTESIAN_POINT('Ctrl Pts',(88.718130837024,-38.8337014744139,112.422899296275));
#33781=CARTESIAN_POINT('Ctrl Pts',(87.8899751022099,-38.8736245800664,112.370249788544));
#33782=CARTESIAN_POINT('Ctrl Pts',(87.0618193673958,-38.9135476857189,112.317600280813));
#33783=CARTESIAN_POINT('Ctrl Pts',(86.212049605753,-38.5051143827689,112.264950773082));
#33784=CARTESIAN_POINT('Ctrl Pts',(85.7258960164326,-37.8334816981404,112.212301265351));
#33785=CARTESIAN_POINT('Ctrl Pts',(85.4189716806808,-37.4094584673606,112.179061944398));
#33786=CARTESIAN_POINT('Ctrl Pts',(85.2569775300586,-36.880529189996,112.145822623445));
#33787=CARTESIAN_POINT('Ctrl Pts',(85.2538920866812,-36.3533353395906,112.112583302492));
#33788=CARTESIAN_POINT('Ctrl Pts',(85.2487565565375,-36.3531221774957,112.387416697508));
#33789=CARTESIAN_POINT('Ctrl Pts',(85.2545476185725,-37.0666673414699,112.432640667823));
#33790=CARTESIAN_POINT('Ctrl Pts',(85.572777540667,-37.7847328563774,112.477864638137));
#33791=CARTESIAN_POINT('Ctrl Pts',(86.1089760963731,-38.2534472184562,112.523088608452));
#33792=CARTESIAN_POINT('Ctrl Pts',(86.7332156270358,-38.7991220068071,112.575738116183));
#33793=CARTESIAN_POINT('Ctrl Pts',(87.652878805794,-39.0068388697222,112.628387623914));
#33794=CARTESIAN_POINT('Ctrl Pts',(88.4510503157032,-38.7824325261102,112.681037131644));
#33795=CARTESIAN_POINT('Ctrl Pts',(89.2492218256123,-38.5580261824983,112.733686639375));
#33796=CARTESIAN_POINT('Ctrl Pts',(89.9259016666724,-37.9014966323593,112.786336147106));
#33797=CARTESIAN_POINT('Ctrl Pts',(90.1743273230824,-37.110471563527,112.838985654837));
#33798=CARTESIAN_POINT('Ctrl Pts',(90.4227529794924,-36.3194464946947,112.891635162568));
#33799=CARTESIAN_POINT('Ctrl Pts',(90.2429244512524,-35.3939259071691,112.944284670298));
#33800=CARTESIAN_POINT('Ctrl Pts',(89.7163642670212,-34.7534804850867,112.996934178029));
#33801=CARTESIAN_POINT('Ctrl Pts',(89.1898040827899,-34.1130350630043,113.04958368576));
#33802=CARTESIAN_POINT('Ctrl Pts',(88.3165122425674,-33.7576648063653,113.102233193491));
#33803=CARTESIAN_POINT('Ctrl Pts',(87.4923823221333,-33.8484714169679,113.154882701222));
#33804=CARTESIAN_POINT('Ctrl Pts',(86.6682524016991,-33.9392780275705,113.207532208953));
#33805=CARTESIAN_POINT('Ctrl Pts',(85.8932844010533,-34.4762615054149,113.260181716683));
#33806=CARTESIAN_POINT('Ctrl Pts',(85.5187982784954,-35.2159885566273,113.312831224414));
#33807=CARTESIAN_POINT('Ctrl Pts',(85.3419607617305,-35.5652978819683,113.337693048779));
#33808=CARTESIAN_POINT('Ctrl Pts',(85.2544250479382,-35.9598161609063,113.362554873143));
#33809=CARTESIAN_POINT('Ctrl Pts',(85.254950234978,-36.3545547484977,113.387416697508));
#33810=CARTESIAN_POINT('Origin',(87.7685555885722,-36.3549260746835,114.));
#33811=CARTESIAN_POINT('',(85.2500677995525,-36.3570794361965,114.387416697508));
#33812=CARTESIAN_POINT('',(85.2470414567978,-36.3544600798358,114.112583302492));
#33813=CARTESIAN_POINT('',(85.2510555885723,-36.3549260746835,114.));
#33814=CARTESIAN_POINT('Ctrl Pts',(85.2470414567978,-36.3544600798358,114.112583302492));
#33815=CARTESIAN_POINT('Ctrl Pts',(85.2469753692349,-36.3287368261812,114.110950049548));
#33816=CARTESIAN_POINT('Ctrl Pts',(85.2473353127159,-36.3030154666756,114.109316796605));
#33817=CARTESIAN_POINT('Ctrl Pts',(85.2481270136682,-36.2773074034965,114.107683543661));
#33818=CARTESIAN_POINT('Ctrl Pts',(85.2736482690049,-35.4485828165579,114.05503403593));
#33819=CARTESIAN_POINT('Ctrl Pts',(85.7478339046031,-34.6336752182663,114.002384528199));
#33820=CARTESIAN_POINT('Ctrl Pts',(86.4557190734163,-34.2020105761599,113.949735020469));
#33821=CARTESIAN_POINT('Ctrl Pts',(87.1636042422294,-33.7703459340536,113.897085512738));
#33822=CARTESIAN_POINT('Ctrl Pts',(88.1051889442577,-33.7219242481326,113.844436005007));
#33823=CARTESIAN_POINT('Ctrl Pts',(88.8536200733386,-34.0786967533697,113.791786497276));
#33824=CARTESIAN_POINT('Ctrl Pts',(89.6020512024195,-34.4354692586068,113.739136989545));
#33825=CARTESIAN_POINT('Ctrl Pts',(90.157328758553,-35.197435955002,113.686487481814));
#33826=CARTESIAN_POINT('Ctrl Pts',(90.2677261056678,-36.0191708278293,113.633837974084));
#33827=CARTESIAN_POINT('Ctrl Pts',(90.3781234527826,-36.8409057006566,113.581188466353));
#33828=CARTESIAN_POINT('Ctrl Pts',(90.0436405908786,-37.7224087499159,113.528538958622));
#33829=CARTESIAN_POINT('Ctrl Pts',(89.4159102389819,-38.2640639730773,113.475889450891));
#33830=CARTESIAN_POINT('Ctrl Pts',(88.7881798870852,-38.8057191962387,113.42323994316));
#33831=CARTESIAN_POINT('Ctrl Pts',(87.8672020451956,-39.0075265933022,113.37059043543));
#33832=CARTESIAN_POINT('Ctrl Pts',(87.0704880127964,-38.7779998496562,113.317940927699));
#33833=CARTESIAN_POINT('Ctrl Pts',(86.2737739803972,-38.5484731060102,113.265291419968));
#33834=CARTESIAN_POINT('Ctrl Pts',(85.6013237574885,-37.8876122216548,113.212641912237));
#33835=CARTESIAN_POINT('Ctrl Pts',(85.3579824268013,-37.0950084289249,113.159992404506));
#33836=CARTESIAN_POINT('Ctrl Pts',(85.2849422125742,-36.8571041211991,113.144189370502));
#33837=CARTESIAN_POINT('Ctrl Pts',(85.2505618188879,-36.6073306649015,113.128386336497));
#33838=CARTESIAN_POINT('Ctrl Pts',(85.2525639081684,-36.3570196911117,113.112583302492));
#33839=CARTESIAN_POINT('Ctrl Pts',(85.254950234978,-36.3545547484977,113.387416697508));
#33840=CARTESIAN_POINT('Ctrl Pts',(85.2555372285531,-36.7957480705789,113.415204380874));
#33841=CARTESIAN_POINT('Ctrl Pts',(85.3661316014678,-37.237216606488,113.44299206424));
#33842=CARTESIAN_POINT('Ctrl Pts',(85.5850007646286,-37.6161457046895,113.470779747607));
#33843=CARTESIAN_POINT('Ctrl Pts',(85.9996936177896,-38.3341051769587,113.523429255337));
#33844=CARTESIAN_POINT('Ctrl Pts',(86.8030835685816,-38.8275534969166,113.576078763068));
#33845=CARTESIAN_POINT('Ctrl Pts',(87.6309659998135,-38.8727933724864,113.628728270799));
#33846=CARTESIAN_POINT('Ctrl Pts',(88.4588484310453,-38.9180332480561,113.68137777853));
#33847=CARTESIAN_POINT('Ctrl Pts',(89.311223342717,-38.5150646792378,113.734027286261));
#33848=CARTESIAN_POINT('Ctrl Pts',(89.8016795305277,-37.8465673388377,113.786676793992));
#33849=CARTESIAN_POINT('Ctrl Pts',(90.2921357183384,-37.1780699984375,113.839326301722));
#33850=CARTESIAN_POINT('Ctrl Pts',(90.4206731822881,-36.2440438864555,113.891975809453));
#33851=CARTESIAN_POINT('Ctrl Pts',(90.1290214177404,-35.4679155371987,113.944625317184));
#33852=CARTESIAN_POINT('Ctrl Pts',(89.8373696531927,-34.6917871879419,113.997274824915));
#33853=CARTESIAN_POINT('Ctrl Pts',(89.1255286601476,-34.0735566014102,114.049924332646));
#33854=CARTESIAN_POINT('Ctrl Pts',(88.3162007279694,-33.8934892126912,114.102573840377));
#33855=CARTESIAN_POINT('Ctrl Pts',(87.5068727957913,-33.7134218239722,114.155223348107));
#33856=CARTESIAN_POINT('Ctrl Pts',(86.60005792448,-33.9715176330658,114.207872855838));
#33857=CARTESIAN_POINT('Ctrl Pts',(86.0068468461809,-34.550772829734,114.260522363569));
#33858=CARTESIAN_POINT('Ctrl Pts',(85.5302667354934,-35.0161409185027,114.302820474882));
#33859=CARTESIAN_POINT('Ctrl Pts',(85.2560978662429,-35.6887969029749,114.345118586195));
#33860=CARTESIAN_POINT('Ctrl Pts',(85.2500677995525,-36.3570794361965,114.387416697508));
#33861=CARTESIAN_POINT('Origin',(87.7685555885722,-36.3549260746835,114.));
#33862=CARTESIAN_POINT('',(85.2486157516665,-36.3531793386365,115.387416697508));
#33863=CARTESIAN_POINT('',(85.2537848649131,-36.3532747669305,115.112583302492));
#33864=CARTESIAN_POINT('',(85.2510555885723,-36.3549260746835,114.));
#33865=CARTESIAN_POINT('Ctrl Pts',(85.2537848649131,-36.3532747669305,115.112583302492));
#33866=CARTESIAN_POINT('Ctrl Pts',(85.2519423002258,-36.0508538406101,115.0935137626));
#33867=CARTESIAN_POINT('Ctrl Pts',(85.3024544519066,-35.7490276611798,115.074444222708));
#33868=CARTESIAN_POINT('Ctrl Pts',(85.4080900870048,-35.4679156603028,115.055374682816));
#33869=CARTESIAN_POINT('Ctrl Pts',(85.6997418110755,-34.6917874187621,115.002725175085));
#33870=CARTESIAN_POINT('Ctrl Pts',(86.4115827053271,-34.0735569180327,114.950075667354));
#33871=CARTESIAN_POINT('Ctrl Pts',(87.2209105251817,-33.8934895543048,114.897426159623));
#33872=CARTESIAN_POINT('Ctrl Pts',(88.0302383450363,-33.713422190577,114.844776651893));
#33873=CARTESIAN_POINT('Ctrl Pts',(88.9370530904939,-33.9715179638508,114.792127144162));
#33874=CARTESIAN_POINT('Ctrl Pts',(89.5302640864631,-34.5507730801265,114.739477636431));
#33875=CARTESIAN_POINT('Ctrl Pts',(90.1234750824323,-35.1300281964022,114.6868281287));
#33876=CARTESIAN_POINT('Ctrl Pts',(90.4030823289133,-36.0304426556799,114.634178620969));
#33877=CARTESIAN_POINT('Ctrl Pts',(90.2423301326488,-36.84382725528,114.581529113239));
#33878=CARTESIAN_POINT('Ctrl Pts',(90.0815779363843,-37.6572118548801,114.528879605508));
#33879=CARTESIAN_POINT('Ctrl Pts',(89.4804662973744,-38.3835665948026,114.476230097777));
#33880=CARTESIAN_POINT('Ctrl Pts',(88.7115000361721,-38.693609599244,114.423580590046));
#33881=CARTESIAN_POINT('Ctrl Pts',(87.9425337749698,-39.0036526036854,114.370931082315));
#33882=CARTESIAN_POINT('Ctrl Pts',(87.0057128915752,-38.8973838726457,114.318281574584));
#33883=CARTESIAN_POINT('Ctrl Pts',(86.3257308874156,-38.4229787193331,114.265632066854));
#33884=CARTESIAN_POINT('Ctrl Pts',(85.6668427672787,-37.9632902014939,114.214615812066));
#33885=CARTESIAN_POINT('Ctrl Pts',(85.2491057665298,-37.1579510929692,114.163599557279));
#33886=CARTESIAN_POINT('Ctrl Pts',(85.2470414567978,-36.3544600798358,114.112583302492));
#33887=CARTESIAN_POINT('Ctrl Pts',(85.2500677995525,-36.3570794361965,114.387416697508));
#33888=CARTESIAN_POINT('Ctrl Pts',(85.2485920927467,-36.5206247389477,114.397768093926));
#33889=CARTESIAN_POINT('Ctrl Pts',(85.2631752786074,-36.6839081147284,114.408119490344));
#33890=CARTESIAN_POINT('Ctrl Pts',(85.2947807011693,-36.8438273231319,114.418470886761));
#33891=CARTESIAN_POINT('Ctrl Pts',(85.4555329197437,-37.6572120356188,114.471120394492));
#33892=CARTESIAN_POINT('Ctrl Pts',(86.0566446421795,-38.3835668763496,114.523769902223));
#33893=CARTESIAN_POINT('Ctrl Pts',(86.8256110101037,-38.693609923821,114.576419409954));
#33894=CARTESIAN_POINT('Ctrl Pts',(87.5945773780279,-39.0036529712925,114.629068917685));
#33895=CARTESIAN_POINT('Ctrl Pts',(88.5313983914405,-38.8973842255045,114.681718425416));
#33896=CARTESIAN_POINT('Ctrl Pts',(89.2113804899725,-38.4229790063511,114.734367933146));
#33897=CARTESIAN_POINT('Ctrl Pts',(89.8913625885046,-37.9485737871978,114.787017440877));
#33898=CARTESIAN_POINT('Ctrl Pts',(90.314505772156,-37.1060320946792,114.839666948608));
#33899=CARTESIAN_POINT('Ctrl Pts',(90.2889845132775,-36.2773073927249,114.892316456339));
#33900=CARTESIAN_POINT('Ctrl Pts',(90.263463254399,-35.4485826907707,114.94496596407));
#33901=CARTESIAN_POINT('Ctrl Pts',(89.7892775529907,-34.6336749793808,114.997615471801));
#33902=CARTESIAN_POINT('Ctrl Pts',(89.0813922859328,-34.2020102773651,115.050264979531));
#33903=CARTESIAN_POINT('Ctrl Pts',(88.373507018875,-33.7703455753493,115.102914487262));
#33904=CARTESIAN_POINT('Ctrl Pts',(87.4319221861676,-33.7219238827077,115.155563994993));
#33905=CARTESIAN_POINT('Ctrl Pts',(86.6834909532146,-34.0786964374597,115.208213502724));
#33906=CARTESIAN_POINT('Ctrl Pts',(85.9350597202615,-34.4354689922117,115.260863010455));
#33907=CARTESIAN_POINT('Ctrl Pts',(85.3797820870628,-35.1974357943573,115.313512518185));
#33908=CARTESIAN_POINT('Ctrl Pts',(85.269384724626,-36.0191707812301,115.366162025916));
#33909=CARTESIAN_POINT('Ctrl Pts',(85.2545288738985,-36.1297492591316,115.373246916447));
#33910=CARTESIAN_POINT('Ctrl Pts',(85.2477290481687,-36.2414100371975,115.380331806977));
#33911=CARTESIAN_POINT('Ctrl Pts',(85.2486157516665,-36.3531793386365,115.387416697508));
#33912=CARTESIAN_POINT('Origin',(87.7685555885722,-36.3549260746835,114.));
#33913=CARTESIAN_POINT('',(85.2549234958158,-36.3544693504482,116.387416697508));
#33914=CARTESIAN_POINT('',(85.2527054364363,-36.3569864150889,116.112583302492));
#33915=CARTESIAN_POINT('',(85.2510555885723,-36.3549260746835,114.));
#33916=CARTESIAN_POINT('Ctrl Pts',(85.2527054364363,-36.3569864150889,116.112583302492));
#33917=CARTESIAN_POINT('Ctrl Pts',(85.2572379948492,-35.7786727106942,116.076077475652));
#33918=CARTESIAN_POINT('Ctrl Pts',(85.4556438192389,-35.1975491790577,116.039571648811));
#33919=CARTESIAN_POINT('Ctrl Pts',(85.8207471804533,-34.7534807073448,116.003065821971));
#33920=CARTESIAN_POINT('Ctrl Pts',(86.3473072916053,-34.1130353741477,115.95041631424));
#33921=CARTESIAN_POINT('Ctrl Pts',(87.2205990106268,-33.7576651668295,115.897766806509));
#33922=CARTESIAN_POINT('Ctrl Pts',(88.0447288166829,-33.8484717648297,115.845117298778));
#33923=CARTESIAN_POINT('Ctrl Pts',(88.8688586227391,-33.9392783628299,115.792467791047));
#33924=CARTESIAN_POINT('Ctrl Pts',(89.6438265158298,-34.4762617661486,115.739818283317));
#33925=CARTESIAN_POINT('Ctrl Pts',(90.0183125864139,-35.2159887146971,115.687168775586));
#33926=CARTESIAN_POINT('Ctrl Pts',(90.3927986569979,-35.9557156632457,115.634519267855));
#33927=CARTESIAN_POINT('Ctrl Pts',(90.3668029050753,-36.8981861570242,115.581869760124));
#33928=CARTESIAN_POINT('Ctrl Pts',(89.9521101094678,-37.6161455296502,115.529220252393));
#33929=CARTESIAN_POINT('Ctrl Pts',(89.5374173138602,-38.3341049022763,115.476570744662));
#33930=CARTESIAN_POINT('Ctrl Pts',(88.7340274745676,-38.82755315375,115.423921236932));
#33931=CARTESIAN_POINT('Ctrl Pts',(87.9061451582346,-38.8727930230408,115.371271729201));
#33932=CARTESIAN_POINT('Ctrl Pts',(87.0782628419015,-38.9180328923316,115.31862222147));
#33933=CARTESIAN_POINT('Ctrl Pts',(86.225888048528,-38.5150643794395,115.265972713739));
#33934=CARTESIAN_POINT('Ctrl Pts',(85.7354319287861,-37.8465671318175,115.213323206008));
#33935=CARTESIAN_POINT('Ctrl Pts',(85.4226179740676,-37.4201981676435,115.17974323817));
#33936=CARTESIAN_POINT('Ctrl Pts',(85.2570294771738,-36.8858143581896,115.146163270331));
#33937=CARTESIAN_POINT('Ctrl Pts',(85.2537848649131,-36.3532747669305,115.112583302492));
#33938=CARTESIAN_POINT('Ctrl Pts',(85.2486157516665,-36.3531793386365,115.387416697508));
#33939=CARTESIAN_POINT('Ctrl Pts',(85.2543183528958,-37.0719943171931,115.432981314708));
#33940=CARTESIAN_POINT('Ctrl Pts',(85.5779421228608,-37.795297911688,115.478545931909));
#33941=CARTESIAN_POINT('Ctrl Pts',(86.1212007095315,-38.2640642380391,115.524110549109));
#33942=CARTESIAN_POINT('Ctrl Pts',(86.7489311485485,-38.8057195363751,115.57676005684));
#33943=CARTESIAN_POINT('Ctrl Pts',(87.6699091182572,-39.0075269614469,115.62940956457));
#33944=CARTESIAN_POINT('Ctrl Pts',(88.4666232612295,-38.7780001859461,115.682059072301));
#33945=CARTESIAN_POINT('Ctrl Pts',(89.2633374042018,-38.5484734104452,115.734708580032));
#33946=CARTESIAN_POINT('Ctrl Pts',(89.9357877204377,-37.8876124343716,115.787358087763));
#33947=CARTESIAN_POINT('Ctrl Pts',(90.1791290848976,-37.0950085316391,115.840007595494));
#33948=CARTESIAN_POINT('Ctrl Pts',(90.4224704493576,-36.3024046289067,115.892657103225));
#33949=CARTESIAN_POINT('Ctrl Pts',(90.2367028620415,-35.3780577995155,115.945306610955));
#33950=CARTESIAN_POINT('Ctrl Pts',(89.7060412337264,-34.741006622201,115.997956118686));
#33951=CARTESIAN_POINT('Ctrl Pts',(89.1753796054112,-34.1039554448865,116.050605626417));
#33952=CARTESIAN_POINT('Ctrl Pts',(88.2998239360969,-33.7541999196487,116.103255134148));
#33953=CARTESIAN_POINT('Ctrl Pts',(87.4762940740561,-33.8502963951874,116.155904641879));
#33954=CARTESIAN_POINT('Ctrl Pts',(86.6527642120154,-33.9463928707262,116.20855414961));
#33955=CARTESIAN_POINT('Ctrl Pts',(85.881260157248,-34.4883413470415,116.26120365734));
#33956=CARTESIAN_POINT('Ctrl Pts',(85.5115315408654,-35.2304577237047,116.313853165071));
#33957=CARTESIAN_POINT('Ctrl Pts',(85.3393327604376,-35.5760937641259,116.33837434255));
#33958=CARTESIAN_POINT('Ctrl Pts',(85.2542859874774,-35.9651496671849,116.362895520029));
#33959=CARTESIAN_POINT('Ctrl Pts',(85.2549234958158,-36.3544693504482,116.387416697508));
#33960=CARTESIAN_POINT('Origin',(87.7685555885722,-36.3549260746835,114.));
#33961=CARTESIAN_POINT('',(85.2502276901495,-36.3571029251275,117.387416697508));
#33962=CARTESIAN_POINT('',(85.2470013985646,-36.3545560533907,117.112583302492));
#33963=CARTESIAN_POINT('',(85.2510555885723,-36.3549260746835,114.));
#33964=CARTESIAN_POINT('Ctrl Pts',(85.2470013985646,-36.3545560533907,117.112583302492));
#33965=CARTESIAN_POINT('Ctrl Pts',(85.246959225422,-36.3341987570445,117.111290696434));
#33966=CARTESIAN_POINT('Ctrl Pts',(85.2471846617478,-36.3138424184026,117.109998090376));
#33967=CARTESIAN_POINT('Ctrl Pts',(85.2476805824931,-36.2934926714317,117.108705484318));
#33968=CARTESIAN_POINT('Ctrl Pts',(85.2678800724692,-35.464621296564,117.056055976587));
#33969=CARTESIAN_POINT('Ctrl Pts',(85.7368234124319,-34.6466857522417,117.003406468856));
#33970=CARTESIAN_POINT('Ctrl Pts',(86.4419222703427,-34.2104846792909,116.950756961126));
#33971=CARTESIAN_POINT('Ctrl Pts',(87.1470211282534,-33.7742836063402,116.898107453395));
#33972=CARTESIAN_POINT('Ctrl Pts',(88.0882755041123,-33.7198170047611,116.845457945664));
#33973=CARTESIAN_POINT('Ctrl Pts',(88.8389820401025,-34.0717764801159,116.792808437933));
#33974=CARTESIAN_POINT('Ctrl Pts',(89.5896885760928,-34.4237359554708,116.740158930202));
#33975=CARTESIAN_POINT('Ctrl Pts',(90.1498472722143,-35.1821215077596,116.687509422471));
#33976=CARTESIAN_POINT('Ctrl Pts',(90.2655187018088,-36.0031305794793,116.634859914741));
#33977=CARTESIAN_POINT('Ctrl Pts',(90.3811901314033,-36.824139651199,116.58221040701));
#33978=CARTESIAN_POINT('Ctrl Pts',(90.0523742944708,-37.7077722423495,116.529560899279));
#33979=CARTESIAN_POINT('Ctrl Pts',(89.4281348504437,-38.253446954968,116.476911391548));
#33980=CARTESIAN_POINT('Ctrl Pts',(88.8038954064167,-38.7991216675865,116.424261883817));
#33981=CARTESIAN_POINT('Ctrl Pts',(87.8842323552952,-39.0068385016729,116.371612376086));
#33982=CARTESIAN_POINT('Ctrl Pts',(87.0860609561614,-38.7824321892052,116.318962868356));
#33983=CARTESIAN_POINT('Ctrl Pts',(86.2878895570277,-38.5580258767375,116.266313360625));
#33984=CARTESIAN_POINT('Ctrl Pts',(85.6112098098817,-37.9014964177156,116.213663852894));
#33985=CARTESIAN_POINT('Ctrl Pts',(85.3627841879501,-37.1104714586667,116.161014345163));
#33986=CARTESIAN_POINT('Ctrl Pts',(85.2866105609152,-36.867923046239,116.144870664273));
#33987=CARTESIAN_POINT('Ctrl Pts',(85.2507010392491,-36.6127294760279,116.128726983382));
#33988=CARTESIAN_POINT('Ctrl Pts',(85.2527054364363,-36.3569864150889,116.112583302492));
#33989=CARTESIAN_POINT('Ctrl Pts',(85.2549234958158,-36.3544693504482,116.387416697508));
#33990=CARTESIAN_POINT('Ctrl Pts',(85.2556547839073,-36.8010593493897,116.41554502776));
#33991=CARTESIAN_POINT('Ctrl Pts',(85.3691334424466,-37.2479964426169,116.443673358012));
#33992=CARTESIAN_POINT('Ctrl Pts',(85.5931440674471,-37.6301403068955,116.471801688264));
#33993=CARTESIAN_POINT('Ctrl Pts',(86.0124383884093,-38.3454222364119,116.524451195994));
#33994=CARTESIAN_POINT('Ctrl Pts',(86.8189802083315,-38.8337018184338,116.577100703725));
#33995=CARTESIAN_POINT('Ctrl Pts',(87.6471360580823,-38.8736249296274,116.629750211456));
#33996=CARTESIAN_POINT('Ctrl Pts',(88.4752919078331,-38.913548040821,116.682399719187));
#33997=CARTESIAN_POINT('Ctrl Pts',(89.3250617874126,-38.5051146811863,116.735049226918));
#33998=CARTESIAN_POINT('Ctrl Pts',(89.8112154442046,-37.8334819033445,116.787698734649));
#33999=CARTESIAN_POINT('Ctrl Pts',(90.2973691009967,-37.1618491255027,116.840348242379));
#34000=CARTESIAN_POINT('Ctrl Pts',(90.4199065350014,-36.2270169294537,116.89299775011));
#34001=CARTESIAN_POINT('Ctrl Pts',(90.1232772639163,-35.4527772754578,116.945647257841));
#34002=CARTESIAN_POINT('Ctrl Pts',(89.8266479928313,-34.6785376214619,116.998296765572));
#34003=CARTESIAN_POINT('Ctrl Pts',(89.1108520166566,-34.064890509519,117.050946273303));
#34004=CARTESIAN_POINT('Ctrl Pts',(88.3003845562159,-33.890023526213,117.103595781033));
#34005=CARTESIAN_POINT('Ctrl Pts',(87.4899170957753,-33.715156542907,117.156245288764));
#34006=CARTESIAN_POINT('Ctrl Pts',(86.5847781510686,-33.979069688238,117.208894796495));
#34007=CARTESIAN_POINT('Ctrl Pts',(85.9952986984001,-34.5621219510453,117.261544304226));
#34008=CARTESIAN_POINT('Ctrl Pts',(85.5255305233118,-35.0267681677034,117.303501768653));
#34009=CARTESIAN_POINT('Ctrl Pts',(85.2562320265711,-35.6940939103772,117.345459233081));
#34010=CARTESIAN_POINT('Ctrl Pts',(85.2502276901495,-36.3571029251275,117.387416697508));
#34011=CARTESIAN_POINT('Origin',(87.7685555885722,-36.3549260746835,114.));
#34012=CARTESIAN_POINT('',(85.2484784217854,-36.3532397189627,118.387416697508));
#34013=CARTESIAN_POINT('',(85.2536734366772,-36.353216668893,118.112583302492));
#34014=CARTESIAN_POINT('',(85.2510555885723,-36.3549260746835,114.));
#34015=CARTESIAN_POINT('Ctrl Pts',(85.2536734366772,-36.353216668893,118.112583302492));
#34016=CARTESIAN_POINT('Ctrl Pts',(85.2517947257147,-36.0562311247923,118.093854409486));
#34017=CARTESIAN_POINT('Ctrl Pts',(85.3004695466827,-35.7598413530357,118.075125516479));
#34018=CARTESIAN_POINT('Ctrl Pts',(85.4024432551376,-35.4830904910718,118.056396623473));
#34019=CARTESIAN_POINT('Ctrl Pts',(85.689105448669,-34.7051055540288,118.003747115742));
#34020=CARTESIAN_POINT('Ctrl Pts',(86.3969620113841,-34.082317068762,117.951097608011));
#34021=CARTESIAN_POINT('Ctrl Pts',(87.2051169348331,-33.8970567244546,117.89844810028));
#34022=CARTESIAN_POINT('Ctrl Pts',(88.0132718582821,-33.7117963801472,117.845798592549));
#34023=CARTESIAN_POINT('Ctrl Pts',(88.9217251424651,-33.9640641767992,117.793149084819));
#34024=CARTESIAN_POINT('Ctrl Pts',(89.5186433056692,-34.5394983449801,117.740499577088));
#34025=CARTESIAN_POINT('Ctrl Pts',(90.1155614688732,-35.1149325131609,117.687850069357));
#34026=CARTESIAN_POINT('Ctrl Pts',(90.4009445110984,-36.0135330528707,117.635200561626));
#34027=CARTESIAN_POINT('Ctrl Pts',(90.2454183699218,-36.8279330742855,117.582551053895));
#34028=CARTESIAN_POINT('Ctrl Pts',(90.0898922287453,-37.6423330957004,117.529901546165));
#34029=CARTESIAN_POINT('Ctrl Pts',(89.493456904167,-38.3725325988204,117.477252038434));
#34030=CARTESIAN_POINT('Ctrl Pts',(88.7264972807027,-38.6875067429112,117.424602530703));
#34031=CARTESIAN_POINT('Ctrl Pts',(87.9595376572385,-39.0024808870021,117.371953022972));
#34032=CARTESIAN_POINT('Ctrl Pts',(87.0220537348881,-38.9022296720638,117.319303515241));
#34033=CARTESIAN_POINT('Ctrl Pts',(86.3390395937077,-38.4322004618881,117.26665400751));
#34034=CARTESIAN_POINT('Ctrl Pts',(85.6727942364087,-37.9737110102155,117.215297105838));
#34035=CARTESIAN_POINT('Ctrl Pts',(85.2486769917781,-37.1633776276781,117.163940204165));
#34036=CARTESIAN_POINT('Ctrl Pts',(85.2470013985646,-36.3545560533907,117.112583302492));
#34037=CARTESIAN_POINT('Ctrl Pts',(85.2502276901495,-36.3571029251275,117.387416697508));
#34038=CARTESIAN_POINT('Ctrl Pts',(85.2486976018588,-36.5260578701663,117.398108740812));
#34039=CARTESIAN_POINT('Ctrl Pts',(85.2642654687678,-36.6947324929201,117.408800784115));
#34040=CARTESIAN_POINT('Ctrl Pts',(85.2979709317325,-36.8597013491054,117.419492827418));
#34041=CARTESIAN_POINT('Ctrl Pts',(85.463942578364,-37.6720371040742,117.472142335149));
#34042=CARTESIAN_POINT('Ctrl Pts',(86.0697058322574,-38.394517233728,117.52479184288));
#34043=CARTESIAN_POINT('Ctrl Pts',(86.8406471339867,-38.699616357898,117.577441350611));
#34044=CARTESIAN_POINT('Ctrl Pts',(87.6115884357159,-39.004715482068,117.630090858342));
#34045=CARTESIAN_POINT('Ctrl Pts',(88.5477077852809,-38.8924336007541,117.682740366073));
#34046=CARTESIAN_POINT('Ctrl Pts',(89.2246297109517,-38.4136719974215,117.735389873803));
#34047=CARTESIAN_POINT('Ctrl Pts',(89.9015516366226,-37.9349103940889,117.788039381534));
#34048=CARTESIAN_POINT('Ctrl Pts',(90.3192761383994,-37.0896690687376,117.840688889265));
#34049=CARTESIAN_POINT('Ctrl Pts',(90.2884341656518,-36.2611253227459,117.893338396996));
#34050=CARTESIAN_POINT('Ctrl Pts',(90.2575921929042,-35.4325815767542,117.945987904727));
#34051=CARTESIAN_POINT('Ctrl Pts',(89.7781837456322,-34.6207354101222,117.998637412457));
#34052=CARTESIAN_POINT('Ctrl Pts',(89.0675413531486,-34.1936249369889,118.051286920188));
#34053=CARTESIAN_POINT('Ctrl Pts',(88.3568989606649,-33.7665144638555,118.103936427919));
#34054=CARTESIAN_POINT('Ctrl Pts',(87.4150226229695,-33.7241396842209,118.15658593565));
#34055=CARTESIAN_POINT('Ctrl Pts',(86.6688976547862,-34.085710559864,118.209235443381));
#34056=CARTESIAN_POINT('Ctrl Pts',(85.9227726866028,-34.4472814355072,118.261884951112));
#34057=CARTESIAN_POINT('Ctrl Pts',(85.3723990879314,-35.2127979664282,118.314534458842));
#34058=CARTESIAN_POINT('Ctrl Pts',(85.2672803603705,-36.0352248747766,118.367183966573));
#34059=CARTESIAN_POINT('Ctrl Pts',(85.2538149674186,-36.1405752890371,118.373928210218));
#34060=CARTESIAN_POINT('Ctrl Pts',(85.2476556902819,-36.2468595365593,118.380672453863));
#34061=CARTESIAN_POINT('Ctrl Pts',(85.2484784217854,-36.3532397189627,118.387416697508));
#34062=CARTESIAN_POINT('Origin',(87.7685555885722,-36.3549260746835,114.));
#34063=CARTESIAN_POINT('',(85.2548912454248,-36.3543846295848,119.387416697508));
#34064=CARTESIAN_POINT('',(85.2528440754712,-36.356949956235,119.112583302492));
#34065=CARTESIAN_POINT('',(85.2510555885723,-36.3549260746835,114.));
#34066=CARTESIAN_POINT('Ctrl Pts',(85.2528440754712,-36.356949956235,119.112583302492));
#34067=CARTESIAN_POINT('Ctrl Pts',(85.2572372892863,-35.7839527661201,119.076418122537));
#34068=CARTESIAN_POINT('Ctrl Pts',(85.4516401968638,-35.2082587139073,119.040252942582));
#34069=CARTESIAN_POINT('Ctrl Pts',(85.8105044563501,-34.7660205958344,119.004087762628));
#34070=CARTESIAN_POINT('Ctrl Pts',(86.3329414144337,-34.1222074240089,118.951438254897));
#34071=CARTESIAN_POINT('Ctrl Pts',(87.2039332985395,-33.761237137223,118.898788747166));
#34072=CARTESIAN_POINT('Ctrl Pts',(88.0286291841641,-33.8467501269348,118.846139239435));
#34073=CARTESIAN_POINT('Ctrl Pts',(88.8533250697887,-33.9322631166466,118.793489731704));
#34074=CARTESIAN_POINT('Ctrl Pts',(89.6317249569322,-34.4642593828561,118.740840223974));
#34075=CARTESIAN_POINT('Ctrl Pts',(90.0109530931821,-35.2015665076848,118.688190716243));
#34076=CARTESIAN_POINT('Ctrl Pts',(90.390181229432,-35.9388736325135,118.635541208512));
#34077=CARTESIAN_POINT('Ctrl Pts',(90.3702376147884,-36.8814916159616,118.582891700781));
#34078=CARTESIAN_POINT('Ctrl Pts',(89.960163383942,-37.60209892972,118.53024219305));
#34079=CARTESIAN_POINT('Ctrl Pts',(89.5500891530956,-38.3227062434784,118.477592685319));
#34080=CARTESIAN_POINT('Ctrl Pts',(88.7498843060464,-38.8213028875472,118.424943177589));
#34081=CARTESIAN_POINT('Ctrl Pts',(87.9223095415073,-38.8718576552712,118.372293669858));
#34082=CARTESIAN_POINT('Ctrl Pts',(87.0947347769682,-38.9224124229951,118.319644162127));
#34083=CARTESIAN_POINT('Ctrl Pts',(86.2397900949392,-38.5249253143742,118.266994654396));
#34084=CARTESIAN_POINT('Ctrl Pts',(85.7450516660987,-37.8595910656541,118.214345146665));
#34085=CARTESIAN_POINT('Ctrl Pts',(85.4263054449591,-37.4309346985486,118.180424531941));
#34086=CARTESIAN_POINT('Ctrl Pts',(85.2570760419841,-36.8910985510045,118.146503917216));
#34087=CARTESIAN_POINT('Ctrl Pts',(85.2536734366772,-36.353216668893,118.112583302492));
#34088=CARTESIAN_POINT('Ctrl Pts',(85.2484784217854,-36.3532397189627,118.387416697508));
#34089=CARTESIAN_POINT('Ctrl Pts',(85.2540784132636,-37.0773254169046,118.433321961594));
#34090=CARTESIAN_POINT('Ctrl Pts',(85.583152017838,-37.8058557387736,118.47922722568));
#34091=CARTESIAN_POINT('Ctrl Pts',(86.1334932425857,-38.2746025447411,118.525132489766));
#34092=CARTESIAN_POINT('Ctrl Pts',(86.7646887088122,-38.8122160205814,118.577781997496));
#34093=CARTESIAN_POINT('Ctrl Pts',(87.6869434977158,-39.0081056864863,118.630431505227));
#34094=CARTESIAN_POINT('Ctrl Pts',(88.4821674255945,-38.7734679428665,118.683081012958));
#34095=CARTESIAN_POINT('Ctrl Pts',(89.2773913534732,-38.5388301992467,118.735730520689));
#34096=CARTESIAN_POINT('Ctrl Pts',(89.9455844203271,-37.8736650461022,118.78838002842));
#34097=CARTESIAN_POINT('Ctrl Pts',(90.1838314597843,-37.0795149872964,118.841029536151));
#34098=CARTESIAN_POINT('Ctrl Pts',(90.4220784992415,-36.2853649284906,118.893679043881));
#34099=CARTESIAN_POINT('Ctrl Pts',(90.2303795113019,-35.3622299640236,118.946328551612));
#34100=CARTESIAN_POINT('Ctrl Pts',(89.6956383182525,-34.7285992988272,118.998978059343));
#34101=CARTESIAN_POINT('Ctrl Pts',(89.1608971252032,-34.0949686336307,119.051627567074));
#34102=CARTESIAN_POINT('Ctrl Pts',(88.283113727044,-33.7508422677048,119.104277074805));
#34103=CARTESIAN_POINT('Ctrl Pts',(87.4602178765024,-33.852224642133,119.156926582536));
#34104=CARTESIAN_POINT('Ctrl Pts',(86.6373220259608,-33.9536070165613,119.209576090266));
#34105=CARTESIAN_POINT('Ctrl Pts',(85.8693137230369,-34.5004981313436,119.262225597997));
#34106=CARTESIAN_POINT('Ctrl Pts',(85.5043578581278,-35.2449732445367,119.314875105728));
#34107=CARTESIAN_POINT('Ctrl Pts',(85.3367432528447,-35.5868910330671,119.339055636321));
#34108=CARTESIAN_POINT('Ctrl Pts',(85.2541454125404,-35.9704856625546,119.363236166915));
#34109=CARTESIAN_POINT('Ctrl Pts',(85.2548912454248,-36.3543846295848,119.387416697508));
#34110=CARTESIAN_POINT('Origin',(87.7685555885722,-36.3549260746835,114.));
#34111=CARTESIAN_POINT('',(85.2503884478834,-36.3571243043025,120.387416697508));
#34112=CARTESIAN_POINT('',(85.2469700844899,-36.3546528234761,120.112583302492));
#34113=CARTESIAN_POINT('',(85.2510555885723,-36.3549260746835,114.));
#34114=CARTESIAN_POINT('Ctrl Pts',(85.2469700844899,-36.3546528234761,120.112583302492));
#34115=CARTESIAN_POINT('Ctrl Pts',(85.2469467853652,-36.3396608858275,120.11163134332));
#34116=CARTESIAN_POINT('Ctrl Pts',(85.2470690489527,-36.3246693383145,120.110679384147));
#34117=CARTESIAN_POINT('Ctrl Pts',(85.2473380380648,-36.3096804239763,120.109727424975));
#34118=CARTESIAN_POINT('Ctrl Pts',(85.2622148781136,-35.4806963832532,120.057077917244));
#34119=CARTESIAN_POINT('Ctrl Pts',(85.7258966860521,-34.6597667145453,120.004428409513));
#34120=CARTESIAN_POINT('Ctrl Pts',(86.4281801872503,-34.2190472204532,119.951778901782));
#34121=CARTESIAN_POINT('Ctrl Pts',(87.1304636884485,-33.778327726361,119.899129394052));
#34122=CARTESIAN_POINT('Ctrl Pts',(88.0713488829063,-33.7178184068845,119.846479886321));
#34123=CARTESIAN_POINT('Ctrl Pts',(88.8242998622034,-34.0649503288953,119.79383037859));
#34124=CARTESIAN_POINT('Ctrl Pts',(89.5772508415005,-34.4120822509062,119.741180870859));
#34125=CARTESIAN_POINT('Ctrl Pts',(90.1422676056369,-35.1668554144045,119.688531363128));
#34126=CARTESIAN_POINT('Ctrl Pts',(90.2632083545705,-35.9871048410839,119.635881855397));
#34127=CARTESIAN_POINT('Ctrl Pts',(90.3841491035041,-36.8073542677633,119.583232347667));
#34128=CARTESIAN_POINT('Ctrl Pts',(90.0610138372351,-37.6930799576239,119.530582839936));
#34129=CARTESIAN_POINT('Ctrl Pts',(89.4402910353544,-38.2427516588164,119.477933332205));
#34130=CARTESIAN_POINT('Ctrl Pts',(88.8195682334738,-38.7924233600089,119.425283824474));
#34131=CARTESIAN_POINT('Ctrl Pts',(87.9012578959816,-39.0060410725332,119.372634316743));
#34132=CARTESIAN_POINT('Ctrl Pts',(87.1016620398446,-38.7867644448508,119.319984809013));
#34133=CARTESIAN_POINT('Ctrl Pts',(86.3020661837075,-38.5674878171683,119.267335301282));
#34134=CARTESIAN_POINT('Ctrl Pts',(85.6211848089255,-37.915316849279,119.214685793551));
#34135=CARTESIAN_POINT('Ctrl Pts',(85.3676851375653,-37.1259033369019,119.16203628582));
#34136=CARTESIAN_POINT('Ctrl Pts',(85.2883155127783,-36.8787414611372,119.145551958044));
#34137=CARTESIAN_POINT('Ctrl Pts',(85.2508416196115,-36.6181258582599,119.129067630268));
#34138=CARTESIAN_POINT('Ctrl Pts',(85.2528440754712,-36.356949956235,119.112583302492));
#34139=CARTESIAN_POINT('Ctrl Pts',(85.2548912454248,-36.3543846295848,119.387416697508));
#34140=CARTESIAN_POINT('Ctrl Pts',(85.2557693526794,-36.8063685458726,119.415885674645));
#34141=CARTESIAN_POINT('Ctrl Pts',(85.372174783394,-37.2587743214379,119.444354651783));
#34142=CARTESIAN_POINT('Ctrl Pts',(85.6013770646085,-37.6440823482595,119.47282362892));
#34143=CARTESIAN_POINT('Ctrl Pts',(86.0252555628928,-38.3566572271855,119.525473136651));
#34144=CARTESIAN_POINT('Ctrl Pts',(86.8349159863556,-38.8397478734336,119.578122644382));
#34145=CARTESIAN_POINT('Ctrl Pts',(87.6633111164763,-38.8743526092352,119.630772152113));
#34146=CARTESIAN_POINT('Ctrl Pts',(88.4917062465969,-38.9089573450367,119.683421659844));
#34147=CARTESIAN_POINT('Ctrl Pts',(89.3388360833753,-38.4950761703916,119.736071167575));
#34148=CARTESIAN_POINT('Ctrl Pts',(89.820667151996,-37.8203355743053,119.788720675305));
#34149=CARTESIAN_POINT('Ctrl Pts',(90.3024982206167,-37.1455949782191,119.841370183036));
#34150=CARTESIAN_POINT('Ctrl Pts',(90.4190305210798,-36.2099949606916,119.894019690767));
#34151=CARTESIAN_POINT('Ctrl Pts',(90.1174360005457,-35.4376760716325,119.946669198498));
#34152=CARTESIAN_POINT('Ctrl Pts',(89.8158414800116,-34.6653571825733,119.999318706229));
#34153=CARTESIAN_POINT('Ctrl Pts',(89.0961201384803,-34.0563194219826,120.051968213959));
#34154=CARTESIAN_POINT('Ctrl Pts',(88.2845465091856,-33.8866597493,120.10461772169));
#34155=CARTESIAN_POINT('Ctrl Pts',(87.4729728798908,-33.7170000766173,120.157267229421));
#34156=CARTESIAN_POINT('Ctrl Pts',(86.5695469628327,-33.9867184918427,120.209916737152));
#34157=CARTESIAN_POINT('Ctrl Pts',(85.9838235547468,-34.5735444080027,120.262566244883));
#34158=CARTESIAN_POINT('Ctrl Pts',(85.5208383293416,-35.0374011112114,120.304183062425));
#34159=CARTESIAN_POINT('Ctrl Pts',(85.2563573256464,-35.6993902681898,120.345799879966));
#34160=CARTESIAN_POINT('Ctrl Pts',(85.2503884478834,-36.3571243043025,120.387416697508));
#34161=CARTESIAN_POINT('Origin',(87.7685555885722,-36.3549260746835,114.));
#34162=CARTESIAN_POINT('',(85.2483528516199,-36.3533471753035,121.387416697508));
#34163=CARTESIAN_POINT('',(85.2535610703604,-36.3531642914838,121.112583302492));
#34164=CARTESIAN_POINT('',(85.2510555885723,-36.3549260746835,114.));
#34165=CARTESIAN_POINT('',(89.6820215852375,-34.7189388713088,122.));
#34166=CARTESIAN_POINT('Ctrl Pts',(85.2483528516199,-36.3533471753035,121.387416697508));
#34167=CARTESIAN_POINT('Ctrl Pts',(85.253810887375,-37.0825701143354,121.43366260848));
#34168=CARTESIAN_POINT('Ctrl Pts',(85.5883405994922,-37.816044282996,121.479908519451));
#34169=CARTESIAN_POINT('Ctrl Pts',(86.1458176873049,-38.2848775789271,121.526154430423));
#34170=CARTESIAN_POINT('Ctrl Pts',(86.7804877290006,-38.8186294657434,121.578803938153));
#34171=CARTESIAN_POINT('Ctrl Pts',(87.7041221542809,-39.0093775992254,121.631453445884));
#34172=CARTESIAN_POINT('Ctrl Pts',(88.4977390504798,-38.7692237839494,121.684102953615));
#34173=CARTESIAN_POINT('Ctrl Pts',(89.2913559466788,-38.5290699686735,121.736752461346));
#34174=CARTESIAN_POINT('Ctrl Pts',(89.9549553137964,-37.8580142046394,121.789401969077));
#34175=CARTESIAN_POINT('Ctrl Pts',(90.1879205700165,-37.0637282318536,121.842051476808));
#34176=CARTESIAN_POINT('Ctrl Pts',(90.4208858262365,-36.2694422590678,121.894700984538));
#34177=CARTESIAN_POINT('Ctrl Pts',(90.223216971559,-35.3519260775303,121.947350492269));
#34178=CARTESIAN_POINT('Ctrl Pts',(89.6820215852375,-34.7189388713087,122.));
#34179=CARTESIAN_POINT('',(85.8514455075092,-34.7163982291022,122.));
#34180=CARTESIAN_POINT('Origin',(87.7685555885722,-36.3549260746835,122.));
#34181=CARTESIAN_POINT('Ctrl Pts',(85.8514366626952,-34.7163920625306,122.));
#34182=CARTESIAN_POINT('Ctrl Pts',(86.3742572722501,-34.1076767185939,121.949053726697));
#34183=CARTESIAN_POINT('Ctrl Pts',(87.2139816526743,-33.767500880252,121.898107453395));
#34184=CARTESIAN_POINT('Ctrl Pts',(88.012652402947,-33.8452637608976,121.847161180092));
#34185=CARTESIAN_POINT('Ctrl Pts',(88.838024292095,-33.9256264080613,121.794511672361));
#34186=CARTESIAN_POINT('Ctrl Pts',(89.619551657879,-34.4523399348362,121.74186216463));
#34187=CARTESIAN_POINT('Ctrl Pts',(90.003436239116,-35.1871265566876,121.6892126569));
#34188=CARTESIAN_POINT('Ctrl Pts',(90.3873208203531,-35.9219131785391,121.636563149169));
#34189=CARTESIAN_POINT('Ctrl Pts',(90.3735626170432,-36.864772895467,121.583913641438));
#34190=CARTESIAN_POINT('Ctrl Pts',(89.9681578782027,-37.5880326323531,121.531264133707));
#34191=CARTESIAN_POINT('Ctrl Pts',(89.5627531393622,-38.3112923692392,121.478614625976));
#34192=CARTESIAN_POINT('Ctrl Pts',(88.765701864991,-38.8149521260835,121.425965118245));
#34193=CARTESIAN_POINT('Ctrl Pts',(87.9384522287811,-38.8708030839915,121.373315610515));
#34194=CARTESIAN_POINT('Ctrl Pts',(87.1112025925711,-38.9266540418996,121.320666102784));
#34195=CARTESIAN_POINT('Ctrl Pts',(86.2537545945224,-38.5346962008713,121.268016595053));
#34196=CARTESIAN_POINT('Ctrl Pts',(85.7547622998719,-37.8725604668736,121.215367087322));
#34197=CARTESIAN_POINT('Ctrl Pts',(85.430046907739,-37.4416807382379,121.181105825712));
#34198=CARTESIAN_POINT('Ctrl Pts',(85.2571251526924,-36.8963899829528,121.146844564102));
#34199=CARTESIAN_POINT('Ctrl Pts',(85.2535610703604,-36.3531642914838,121.112583302492));
#34200=CARTESIAN_POINT('Origin',(87.7685555885722,-36.3549260746835,124.208423447177));
#34201=CARTESIAN_POINT('',(84.6902859389797,-36.3541125877401,107.791576552823));
#34202=CARTESIAN_POINT('',(84.6999263673563,-36.3546117753717,107.708423447177));
#34203=CARTESIAN_POINT('',(84.6950555885722,-36.3549260746832,124.208423447177));
#34204=CARTESIAN_POINT('',(88.5623548711046,-39.3241490284293,107.));
#34205=CARTESIAN_POINT('Ctrl Pts',(84.6999263673563,-36.3546117753717,107.708423447177));
#34206=CARTESIAN_POINT('Ctrl Pts',(84.6996065051311,-35.8594362872189,107.682880329042));
#34207=CARTESIAN_POINT('Ctrl Pts',(85.0458587978589,-34.3441196884525,107.604687703175));
#34208=CARTESIAN_POINT('Ctrl Pts',(87.4170212023543,-32.7460640346786,107.473845569577));
#34209=CARTESIAN_POINT('Ctrl Pts',(90.6005809066571,-34.0865213418793,107.315897046385));
#34210=CARTESIAN_POINT('Ctrl Pts',(91.2113486315107,-37.4887066956559,107.157948523193));
#34211=CARTESIAN_POINT('Ctrl Pts',(89.5445934608762,-39.0615549760519,107.052649507731));
#34212=CARTESIAN_POINT('Ctrl Pts',(88.5623548711045,-39.3241490284294,107.));
#34213=CARTESIAN_POINT('',(86.9747563060389,-39.3241490284291,107.));
#34214=CARTESIAN_POINT('Origin',(87.7685555885722,-36.3549260746835,107.));
#34215=CARTESIAN_POINT('Ctrl Pts',(84.6902859389797,-36.3541125877401,107.791576552823));
#34216=CARTESIAN_POINT('Ctrl Pts',(84.6901298701282,-36.3096037501105,107.789262006108));
#34217=CARTESIAN_POINT('Ctrl Pts',(84.7110895869572,-35.252794330332,107.734297951662));
#34218=CARTESIAN_POINT('Ctrl Pts',(85.9203584351496,-33.2347633730889,107.626684389485));
#34219=CARTESIAN_POINT('Ctrl Pts',(89.3710240668315,-33.1013877392709,107.468735866293));
#34220=CARTESIAN_POINT('Ctrl Pts',(91.3686331795228,-35.9187012093704,107.3107873431));
#34221=CARTESIAN_POINT('Ctrl Pts',(90.1161178614875,-39.0952438942321,107.154542054336));
#34222=CARTESIAN_POINT('Ctrl Pts',(87.9198088452516,-39.5801184192997,107.050946273303));
#34223=CARTESIAN_POINT('Ctrl Pts',(86.9728422903211,-39.3292375489681,107.));
#34224=CARTESIAN_POINT('Origin',(87.7685555885722,-36.3549260746835,124.208423447177));
#34225=CARTESIAN_POINT('',(84.6986441861196,-36.3530606800421,108.791576552823));
#34226=CARTESIAN_POINT('',(84.6934625360053,-36.357484352344,108.708423447177));
#34227=CARTESIAN_POINT('',(84.6950555885722,-36.3549260746832,124.208423447177));
#34228=CARTESIAN_POINT('Ctrl Pts',(84.6934625360053,-36.357484352344,108.708423447177));
#34229=CARTESIAN_POINT('Ctrl Pts',(84.7008503927251,-35.5287362890068,108.665444042093));
#34230=CARTESIAN_POINT('Ctrl Pts',(85.4724994656418,-33.6726457957907,108.569815129278));
#34231=CARTESIAN_POINT('Ctrl Pts',(88.6015534510421,-32.8253527833924,108.421536708732));
#34232=CARTESIAN_POINT('Ctrl Pts',(91.1794497561267,-35.1229272408109,108.26358818554));
#34233=CARTESIAN_POINT('Ctrl Pts',(90.6647257407023,-38.5375841171318,108.105639662347));
#34234=CARTESIAN_POINT('Ctrl Pts',(87.5242687243508,-39.9731544640366,107.947691139155));
#34235=CARTESIAN_POINT('Ctrl Pts',(85.0771139192411,-38.4267875479491,107.815285734098));
#34236=CARTESIAN_POINT('Ctrl Pts',(84.7002658055582,-36.8800926359444,107.735529836772));
#34237=CARTESIAN_POINT('Ctrl Pts',(84.6999263673563,-36.3546117753717,107.708423447177));
#34238=CARTESIAN_POINT('Ctrl Pts',(84.6986441861196,-36.3530606800421,108.791576552823));
#34239=CARTESIAN_POINT('Ctrl Pts',(84.6965000548819,-35.9705777414508,108.771825719159));
#34240=CARTESIAN_POINT('Ctrl Pts',(84.9394944552829,-34.5711418157649,108.699425377765));
#34241=CARTESIAN_POINT('Ctrl Pts',(87.0264678663363,-32.8051171947587,108.57437552864));
#34242=CARTESIAN_POINT('Ctrl Pts',(90.3353208987278,-33.792977483537,108.416427005448));
#34243=CARTESIAN_POINT('Ctrl Pts',(91.3169639431757,-37.1036892864445,108.258478482255));
#34244=CARTESIAN_POINT('Ctrl Pts',(89.0813770537997,-39.7354983689013,108.100529959063));
#34245=CARTESIAN_POINT('Ctrl Pts',(85.70568896844,-39.3086385235238,107.944895982585));
#34246=CARTESIAN_POINT('Ctrl Pts',(84.6936800029274,-37.3220561563539,107.841911513838));
#34247=CARTESIAN_POINT('Ctrl Pts',(84.6902859389797,-36.3541125877401,107.791576552823));
#34248=CARTESIAN_POINT('Origin',(87.7685555885722,-36.3549260746835,124.208423447177));
#34249=CARTESIAN_POINT('',(84.6967209343146,-36.3575187349746,109.791576552823));
#34250=CARTESIAN_POINT('',(84.6924245878599,-36.3526580233552,109.708423447177));
#34251=CARTESIAN_POINT('',(84.6950555885722,-36.3549260746832,124.208423447177));
#34252=CARTESIAN_POINT('Ctrl Pts',(84.6924245878599,-36.3526580233552,109.708423447177));
#34253=CARTESIAN_POINT('Ctrl Pts',(84.6911854664029,-36.203038268201,109.700657262876));
#34254=CARTESIAN_POINT('Ctrl Pts',(84.7688483649364,-35.0403882407784,109.640241570843));
#34255=CARTESIAN_POINT('Ctrl Pts',(86.2502054927865,-33.0615290694994,109.527176371079));
#34256=CARTESIAN_POINT('Ctrl Pts',(89.6962563926914,-33.2831482377538,109.369227847887));
#34257=CARTESIAN_POINT('Ctrl Pts',(91.3945200278872,-36.2898545193635,109.211279324695));
#34258=CARTESIAN_POINT('Ctrl Pts',(89.805231108493,-39.3555600803365,109.053330801502));
#34259=CARTESIAN_POINT('Ctrl Pts',(86.3693522399246,-39.7006802402578,108.89538227831));
#34260=CARTESIAN_POINT('Ctrl Pts',(84.7918203783131,-37.7438433959039,108.780413160201));
#34261=CARTESIAN_POINT('Ctrl Pts',(84.6918003135367,-36.5439475857204,108.718093549824));
#34262=CARTESIAN_POINT('Ctrl Pts',(84.6934625360053,-36.357484352344,108.708423447177));
#34263=CARTESIAN_POINT('Ctrl Pts',(84.6967209343146,-36.3575187349745,109.791576552823));
#34264=CARTESIAN_POINT('Ctrl Pts',(84.7025803795521,-35.6385126094882,109.754389432211));
#34265=CARTESIAN_POINT('Ctrl Pts',(85.3117912843899,-33.8925909032789,109.664552803868));
#34266=CARTESIAN_POINT('Ctrl Pts',(88.2120005461565,-32.7555923274475,109.522066667795));
#34267=CARTESIAN_POINT('Ctrl Pts',(91.0248782320717,-34.7586147002439,109.364118144602));
#34268=CARTESIAN_POINT('Ctrl Pts',(90.8853471879654,-38.2089641874212,109.20616962141));
#34269=CARTESIAN_POINT('Ctrl Pts',(87.9199160465446,-39.9783134162844,109.048221098218));
#34270=CARTESIAN_POINT('Ctrl Pts',(85.2052267935342,-38.6520010530253,108.910023408688));
#34271=CARTESIAN_POINT('Ctrl Pts',(84.7022156340872,-36.9901569033004,108.82447522689));
#34272=CARTESIAN_POINT('Ctrl Pts',(84.6986441861196,-36.3530606800421,108.791576552823));
#34273=CARTESIAN_POINT('Origin',(87.7685555885722,-36.3549260746835,124.208423447177));
#34274=CARTESIAN_POINT('',(84.6902141559912,-36.3542412678362,110.791576552823));
#34275=CARTESIAN_POINT('',(84.6998362604058,-36.3545776583035,110.708423447177));
#34276=CARTESIAN_POINT('',(84.6950555885722,-36.3549260746832,124.208423447177));
#34277=CARTESIAN_POINT('Ctrl Pts',(84.6998362604058,-36.3545776583035,110.708423447177));
#34278=CARTESIAN_POINT('Ctrl Pts',(84.6993369649495,-35.8660461176461,110.683220975927));
#34279=CARTESIAN_POINT('Ctrl Pts',(85.0389980437079,-34.3575980587991,110.605368996946));
#34280=CARTESIAN_POINT('Ctrl Pts',(87.3945229855647,-32.747717976947,110.474867510234));
#34281=CARTESIAN_POINT('Ctrl Pts',(90.584585262429,-34.069794239593,110.316918987042));
#34282=CARTESIAN_POINT('Ctrl Pts',(91.221439085307,-37.4637300323244,110.158970463849));
#34283=CARTESIAN_POINT('Ctrl Pts',(88.7276684448237,-39.8523470110271,110.001021940657));
#34284=CARTESIAN_POINT('Ctrl Pts',(85.5296731500474,-39.1084280856274,109.850839601766));
#34285=CARTESIAN_POINT('Ctrl Pts',(84.6995858767197,-37.217359606649,109.753306770606));
#34286=CARTESIAN_POINT('Ctrl Pts',(84.6924245878599,-36.3526580233552,109.708423447177));
#34287=CARTESIAN_POINT('Ctrl Pts',(84.6902141559913,-36.3542412678362,110.791576552823));
#34288=CARTESIAN_POINT('Ctrl Pts',(84.6900985120232,-36.3162849815638,110.789602652993));
#34289=CARTESIAN_POINT('Ctrl Pts',(84.7078624516269,-35.2660376004022,110.734979245433));
#34290=CARTESIAN_POINT('Ctrl Pts',(85.9003809608462,-33.2465872009442,110.627706330142));
#34291=CARTESIAN_POINT('Ctrl Pts',(89.3500610269517,-33.0913869620613,110.46975780695));
#34292=CARTESIAN_POINT('Ctrl Pts',(91.3658382115574,-35.895138379632,110.311809283757));
#34293=CARTESIAN_POINT('Ctrl Pts',(90.1200686479678,-39.1157653183575,110.153860760565));
#34294=CARTESIAN_POINT('Ctrl Pts',(86.7422537121608,-39.8332232781445,109.995912237372));
#34295=CARTESIAN_POINT('Ctrl Pts',(84.8711430366209,-37.9705915317642,109.875150834792));
#34296=CARTESIAN_POINT('Ctrl Pts',(84.6942845797629,-36.6564811410552,109.807038939942));
#34297=CARTESIAN_POINT('Ctrl Pts',(84.6967209343146,-36.3575187349745,109.791576552823));
#34298=CARTESIAN_POINT('Origin',(87.7685555885722,-36.3549260746835,124.208423447177));
#34299=CARTESIAN_POINT('',(84.6985185386966,-36.3529840193472,111.791576552823));
#34300=CARTESIAN_POINT('',(84.6936554590675,-36.3575218684262,111.708423447177));
#34301=CARTESIAN_POINT('',(84.6950555885722,-36.3549260746832,124.208423447177));
#34302=CARTESIAN_POINT('Ctrl Pts',(84.6936554590675,-36.3575218684262,111.708423447177));
#34303=CARTESIAN_POINT('Ctrl Pts',(84.7010363386306,-35.5352098446355,111.665784688979));
#34304=CARTESIAN_POINT('Ctrl Pts',(85.4624963011915,-33.6854549308403,111.570496423049));
#34305=CARTESIAN_POINT('Ctrl Pts',(88.5788817046039,-32.8200679121307,111.422558649389));
#34306=CARTESIAN_POINT('Ctrl Pts',(91.1714506588609,-35.1010697096973,111.264610126197));
#34307=CARTESIAN_POINT('Ctrl Pts',(90.6787181473369,-38.5189049390048,111.106661603004));
#34308=CARTESIAN_POINT('Ctrl Pts',(87.5474297522212,-39.9747263466277,110.948713079812));
#34309=CARTESIAN_POINT('Ctrl Pts',(85.0842717295461,-38.4399664305319,110.815967027869));
#34310=CARTESIAN_POINT('Ctrl Pts',(84.700380023772,-36.8866184603822,110.735870483658));
#34311=CARTESIAN_POINT('Ctrl Pts',(84.6998362604058,-36.3545776583035,110.708423447177));
#34312=CARTESIAN_POINT('Ctrl Pts',(84.6985185386966,-36.3529840193472,111.791576552823));
#34313=CARTESIAN_POINT('Ctrl Pts',(84.6963188618144,-35.9771365370321,111.772166366045));
#34314=CARTESIAN_POINT('Ctrl Pts',(84.9337531498146,-34.5844970198617,111.700106671536));
#34315=CARTESIAN_POINT('Ctrl Pts',(87.0036900983236,-32.8099538921628,111.575397469297));
#34316=CARTESIAN_POINT('Ctrl Pts',(90.3188172011552,-33.7765520327001,111.417448946105));
#34317=CARTESIAN_POINT('Ctrl Pts',(91.3216996625609,-37.0808834993901,111.259500422912));
#34318=CARTESIAN_POINT('Ctrl Pts',(89.1030544560686,-39.7270114481203,111.10155189972));
#34319=CARTESIAN_POINT('Ctrl Pts',(85.7173072338234,-39.3209114482164,110.945577276356));
#34320=CARTESIAN_POINT('Ctrl Pts',(84.6931830646942,-37.3286868055508,110.842252160724));
#34321=CARTESIAN_POINT('Ctrl Pts',(84.6902141559913,-36.3542412678362,110.791576552823));
#34322=CARTESIAN_POINT('Origin',(87.7685555885722,-36.3549260746835,124.208423447177));
#34323=CARTESIAN_POINT('',(84.6968970266175,-36.35748207472,112.791576552823));
#34324=CARTESIAN_POINT('',(84.6922488060663,-36.3527237795464,112.708423447177));
#34325=CARTESIAN_POINT('',(84.6950555885722,-36.3549260746832,124.208423447177));
#34326=CARTESIAN_POINT('Ctrl Pts',(84.6922488060663,-36.3527237795464,112.708423447177));
#34327=CARTESIAN_POINT('Ctrl Pts',(84.6910879425595,-36.2096880917331,112.700997909761));
#34328=CARTESIAN_POINT('Ctrl Pts',(84.7648942734634,-35.0536859391401,112.640922864614));
#34329=CARTESIAN_POINT('Ctrl Pts',(86.2290898398163,-33.0713463433522,112.528198311736));
#34330=CARTESIAN_POINT('Ctrl Pts',(89.6764928893144,-33.2708336798222,112.370249788544));
#34331=CARTESIAN_POINT('Ctrl Pts',(91.3940272155189,-36.2665737922834,112.212301265351));
#34332=CARTESIAN_POINT('Ctrl Pts',(89.8244566813072,-39.3424202320825,112.054352742159));
#34333=CARTESIAN_POINT('Ctrl Pts',(86.3908631537158,-39.7095965798975,111.896404218966));
#34334=CARTESIAN_POINT('Ctrl Pts',(84.7960899574643,-37.7571592451098,111.781094453973));
#34335=CARTESIAN_POINT('Ctrl Pts',(84.6919225723758,-36.5505847073844,111.71843419671));
#34336=CARTESIAN_POINT('Ctrl Pts',(84.6936554590675,-36.3575218684262,111.708423447177));
#34337=CARTESIAN_POINT('Ctrl Pts',(84.6968970266175,-36.35748207472,112.791576552823));
#34338=CARTESIAN_POINT('Ctrl Pts',(84.7025960788243,-35.6449587514818,112.754730079097));
#34339=CARTESIAN_POINT('Ctrl Pts',(85.3029473196868,-33.9056538204367,112.66523409764));
#34340=CARTESIAN_POINT('Ctrl Pts',(88.1888800917162,-32.7528191488601,112.523088608452));
#34341=CARTESIAN_POINT('Ctrl Pts',(91.0145611839512,-34.7377388042116,112.365140085259));
#34342=CARTESIAN_POINT('Ctrl Pts',(90.8971877256538,-38.1889129731724,112.207191562067));
#34343=CARTESIAN_POINT('Ctrl Pts',(87.9431786617096,-39.9772669994637,112.049243038874));
#34344=CARTESIAN_POINT('Ctrl Pts',(85.2133168410851,-38.6651863273541,111.91070470246));
#34345=CARTESIAN_POINT('Ctrl Pts',(84.702285414653,-36.9966107519078,111.824815873776));
#34346=CARTESIAN_POINT('Ctrl Pts',(84.6985185386966,-36.3529840193472,111.791576552823));
#34347=CARTESIAN_POINT('Origin',(87.7685555885722,-36.3549260746835,124.208423447177));
#34348=CARTESIAN_POINT('',(84.6901549196512,-36.3543571629991,113.791576552823));
#34349=CARTESIAN_POINT('',(84.6998103833004,-36.354472739616,113.708423447177));
#34350=CARTESIAN_POINT('',(84.6950555885722,-36.3549260746832,124.208423447177));
#34351=CARTESIAN_POINT('Ctrl Pts',(84.6998103833004,-36.354472739616,113.708423447177));
#34352=CARTESIAN_POINT('Ctrl Pts',(84.6991692065907,-35.8725545473769,113.683561622813));
#34353=CARTESIAN_POINT('Ctrl Pts',(85.0323509698878,-34.3709240683999,113.606050290717));
#34354=CARTESIAN_POINT('Ctrl Pts',(87.3713688180184,-32.7501940024069,113.475889450891));
#34355=CARTESIAN_POINT('Ctrl Pts',(90.5698543841637,-34.0517596235948,113.317940927699));
#34356=CARTESIAN_POINT('Ctrl Pts',(91.2284875299979,-37.4415362183437,113.159992404506));
#34357=CARTESIAN_POINT('Ctrl Pts',(88.7501056136147,-39.8461164435895,113.002043881314));
#34358=CARTESIAN_POINT('Ctrl Pts',(85.5401350753849,-39.1211064337822,112.851520895538));
#34359=CARTESIAN_POINT('Ctrl Pts',(84.6993188474424,-37.2238582627538,112.753647417492));
#34360=CARTESIAN_POINT('Ctrl Pts',(84.6922488060663,-36.3527237795464,112.708423447177));
#34361=CARTESIAN_POINT('Ctrl Pts',(84.6901549196511,-36.3543571629991,113.791576552823));
#34362=CARTESIAN_POINT('Ctrl Pts',(84.6900742363842,-36.32295282532,113.789943299879));
#34363=CARTESIAN_POINT('Ctrl Pts',(84.7046794034006,-35.2792757725774,113.735660539204));
#34364=CARTESIAN_POINT('Ctrl Pts',(85.8804608339871,-33.2586468252107,113.628728270799));
#34365=CARTESIAN_POINT('Ctrl Pts',(89.3290732451296,-33.0812993952069,113.470779747607));
#34366=CARTESIAN_POINT('Ctrl Pts',(91.3628117580707,-35.8720497126298,113.312831224414));
#34367=CARTESIAN_POINT('Ctrl Pts',(90.1377475164876,-39.100609341506,113.154882701222));
#34368=CARTESIAN_POINT('Ctrl Pts',(86.7646090095788,-39.8397414585361,112.996934178029));
#34369=CARTESIAN_POINT('Ctrl Pts',(84.876265246591,-37.9839423426147,112.875832128563));
#34370=CARTESIAN_POINT('Ctrl Pts',(84.6944527678673,-36.6630752337838,112.807379586827));
#34371=CARTESIAN_POINT('Ctrl Pts',(84.6968970266175,-36.35748207472,112.791576552823));
#34372=CARTESIAN_POINT('Origin',(87.7685555885722,-36.3549260746835,124.208423447177));
#34373=CARTESIAN_POINT('',(84.6983876365698,-36.3529100689715,114.791576552823));
#34374=CARTESIAN_POINT('',(84.6938496423748,-36.3575550147471,114.708423447177));
#34375=CARTESIAN_POINT('',(84.6950555885722,-36.3549260746832,124.208423447177));
#34376=CARTESIAN_POINT('Ctrl Pts',(84.6938496423747,-36.3575550147471,114.708423447177));
#34377=CARTESIAN_POINT('Ctrl Pts',(84.7012114735458,-35.5416795963333,114.666125335864));
#34378=CARTESIAN_POINT('Ctrl Pts',(85.4525661295013,-33.6982784575714,114.571177716821));
#34379=CARTESIAN_POINT('Ctrl Pts',(88.5561676812683,-32.8149376799226,114.423580590046));
#34380=CARTESIAN_POINT('Ctrl Pts',(91.1633294990928,-35.0792455739108,114.265632066854));
#34381=CARTESIAN_POINT('Ctrl Pts',(90.6925530596296,-38.5001741798809,114.107683543661));
#34382=CARTESIAN_POINT('Ctrl Pts',(87.5706770425218,-39.9760715736404,113.949735020469));
#34383=CARTESIAN_POINT('Ctrl Pts',(85.0913691036972,-38.4532614664624,113.816648321641));
#34384=CARTESIAN_POINT('Ctrl Pts',(84.7005270167674,-36.8931053812909,113.736211130544));
#34385=CARTESIAN_POINT('Ctrl Pts',(84.6998103833004,-36.354472739616,113.708423447177));
#34386=CARTESIAN_POINT('Ctrl Pts',(84.6983876365698,-36.3529100689715,114.791576552823));
#34387=CARTESIAN_POINT('Ctrl Pts',(84.6961381340608,-35.9836982647827,114.77250701293));
#34388=CARTESIAN_POINT('Ctrl Pts',(84.9280665202918,-34.5978523566551,114.700787965308));
#34389=CARTESIAN_POINT('Ctrl Pts',(86.9809436051873,-32.8149381712244,114.576419409954));
#34390=CARTESIAN_POINT('Ctrl Pts',(90.3022088923736,-33.7602299596934,114.418470886762));
#34391=CARTESIAN_POINT('Ctrl Pts',(91.3262877865851,-37.0580538015087,114.260522363569));
#34392=CARTESIAN_POINT('Ctrl Pts',(89.124679100392,-39.7183731180749,114.102573840377));
#34393=CARTESIAN_POINT('Ctrl Pts',(85.7289941295958,-39.3331819473256,113.946258570128));
#34394=CARTESIAN_POINT('Ctrl Pts',(84.6926751404897,-37.3353023979011,113.84259280761));
#34395=CARTESIAN_POINT('Ctrl Pts',(84.6901549196511,-36.3543571629991,113.791576552823));
#34396=CARTESIAN_POINT('Origin',(87.7685555885722,-36.3549260746835,124.208423447177));
#34397=CARTESIAN_POINT('',(84.6970698119725,-36.3574414495534,115.791576552823));
#34398=CARTESIAN_POINT('',(84.6920769038732,-36.3527935649553,115.708423447177));
#34399=CARTESIAN_POINT('',(84.6950555885722,-36.3549260746832,124.208423447177));
#34400=CARTESIAN_POINT('Ctrl Pts',(84.6920769038732,-36.3527935649552,115.708423447177));
#34401=CARTESIAN_POINT('Ctrl Pts',(84.6909943683417,-36.2163395637745,115.701338556647));
#34402=CARTESIAN_POINT('Ctrl Pts',(84.7609870881033,-35.0669804686883,115.641604158386));
#34403=CARTESIAN_POINT('Ctrl Pts',(86.2080377154374,-33.0812989408716,115.529220252393));
#34404=CARTESIAN_POINT('Ctrl Pts',(89.6566506052006,-33.2586463954901,115.371271729201));
#34405=CARTESIAN_POINT('Ctrl Pts',(91.3933851672007,-36.2432964661436,115.213323206008));
#34406=CARTESIAN_POINT('Ctrl Pts',(89.8435969944667,-39.3291577077992,115.055374682816));
#34407=CARTESIAN_POINT('Ctrl Pts',(86.4124318885398,-39.718373584875,114.897426159624));
#34408=CARTESIAN_POINT('Ctrl Pts',(84.8004067708206,-37.7704790356049,114.781775747744));
#34409=CARTESIAN_POINT('Ctrl Pts',(84.6920480197858,-36.557219955365,114.718774843595));
#34410=CARTESIAN_POINT('Ctrl Pts',(84.6938496423747,-36.3575550147471,114.708423447177));
#34411=CARTESIAN_POINT('Ctrl Pts',(84.6970698119725,-36.3574414495534,115.791576552823));
#34412=CARTESIAN_POINT('Ctrl Pts',(84.7026034041402,-35.6514048376539,115.755070725982));
#34413=CARTESIAN_POINT('Ctrl Pts',(85.2941695333478,-33.9187288980288,115.665915391411));
#34414=CARTESIAN_POINT('Ctrl Pts',(88.1657423040033,-32.7501945026947,115.524110549109));
#34415=CARTESIAN_POINT('Ctrl Pts',(91.0041103112496,-34.7169295455148,115.366162025916));
#34416=CARTESIAN_POINT('Ctrl Pts',(90.9088992563929,-38.1687862239197,115.208213502724));
#34417=CARTESIAN_POINT('Ctrl Pts',(87.9664341071585,-39.9760710710749,115.050264979531));
#34418=CARTESIAN_POINT('Ctrl Pts',(85.2214707589106,-38.678362824672,114.911385996231));
#34419=CARTESIAN_POINT('Ctrl Pts',(84.7023488344975,-37.0030631707532,114.825156520661));
#34420=CARTESIAN_POINT('Ctrl Pts',(84.6983876365698,-36.3529100689715,114.791576552823));
#34421=CARTESIAN_POINT('Origin',(87.7685555885722,-36.3549260746835,124.208423447177));
#34422=CARTESIAN_POINT('',(84.6901060143961,-36.3544743326999,116.791576552823));
#34423=CARTESIAN_POINT('',(84.6997777386867,-36.354368481064,116.708423447177));
#34424=CARTESIAN_POINT('',(84.6950555885722,-36.3549260746832,124.208423447177));
#34425=CARTESIAN_POINT('Ctrl Pts',(84.6997777386867,-36.354368481064,116.708423447177));
#34426=CARTESIAN_POINT('Ctrl Pts',(84.6989994340679,-35.8790659799677,116.683902269698));
#34427=CARTESIAN_POINT('Ctrl Pts',(85.025762237394,-34.3842532656316,116.606731584489));
#34428=CARTESIAN_POINT('Ctrl Pts',(87.3482310270943,-32.7528186489366,116.476911391548));
#34429=CARTESIAN_POINT('Ctrl Pts',(90.5550080077946,-34.0338199678859,116.318962868355));
#34430=CARTESIAN_POINT('Ctrl Pts',(91.2353933261053,-37.4192976006176,116.161014345163));
#34431=CARTESIAN_POINT('Ctrl Pts',(88.7725023068986,-39.8397419421814,116.003065821971));
#34432=CARTESIAN_POINT('Ctrl Pts',(85.5506678195318,-39.1337640107994,115.852202189309));
#34433=CARTESIAN_POINT('Ctrl Pts',(84.699038947519,-37.2303617224901,115.753988064378));
#34434=CARTESIAN_POINT('Ctrl Pts',(84.6920769038732,-36.3527935649552,115.708423447177));
#34435=CARTESIAN_POINT('Ctrl Pts',(84.6901060143962,-36.3544743326999,116.791576552823));
#34436=CARTESIAN_POINT('Ctrl Pts',(84.6900545271454,-36.3296210455818,116.790283946765));
#34437=CARTESIAN_POINT('Ctrl Pts',(84.7015400140162,-35.2925101923577,116.736341832976));
#34438=CARTESIAN_POINT('Ctrl Pts',(85.860618552627,-33.2708341078515,116.629750211456));
#34439=CARTESIAN_POINT('Ctrl Pts',(89.3080211236725,-33.0713467990688,116.471801688264));
#34440=CARTESIAN_POINT('Ctrl Pts',(91.3596371147702,-35.8489809539364,116.313853165071));
#34441=CARTESIAN_POINT('Ctrl Pts',(90.1553287038718,-39.0853401621602,116.155904641879));
#34442=CARTESIAN_POINT('Ctrl Pts',(86.7870056997543,-39.8461159590596,115.997956118686));
#34443=CARTESIAN_POINT('Ctrl Pts',(84.8814396668467,-37.997294205502,115.876513422334));
#34444=CARTESIAN_POINT('Ctrl Pts',(84.6946227356051,-36.6696663940604,115.807720233713));
#34445=CARTESIAN_POINT('Ctrl Pts',(84.6970698119725,-36.3574414495534,115.791576552823));
#34446=CARTESIAN_POINT('Origin',(87.7685555885722,-36.3549260746835,124.208423447177));
#34447=CARTESIAN_POINT('',(84.6982515989598,-36.3528391397487,117.791576552823));
#34448=CARTESIAN_POINT('',(84.6940448454532,-36.3575836913029,117.708423447177));
#34449=CARTESIAN_POINT('',(84.6950555885722,-36.3549260746832,124.208423447177));
#34450=CARTESIAN_POINT('Ctrl Pts',(84.6940448454532,-36.3575836913029,117.708423447177));
#34451=CARTESIAN_POINT('Ctrl Pts',(84.7013752637221,-35.5481464691242,117.66646598275));
#34452=CARTESIAN_POINT('Ctrl Pts',(85.4427052641639,-33.7111195302489,117.571859010592));
#34453=CARTESIAN_POINT('Ctrl Pts',(88.5334211849751,-32.8099534001692,117.424602530703));
#34454=CARTESIAN_POINT('Ctrl Pts',(91.1550683739797,-35.0574740340002,117.26665400751));
#34455=CARTESIAN_POINT('Ctrl Pts',(90.7062674165854,-38.4813549728958,117.108705484318));
#34456=CARTESIAN_POINT('Ctrl Pts',(87.5939324911983,-39.9772675021952,116.950756961125));
#34457=CARTESIAN_POINT('Ctrl Pts',(85.0985268023629,-38.4665514839768,116.817329615412));
#34458=CARTESIAN_POINT('Ctrl Pts',(84.7006705346943,-36.8995896773883,116.736551777429));
#34459=CARTESIAN_POINT('Ctrl Pts',(84.6997777386867,-36.354368481064,116.708423447177));
#34460=CARTESIAN_POINT('Ctrl Pts',(84.6982515989598,-36.3528391397487,117.791576552823));
#34461=CARTESIAN_POINT('Ctrl Pts',(84.6959579671254,-35.9902631438032,117.772847659816));
#34462=CARTESIAN_POINT('Ctrl Pts',(84.9224342902478,-34.6112079283206,117.701469259079));
#34463=CARTESIAN_POINT('Ctrl Pts',(86.9582295850041,-32.8200684027204,117.577441350611));
#34464=CARTESIAN_POINT('Ctrl Pts',(90.2854961219689,-33.7440148650956,117.419492827418));
#34465=CARTESIAN_POINT('Ctrl Pts',(91.3307292265714,-37.0351951139114,117.261544304226));
#34466=CARTESIAN_POINT('Ctrl Pts',(89.1462478322224,-39.7095961143156,117.103595781033));
#34467=CARTESIAN_POINT('Ctrl Pts',(85.740754335939,-39.3454246844624,116.946939863899));
#34468=CARTESIAN_POINT('Ctrl Pts',(84.6921516691098,-37.3419274046254,116.842933454495));
#34469=CARTESIAN_POINT('Ctrl Pts',(84.6901060143962,-36.3544743326999,116.791576552823));
#34470=CARTESIAN_POINT('Origin',(87.7685555885722,-36.3549260746835,124.208423447177));
#34471=CARTESIAN_POINT('',(84.6972390699959,-36.357396938615,118.791576552823));
#34472=CARTESIAN_POINT('',(84.6919092441355,-36.3528672805194,118.708423447177));
#34473=CARTESIAN_POINT('',(84.6950555885722,-36.3549260746832,124.208423447177));
#34474=CARTESIAN_POINT('Ctrl Pts',(84.6919092441355,-36.3528672805194,118.708423447177));
#34475=CARTESIAN_POINT('Ctrl Pts',(84.6909048090706,-36.2229926069874,118.701679203533));
#34476=CARTESIAN_POINT('Ctrl Pts',(84.7571266102654,-35.0802717724924,118.642285452157));
#34477=CARTESIAN_POINT('Ctrl Pts',(86.1870499307028,-33.0913865091248,118.53024219305));
#34478=CARTESIAN_POINT('Ctrl Pts',(89.6367304755765,-33.2465867695503,118.372293669858));
#34479=CARTESIAN_POINT('Ctrl Pts',(91.3925936684549,-36.2200237425119,118.214345146665));
#34480=CARTESIAN_POINT('Ctrl Pts',(89.8626517544002,-39.3157725569713,118.056396623473));
#34481=CARTESIAN_POINT('Ctrl Pts',(86.4340565358644,-39.7270119161192,117.89844810028));
#34482=CARTESIAN_POINT('Ctrl Pts',(84.8047722789476,-37.7838014397254,117.782457041515));
#34483=CARTESIAN_POINT('Ctrl Pts',(84.6921768310097,-36.5638530154645,117.719115490481));
#34484=CARTESIAN_POINT('Ctrl Pts',(84.6940448454532,-36.3575836913029,117.708423447177));
#34485=CARTESIAN_POINT('Ctrl Pts',(84.6972390699959,-36.357396938615,118.791576552823));
#34486=CARTESIAN_POINT('Ctrl Pts',(84.702602542751,-35.6578510145562,118.755411372868));
#34487=CARTESIAN_POINT('Ctrl Pts',(85.2854577178621,-33.9318158343519,118.666596685182));
#34488=CARTESIAN_POINT('Ctrl Pts',(88.1425881396678,-32.7477184775748,118.525132489766));
#34489=CARTESIAN_POINT('Ctrl Pts',(90.9935260381413,-34.6961878212031,118.367183966573));
#34490=CARTESIAN_POINT('Ctrl Pts',(90.9204813116975,-38.1485846896768,118.209235443381));
#34491=CARTESIAN_POINT('Ctrl Pts',(87.9896813942331,-39.9747258442494,118.051286920188));
#34492=CARTESIAN_POINT('Ctrl Pts',(85.2296888152546,-38.6915299918233,117.912067290002));
#34493=CARTESIAN_POINT('Ctrl Pts',(84.7024056833334,-37.0095143988034,117.825497167547));
#34494=CARTESIAN_POINT('Ctrl Pts',(84.6982515989598,-36.3528391397487,117.791576552823));
#34495=CARTESIAN_POINT('Origin',(87.7685555885722,-36.3549260746835,124.208423447177));
#34496=CARTESIAN_POINT('',(84.6900677844821,-36.3545924748475,119.791576552823));
#34497=CARTESIAN_POINT('',(84.6997383656671,-36.3542650492571,119.708423447177));
#34498=CARTESIAN_POINT('',(84.6950555885722,-36.3549260746832,124.208423447177));
#34499=CARTESIAN_POINT('Ctrl Pts',(84.6997383656671,-36.3542650492571,119.708423447177));
#34500=CARTESIAN_POINT('Ctrl Pts',(84.6988278125906,-35.8855804513753,119.684242916584));
#34501=CARTESIAN_POINT('Ctrl Pts',(85.0192316092183,-34.3975854238898,119.60741287826));
#34502=CARTESIAN_POINT('Ctrl Pts',(87.3251105694465,-32.7555918278425,119.477933332205));
#34503=CARTESIAN_POINT('Ctrl Pts',(90.540046745306,-34.0159760014353,119.319984809013));
#34504=CARTESIAN_POINT('Ctrl Pts',(91.2421561865363,-37.3970151036668,119.16203628582));
#34505=CARTESIAN_POINT('Ctrl Pts',(88.7948576074191,-39.8332237608939,119.004087762628));
#34506=CARTESIAN_POINT('Ctrl Pts',(85.5612715353611,-39.1464004416207,118.85288348308));
#34507=CARTESIAN_POINT('Ctrl Pts',(84.698746016254,-37.2368702170138,118.754328711263));
#34508=CARTESIAN_POINT('Ctrl Pts',(84.6919092441355,-36.3528672805194,118.708423447177));
#34509=CARTESIAN_POINT('Ctrl Pts',(84.6900677844821,-36.3545924748475,119.791576552823));
#34510=CARTESIAN_POINT('Ctrl Pts',(84.690039339652,-36.3362895074741,119.79062459365));
#34511=CARTESIAN_POINT('Ctrl Pts',(84.6984439817714,-35.3057407212815,119.737023126747));
#34512=CARTESIAN_POINT('Ctrl Pts',(85.8408550522478,-33.2831486644916,119.630772152113));
#34513=CARTESIAN_POINT('Ctrl Pts',(89.2869054734986,-33.0615295263651,119.472823628921));
#34514=CARTESIAN_POINT('Ctrl Pts',(91.3563144402191,-35.8259330830824,119.314875105728));
#34515=CARTESIAN_POINT('Ctrl Pts',(90.1728114719436,-39.0699583952412,119.156926582536));
#34516=CARTESIAN_POINT('Ctrl Pts',(86.8094428654503,-39.8523465256606,118.998978059343));
#34517=CARTESIAN_POINT('Ctrl Pts',(84.8866665229963,-38.0106469951155,118.877194716105));
#34518=CARTESIAN_POINT('Ctrl Pts',(84.694794363706,-36.6762545890117,118.808060880599));
#34519=CARTESIAN_POINT('Ctrl Pts',(84.6972390699959,-36.357396938615,118.791576552823));
#34520=CARTESIAN_POINT('Origin',(87.7685555885722,-36.3549260746835,124.208423447177));
#34521=CARTESIAN_POINT('',(84.69811441609,-36.3527751945784,120.791576552823));
#34522=CARTESIAN_POINT('',(84.6942411071791,-36.3576097921547,120.708423447177));
#34523=CARTESIAN_POINT('',(84.6950555885722,-36.3549260746832,124.208423447177));
#34524=CARTESIAN_POINT('Ctrl Pts',(84.6942411071791,-36.3576097921547,120.708423447177));
#34525=CARTESIAN_POINT('Ctrl Pts',(84.701528235602,-35.5546125488608,120.666806629636));
#34526=CARTESIAN_POINT('Ctrl Pts',(85.4329130412516,-33.7239751716799,120.572540304363));
#34527=CARTESIAN_POINT('Ctrl Pts',(88.5106434141715,-32.8051166986153,120.42562447136));
#34528=CARTESIAN_POINT('Ctrl Pts',(91.1466674974244,-35.0357552970371,120.267675948167));
#34529=CARTESIAN_POINT('Ctrl Pts',(90.7198607143381,-38.4624484297529,120.109727424975));
#34530=CARTESIAN_POINT('Ctrl Pts',(87.6171951095654,-39.9783139196497,119.951778901782));
#34531=CARTESIAN_POINT('Ctrl Pts',(85.105745062361,-38.4798362972224,119.818010909183));
#34532=CARTESIAN_POINT('Ctrl Pts',(84.7008104064405,-36.9060714312672,119.736892424315));
#34533=CARTESIAN_POINT('Ctrl Pts',(84.6997383656671,-36.3542650492571,119.708423447177));
#34534=CARTESIAN_POINT('Ctrl Pts',(84.69811441609,-36.3527751945784,120.791576552823));
#34535=CARTESIAN_POINT('Ctrl Pts',(84.6957790852043,-35.9968317519122,120.773188306702));
#34536=CARTESIAN_POINT('Ctrl Pts',(84.9168438604484,-34.6245511594877,120.70215055285));
#34537=CARTESIAN_POINT('Ctrl Pts',(86.935557851387,-32.8253532951761,120.578463291268));
#34538=CARTESIAN_POINT('Ctrl Pts',(90.2686752620247,-33.7279030795955,120.420514768075));
#34539=CARTESIAN_POINT('Ctrl Pts',(91.3350258987628,-37.0123104885738,120.262566244883));
#34540=CARTESIAN_POINT('Ctrl Pts',(89.167758741363,-39.7006797728369,120.10461772169));
#34541=CARTESIAN_POINT('Ctrl Pts',(85.7525884657271,-39.3576397118412,119.94762115767));
#34542=CARTESIAN_POINT('Ctrl Pts',(84.6916125229857,-37.3485621449868,119.843274101381));
#34543=CARTESIAN_POINT('Ctrl Pts',(84.6900677844821,-36.3545924748475,119.791576552823));
#34544=CARTESIAN_POINT('Origin',(87.7685555885722,-36.3549260746835,124.208423447177));
#34545=CARTESIAN_POINT('',(84.6982768768212,-36.3579423122256,121.791576552823));
#34546=CARTESIAN_POINT('',(84.691755941294,-36.3529984690253,121.708423447177));
#34547=CARTESIAN_POINT('',(84.6950555885722,-36.3549260746832,124.208423447177));
#34548=CARTESIAN_POINT('',(86.9747563060389,-39.3241490284291,122.));
#34549=CARTESIAN_POINT('Ctrl Pts',(86.9747563060389,-39.3241490284291,122.));
#34550=CARTESIAN_POINT('Ctrl Pts',(85.9925177162673,-39.0615549760513,121.947350492269));
#34551=CARTESIAN_POINT('Ctrl Pts',(84.8928208152446,-38.023819855789,121.877876009877));
#34552=CARTESIAN_POINT('Ctrl Pts',(84.6959356655866,-36.6834182514038,121.808401527484));
#34553=CARTESIAN_POINT('Ctrl Pts',(84.6982768768212,-36.3579423122256,121.791576552823));
#34554=CARTESIAN_POINT('',(88.5642643959444,-39.3292255199611,122.));
#34555=CARTESIAN_POINT('Origin',(87.7685555885722,-36.3549260746835,122.));
#34556=CARTESIAN_POINT('Ctrl Pts',(88.5642690312351,-39.3292378429293,122.));
#34557=CARTESIAN_POINT('Ctrl Pts',(87.6173028025204,-39.5801183881388,121.949053726697));
#34558=CARTESIAN_POINT('Ctrl Pts',(85.5567536487794,-39.1252166604105,121.851861542423));
#34559=CARTESIAN_POINT('Ctrl Pts',(84.698419406197,-37.2432732269655,121.754669358149));
#34560=CARTESIAN_POINT('Ctrl Pts',(84.691755941294,-36.3529984690253,121.708423447177));
#34561=CARTESIAN_POINT('Origin',(36.3549260746835,87.7685555885722,114.));
#34562=CARTESIAN_POINT('',(33.8414156476497,87.7688130130942,107.387416697508));
#34563=CARTESIAN_POINT('',(33.8393353393333,87.7649829964101,107.112583302492));
#34564=CARTESIAN_POINT('',(33.8374260746835,87.7685555885722,114.));
#34565=CARTESIAN_POINT('',(34.4414600780189,89.4045427919477,107.));
#34566=CARTESIAN_POINT('Ctrl Pts',(33.8393353393333,87.7649829964101,107.112583302492));
#34567=CARTESIAN_POINT('Ctrl Pts',(33.844480764459,88.3576176201294,107.075055534995));
#34568=CARTESIAN_POINT('Ctrl Pts',(34.0557042465997,88.9533591488772,107.037527767497));
#34569=CARTESIAN_POINT('Ctrl Pts',(34.441460078019,89.4045427919478,107.));
#34570=CARTESIAN_POINT('',(33.8374260746835,87.7685555885722,107.));
#34571=CARTESIAN_POINT('Origin',(36.3549260746835,87.7685555885722,107.));
#34572=CARTESIAN_POINT('',(33.8374260746835,87.7685555885722,106.));
#34573=CARTESIAN_POINT('',(33.8374260746835,87.7685555885722,114.));
#34574=CARTESIAN_POINT('Origin',(36.3549260746835,87.7685555885722,106.));
#34575=CARTESIAN_POINT('',(38.2720364380598,89.4070835930084,107.));
#34576=CARTESIAN_POINT('Origin',(36.3549260746835,87.7685555885722,107.));
#34577=CARTESIAN_POINT('Ctrl Pts',(38.2720452848186,89.4070897608439,107.));
#34578=CARTESIAN_POINT('Ctrl Pts',(37.7492247595626,90.0158046540078,107.050946273303));
#34579=CARTESIAN_POINT('Ctrl Pts',(36.9095001729433,90.355981333293,107.101892546605));
#34580=CARTESIAN_POINT('Ctrl Pts',(36.1108292450109,90.2782186082904,107.152838819908));
#34581=CARTESIAN_POINT('Ctrl Pts',(35.2854571722635,90.1978561219734,107.205488327639));
#34582=CARTESIAN_POINT('Ctrl Pts',(34.5039296533554,89.6711420241569,107.25813783537));
#34583=CARTESIAN_POINT('Ctrl Pts',(34.1200450165566,88.9363551677885,107.3107873431));
#34584=CARTESIAN_POINT('Ctrl Pts',(33.933801857771,88.5798704011529,107.336330461236));
#34585=CARTESIAN_POINT('Ctrl Pts',(33.8411536469158,88.1744106374066,107.361873579372));
#34586=CARTESIAN_POINT('Ctrl Pts',(33.8414156476497,87.7688130130942,107.387416697508));
#34587=CARTESIAN_POINT('Origin',(36.3549260746835,87.7685555885722,114.));
#34588=CARTESIAN_POINT('',(33.8361211319563,87.7664601065544,108.387416697508));
#34589=CARTESIAN_POINT('',(33.8335191542225,87.7692219086659,108.112583302492));
#34590=CARTESIAN_POINT('',(33.8374260746835,87.7685555885722,114.));
#34591=CARTESIAN_POINT('Ctrl Pts',(33.8335191542225,87.7692219086659,108.112583302492));
#34592=CARTESIAN_POINT('Ctrl Pts',(33.8333913183595,87.8056790435099,108.110268755777));
#34593=CARTESIAN_POINT('Ctrl Pts',(33.834114269325,87.8421309416024,108.107954209062));
#34594=CARTESIAN_POINT('Ctrl Pts',(33.8357038858111,87.8785449414407,108.105639662347));
#34595=CARTESIAN_POINT('Ctrl Pts',(33.8718632447615,88.7068622761646,108.052990154616));
#34596=CARTESIAN_POINT('Ctrl Pts',(34.3564666344665,89.5155696857969,108.000340646886));
#34597=CARTESIAN_POINT('Ctrl Pts',(35.0698410055614,89.938131343294,107.947691139155));
#34598=CARTESIAN_POINT('Ctrl Pts',(35.7832153766562,90.3606930007911,107.895041631424));
#34599=CARTESIAN_POINT('Ctrl Pts',(36.725360729141,90.3971089061531,107.842392123693));
#34600=CARTESIAN_POINT('Ctrl Pts',(37.4691399227335,90.0307072168534,107.789742615962));
#34601=CARTESIAN_POINT('Ctrl Pts',(38.212919116326,89.6643055275537,107.737093108231));
#34602=CARTESIAN_POINT('Ctrl Pts',(38.7583321510263,88.8950862435923,107.684443600501));
#34603=CARTESIAN_POINT('Ctrl Pts',(38.8581857832189,88.0720989400536,107.63179409277));
#34604=CARTESIAN_POINT('Ctrl Pts',(38.9580394154116,87.2491116365149,107.579144585039));
#34605=CARTESIAN_POINT('Ctrl Pts',(38.6123336450968,86.3723563133988,107.526495077308));
#34606=CARTESIAN_POINT('Ctrl Pts',(37.9776637412943,85.8386044103528,107.473845569577));
#34607=CARTESIAN_POINT('Ctrl Pts',(37.3429938374919,85.3048525073067,107.421196061847));
#34608=CARTESIAN_POINT('Ctrl Pts',(36.4193598002019,85.1141040243308,107.368546554116));
#34609=CARTESIAN_POINT('Ctrl Pts',(35.625742673972,85.3542580662575,107.315897046385));
#34610=CARTESIAN_POINT('Ctrl Pts',(34.8321255477422,85.5944121081842,107.263247538654));
#34611=CARTESIAN_POINT('Ctrl Pts',(34.1685253325724,86.2654686750135,107.210598030923));
#34612=CARTESIAN_POINT('Ctrl Pts',(33.9355601185611,87.0597545443991,107.157948523192));
#34613=CARTESIAN_POINT('Ctrl Pts',(33.8686489620936,87.2878855394576,107.142826782959));
#34614=CARTESIAN_POINT('Ctrl Pts',(33.8372620003811,87.5261820383226,107.127705042725));
#34615=CARTESIAN_POINT('Ctrl Pts',(33.8393353393333,87.7649829964101,107.112583302492));
#34616=CARTESIAN_POINT('Ctrl Pts',(33.8414156476497,87.7688130130942,107.387416697508));
#34617=CARTESIAN_POINT('Ctrl Pts',(33.8416936831633,87.3383922960573,107.414523087103));
#34618=CARTESIAN_POINT('Ctrl Pts',(33.9466023816844,86.9078163275987,107.441629476698));
#34619=CARTESIAN_POINT('Ctrl Pts',(34.1553234354522,86.5354488974857,107.468735866293));
#34620=CARTESIAN_POINT('Ctrl Pts',(34.5607282458358,85.8121890984717,107.521385374024));
#34621=CARTESIAN_POINT('Ctrl Pts',(35.3577796212926,85.3085291153642,107.574034881755));
#34622=CARTESIAN_POINT('Ctrl Pts',(36.1850293919425,85.2526781151853,107.626684389485));
#34623=CARTESIAN_POINT('Ctrl Pts',(37.0122791625924,85.1968271150065,107.679333897216));
#34624=CARTESIAN_POINT('Ctrl Pts',(37.8697273284356,85.5887850977564,107.731983404947));
#34625=CARTESIAN_POINT('Ctrl Pts',(38.3687197115474,86.2509209612129,107.784632912678));
#34626=CARTESIAN_POINT('Ctrl Pts',(38.8677120946593,86.9130568246694,107.837282420409));
#34627=CARTESIAN_POINT('Ctrl Pts',(39.0082486950399,87.8453705688325,107.889931928139));
#34628=CARTESIAN_POINT('Ctrl Pts',(38.7265917130798,88.625184178848,107.94258143587));
#34629=CARTESIAN_POINT('Ctrl Pts',(38.4449347311198,89.4049977888636,107.995230943601));
#34630=CARTESIAN_POINT('Ctrl Pts',(37.7410841668192,90.0323112647315,108.047880451332));
#34631=CARTESIAN_POINT('Ctrl Pts',(36.9341334227374,90.2227550766996,108.100529959063));
#34632=CARTESIAN_POINT('Ctrl Pts',(36.1271826786556,90.4131988886677,108.153179466794));
#34633=CARTESIAN_POINT('Ctrl Pts',(35.2171317547927,90.1667730367359,108.205828974524));
#34634=CARTESIAN_POINT('Ctrl Pts',(34.6165318579143,89.5951843722506,108.258478482255));
#34635=CARTESIAN_POINT('Ctrl Pts',(34.1262437740546,89.1285790456046,108.301457887339));
#34636=CARTESIAN_POINT('Ctrl Pts',(33.842172516144,88.4452866270629,108.344437292424));
#34637=CARTESIAN_POINT('Ctrl Pts',(33.8361211319563,87.7664601065544,108.387416697508));
#34638=CARTESIAN_POINT('Origin',(36.3549260746835,87.7685555885722,114.));
#34639=CARTESIAN_POINT('',(33.8352709498557,87.7704133466358,109.387416697508));
#34640=CARTESIAN_POINT('',(33.8403653828405,87.7700835309277,109.112583302492));
#34641=CARTESIAN_POINT('',(33.8374260746835,87.7685555885722,114.));
#34642=CARTESIAN_POINT('Ctrl Pts',(33.8403653828405,87.7700835309277,109.112583302492));
#34643=CARTESIAN_POINT('Ctrl Pts',(33.8386091275561,88.0833748401921,109.092832468829));
#34644=CARTESIAN_POINT('Ctrl Pts',(33.8929063186919,88.3960793297297,109.073081635165));
#34645=CARTESIAN_POINT('Ctrl Pts',(34.0060458881645,88.6858055038443,109.053330801502));
#34646=CARTESIAN_POINT('Ctrl Pts',(34.3076403797772,89.4581243185282,109.000681293771));
#34647=CARTESIAN_POINT('Ctrl Pts',(35.0273616523211,90.0671620196572,108.94803178604));
#34648=CARTESIAN_POINT('Ctrl Pts',(35.8389352036457,90.2368216765074,108.89538227831));
#34649=CARTESIAN_POINT('Ctrl Pts',(36.6505087549703,90.4064813333576,108.842732770579));
#34650=CARTESIAN_POINT('Ctrl Pts',(37.5539345850756,90.136762945929,108.790083262848));
#34651=CARTESIAN_POINT('Ctrl Pts',(38.1396579370872,89.5499370852442,108.737433755117));
#34652=CARTESIAN_POINT('Ctrl Pts',(38.7253812890987,88.9631112245596,108.684784247386));
#34653=CARTESIAN_POINT('Ctrl Pts',(38.9934021630165,88.0591778906187,108.632134739655));
#34654=CARTESIAN_POINT('Ctrl Pts',(38.8222181837362,87.247925952964,108.579485231925));
#34655=CARTESIAN_POINT('Ctrl Pts',(38.6510342044558,86.4366740153094,108.526835724194));
#34656=CARTESIAN_POINT('Ctrl Pts',(38.0406453719773,85.7181034739408,108.474186216463));
#34657=CARTESIAN_POINT('Ctrl Pts',(37.2677605108997,85.4179582290087,108.421536708732));
#34658=CARTESIAN_POINT('Ctrl Pts',(36.4948756498221,85.1178129840766,108.368887201001));
#34659=CARTESIAN_POINT('Ctrl Pts',(35.5594947601453,85.236093035581,108.316237693271));
#34660=CARTESIAN_POINT('Ctrl Pts',(34.8856619794049,85.7191966912411,108.26358818554));
#34661=CARTESIAN_POINT('Ctrl Pts',(34.2414518393365,86.1810624279278,108.213253224524));
#34662=CARTESIAN_POINT('Ctrl Pts',(33.8362992291002,86.9763805072392,108.162918263508));
#34663=CARTESIAN_POINT('Ctrl Pts',(33.8335191542225,87.7692219086659,108.112583302492));
#34664=CARTESIAN_POINT('Ctrl Pts',(33.8361211319563,87.7664601065544,108.387416697508));
#34665=CARTESIAN_POINT('Ctrl Pts',(33.8347596076138,87.6137283011781,108.397086800155));
#34666=CARTESIAN_POINT('Ctrl Pts',(33.8474720723731,87.4612225695691,108.406756902801));
#34667=CARTESIAN_POINT('Ctrl Pts',(33.8750763409706,87.3114617765907,108.416427005448));
#34668=CARTESIAN_POINT('Ctrl Pts',(34.0253695907989,86.4960793224549,108.469076513179));
#34669=CARTESIAN_POINT('Ctrl Pts',(34.6171049603491,85.7620658912221,108.521726020909));
#34670=CARTESIAN_POINT('Ctrl Pts',(35.3820266721296,85.4421737589331,108.57437552864));
#34671=CARTESIAN_POINT('Ctrl Pts',(36.1469483839101,85.1222816266441,108.627025036371));
#34672=CARTESIAN_POINT('Ctrl Pts',(37.0850564379207,85.2165107932989,108.679674544102));
#34673=CARTESIAN_POINT('Ctrl Pts',(37.7710745652258,85.6821446532133,108.732324051833));
#34674=CARTESIAN_POINT('Ctrl Pts',(38.4570926925308,86.1477785131277,108.784973559563));
#34675=CARTESIAN_POINT('Ctrl Pts',(38.8910208931303,86.9848170663018,108.837623067294));
#34676=CARTESIAN_POINT('Ctrl Pts',(38.8761440504648,87.8138012467044,108.890272575025));
#34677=CARTESIAN_POINT('Ctrl Pts',(38.8612672077993,88.642785427107,108.942922082756));
#34678=CARTESIAN_POINT('Ctrl Pts',(38.397585321869,89.4637152347382,108.995571590487));
#34679=CARTESIAN_POINT('Ctrl Pts',(37.6953017022331,89.9044348032924,109.048221098218));
#34680=CARTESIAN_POINT('Ctrl Pts',(36.9930180825973,90.3451543718466,109.100870605948));
#34681=CARTESIAN_POINT('Ctrl Pts',(36.052132729256,90.4056637013238,109.153520113679));
#34682=CARTESIAN_POINT('Ctrl Pts',(35.2991816228838,90.0585317206909,109.20616962141));
#34683=CARTESIAN_POINT('Ctrl Pts',(34.5462305165115,89.711399740058,109.258819129141));
#34684=CARTESIAN_POINT('Ctrl Pts',(33.9812136571084,88.9566264493151,109.311468636872));
#34685=CARTESIAN_POINT('Ctrl Pts',(33.8602728877845,88.1363768842624,109.364118144603));
#34686=CARTESIAN_POINT('Ctrl Pts',(33.8424332470232,88.0153841234512,109.371884328904));
#34687=CARTESIAN_POINT('Ctrl Pts',(33.834255986992,87.8929667043318,109.379650513206));
#34688=CARTESIAN_POINT('Ctrl Pts',(33.8352709498557,87.7704133466358,109.387416697508));
#34689=CARTESIAN_POINT('Origin',(36.3549260746835,87.7685555885722,114.));
#34690=CARTESIAN_POINT('',(33.8413418417317,87.7688409760013,110.387416697508));
#34691=CARTESIAN_POINT('',(33.8387900496171,87.766431943684,110.112583302492));
#34692=CARTESIAN_POINT('',(33.8374260746835,87.7685555885722,114.));
#34693=CARTESIAN_POINT('Ctrl Pts',(33.8387900496171,87.766431943684,110.112583302492));
#34694=CARTESIAN_POINT('Ctrl Pts',(33.8435895140767,88.3553689856135,110.07539618188));
#34695=CARTESIAN_POINT('Ctrl Pts',(34.0501480074608,88.947339605864,110.038209061269));
#34696=CARTESIAN_POINT('Ctrl Pts',(34.4278435299873,89.3948822083208,110.001021940657));
#34697=CARTESIAN_POINT('Ctrl Pts',(34.9625846717064,90.0285128126893,109.948372432926));
#34698=CARTESIAN_POINT('Ctrl Pts',(35.8403679856063,90.3726391455629,109.895722925195));
#34699=CARTESIAN_POINT('Ctrl Pts',(36.6632637571565,90.2712567808753,109.843073417464));
#34700=CARTESIAN_POINT('Ctrl Pts',(37.4861595287068,90.1698744161876,109.790423909734));
#34701=CARTESIAN_POINT('Ctrl Pts',(38.2541677579075,89.6229833539386,109.737774402003));
#34702=CARTESIAN_POINT('Ctrl Pts',(38.6191235877846,88.8785083121911,109.685124894272));
#34703=CARTESIAN_POINT('Ctrl Pts',(38.9840794176617,88.1340332704436,109.632475386541));
#34704=CARTESIAN_POINT('Ctrl Pts',(38.9459828482152,87.1919742491975,109.57982587881));
#34705=CARTESIAN_POINT('Ctrl Pts',(38.5221043906172,86.4793994387067,109.527176371079));
#34706=CARTESIAN_POINT('Ctrl Pts',(38.0982259330193,85.7668246282158,109.474526863349));
#34707=CARTESIAN_POINT('Ctrl Pts',(37.2885655872697,85.2837340284801,109.421877355618));
#34708=CARTESIAN_POINT('Ctrl Pts',(36.4601705366731,85.2491292959353,109.369227847887));
#34709=CARTESIAN_POINT('Ctrl Pts',(35.6317754860765,85.2145245633906,109.316578340156));
#34710=CARTESIAN_POINT('Ctrl Pts',(34.7846457306328,85.6284056980367,109.263928832425));
#34711=CARTESIAN_POINT('Ctrl Pts',(34.3028147082516,86.3031462294792,109.211279324695));
#34712=CARTESIAN_POINT('Ctrl Pts',(34.0017368360334,86.724765913704,109.178380650627));
#34713=CARTESIAN_POINT('Ctrl Pts',(33.8432907515194,87.2482387902261,109.14548197656));
#34714=CARTESIAN_POINT('Ctrl Pts',(33.8403653828405,87.7700835309277,109.112583302492));
#34715=CARTESIAN_POINT('Ctrl Pts',(33.8352709498557,87.7704133466358,109.387416697508));
#34716=CARTESIAN_POINT('Ctrl Pts',(33.8411367527663,87.0621373417162,109.432300020937));
#34717=CARTESIAN_POINT('Ctrl Pts',(34.1540285705701,86.3493209030035,109.477183344366));
#34718=CARTESIAN_POINT('Ctrl Pts',(34.6831903458215,85.8807296858958,109.522066667795));
#34719=CARTESIAN_POINT('Ctrl Pts',(35.3039132524271,85.3310578919444,109.574716175526));
#34720=CARTESIAN_POINT('Ctrl Pts',(36.2222237448829,85.1174401434039,109.627365683257));
#34721=CARTESIAN_POINT('Ctrl Pts',(37.0218197359392,85.3367168080912,109.680015190987));
#34722=CARTESIAN_POINT('Ctrl Pts',(37.8214157269956,85.5559934727784,109.732664698718));
#34723=CARTESIAN_POINT('Ctrl Pts',(38.5022972166524,86.2081645506933,109.785314206449));
#34724=CARTESIAN_POINT('Ctrl Pts',(38.7557969307832,86.9975781962635,109.83796371418));
#34725=CARTESIAN_POINT('Ctrl Pts',(39.0092966449141,87.7869918418337,109.890613221911));
#34726=CARTESIAN_POINT('Ctrl Pts',(38.835414583519,88.7136480550593,109.943262729642));
#34727=CARTESIAN_POINT('Ctrl Pts',(38.3129775372868,89.3574613355163,109.995912237372));
#34728=CARTESIAN_POINT('Ctrl Pts',(37.7905404910545,90.0012746159734,110.048561745103));
#34729=CARTESIAN_POINT('Ctrl Pts',(36.9195484599851,90.362244963662,110.101211252834));
#34730=CARTESIAN_POINT('Ctrl Pts',(36.0948524352101,90.2767319595211,110.153860760565));
#34731=CARTESIAN_POINT('Ctrl Pts',(35.270156410435,90.1912189553803,110.206510268296));
#34732=CARTESIAN_POINT('Ctrl Pts',(34.4917563919543,89.6592225994099,110.259159776027));
#34733=CARTESIAN_POINT('Ctrl Pts',(34.1125281917178,88.921915350177,110.311809283757));
#34734=CARTESIAN_POINT('Ctrl Pts',(33.9309977610326,88.5689782468258,110.337011755008));
#34735=CARTESIAN_POINT('Ctrl Pts',(33.8409328694367,88.1689965609794,110.362214226258));
#34736=CARTESIAN_POINT('Ctrl Pts',(33.8413418417317,87.7688409760013,110.387416697508));
#34737=CARTESIAN_POINT('Origin',(36.3549260746835,87.7685555885722,114.));
#34738=CARTESIAN_POINT('',(33.8362791549462,87.7664293771055,111.387416697508));
#34739=CARTESIAN_POINT('',(33.833460355415,87.7691165130268,111.112583302492));
#34740=CARTESIAN_POINT('',(33.8374260746835,87.7685555885722,114.));
#34741=CARTESIAN_POINT('Ctrl Pts',(33.833460355415,87.7691165130268,111.112583302492));
#34742=CARTESIAN_POINT('Ctrl Pts',(33.8333656315816,87.8002064608974,111.110609402663));
#34743=CARTESIAN_POINT('Ctrl Pts',(33.8338914331638,87.8312931312554,111.108635502833));
#34744=CARTESIAN_POINT('Ctrl Pts',(33.8350477394907,87.8623563315067,111.106661603004));
#34745=CARTESIAN_POINT('Ctrl Pts',(33.8658897092781,88.6908999979653,111.054012095273));
#34746=CARTESIAN_POINT('Ctrl Pts',(34.3452981105313,89.5027460866671,111.001362587543));
#34747=CARTESIAN_POINT('Ctrl Pts',(35.0559404347995,89.9298565188012,110.948713079812));
#34748=CARTESIAN_POINT('Ctrl Pts',(35.7665827590678,90.3569669509352,110.896063572081));
#34749=CARTESIAN_POINT('Ctrl Pts',(36.7084590063511,90.3993417265016,110.84341406435));
#34750=CARTESIAN_POINT('Ctrl Pts',(37.4545839029127,90.037770885566,110.790764556619));
#34751=CARTESIAN_POINT('Ctrl Pts',(38.2007087994744,89.6762000446304,110.738115048888));
#34752=CARTESIAN_POINT('Ctrl Pts',(38.7510823453145,88.9106835871929,110.685465541158));
#34753=CARTESIAN_POINT('Ctrl Pts',(38.8562010627845,88.08825675779,110.632816033427));
#34754=CARTESIAN_POINT('Ctrl Pts',(38.9613197802546,87.2658299283872,110.580166525696));
#34755=CARTESIAN_POINT('Ctrl Pts',(38.6211836693548,86.3864927270191,110.527517017965));
#34756=CARTESIAN_POINT('Ctrl Pts',(37.9899882637174,85.8488793027858,110.474867510234));
#34757=CARTESIAN_POINT('Ctrl Pts',(37.35879285808,85.3112658785526,110.422218002503));
#34758=CARTESIAN_POINT('Ctrl Pts',(36.4365381577051,85.1153762314543,110.369568494773));
#34759=CARTESIAN_POINT('Ctrl Pts',(35.6413143061611,85.35001395255,110.316918987042));
#34760=CARTESIAN_POINT('Ctrl Pts',(34.8460904546171,85.5846516736457,110.264269479311));
#34761=CARTESIAN_POINT('Ctrl Pts',(34.1778974519041,86.2498167629355,110.21161997158));
#34762=CARTESIAN_POINT('Ctrl Pts',(33.9396504353168,87.0439667455121,110.158970463849));
#34763=CARTESIAN_POINT('Ctrl Pts',(33.8696807858515,87.2771969311392,110.14350807673));
#34764=CARTESIAN_POINT('Ctrl Pts',(33.8367944345703,87.5215522008777,110.128045689611));
#34765=CARTESIAN_POINT('Ctrl Pts',(33.8387900496171,87.766431943684,110.112583302492));
#34766=CARTESIAN_POINT('Ctrl Pts',(33.8413418417317,87.7688409760013,110.387416697508));
#34767=CARTESIAN_POINT('Ctrl Pts',(33.8417872376371,87.3330470084274,110.414863733989));
#34768=CARTESIAN_POINT('Ctrl Pts',(33.9495395712668,86.8970467869974,110.442310770469));
#34769=CARTESIAN_POINT('Ctrl Pts',(34.1633179095263,86.5213825231027,110.46975780695));
#34770=CARTESIAN_POINT('Ctrl Pts',(34.5733922095635,85.8007750877568,110.522407314681));
#34771=CARTESIAN_POINT('Ctrl Pts',(35.3735971916303,85.3021783595606,110.575056822411));
#34772=CARTESIAN_POINT('Ctrl Pts',(36.201172095805,85.2516235833065,110.627706330142));
#34773=CARTESIAN_POINT('Ctrl Pts',(37.0287469999796,85.2010688070523,110.680355837873));
#34774=CARTESIAN_POINT('Ctrl Pts',(37.8836918262622,85.5985559827401,110.733005345604));
#34775=CARTESIAN_POINT('Ctrl Pts',(38.3784303385795,86.2638903437209,110.785654853335));
#34776=CARTESIAN_POINT('Ctrl Pts',(38.8731688508967,86.9292247047016,110.838304361066));
#34777=CARTESIAN_POINT('Ctrl Pts',(39.0077010492487,87.8624062509753,110.890953868796));
#34778=CARTESIAN_POINT('Ctrl Pts',(38.7210388073494,88.6403913192867,110.943603376527));
#34779=CARTESIAN_POINT('Ctrl Pts',(38.4343765654501,89.4183763875982,110.996252884258));
#34780=CARTESIAN_POINT('Ctrl Pts',(37.7265198832995,90.0411649779474,111.048902391989));
#34781=CARTESIAN_POINT('Ctrl Pts',(36.9183648234917,90.2264253535138,111.10155189972));
#34782=CARTESIAN_POINT('Ctrl Pts',(36.1102097636839,90.4116857290801,111.15420140745));
#34783=CARTESIAN_POINT('Ctrl Pts',(35.2017563262188,90.1594178898637,111.206850915181));
#34784=CARTESIAN_POINT('Ctrl Pts',(34.6048380622974,89.5839836245909,111.259500422912));
#34785=CARTESIAN_POINT('Ctrl Pts',(34.1214175211251,89.1179621259357,111.302139181111));
#34786=CARTESIAN_POINT('Ctrl Pts',(33.8423248243317,88.4399841458963,111.344777939309));
#34787=CARTESIAN_POINT('Ctrl Pts',(33.8362791549462,87.7664293771055,111.387416697508));
#34788=CARTESIAN_POINT('Origin',(36.3549260746835,87.7685555885722,114.));
#34789=CARTESIAN_POINT('',(33.8351269672004,87.770359485814,112.387416697508));
#34790=CARTESIAN_POINT('',(33.8402624651776,87.7701463237333,112.112583302492));
#34791=CARTESIAN_POINT('',(33.8374260746835,87.7685555885722,114.));
#34792=CARTESIAN_POINT('Ctrl Pts',(33.8402624651776,87.7701463237333,112.112583302492));
#34793=CARTESIAN_POINT('Ctrl Pts',(33.8384607125217,88.0780025388695,112.093173115714));
#34794=CARTESIAN_POINT('Ctrl Pts',(33.8908469266789,88.3852669723462,112.073762928937));
#34795=CARTESIAN_POINT('Ctrl Pts',(34.0002046253728,88.6707043012003,112.054352742159));
#34796=CARTESIAN_POINT('Ctrl Pts',(34.2968338679842,89.4449438808758,112.001703234428));
#34797=CARTESIAN_POINT('Ctrl Pts',(35.0126297754489,90.0585909339135,111.949053726697));
#34798=CARTESIAN_POINT('Ctrl Pts',(35.8230971580917,90.2334579004335,111.896404218967));
#34799=CARTESIAN_POINT('Ctrl Pts',(36.6335645407346,90.4083248669535,111.843754711236));
#34800=CARTESIAN_POINT('Ctrl Pts',(37.5387033985555,90.1444117469556,111.791105203505));
#34801=CARTESIAN_POINT('Ctrl Pts',(38.1281827946389,89.561359540116,111.738455695774));
#34802=CARTESIAN_POINT('Ctrl Pts',(38.7176621907223,88.9783073332764,111.685806188043));
#34803=CARTESIAN_POINT('Ctrl Pts',(38.9914821250682,88.0761160395951,111.633156680312));
#34804=CARTESIAN_POINT('Ctrl Pts',(38.8255104943682,87.2637803626035,111.580507172582));
#34805=CARTESIAN_POINT('Ctrl Pts',(38.6595388636683,86.451444685612,111.527857664851));
#34806=CARTESIAN_POINT('Ctrl Pts',(38.0537756679227,85.7289646253103,111.47520815712));
#34807=CARTESIAN_POINT('Ctrl Pts',(37.2828344401971,85.4238655304275,111.422558649389));
#34808=CARTESIAN_POINT('Ctrl Pts',(36.5118932124715,85.1187664355448,111.369909141658));
#34809=CARTESIAN_POINT('Ctrl Pts',(35.5757739527659,85.2310483060809,111.317259633927));
#34810=CARTESIAN_POINT('Ctrl Pts',(34.8988520920738,85.7098098634567,111.264610126197));
#34811=CARTESIAN_POINT('Ctrl Pts',(34.2473089291673,86.1706220154706,111.213934518295));
#34812=CARTESIAN_POINT('Ctrl Pts',(33.8358921849187,86.9709493595603,111.163258910394));
#34813=CARTESIAN_POINT('Ctrl Pts',(33.833460355415,87.7691165130268,111.112583302492));
#34814=CARTESIAN_POINT('Ctrl Pts',(33.8362791549462,87.7664293771055,111.387416697508));
#34815=CARTESIAN_POINT('Ctrl Pts',(33.8348597495852,87.6082918428188,111.39742744704));
#34816=CARTESIAN_POINT('Ctrl Pts',(33.8484912122645,87.4503981242932,111.407438196572));
#34817=CARTESIAN_POINT('Ctrl Pts',(33.8780628754162,87.2955485091613,111.417448946105));
#34818=CARTESIAN_POINT('Ctrl Pts',(34.0335890428342,86.4811483503338,111.470098453835));
#34819=CARTESIAN_POINT('Ctrl Pts',(34.6300244680478,85.7509487240081,111.522747961566));
#34820=CARTESIAN_POINT('Ctrl Pts',(35.39698422092,85.4359745267719,111.575397469297));
#34821=CARTESIAN_POINT('Ctrl Pts',(36.1639439737922,85.1210003295356,111.628046977028));
#34822=CARTESIAN_POINT('Ctrl Pts',(37.101428054323,85.2212515613887,111.680696484759));
#34823=CARTESIAN_POINT('Ctrl Pts',(37.7844423107475,85.6912808508716,111.73334599249));
#34824=CARTESIAN_POINT('Ctrl Pts',(38.4674565671721,86.1613101403543,111.78599550022));
#34825=CARTESIAN_POINT('Ctrl Pts',(38.8960009994905,87.0011174874669,111.838645007951));
#34826=CARTESIAN_POINT('Ctrl Pts',(38.8758015061064,87.8299890021889,111.891294515682));
#34827=CARTESIAN_POINT('Ctrl Pts',(38.8556020127223,88.6588605169108,111.943944023413));
#34828=CARTESIAN_POINT('Ctrl Pts',(38.3866585936358,89.4767961992423,111.996593531144));
#34829=CARTESIAN_POINT('Ctrl Pts',(37.6815596167549,89.9129973457929,112.049243038874));
#34830=CARTESIAN_POINT('Ctrl Pts',(36.9764606398739,90.3491984923434,112.101892546605));
#34831=CARTESIAN_POINT('Ctrl Pts',(36.0352061051984,90.4036651031131,112.154542054336));
#34832=CARTESIAN_POINT('Ctrl Pts',(35.2844994425424,90.0517055683729,112.207191562067));
#34833=CARTESIAN_POINT('Ctrl Pts',(34.5337927798864,89.6997460336326,112.259841069798));
#34834=CARTESIAN_POINT('Ctrl Pts',(33.9736339892499,88.9413603533826,112.312490577529));
#34835=CARTESIAN_POINT('Ctrl Pts',(33.857962540138,88.1203511431353,112.365140085259));
#34836=CARTESIAN_POINT('Ctrl Pts',(33.8416485666483,88.0045583300114,112.372565622676));
#34837=CARTESIAN_POINT('Ctrl Pts',(33.8341761053276,87.8875198420373,112.379991160092));
#34838=CARTESIAN_POINT('Ctrl Pts',(33.8351269672004,87.770359485814,112.387416697508));
#34839=CARTESIAN_POINT('Origin',(36.3549260746835,87.7685555885722,114.));
#34840=CARTESIAN_POINT('',(33.8413206458264,87.7689269147693,113.387416697508));
#34841=CARTESIAN_POINT('',(33.8389342866079,87.7664619720545,113.112583302492));
#34842=CARTESIAN_POINT('',(33.8374260746835,87.7685555885722,114.));
#34843=CARTESIAN_POINT('Ctrl Pts',(33.8389342866079,87.7664619720545,113.112583302492));
#34844=CARTESIAN_POINT('Ctrl Pts',(33.8436023733314,88.3500889585574,113.075736828766));
#34845=CARTESIAN_POINT('Ctrl Pts',(34.0460599756738,88.9366381019817,113.03889035504));
#34846=CARTESIAN_POINT('Ctrl Pts',(34.4174406155119,89.3824748861331,113.002043881314));
#34847=CARTESIAN_POINT('Ctrl Pts',(34.9481021928884,90.019526002296,112.949394373583));
#34848=CARTESIAN_POINT('Ctrl Pts',(35.823657778157,90.36928149396,112.896744865852));
#34849=CARTESIAN_POINT('Ctrl Pts',(36.6471875611459,90.2731850276454,112.844095358121));
#34850=CARTESIAN_POINT('Ctrl Pts',(37.4707173441349,90.1770885613307,112.791445850391));
#34851=CARTESIAN_POINT('Ctrl Pts',(38.2422213248443,89.6351401370375,112.73879634266));
#34852=CARTESIAN_POINT('Ctrl Pts',(38.6119499057358,88.8930238316109,112.686146834929));
#34853=CARTESIAN_POINT('Ctrl Pts',(38.9816784866274,88.1509075261844,112.633497327198));
#34854=CARTESIAN_POINT('Ctrl Pts',(38.9496316677012,87.2086233396246,112.580847819467));
#34855=CARTESIAN_POINT('Ctrl Pts',(38.5303373869874,86.4933414787692,112.528198311736));
#34856=CARTESIAN_POINT('Ctrl Pts',(38.1110431062737,85.7780596179138,112.475548804006));
#34857=CARTESIAN_POINT('Ctrl Pts',(37.3045013637724,85.2897800827628,112.422899296275));
#34858=CARTESIAN_POINT('Ctrl Pts',(36.4763455935174,85.2498569754018,112.370249788544));
#34859=CARTESIAN_POINT('Ctrl Pts',(35.6481898232623,85.2099338680407,112.317600280813));
#34860=CARTESIAN_POINT('Ctrl Pts',(34.7984200252536,85.6183671884695,112.264950773082));
#34861=CARTESIAN_POINT('Ctrl Pts',(34.3122664151284,86.2899999018406,112.212301265351));
#34862=CARTESIAN_POINT('Ctrl Pts',(34.0053420662418,86.7140231507665,112.179061944398));
#34863=CARTESIAN_POINT('Ctrl Pts',(33.843347908687,87.2429524507666,112.145822623445));
#34864=CARTESIAN_POINT('Ctrl Pts',(33.8402624651776,87.7701463237333,112.112583302492));
#34865=CARTESIAN_POINT('Ctrl Pts',(33.8351269672004,87.770359485814,112.387416697508));
#34866=CARTESIAN_POINT('Ctrl Pts',(33.8409180294089,87.0568143004748,112.432640667823));
#34867=CARTESIAN_POINT('Ctrl Pts',(34.1591479610319,86.3387487640668,112.477864638137));
#34868=CARTESIAN_POINT('Ctrl Pts',(34.6953465327929,85.8700343879536,112.523088608452));
#34869=CARTESIAN_POINT('Ctrl Pts',(35.3195860821468,85.324359583264,112.575738116183));
#34870=CARTESIAN_POINT('Ctrl Pts',(36.2392492884418,85.1166427141294,112.628387623914));
#34871=CARTESIAN_POINT('Ctrl Pts',(37.0374208222499,85.3410490644606,112.681037131644));
#34872=CARTESIAN_POINT('Ctrl Pts',(37.8355923560581,85.5654554147918,112.733686639375));
#34873=CARTESIAN_POINT('Ctrl Pts',(38.5122722173794,86.2219849845887,112.786336147106));
#34874=CARTESIAN_POINT('Ctrl Pts',(38.7606978812279,87.0130100771061,112.838985654837));
#34875=CARTESIAN_POINT('Ctrl Pts',(39.0091235450763,87.8040351696234,112.891635162568));
#34876=CARTESIAN_POINT('Ctrl Pts',(38.8292950114517,88.7295557848613,112.944284670298));
#34877=CARTESIAN_POINT('Ctrl Pts',(38.3027348114541,89.37000122612,112.996934178029));
#34878=CARTESIAN_POINT('Ctrl Pts',(37.7761746114565,90.0104466673787,113.04958368576));
#34879=CARTESIAN_POINT('Ctrl Pts',(36.9028827450857,90.3658169346583,113.102233193491));
#34880=CARTESIAN_POINT('Ctrl Pts',(36.0787527999753,90.2750103213367,113.154882701222));
#34881=CARTESIAN_POINT('Ctrl Pts',(35.2546228548649,90.184203708015,113.207532208953));
#34882=CARTESIAN_POINT('Ctrl Pts',(34.4796548310148,89.6472202140922,113.260181716683));
#34883=CARTESIAN_POINT('Ctrl Pts',(34.105168697244,88.9074931407307,113.312831224414));
#34884=CARTESIAN_POINT('Ctrl Pts',(33.9283311751842,88.5581838049307,113.337693048779));
#34885=CARTESIAN_POINT('Ctrl Pts',(33.8407954587709,88.16366551418,113.362554873143));
#34886=CARTESIAN_POINT('Ctrl Pts',(33.8413206458264,87.7689269147693,113.387416697508));
#34887=CARTESIAN_POINT('Origin',(36.3549260746835,87.7685555885722,114.));
#34888=CARTESIAN_POINT('',(33.8364382102547,87.7664022269947,114.387416697508));
#34889=CARTESIAN_POINT('',(33.8334118350009,87.76902158344,114.112583302492));
#34890=CARTESIAN_POINT('',(33.8374260746835,87.7685555885722,114.));
#34891=CARTESIAN_POINT('Ctrl Pts',(33.8334118350009,87.76902158344,114.112583302492));
#34892=CARTESIAN_POINT('Ctrl Pts',(33.8333457474352,87.7947448381954,114.110950049548));
#34893=CARTESIAN_POINT('Ctrl Pts',(33.8337056909317,87.8204661988017,114.109316796605));
#34894=CARTESIAN_POINT('Ctrl Pts',(33.8344973919178,87.846174263081,114.107683543661));
#34895=CARTESIAN_POINT('Ctrl Pts',(33.8600186483467,88.6748988854847,114.05503403593));
#34896=CARTESIAN_POINT('Ctrl Pts',(34.3342043042376,89.4898065186503,114.002384528199));
#34897=CARTESIAN_POINT('Ctrl Pts',(35.0420895033447,89.9214711792297,113.949735020469));
#34898=CARTESIAN_POINT('Ctrl Pts',(35.7499747024518,90.3531358398091,113.897085512738));
#34899=CARTESIAN_POINT('Ctrl Pts',(36.6915594447751,90.4015575278024,113.844436005007));
#34900=CARTESIAN_POINT('Ctrl Pts',(37.4399906058851,90.0447850072972,113.791786497276));
#34901=CARTESIAN_POINT('Ctrl Pts',(38.1884217669951,89.6880124867921,113.739136989545));
#34902=CARTESIAN_POINT('Ctrl Pts',(38.7436993468918,88.9260457577886,113.686487481814));
#34903=CARTESIAN_POINT('Ctrl Pts',(38.854096698731,88.1043108497952,113.633837974084));
#34904=CARTESIAN_POINT('Ctrl Pts',(38.9644940505703,87.2825759418018,113.581188466353));
#34905=CARTESIAN_POINT('Ctrl Pts',(38.6300111743521,86.4010728548185,113.528538958622));
#34906=CARTESIAN_POINT('Ctrl Pts',(38.0022807955917,85.8594176084769,113.475889450891));
#34907=CARTESIAN_POINT('Ctrl Pts',(37.3745504168312,85.3177623621354,113.42323994316));
#34908=CARTESIAN_POINT('Ctrl Pts',(36.4535725355285,85.1159549564357,113.37059043543));
#34909=CARTESIAN_POINT('Ctrl Pts',(35.656858469034,85.3454817099042,113.317940927699));
#34910=CARTESIAN_POINT('Ctrl Pts',(34.8601444025395,85.5750084633728,113.265291419968));
#34911=CARTESIAN_POINT('Ctrl Pts',(34.1876941508532,86.2358693760097,113.212641912237));
#34912=CARTESIAN_POINT('Ctrl Pts',(33.9443528097522,87.028473202659,113.159992404506));
#34913=CARTESIAN_POINT('Ctrl Pts',(33.8713125923993,87.2663775205659,113.144189370502));
#34914=CARTESIAN_POINT('Ctrl Pts',(33.8369321972417,87.5161509875526,113.128386336497));
#34915=CARTESIAN_POINT('Ctrl Pts',(33.8389342866079,87.7664619720545,113.112583302492));
#34916=CARTESIAN_POINT('Ctrl Pts',(33.8413206458264,87.7689269147693,113.387416697508));
#34917=CARTESIAN_POINT('Ctrl Pts',(33.8419076394191,87.3277335794778,113.415204380874));
#34918=CARTESIAN_POINT('Ctrl Pts',(33.9525020156452,86.88626503035,113.44299206424));
#34919=CARTESIAN_POINT('Ctrl Pts',(34.1713711853595,86.5073359208025,113.470779747607));
#34920=CARTESIAN_POINT('Ctrl Pts',(34.5860640509373,85.7893764270359,113.523429255337));
#34921=CARTESIAN_POINT('Ctrl Pts',(35.3894540257846,85.2959280923031,113.576078763068));
#34922=CARTESIAN_POINT('Ctrl Pts',(36.2173364818051,85.2506882153788,113.628728270799));
#34923=CARTESIAN_POINT('Ctrl Pts',(37.0452189378256,85.2054483384545,113.68137777853));
#34924=CARTESIAN_POINT('Ctrl Pts',(37.8975938750193,85.6084169193387,113.734027286261));
#34925=CARTESIAN_POINT('Ctrl Pts',(38.3880500775153,86.2769142797552,113.786676793992));
#34926=CARTESIAN_POINT('Ctrl Pts',(38.8785062800113,86.9454116401717,113.839326301723));
#34927=CARTESIAN_POINT('Ctrl Pts',(39.0070437478097,87.8794377801204,113.891975809453));
#34928=CARTESIAN_POINT('Ctrl Pts',(38.7153919745293,88.6555661526162,113.944625317184));
#34929=CARTESIAN_POINT('Ctrl Pts',(38.4237402012488,89.431694525112,113.997274824915));
#34930=CARTESIAN_POINT('Ctrl Pts',(37.7118991868896,90.0499251301549,114.049924332646));
#34931=CARTESIAN_POINT('Ctrl Pts',(36.9025712304783,90.2299925242655,114.102573840377));
#34932=CARTESIAN_POINT('Ctrl Pts',(36.093243274067,90.4100599183761,114.155223348107));
#34933=CARTESIAN_POINT('Ctrl Pts',(35.1864283756038,90.1519641015545,114.207872855838));
#34934=CARTESIAN_POINT('Ctrl Pts',(34.5932172795427,89.5727088875421,114.260522363569));
#34935=CARTESIAN_POINT('Ctrl Pts',(34.1166371545854,89.1073407848392,114.302820474882));
#34936=CARTESIAN_POINT('Ctrl Pts',(33.8424682771257,88.4346847802262,114.345118586195));
#34937=CARTESIAN_POINT('Ctrl Pts',(33.8364382102547,87.7664022269947,114.387416697508));
#34938=CARTESIAN_POINT('Origin',(36.3549260746835,87.7685555885722,114.));
#34939=CARTESIAN_POINT('',(33.8349861623252,87.7703023246717,115.387416697508));
#34940=CARTESIAN_POINT('',(33.8401552434049,87.770206896396,115.112583302492));
#34941=CARTESIAN_POINT('',(33.8374260746835,87.7685555885722,114.));
#34942=CARTESIAN_POINT('Ctrl Pts',(33.8401552434049,87.770206896396,115.112583302492));
#34943=CARTESIAN_POINT('Ctrl Pts',(33.8383126786388,88.0726278356584,115.0935137626));
#34944=CARTESIAN_POINT('Ctrl Pts',(33.8888248324812,88.3744540280053,115.074444222708));
#34945=CARTESIAN_POINT('Ctrl Pts',(33.9944604721,88.6555660409125,115.055374682816));
#34946=CARTESIAN_POINT('Ctrl Pts',(34.2861122086519,89.4316943156675,115.002725175085));
#34947=CARTESIAN_POINT('Ctrl Pts',(34.9979531333667,90.0499248428541,114.950075667354));
#34948=CARTESIAN_POINT('Ctrl Pts',(35.8072809878564,90.229992214288,114.897426159623));
#34949=CARTESIAN_POINT('Ctrl Pts',(36.6166088423462,90.4100595857218,114.844776651893));
#34950=CARTESIAN_POINT('Ctrl Pts',(37.5234236266108,90.1519638014029,114.792127144162));
#34951=CARTESIAN_POINT('Ctrl Pts',(38.1166346479666,89.572708660338,114.739477636431));
#34952=CARTESIAN_POINT('Ctrl Pts',(38.7098456693223,88.993453519273,114.6868281287));
#34953=CARTESIAN_POINT('Ctrl Pts',(38.9894529277691,88.0930390214621,114.634178620969));
#34954=CARTESIAN_POINT('Ctrl Pts',(38.8287007246252,87.2796543870533,114.581529113239));
#34955=CARTESIAN_POINT('Ctrl Pts',(38.6679485214813,86.4662697526444,114.528879605508));
#34956=CARTESIAN_POINT('Ctrl Pts',(38.0668368567469,85.7399149816376,114.476230097777));
#34957=CARTESIAN_POINT('Ctrl Pts',(37.2978705626367,85.429871963928,114.423580590046));
#34958=CARTESIAN_POINT('Ctrl Pts',(36.5289042685266,85.1198289462183,114.370931082315));
#34959=CARTESIAN_POINT('Ctrl Pts',(35.5920833450407,85.2260976818057,114.318281574584));
#34960=CARTESIAN_POINT('Ctrl Pts',(34.9121013117813,85.7005028554204,114.265632066854));
#34961=CARTESIAN_POINT('Ctrl Pts',(34.2532131634472,86.1601913929319,114.214615812066));
#34962=CARTESIAN_POINT('Ctrl Pts',(33.8354761448212,86.9655305359212,114.163599557279));
#34963=CARTESIAN_POINT('Ctrl Pts',(33.8334118350009,87.76902158344,114.112583302492));
#34964=CARTESIAN_POINT('Ctrl Pts',(33.8364382102547,87.7664022269947,114.387416697508));
#34965=CARTESIAN_POINT('Ctrl Pts',(33.8349625034047,87.6028569193466,114.397768093926));
#34966=CARTESIAN_POINT('Ctrl Pts',(33.8495456897021,87.4395735386768,114.408119490344));
#34967=CARTESIAN_POINT('Ctrl Pts',(33.8811511132103,87.2796543254849,114.418470886762));
#34968=CARTESIAN_POINT('Ctrl Pts',(34.041903336598,86.4662695886435,114.471120394492));
#34969=CARTESIAN_POINT('Ctrl Pts',(34.6430150770324,85.739914726164,114.523769902223));
#34970=CARTESIAN_POINT('Ctrl Pts',(35.4119814679812,85.4298716694093,114.576419409954));
#34971=CARTESIAN_POINT('Ctrl Pts',(36.18094785893,85.1198286126545,114.629068917685));
#34972=CARTESIAN_POINT('Ctrl Pts',(37.1177689003931,85.2260973616245,114.681718425416));
#34973=CARTESIAN_POINT('Ctrl Pts',(37.7977510192853,85.7005025949826,114.734367933146));
#34974=CARTESIAN_POINT('Ctrl Pts',(38.4777331381775,86.1749078283407,114.787017440877));
#34975=CARTESIAN_POINT('Ctrl Pts',(38.9008763344987,87.0174495460869,114.839666948608));
#34976=CARTESIAN_POINT('Ctrl Pts',(38.875355074856,87.846174272855,114.892316456339));
#34977=CARTESIAN_POINT('Ctrl Pts',(38.8498338152134,88.6748989996231,114.94496596407));
#34978=CARTESIAN_POINT('Ctrl Pts',(38.3756480996068,89.4898067354131,114.997615471801));
#34979=CARTESIAN_POINT('Ctrl Pts',(37.6677628113533,89.9214714503538,115.050264979531));
#34980=CARTESIAN_POINT('Ctrl Pts',(36.9598775230998,90.3531361652945,115.102914487262));
#34981=CARTESIAN_POINT('Ctrl Pts',(36.0182926621993,90.4015578593859,115.155563994993));
#34982=CARTESIAN_POINT('Ctrl Pts',(35.2698614068365,90.0447852939514,115.208213502724));
#34983=CARTESIAN_POINT('Ctrl Pts',(34.5214301514738,89.6880127285168,115.260863010455));
#34984=CARTESIAN_POINT('Ctrl Pts',(33.9661525016488,88.9260459035562,115.313512518185));
#34985=CARTESIAN_POINT('Ctrl Pts',(33.8557551359065,88.1043108920788,115.366162025916));
#34986=CARTESIAN_POINT('Ctrl Pts',(33.8408992847342,87.9937324108665,115.373246916447));
#34987=CARTESIAN_POINT('Ctrl Pts',(33.8340994588008,87.8820716294572,115.380331806977));
#34988=CARTESIAN_POINT('Ctrl Pts',(33.8349861623252,87.7703023246717,115.387416697508));
#34989=CARTESIAN_POINT('Origin',(36.3549260746835,87.7685555885722,114.));
#34990=CARTESIAN_POINT('',(33.8412939066634,87.7690123128212,116.387416697508));
#34991=CARTESIAN_POINT('',(33.8390758148819,87.7664952480788,116.112583302492));
#34992=CARTESIAN_POINT('',(33.8374260746835,87.7685555885722,114.));
#34993=CARTESIAN_POINT('Ctrl Pts',(33.8390758148819,87.7664952480788,116.112583302492));
#34994=CARTESIAN_POINT('Ctrl Pts',(33.8436083734887,88.3448089772224,116.076077475652));
#34995=CARTESIAN_POINT('Ctrl Pts',(34.0420142063692,88.925932533728,116.039571648811));
#34996=CARTESIAN_POINT('Ctrl Pts',(34.407117583208,89.3700010244447,116.003065821971));
#34997=CARTESIAN_POINT('Ctrl Pts',(34.9336777168943,90.0104463850497,115.95041631424));
#34998=CARTESIAN_POINT('Ctrl Pts',(35.8069694732883,90.3658166075759,115.897766806509));
#34999=CARTESIAN_POINT('Ctrl Pts',(36.631099314613,90.2750100056896,115.845117298778));
#35000=CARTESIAN_POINT('Ctrl Pts',(37.4552291559377,90.1842034038034,115.792467791047));
#35001=CARTESIAN_POINT('Ctrl Pts',(38.2301970821931,89.6472199775046,115.739818283317));
#35002=CARTESIAN_POINT('Ctrl Pts',(38.6046831688033,88.9074929972995,115.687168775586));
#35003=CARTESIAN_POINT('Ctrl Pts',(38.9791692554135,88.1677660170944,115.634519267855));
#35004=CARTESIAN_POINT('Ctrl Pts',(38.9531735023785,87.225295482983,115.581869760124));
#35005=CARTESIAN_POINT('Ctrl Pts',(38.5384806890242,86.5073360796318,115.529220252393));
#35006=CARTESIAN_POINT('Ctrl Pts',(38.1237878756699,85.7893766762806,115.476570744662));
#35007=CARTESIAN_POINT('Ctrl Pts',(37.3203980019963,85.2959284036898,115.423921236932));
#35008=CARTESIAN_POINT('Ctrl Pts',(36.492515650234,85.2506885324629,115.371271729201));
#35009=CARTESIAN_POINT('Ctrl Pts',(35.6646332984718,85.2054486612361,115.31862222147));
#35010=CARTESIAN_POINT('Ctrl Pts',(34.8122584686209,85.6084171913732,115.265972713739));
#35011=CARTESIAN_POINT('Ctrl Pts',(34.32180232789,86.2769144676035,115.213323206008));
#35012=CARTESIAN_POINT('Ctrl Pts',(34.0089883597845,86.703283450024,115.17974323817));
#35013=CARTESIAN_POINT('Ctrl Pts',(33.8433998558045,87.2376672823468,115.146163270331));
#35014=CARTESIAN_POINT('Ctrl Pts',(33.8401552434049,87.770206896396,115.112583302492));
#35015=CARTESIAN_POINT('Ctrl Pts',(33.8349861623252,87.7703023246717,115.387416697508));
#35016=CARTESIAN_POINT('Ctrl Pts',(33.8406887637253,87.051487324592,115.432981314708));
#35017=CARTESIAN_POINT('Ctrl Pts',(34.1643125433803,86.3281837084398,115.478545931909));
#35018=CARTESIAN_POINT('Ctrl Pts',(34.7075711463174,85.8594173680528,115.524110549109));
#35019=CARTESIAN_POINT('Ctrl Pts',(35.3353016041301,85.3177620534985,115.57676005684));
#35020=CARTESIAN_POINT('Ctrl Pts',(36.2562796014149,85.115954622384,115.62940956457));
#35021=CARTESIAN_POINT('Ctrl Pts',(37.0529937682425,85.3454814047575,115.682059072301));
#35022=CARTESIAN_POINT('Ctrl Pts',(37.8497079350702,85.5750081871309,115.734708580032));
#35023=CARTESIAN_POINT('Ctrl Pts',(38.5221582714408,86.2358691829923,115.787358087763));
#35024=CARTESIAN_POINT('Ctrl Pts',(38.7654996431869,87.028473109457,115.840007595494));
#35025=CARTESIAN_POINT('Ctrl Pts',(39.008841014933,87.8210770359218,115.892657103225));
#35026=CARTESIAN_POINT('Ctrl Pts',(38.8230734220546,88.74542389299,115.945306610955));
#35027=CARTESIAN_POINT('Ctrl Pts',(38.2924117778502,89.3824750893792,115.997956118686));
#35028=CARTESIAN_POINT('Ctrl Pts',(37.7617501336458,90.0195262857684,116.050605626417));
#35029=CARTESIAN_POINT('Ctrl Pts',(36.8861944381154,90.3692818214786,116.103255134148));
#35030=CARTESIAN_POINT('Ctrl Pts',(36.0626645514163,90.2731853430625,116.155904641879));
#35031=CARTESIAN_POINT('Ctrl Pts',(35.2391346647172,90.1770888646463,116.20855414961));
#35032=CARTESIAN_POINT('Ctrl Pts',(34.4676305868494,89.6351403721039,116.26120365734));
#35033=CARTESIAN_POINT('Ctrl Pts',(34.0979019593964,88.8930239732201,116.313853165071));
#35034=CARTESIAN_POINT('Ctrl Pts',(33.9257031738126,88.5473879224497,116.33837434255));
#35035=CARTESIAN_POINT('Ctrl Pts',(33.8406563983059,88.1583320077416,116.362895520029));
#35036=CARTESIAN_POINT('Ctrl Pts',(33.8412939066634,87.7690123128212,116.387416697508));
#35037=CARTESIAN_POINT('Origin',(36.3549260746835,87.7685555885722,114.));
#35038=CARTESIAN_POINT('',(33.8365981008565,87.7663787380631,117.387416697508));
#35039=CARTESIAN_POINT('',(33.8333717767661,87.768925609881,117.112583302492));
#35040=CARTESIAN_POINT('',(33.8374260746835,87.7685555885722,114.));
#35041=CARTESIAN_POINT('Ctrl Pts',(33.8333717767661,87.768925609881,117.112583302492));
#35042=CARTESIAN_POINT('Ctrl Pts',(33.8333296036217,87.7892829070983,117.111290696434));
#35043=CARTESIAN_POINT('Ctrl Pts',(33.8335550399572,87.8096392466113,117.109998090376));
#35044=CARTESIAN_POINT('Ctrl Pts',(33.8340509607236,87.829988994453,117.108705484318));
#35045=CARTESIAN_POINT('Ctrl Pts',(33.8542504515642,88.6588604047923,117.056055976587));
#35046=CARTESIAN_POINT('Ctrl Pts',(34.3231938115952,89.4767959841181,117.003406468856));
#35047=CARTESIAN_POINT('Ctrl Pts',(35.0282926996806,89.912997075736,116.950756961126));
#35048=CARTESIAN_POINT('Ctrl Pts',(35.733391587766,90.349198167354,116.898107453395));
#35049=CARTESIAN_POINT('Ctrl Pts',(36.6746460039059,90.4036647712641,116.845457945664));
#35050=CARTESIAN_POINT('Ctrl Pts',(37.4253525720226,90.0517052808472,116.792808437933));
#35051=CARTESIAN_POINT('Ctrl Pts',(38.1760591401393,89.6997457904303,116.740158930202));
#35052=CARTESIAN_POINT('Ctrl Pts',(38.7362178602328,88.9413602056864,116.687509422471));
#35053=CARTESIAN_POINT('Ctrl Pts',(38.8518892947775,88.1203510988316,116.634859914741));
#35054=CARTESIAN_POINT('Ctrl Pts',(38.9675607293222,87.2993419919769,116.58221040701));
#35055=CARTESIAN_POINT('Ctrl Pts',(38.638744878318,86.4157093630114,116.529560899279));
#35056=CARTESIAN_POINT('Ctrl Pts',(38.0145054075767,85.8700346270407,116.476911391548));
#35057=CARTESIAN_POINT('Ctrl Pts',(37.3902659368354,85.3243598910701,116.424261883817));
#35058=CARTESIAN_POINT('Ctrl Pts',(36.4706028463569,85.1166430480943,116.371612376086));
#35059=CARTESIAN_POINT('Ctrl Pts',(35.6724314130655,85.3410493701655,116.318962868356));
#35060=CARTESIAN_POINT('Ctrl Pts',(34.874259979774,85.5654556922366,116.266313360625));
#35061=CARTESIAN_POINT('Ctrl Pts',(34.1975802036695,86.2219851793546,116.213663852894));
#35062=CARTESIAN_POINT('Ctrl Pts',(33.9491545711065,87.0130101722554,116.161014345163));
#35063=CARTESIAN_POINT('Ctrl Pts',(33.8729809408117,87.255558595063,116.144870664273));
#35064=CARTESIAN_POINT('Ctrl Pts',(33.8370714176089,87.5107521761952,116.128726983382));
#35065=CARTESIAN_POINT('Ctrl Pts',(33.8390758148819,87.7664952480788,116.112583302492));
#35066=CARTESIAN_POINT('Ctrl Pts',(33.8412939066634,87.7690123128212,116.387416697508));
#35067=CARTESIAN_POINT('Ctrl Pts',(33.8420251947768,87.3224223005078,116.41554502776));
#35068=CARTESIAN_POINT('Ctrl Pts',(33.9555038567139,86.8754851938983,116.443673358012));
#35069=CARTESIAN_POINT('Ctrl Pts',(34.1795144884218,86.4933413181774,116.471801688264));
#35070=CARTESIAN_POINT('Ctrl Pts',(34.5988088219386,85.7780593672439,116.524451195994));
#35071=CARTESIAN_POINT('Ctrl Pts',(35.4053506660105,85.2897797706019,116.577100703725));
#35072=CARTESIAN_POINT('Ctrl Pts',(36.2335065405582,85.2498566582129,116.629750211456));
#35073=CARTESIAN_POINT('Ctrl Pts',(37.0616624151058,85.2099335458239,116.682399719187));
#35074=CARTESIAN_POINT('Ctrl Pts',(37.9114323201292,85.618366917688,116.735049226918));
#35075=CARTESIAN_POINT('Ctrl Pts',(38.3975859914778,86.2899997156401,116.787698734649));
#35076=CARTESIAN_POINT('Ctrl Pts',(38.8837396628263,86.9616325135921,116.840348242379));
#35077=CARTESIAN_POINT('Ctrl Pts',(39.0062771005,87.8964647376321,116.89299775011));
#35078=CARTESIAN_POINT('Ctrl Pts',(38.7096478205332,88.6707044148104,116.945647257841));
#35079=CARTESIAN_POINT('Ctrl Pts',(38.4130185405664,89.4449440919888,116.998296765572));
#35080=CARTESIAN_POINT('Ctrl Pts',(37.6972225429591,90.0585912223056,117.050946273303));
#35081=CARTESIAN_POINT('Ctrl Pts',(36.8867550582512,90.2334582108475,117.103595781034));
#35082=CARTESIAN_POINT('Ctrl Pts',(36.0762875735433,90.4083251993893,117.156245288764));
#35083=CARTESIAN_POINT('Ctrl Pts',(35.1711486017349,90.1444120461562,117.208894796495));
#35084=CARTESIAN_POINT('Ctrl Pts',(34.581669131416,89.5613597658909,117.261544304226));
#35085=CARTESIAN_POINT('Ctrl Pts',(34.1119009422619,89.0967135353203,117.303501768653));
#35086=CARTESIAN_POINT('Ctrl Pts',(33.8426024374579,88.4293877726653,117.345459233081));
#35087=CARTESIAN_POINT('Ctrl Pts',(33.8365981008565,87.7663787380631,117.387416697508));
#35088=CARTESIAN_POINT('Origin',(36.3549260746835,87.7685555885722,114.));
#35089=CARTESIAN_POINT('',(33.83484883244,87.7702419443436,118.387416697508));
#35090=CARTESIAN_POINT('',(33.8400438151642,87.770264994436,118.112583302492));
#35091=CARTESIAN_POINT('',(33.8374260746835,87.7685555885722,114.));
#35092=CARTESIAN_POINT('Ctrl Pts',(33.8400438151642,87.770264994436,118.112583302492));
#35093=CARTESIAN_POINT('Ctrl Pts',(33.8381651041214,88.0672505512461,118.093854409486));
#35094=CARTESIAN_POINT('Ctrl Pts',(33.8868399271723,88.3636403356866,118.075125516479));
#35095=CARTESIAN_POINT('Ctrl Pts',(33.9888136399911,88.640391209494,118.056396623473));
#35096=CARTESIAN_POINT('Ctrl Pts',(34.2754758457902,89.4183761798309,118.003747115742));
#35097=CARTESIAN_POINT('Ctrl Pts',(34.983332438798,90.0411646917499,117.951097608011));
#35098=CARTESIAN_POINT('Ctrl Pts',(35.791487396832,90.2264250439855,117.89844810028));
#35099=CARTESIAN_POINT('Ctrl Pts',(36.5996423548659,90.4116853962211,117.845798592549));
#35100=CARTESIAN_POINT('Ctrl Pts',(37.5080956779261,90.1594175887735,117.793149084819));
#35101=CARTESIAN_POINT('Ctrl Pts',(38.1050138666753,89.583983395967,117.740499577088));
#35102=CARTESIAN_POINT('Ctrl Pts',(38.7019320554245,89.0085492031604,117.687850069357));
#35103=CARTESIAN_POINT('Ctrl Pts',(38.9873151098626,88.109948624995,117.635200561626));
#35104=CARTESIAN_POINT('Ctrl Pts',(38.8317889620303,87.295548568728,117.582551053895));
#35105=CARTESIAN_POINT('Ctrl Pts',(38.6762628141981,86.4811485124609,117.529901546165));
#35106=CARTESIAN_POINT('Ctrl Pts',(38.0798274640955,85.7509489780921,117.477252038434));
#35107=CARTESIAN_POINT('Ctrl Pts',(37.3128678078092,85.4359748205219,117.424602530703));
#35108=CARTESIAN_POINT('Ctrl Pts',(36.545908151523,85.1210006629517,117.371953022972));
#35109=CARTESIAN_POINT('Ctrl Pts',(35.608424189053,85.2212518821802,117.319303515241));
#35110=CARTESIAN_POINT('Ctrl Pts',(34.925410018643,85.6912811124707,117.26665400751));
#35111=CARTESIAN_POINT('Ctrl Pts',(34.259164632832,86.1497705837644,117.215297105838));
#35112=CARTESIAN_POINT('Ctrl Pts',(33.8350473700513,86.96010400098,117.163940204165));
#35113=CARTESIAN_POINT('Ctrl Pts',(33.8333717767661,87.768925609881,117.112583302492));
#35114=CARTESIAN_POINT('Ctrl Pts',(33.8365981008565,87.7663787380631,117.387416697508));
#35115=CARTESIAN_POINT('Ctrl Pts',(33.83506801252,87.5974237879654,117.398108740811));
#35116=CARTESIAN_POINT('Ctrl Pts',(33.8506358798951,87.428749160161,117.408800784115));
#35117=CARTESIAN_POINT('Ctrl Pts',(33.884341343869,87.2637802990361,117.419492827418));
#35118=CARTESIAN_POINT('Ctrl Pts',(34.0503129954701,86.4514445197442,117.472142335149));
#35119=CARTESIAN_POINT('Ctrl Pts',(34.6560762675015,85.7289643684577,117.52479184288));
#35120=CARTESIAN_POINT('Ctrl Pts',(35.4270175923144,85.4238652351525,117.577441350611));
#35121=CARTESIAN_POINT('Ctrl Pts',(36.1979589171274,85.1187661018472,117.630090858342));
#35122=CARTESIAN_POINT('Ctrl Pts',(37.1340782947219,85.2310479865231,117.682740366073));
#35123=CARTESIAN_POINT('Ctrl Pts',(37.8110002406613,85.709809604191,117.735389873803));
#35124=CARTESIAN_POINT('Ctrl Pts',(38.4879221866007,86.1885712218588,117.788039381534));
#35125=CARTESIAN_POINT('Ctrl Pts',(38.905646700885,87.0338125725185,117.840688889265));
#35126=CARTESIAN_POINT('Ctrl Pts',(38.8748047272138,87.8623563433186,117.893338396996));
#35127=CARTESIAN_POINT('Ctrl Pts',(38.8439627535427,88.6909001141187,117.945987904727));
#35128=CARTESIAN_POINT('Ctrl Pts',(38.3645542919161,89.5027463050592,117.998637412458));
#35129=CARTESIAN_POINT('Ctrl Pts',(37.6539118781542,89.9298567909811,118.051286920188));
#35130=CARTESIAN_POINT('Ctrl Pts',(36.9432694643923,90.3569672769031,118.103936427919));
#35131=CARTESIAN_POINT('Ctrl Pts',(36.0013930984951,90.3993420578065,118.15658593565));
#35132=CARTESIAN_POINT('Ctrl Pts',(35.2552681079711,90.0377711713371,118.209235443381));
#35133=CARTESIAN_POINT('Ctrl Pts',(34.5091431174471,89.6762002848676,118.261884951112));
#35134=CARTESIAN_POINT('Ctrl Pts',(33.9587695022963,88.9106837310251,118.314534458842));
#35135=CARTESIAN_POINT('Ctrl Pts',(33.853650771588,88.0882567980515,118.367183966573));
#35136=CARTESIAN_POINT('Ctrl Pts',(33.840185378233,87.9829063806367,118.373928210218));
#35137=CARTESIAN_POINT('Ctrl Pts',(33.8340261009119,87.8766221299322,118.380672453863));
#35138=CARTESIAN_POINT('Ctrl Pts',(33.83484883244,87.7702419443436,118.387416697508));
#35139=CARTESIAN_POINT('Origin',(36.3549260746835,87.7685555885722,114.));
#35140=CARTESIAN_POINT('',(33.8412616562718,87.7690970336947,119.387416697508));
#35141=CARTESIAN_POINT('',(33.8392144539235,87.7665317069332,119.112583302492));
#35142=CARTESIAN_POINT('',(33.8374260746835,87.7685555885722,114.));
#35143=CARTESIAN_POINT('Ctrl Pts',(33.8392144539235,87.7665317069332,119.112583302492));
#35144=CARTESIAN_POINT('Ctrl Pts',(33.8436076679264,88.3395289215697,119.076418122537));
#35145=CARTESIAN_POINT('Ctrl Pts',(34.0380105838227,88.9152229984202,119.040252942582));
#35146=CARTESIAN_POINT('Ctrl Pts',(34.3968748586662,89.3574611354189,119.004087762628));
#35147=CARTESIAN_POINT('Ctrl Pts',(34.9193118391072,90.0012743347968,118.951438254897));
#35148=CARTESIAN_POINT('Ctrl Pts',(35.7903037604876,90.3622446370295,118.898788747166));
#35149=CARTESIAN_POINT('Ctrl Pts',(36.6149996814052,90.276731643658,118.846139239435));
#35150=CARTESIAN_POINT('Ctrl Pts',(37.4396956023229,90.1912186502865,118.793489731704));
#35151=CARTESIAN_POINT('Ctrl Pts',(38.2180955227777,89.6592223613109,118.740840223974));
#35152=CARTESIAN_POINT('Ctrl Pts',(38.5973236752566,88.9219152049292,118.688190716243));
#35153=CARTESIAN_POINT('Ctrl Pts',(38.9765518277355,88.1846080485476,118.635541208512));
#35154=CARTESIAN_POINT('Ctrl Pts',(38.9566082122386,87.24199002476,118.582891700781));
#35155=CARTESIAN_POINT('Ctrl Pts',(38.5465339638431,86.5213826801631,118.53024219305));
#35156=CARTESIAN_POINT('Ctrl Pts',(38.1364597154477,85.8007753355662,118.477592685319));
#35157=CARTESIAN_POINT('Ctrl Pts',(37.3362548341537,85.3021786701601,118.424943177589));
#35158=CARTESIAN_POINT('Ctrl Pts',(36.5086800341986,85.2516239002727,118.372293669858));
#35159=CARTESIAN_POINT('Ctrl Pts',(35.6811052342435,85.2010691303852,118.319644162127));
#35160=CARTESIAN_POINT('Ctrl Pts',(34.8261605156272,85.5985562560164,118.266994654396));
#35161=CARTESIAN_POINT('Ctrl Pts',(34.3314220656143,86.2638905332094,118.214345146665));
#35162=CARTESIAN_POINT('Ctrl Pts',(34.0126758308339,86.6925469186593,118.180424531941));
#35163=CARTESIAN_POINT('Ctrl Pts',(33.8434464206167,87.2323830893058,118.146503917216));
#35164=CARTESIAN_POINT('Ctrl Pts',(33.8400438151642,87.770264994436,118.112583302492));
#35165=CARTESIAN_POINT('Ctrl Pts',(33.83484883244,87.7702419443436,118.387416697508));
#35166=CARTESIAN_POINT('Ctrl Pts',(33.8404488240859,87.046156224721,118.433321961594));
#35167=CARTESIAN_POINT('Ctrl Pts',(34.1695224385136,86.3176258810383,118.47922722568));
#35168=CARTESIAN_POINT('Ctrl Pts',(34.7198636797397,85.8488790610354,118.525132489766));
#35169=CARTESIAN_POINT('Ctrl Pts',(35.3510591648657,85.3112655690975,118.577781997496));
#35170=CARTESIAN_POINT('Ctrl Pts',(36.2733139813835,85.1153758973266,118.630431505227));
#35171=CARTESIAN_POINT('Ctrl Pts',(37.068537933073,85.3500136479724,118.683081012958));
#35172=CARTESIAN_POINT('Ctrl Pts',(37.8637618847625,85.5846513986182,118.735730520689));
#35173=CARTESIAN_POINT('Ctrl Pts',(38.5319549716236,86.2498165716809,118.78838002842));
#35174=CARTESIAN_POINT('Ctrl Pts',(38.7702020182144,87.0439666542645,118.841029536151));
#35175=CARTESIAN_POINT('Ctrl Pts',(39.0084490648051,87.8381167368482,118.893679043881));
#35176=CARTESIAN_POINT('Ctrl Pts',(38.8167500711256,88.7612517289529,118.946328551612));
#35177=CARTESIAN_POINT('Ctrl Pts',(38.2820088620648,89.394882413123,118.998978059343));
#35178=CARTESIAN_POINT('Ctrl Pts',(37.7472676530041,90.0285130972932,119.051627567074));
#35179=CARTESIAN_POINT('Ctrl Pts',(36.8694842285622,90.3726394735288,119.104277074805));
#35180=CARTESIAN_POINT('Ctrl Pts',(36.0465883533813,90.2712570960621,119.156926582536));
#35181=CARTESIAN_POINT('Ctrl Pts',(35.2236924782003,90.1698747185954,119.209576090266));
#35182=CARTESIAN_POINT('Ctrl Pts',(34.4556841522802,89.6229835874264,119.262225597997));
#35183=CARTESIAN_POINT('Ctrl Pts',(34.0907282764438,88.8785084519475,119.314875105728));
#35184=CARTESIAN_POINT('Ctrl Pts',(33.9231136661421,88.5365906531818,119.339055636321));
#35185=CARTESIAN_POINT('Ctrl Pts',(33.840515823365,88.1529960122149,119.363236166915));
#35186=CARTESIAN_POINT('Ctrl Pts',(33.8412616562718,87.7690970336947,119.387416697508));
#35187=CARTESIAN_POINT('Origin',(36.3549260746835,87.7685555885722,114.));
#35188=CARTESIAN_POINT('',(33.836758858704,87.7663573595953,120.387416697508));
#35189=CARTESIAN_POINT('',(33.833340462721,87.7688288397412,120.112583302492));
#35190=CARTESIAN_POINT('',(33.8374260746835,87.7685555885722,114.));
#35191=CARTESIAN_POINT('Ctrl Pts',(33.833340462721,87.7688288397412,120.112583302492));
#35192=CARTESIAN_POINT('Ctrl Pts',(33.8333171635958,87.7838207780303,120.11163134332));
#35193=CARTESIAN_POINT('Ctrl Pts',(33.833439427189,87.7988123261839,120.110679384147));
#35194=CARTESIAN_POINT('Ctrl Pts',(33.8337084163132,87.8138012411625,120.109727424975));
#35195=CARTESIAN_POINT('Ctrl Pts',(33.8485852570257,88.6427853173127,120.057077917244));
#35196=CARTESIAN_POINT('Ctrl Pts',(34.3122670847453,89.4637150212562,120.004428409513));
#35197=CARTESIAN_POINT('Ctrl Pts',(35.014550615983,89.9044345342344,119.951778901782));
#35198=CARTESIAN_POINT('Ctrl Pts',(35.7168341472208,90.3451540472126,119.899129394052));
#35199=CARTESIAN_POINT('Ctrl Pts',(36.6577193819767,90.4056633692255,119.846479886321));
#35200=CARTESIAN_POINT('Ctrl Pts',(37.4106703935041,90.0585314323461,119.79383037859));
#35201=CARTESIAN_POINT('Ctrl Pts',(38.1636214050315,89.7113994954668,119.741180870859));
#35202=CARTESIAN_POINT('Ctrl Pts',(38.7286381933304,88.9566262996952,119.688531363128));
#35203=CARTESIAN_POINT('Ctrl Pts',(38.8495789474356,88.13637683792,119.635881855397));
#35204=CARTESIAN_POINT('Ctrl Pts',(38.9705197015409,87.3161273761447,119.583232347667));
#35205=CARTESIAN_POINT('Ctrl Pts',(38.6473844214524,86.4304016483656,119.530582839936));
#35206=CARTESIAN_POINT('Ctrl Pts',(38.0266615930102,85.8807299236465,119.477933332205));
#35207=CARTESIAN_POINT('Ctrl Pts',(37.4059387645679,85.3310581989274,119.425283824474));
#35208=CARTESIAN_POINT('Ctrl Pts',(36.487628387772,85.1174404772682,119.372634316743));
#35209=CARTESIAN_POINT('Ctrl Pts',(35.6880324974151,85.3367171143363,119.319984809013));
#35210=CARTESIAN_POINT('Ctrl Pts',(34.8884366070581,85.5559937514044,119.267335301282));
#35211=CARTESIAN_POINT('Ctrl Pts',(34.2075552031403,86.2081647471997,119.214685793551));
#35212=CARTESIAN_POINT('Ctrl Pts',(33.9540555209321,86.9975782933589,119.16203628582));
#35213=CARTESIAN_POINT('Ctrl Pts',(33.8746858927486,87.2447401797007,119.145551958044));
#35214=CARTESIAN_POINT('Ctrl Pts',(33.8372119979782,87.5053557937311,119.129067630268));
#35215=CARTESIAN_POINT('Ctrl Pts',(33.8392144539235,87.7665317069332,119.112583302492));
#35216=CARTESIAN_POINT('Ctrl Pts',(33.8412616562718,87.7690970336947,119.387416697508));
#35217=CARTESIAN_POINT('Ctrl Pts',(33.8421397635529,87.3171131038791,119.415885674646));
#35218=CARTESIAN_POINT('Ctrl Pts',(33.958545197753,86.8647073147717,119.444354651783));
#35219=CARTESIAN_POINT('Ctrl Pts',(34.1877474858301,86.4793992764073,119.472823628921));
#35220=CARTESIAN_POINT('Ctrl Pts',(34.6116259968056,85.7668243761348,119.525473136651));
#35221=CARTESIAN_POINT('Ctrl Pts',(35.4212864445094,85.2837337153784,119.578122644382));
#35222=CARTESIAN_POINT('Ctrl Pts',(36.2496815994356,85.2491289785611,119.630772152113));
#35223=CARTESIAN_POINT('Ctrl Pts',(37.0780767543618,85.2145242417438,119.683421659844));
#35224=CARTESIAN_POINT('Ctrl Pts',(37.9252066165105,85.6284054288655,119.736071167575));
#35225=CARTESIAN_POINT('Ctrl Pts',(38.4070376995544,86.3031460451161,119.788720675305));
#35226=CARTESIAN_POINT('Ctrl Pts',(38.8888687825984,86.9778866613667,119.841370183036));
#35227=CARTESIAN_POINT('Ctrl Pts',(39.0054010865376,87.9134867067461,119.894019690767));
#35228=CARTESIAN_POINT('Ctrl Pts',(38.703806556982,88.6858056190045,119.946669198498));
#35229=CARTESIAN_POINT('Ctrl Pts',(38.4022120274264,89.458124531263,119.999318706229));
#35230=CARTESIAN_POINT('Ctrl Pts',(37.6824906643758,90.0671623104004,120.05196821396));
#35231=CARTESIAN_POINT('Ctrl Pts',(36.8709170107602,90.2368219880218,120.10461772169));
#35232=CARTESIAN_POINT('Ctrl Pts',(36.0593433571446,90.4064816656432,120.157267229421));
#35233=CARTESIAN_POINT('Ctrl Pts',(35.1559174129639,90.1367632417485,120.209916737152));
#35234=CARTESIAN_POINT('Ctrl Pts',(34.570193987387,89.5499373082837,120.262566244883));
#35235=CARTESIAN_POINT('Ctrl Pts',(34.1072087481559,89.0860805913963,120.304183062425));
#35236=CARTESIAN_POINT('Ctrl Pts',(33.8427277366527,88.4240914153437,120.345799879966));
#35237=CARTESIAN_POINT('Ctrl Pts',(33.836758858704,87.7663573595953,120.387416697508));
#35238=CARTESIAN_POINT('Origin',(36.3549260746835,87.7685555885722,114.));
#35239=CARTESIAN_POINT('',(33.8347232656258,87.7701345030551,121.387416697508));
#35240=CARTESIAN_POINT('',(33.8399314485466,87.7703173734778,121.112583302492));
#35241=CARTESIAN_POINT('',(33.8374260746835,87.7685555885722,114.));
#35242=CARTESIAN_POINT('',(38.2683920713486,89.4045427919472,122.));
#35243=CARTESIAN_POINT('Ctrl Pts',(33.8347232656258,87.7701345030551,121.387416697508));
#35244=CARTESIAN_POINT('Ctrl Pts',(33.8401812849309,87.0409115185374,121.43366260848));
#35245=CARTESIAN_POINT('Ctrl Pts',(34.1747109746967,86.3074372742024,121.479908519451));
#35246=CARTESIAN_POINT('Ctrl Pts',(34.732188100241,85.8386039826766,121.526154430423));
#35247=CARTESIAN_POINT('Ctrl Pts',(35.366858184893,85.3048521008755,121.578803938153));
#35248=CARTESIAN_POINT('Ctrl Pts',(36.2904927310035,85.1141040762004,121.631453445884));
#35249=CARTESIAN_POINT('Ctrl Pts',(37.0841095554981,85.3542578208156,121.684102953615));
#35250=CARTESIAN_POINT('Ctrl Pts',(37.8777263799928,85.5944115654307,121.736752461346));
#35251=CARTESIAN_POINT('Ctrl Pts',(38.5413254828716,86.265467079336,121.789401969077));
#35252=CARTESIAN_POINT('Ctrl Pts',(38.774290752291,87.0597530844097,121.842051476808));
#35253=CARTESIAN_POINT('Ctrl Pts',(39.0072560217103,87.8540390894835,121.894700984538));
#35254=CARTESIAN_POINT('Ctrl Pts',(38.8095874576702,88.7715555857257,121.947350492269));
#35255=CARTESIAN_POINT('Ctrl Pts',(38.2683920713486,89.4045427919472,122.));
#35256=CARTESIAN_POINT('',(34.4378159219561,89.4070834740737,122.));
#35257=CARTESIAN_POINT('Origin',(36.3549260746835,87.7685555885722,122.));
#35258=CARTESIAN_POINT('Ctrl Pts',(34.437807076635,89.4070896409746,122.));
#35259=CARTESIAN_POINT('Ctrl Pts',(34.9606276647882,90.0158048705303,121.949053726697));
#35260=CARTESIAN_POINT('Ctrl Pts',(35.8003520975665,90.3559809225441,121.898107453395));
#35261=CARTESIAN_POINT('Ctrl Pts',(36.5990228929266,90.2782180814728,121.847161180092));
#35262=CARTESIAN_POINT('Ctrl Pts',(37.4243948286695,90.1978554752066,121.794511672361));
#35263=CARTESIAN_POINT('Ctrl Pts',(38.2059222332878,89.6711418033962,121.74186216463));
#35264=CARTESIAN_POINT('Ctrl Pts',(38.5898068286109,88.9363551220242,121.6892126569));
#35265=CARTESIAN_POINT('Ctrl Pts',(38.973691423934,88.2015684406522,121.636563149169));
#35266=CARTESIAN_POINT('Ctrl Pts',(38.9599332099619,87.2587087497187,121.583913641438));
#35267=CARTESIAN_POINT('Ctrl Pts',(38.5545284529765,86.5354489971012,121.531264133707));
#35268=CARTESIAN_POINT('Ctrl Pts',(38.1491236959911,85.8121892444836,121.478614625976));
#35269=CARTESIAN_POINT('Ctrl Pts',(37.3520723959923,85.3085294301821,121.425965118245));
#35270=CARTESIAN_POINT('Ctrl Pts',(36.5248227256852,85.2526784615377,121.373315610515));
#35271=CARTESIAN_POINT('Ctrl Pts',(35.6975730553781,85.1968274928934,121.320666102784));
#35272=CARTESIAN_POINT('Ctrl Pts',(34.8401250147627,85.5887853699062,121.268016595053));
#35273=CARTESIAN_POINT('Ctrl Pts',(34.3411326976743,86.2509211367476,121.215367087322));
#35274=CARTESIAN_POINT('Ctrl Pts',(34.01641729094,86.681800886756,121.181105825712));
#35275=CARTESIAN_POINT('Ctrl Pts',(33.8434955298159,87.2270916620838,121.146844564102));
#35276=CARTESIAN_POINT('Ctrl Pts',(33.8399314485466,87.7703173734778,121.112583302492));
#35277=CARTESIAN_POINT('Origin',(36.3549260746835,87.7685555885722,124.208423447177));
#35278=CARTESIAN_POINT('',(33.2766562951256,87.7693690681389,107.791576552823));
#35279=CARTESIAN_POINT('',(33.2862967608848,87.7688698663354,107.708423447177));
#35280=CARTESIAN_POINT('',(33.2814260746835,87.7685555885726,124.208423447177));
#35281=CARTESIAN_POINT('',(37.1487253572158,84.7993326348264,107.));
#35282=CARTESIAN_POINT('Ctrl Pts',(33.2862967608848,87.7688698663354,107.708423447177));
#35283=CARTESIAN_POINT('Ctrl Pts',(33.285976896235,88.2640453572287,107.682880329042));
#35284=CARTESIAN_POINT('Ctrl Pts',(33.6322291916214,89.7793619789749,107.604687703175));
#35285=CARTESIAN_POINT('Ctrl Pts',(36.0033916785668,91.377417939733,107.473845569577));
#35286=CARTESIAN_POINT('Ctrl Pts',(39.1869515218405,90.0369600534397,107.315897046385));
#35287=CARTESIAN_POINT('Ctrl Pts',(39.7977189680597,86.63477600283,107.157948523192));
#35288=CARTESIAN_POINT('Ctrl Pts',(38.1309639469874,85.0619266872038,107.052649507731));
#35289=CARTESIAN_POINT('Ctrl Pts',(37.1487253572157,84.7993326348264,107.));
#35290=CARTESIAN_POINT('',(35.5611267921501,84.7993326348267,107.));
#35291=CARTESIAN_POINT('Origin',(36.3549260746835,87.7685555885722,107.));
#35292=CARTESIAN_POINT('Ctrl Pts',(33.2766562951256,87.7693690681389,107.791576552822));
#35293=CARTESIAN_POINT('Ctrl Pts',(33.2765002261982,87.813877907838,107.789262006108));
#35294=CARTESIAN_POINT('Ctrl Pts',(33.2974599420536,88.8706873775284,107.734297951662));
#35295=CARTESIAN_POINT('Ctrl Pts',(34.5067288269183,90.8887184689395,107.626684389486));
#35296=CARTESIAN_POINT('Ctrl Pts',(37.957394655155,91.0220939825006,107.468735866293));
#35297=CARTESIAN_POINT('Ctrl Pts',(39.9550037460998,88.2047806129811,107.310787343101));
#35298=CARTESIAN_POINT('Ctrl Pts',(38.702488609764,85.0282374153775,107.154542054336));
#35299=CARTESIAN_POINT('Ctrl Pts',(36.5061791859533,84.5433632538305,107.050946273303));
#35300=CARTESIAN_POINT('Ctrl Pts',(35.5592127316546,84.7942440238826,107.));
#35301=CARTESIAN_POINT('Origin',(36.3549260746835,87.7685555885722,124.208423447177));
#35302=CARTESIAN_POINT('',(33.2850145408684,87.7704209831421,108.791576552823));
#35303=CARTESIAN_POINT('',(33.2798329301067,87.7659973109231,108.708423447177));
#35304=CARTESIAN_POINT('',(33.2814260746835,87.7685555885726,124.208423447177));
#35305=CARTESIAN_POINT('Ctrl Pts',(33.2798329301067,87.7659973109231,108.708423447178));
#35306=CARTESIAN_POINT('Ctrl Pts',(33.28722078683,88.5947453986223,108.665444042093));
#35307=CARTESIAN_POINT('Ctrl Pts',(34.0588698820238,90.4508359457567,108.569815129278));
#35308=CARTESIAN_POINT('Ctrl Pts',(37.1879239641774,91.2981289902626,108.421536708732));
#35309=CARTESIAN_POINT('Ctrl Pts',(39.7658203407947,89.0005544503459,108.26358818554));
#35310=CARTESIAN_POINT('Ctrl Pts',(39.2510963194207,85.5858974977915,108.105639662347));
#35311=CARTESIAN_POINT('Ctrl Pts',(36.1106391940357,84.1503270588856,107.947691139155));
#35312=CARTESIAN_POINT('Ctrl Pts',(33.6634843338243,85.6966940980861,107.815285734098));
#35313=CARTESIAN_POINT('Ctrl Pts',(33.2866362016597,87.2433890028545,107.735529836772));
#35314=CARTESIAN_POINT('Ctrl Pts',(33.2862967608848,87.7688698663354,107.708423447177));
#35315=CARTESIAN_POINT('Ctrl Pts',(33.2850145408684,87.7704209831421,108.791576552823));
#35316=CARTESIAN_POINT('Ctrl Pts',(33.2828704095411,88.1529039380672,108.771825719159));
#35317=CARTESIAN_POINT('Ctrl Pts',(33.5258648203393,89.5523399236073,108.699425377765));
#35318=CARTESIAN_POINT('Ctrl Pts',(35.6128383205754,91.3183646214857,108.57437552864));
#35319=CARTESIAN_POINT('Ctrl Pts',(38.9216914949492,90.3305042873106,108.416427005448));
#35320=CARTESIAN_POINT('Ctrl Pts',(39.9033345805337,87.019792348641,108.258478482255));
#35321=CARTESIAN_POINT('Ctrl Pts',(37.667747597468,84.3879831424088,108.100529959063));
#35322=CARTESIAN_POINT('Ctrl Pts',(34.2920593632494,84.8148430265618,107.944895982585));
#35323=CARTESIAN_POINT('Ctrl Pts',(33.280050360721,86.80142545452,107.841911513838));
#35324=CARTESIAN_POINT('Ctrl Pts',(33.2766562951256,87.7693690681389,107.791576552822));
#35325=CARTESIAN_POINT('Origin',(36.3549260746835,87.7685555885722,124.208423447177));
#35326=CARTESIAN_POINT('',(33.2830912889668,87.7659629281698,109.791576552823));
#35327=CARTESIAN_POINT('',(33.2787949818699,87.7708236399759,109.708423447177));
#35328=CARTESIAN_POINT('',(33.2814260746835,87.7685555885726,124.208423447177));
#35329=CARTESIAN_POINT('Ctrl Pts',(33.2787949818699,87.7708236399759,109.708423447177));
#35330=CARTESIAN_POINT('Ctrl Pts',(33.2775558603757,87.9204433996099,109.700657262876));
#35331=CARTESIAN_POINT('Ctrl Pts',(33.3552187612325,89.0830934618413,109.640241570843));
#35332=CARTESIAN_POINT('Ctrl Pts',(34.836575933406,91.0619526923221,109.527176371079));
#35333=CARTESIAN_POINT('Ctrl Pts',(38.2826269365773,90.8403335175675,109.369227847887));
#35334=CARTESIAN_POINT('Ctrl Pts',(39.9808906224645,87.8336271456654,109.211279324694));
#35335=CARTESIAN_POINT('Ctrl Pts',(38.3916016557803,84.7679214934147,109.053330801502));
#35336=CARTESIAN_POINT('Ctrl Pts',(34.9557226837823,84.4228013221572,108.89538227831));
#35337=CARTESIAN_POINT('Ctrl Pts',(33.3781907756738,86.3796382265152,108.780413160201));
#35338=CARTESIAN_POINT('Ctrl Pts',(33.2781707076373,87.5795340720654,108.718093549824));
#35339=CARTESIAN_POINT('Ctrl Pts',(33.2798329301067,87.7659973109231,108.708423447178));
#35340=CARTESIAN_POINT('Ctrl Pts',(33.2830912889669,87.7659629281698,109.791576552823));
#35341=CARTESIAN_POINT('Ctrl Pts',(33.2889507344551,88.4849690844241,109.754389432211));
#35342=CARTESIAN_POINT('Ctrl Pts',(33.8981616653641,90.2308908653449,109.664552803868));
#35343=CARTESIAN_POINT('Ctrl Pts',(36.7983710512446,91.3678894898621,109.522066667795));
#35344=CARTESIAN_POINT('Ctrl Pts',(39.6112488575384,89.3648670312859,109.364118144603));
#35345=CARTESIAN_POINT('Ctrl Pts',(39.4717178074565,85.914517396569,109.20616962141));
#35346=CARTESIAN_POINT('Ctrl Pts',(36.5062865391415,84.1451680917577,109.048221098218));
#35347=CARTESIAN_POINT('Ctrl Pts',(33.7915971699313,85.4714805121635,108.910023408688));
#35348=CARTESIAN_POINT('Ctrl Pts',(33.2885859889854,87.1333247326767,108.82447522689));
#35349=CARTESIAN_POINT('Ctrl Pts',(33.2850145408684,87.7704209831421,108.791576552823));
#35350=CARTESIAN_POINT('Origin',(36.3549260746835,87.7685555885722,124.208423447177));
#35351=CARTESIAN_POINT('',(33.276584510365,87.769240395449,110.791576552823));
#35352=CARTESIAN_POINT('',(33.2862066546329,87.7689040049629,110.708423447177));
#35353=CARTESIAN_POINT('',(33.2814260746835,87.7685555885726,124.208423447177));
#35354=CARTESIAN_POINT('Ctrl Pts',(33.2862066546329,87.7689040049629,110.708423447177));
#35355=CARTESIAN_POINT('Ctrl Pts',(33.2857073591617,88.2574355602479,110.683220975927));
#35356=CARTESIAN_POINT('Ctrl Pts',(33.6253684480904,89.7658836642612,110.605368996946));
#35357=CARTESIAN_POINT('Ctrl Pts',(35.980893460476,91.3757637943158,110.474867510234));
#35358=CARTESIAN_POINT('Ctrl Pts',(39.1709558328596,90.0536874920861,110.316918987042));
#35359=CARTESIAN_POINT('Ctrl Pts',(39.8078096748032,86.6597515977284,110.158970463849));
#35360=CARTESIAN_POINT('Ctrl Pts',(37.3140389596571,84.2711345475141,110.001021940657));
#35361=CARTESIAN_POINT('Ctrl Pts',(34.1160435691142,85.0150534951715,109.850839601766));
#35362=CARTESIAN_POINT('Ctrl Pts',(33.2859562709446,86.906122030792,109.753306770606));
#35363=CARTESIAN_POINT('Ctrl Pts',(33.2787949818699,87.7708236399759,109.708423447177));
#35364=CARTESIAN_POINT('Ctrl Pts',(33.276584510365,87.769240395449,110.791576552823));
#35365=CARTESIAN_POINT('Ctrl Pts',(33.276468866392,87.8071966833456,110.789602652993));
#35366=CARTESIAN_POINT('Ctrl Pts',(33.2942328067559,88.8574441094525,110.734979245433));
#35367=CARTESIAN_POINT('Ctrl Pts',(34.4867513670091,90.8768945953326,110.627706330142));
#35368=CARTESIAN_POINT('Ctrl Pts',(37.9364315807433,91.0320948408579,110.46975780695));
#35369=CARTESIAN_POINT('Ctrl Pts',(39.9522088516144,88.2283433032996,110.311809283757));
#35370=CARTESIAN_POINT('Ctrl Pts',(38.7064392347119,85.0077162267496,110.153860760565));
#35371=CARTESIAN_POINT('Ctrl Pts',(35.3286241543516,84.290258236255,109.995912237372));
#35372=CARTESIAN_POINT('Ctrl Pts',(33.4575133987375,86.1528900623526,109.875150834792));
#35373=CARTESIAN_POINT('Ctrl Pts',(33.2806549343109,87.4670005092958,109.807038939942));
#35374=CARTESIAN_POINT('Ctrl Pts',(33.2830912889669,87.7659629281698,109.791576552823));
#35375=CARTESIAN_POINT('Origin',(36.3549260746835,87.7685555885722,124.208423447177));
#35376=CARTESIAN_POINT('',(33.2848888934257,87.7704976439917,111.791576552823));
#35377=CARTESIAN_POINT('',(33.2800258531095,87.7659597947519,111.708423447178));
#35378=CARTESIAN_POINT('',(33.2814260746835,87.7685555885726,124.208423447177));
#35379=CARTESIAN_POINT('Ctrl Pts',(33.2800258531095,87.7659597947519,111.708423447177));
#35380=CARTESIAN_POINT('Ctrl Pts',(33.2874067328936,88.5882718431644,111.665784688979));
#35381=CARTESIAN_POINT('Ctrl Pts',(34.0488667182543,90.4380268123453,111.570496423049));
#35382=CARTESIAN_POINT('Ctrl Pts',(37.1652522149781,91.3034138569667,111.422558649389));
#35383=CARTESIAN_POINT('Ctrl Pts',(39.7578212468625,89.0224119911016,111.264610126197));
#35384=CARTESIAN_POINT('Ctrl Pts',(39.2650887205849,85.6045766594567,111.106661603004));
#35385=CARTESIAN_POINT('Ctrl Pts',(36.1338002317116,84.1487552082432,110.948713079812));
#35386=CARTESIAN_POINT('Ctrl Pts',(33.6706421352838,85.6835151702931,110.81596702787));
#35387=CARTESIAN_POINT('Ctrl Pts',(33.2867504180154,87.2368631869536,110.735870483658));
#35388=CARTESIAN_POINT('Ctrl Pts',(33.2862066546329,87.7689040049629,110.708423447177));
#35389=CARTESIAN_POINT('Ctrl Pts',(33.2848888934257,87.7704976439917,111.791576552823));
#35390=CARTESIAN_POINT('Ctrl Pts',(33.2826892164494,88.1463451423912,111.772166366045));
#35391=CARTESIAN_POINT('Ctrl Pts',(33.5201235146107,89.5389847191594,111.700106671536));
#35392=CARTESIAN_POINT('Ctrl Pts',(35.5900605517025,91.3135279228,111.575397469297));
#35393=CARTESIAN_POINT('Ctrl Pts',(38.9051877964048,90.346929740897,111.417448946105));
#35394=CARTESIAN_POINT('Ctrl Pts',(39.9080703007288,87.0425981327984,111.259500422912));
#35395=CARTESIAN_POINT('Ctrl Pts',(37.6894249992898,84.3964700708273,111.10155189972));
#35396=CARTESIAN_POINT('Ctrl Pts',(34.3036776321515,84.8025700881101,110.945577276356));
#35397=CARTESIAN_POINT('Ctrl Pts',(33.279553419195,86.794794816033,110.842252160724));
#35398=CARTESIAN_POINT('Ctrl Pts',(33.276584510365,87.769240395449,110.791576552823));
#35399=CARTESIAN_POINT('Origin',(36.3549260746835,87.7685555885722,124.208423447177));
#35400=CARTESIAN_POINT('',(33.2832673812772,87.7659995884264,112.791576552823));
#35401=CARTESIAN_POINT('',(33.2786192000661,87.7707578837754,112.708423447177));
#35402=CARTESIAN_POINT('',(33.2814260746835,87.7685555885726,124.208423447177));
#35403=CARTESIAN_POINT('Ctrl Pts',(33.2786192000661,87.7707578837754,112.708423447177));
#35404=CARTESIAN_POINT('Ctrl Pts',(33.2774583365245,87.9137935758715,112.700997909761));
#35405=CARTESIAN_POINT('Ctrl Pts',(33.3512646696384,89.0697957630776,112.640922864614));
#35406=CARTESIAN_POINT('Ctrl Pts',(34.8154602798326,91.0521354182212,112.528198311736));
#35407=CARTESIAN_POINT('Ctrl Pts',(38.2628634325534,90.8526480757781,112.370249788544));
#35408=CARTESIAN_POINT('Ctrl Pts',(39.9803978101849,87.856907873618,112.212301265351));
#35409=CARTESIAN_POINT('Ctrl Pts',(38.4108272289767,84.7810613417211,112.054352742159));
#35410=CARTESIAN_POINT('Ctrl Pts',(34.977233598576,84.4138849829118,111.896404218966));
#35411=CARTESIAN_POINT('Ctrl Pts',(33.3824603545734,86.36632237616,111.781094453973));
#35412=CARTESIAN_POINT('Ctrl Pts',(33.2782929663659,87.5728969500129,111.71843419671));
#35413=CARTESIAN_POINT('Ctrl Pts',(33.2800258531095,87.7659597947519,111.708423447177));
#35414=CARTESIAN_POINT('Ctrl Pts',(33.2832673812772,87.7659995884264,112.791576552823));
#35415=CARTESIAN_POINT('Ctrl Pts',(33.2889664337279,88.478522942157,112.754730079096));
#35416=CARTESIAN_POINT('Ctrl Pts',(33.8893177002825,90.2178279476355,112.66523409764));
#35417=CARTESIAN_POINT('Ctrl Pts',(36.7752505958151,91.3706626685477,112.523088608452));
#35418=CARTESIAN_POINT('Ctrl Pts',(39.6009318089752,89.3857429282516,112.365140085259));
#35419=CARTESIAN_POINT('Ctrl Pts',(39.4835583456547,85.9345686115981,112.207191562067));
#35420=CARTESIAN_POINT('Ctrl Pts',(36.5295491552939,84.1462145087741,112.049243038874));
#35421=CARTESIAN_POINT('Ctrl Pts',(33.799687217845,85.4582952370342,111.91070470246));
#35422=CARTESIAN_POINT('Ctrl Pts',(33.2886557695433,87.1268708838871,111.824815873776));
#35423=CARTESIAN_POINT('Ctrl Pts',(33.2848888934257,87.7704976439917,111.791576552823));
#35424=CARTESIAN_POINT('Origin',(36.3549260746835,87.7685555885722,124.208423447177));
#35425=CARTESIAN_POINT('',(33.2765252740224,87.769124500281,113.791576552823));
#35426=CARTESIAN_POINT('',(33.2861807775267,87.7690089236533,113.708423447177));
#35427=CARTESIAN_POINT('',(33.2814260746835,87.7685555885726,124.208423447177));
#35428=CARTESIAN_POINT('Ctrl Pts',(33.2861807775267,87.7690089236533,113.708423447177));
#35429=CARTESIAN_POINT('Ctrl Pts',(33.2855396007978,88.2509271303222,113.683561622813));
#35430=CARTESIAN_POINT('Ctrl Pts',(33.618721374071,89.7525576542612,113.606050290718));
#35431=CARTESIAN_POINT('Ctrl Pts',(35.9577392922369,91.3732877687825,113.475889450891));
#35432=CARTESIAN_POINT('Ctrl Pts',(39.1562249541521,90.071722108623,113.317940927699));
#35433=CARTESIAN_POINT('Ctrl Pts',(39.8148581197072,86.6819454123766,113.159992404506));
#35434=CARTESIAN_POINT('Ctrl Pts',(37.3364761291159,84.2773651151324,113.002043881314));
#35435=CARTESIAN_POINT('Ctrl Pts',(34.1265054947725,85.0023751466479,112.851520895538));
#35436=CARTESIAN_POINT('Ctrl Pts',(33.2856892416539,86.8996233744842,112.753647417492));
#35437=CARTESIAN_POINT('Ctrl Pts',(33.2786192000661,87.7707578837754,112.708423447177));
#35438=CARTESIAN_POINT('Ctrl Pts',(33.2765252740224,87.769124500281,113.791576552822));
#35439=CARTESIAN_POINT('Ctrl Pts',(33.276444590752,87.800528839304,113.789943299879));
#35440=CARTESIAN_POINT('Ctrl Pts',(33.2910497583934,88.8442059367107,113.735660539204));
#35441=CARTESIAN_POINT('Ctrl Pts',(34.4668312392973,90.8648349705502,113.628728270799));
#35442=CARTESIAN_POINT('Ctrl Pts',(37.915443798023,91.0421824081436,113.470779747607));
#35443=CARTESIAN_POINT('Ctrl Pts',(39.9491823979981,88.2514319712908,113.312831224414));
#35444=CARTESIAN_POINT('Ctrl Pts',(38.7241181039884,85.0228722042484,113.154882701222));
#35445=CARTESIAN_POINT('Ctrl Pts',(35.3509794527264,84.2837400555871,112.996934178029));
#35446=CARTESIAN_POINT('Ctrl Pts',(33.4626356089268,86.1395392509273,112.875832128563));
#35447=CARTESIAN_POINT('Ctrl Pts',(33.2808231224224,87.4604064162848,112.807379586827));
#35448=CARTESIAN_POINT('Ctrl Pts',(33.2832673812772,87.7659995884264,112.791576552823));
#35449=CARTESIAN_POINT('Origin',(36.3549260746835,87.7685555885722,124.208423447177));
#35450=CARTESIAN_POINT('',(33.2847579912934,87.7705715943706,114.791576552823));
#35451=CARTESIAN_POINT('',(33.2802200364225,87.76592664843,114.708423447178));
#35452=CARTESIAN_POINT('',(33.2814260746835,87.7685555885726,124.208423447177));
#35453=CARTESIAN_POINT('Ctrl Pts',(33.2802200364225,87.76592664843,114.708423447177));
#35454=CARTESIAN_POINT('Ctrl Pts',(33.287581867814,88.5818020912728,114.666125335864));
#35455=CARTESIAN_POINT('Ctrl Pts',(34.0389365462666,90.4252032852303,114.571177716821));
#35456=CARTESIAN_POINT('Ctrl Pts',(37.1425381909624,91.3085440893281,114.423580590046));
#35457=CARTESIAN_POINT('Ctrl Pts',(39.749700086851,89.0442361275419,114.265632066853));
#35458=CARTESIAN_POINT('Ctrl Pts',(39.2789236332919,85.6233074191414,114.107683543661));
#35459=CARTESIAN_POINT('Ctrl Pts',(36.1570475227083,84.1474099811903,113.949735020469));
#35460=CARTESIAN_POINT('Ctrl Pts',(33.6777395096476,85.6702201339644,113.816648321641));
#35461=CARTESIAN_POINT('Ctrl Pts',(33.2868974110151,87.2303762658505,113.736211130544));
#35462=CARTESIAN_POINT('Ctrl Pts',(33.2861807775267,87.7690089236533,113.708423447177));
#35463=CARTESIAN_POINT('Ctrl Pts',(33.2847579912934,87.7705715943706,114.791576552823));
#35464=CARTESIAN_POINT('Ctrl Pts',(33.2825084886882,88.1397834143597,114.772507012931));
#35465=CARTESIAN_POINT('Ctrl Pts',(33.5144368848445,89.5256293817944,114.700787965308));
#35466=CARTESIAN_POINT('Ctrl Pts',(35.5673140575926,91.308543643525,114.576419409954));
#35467=CARTESIAN_POINT('Ctrl Pts',(38.8885794869123,90.3632518146024,114.418470886761));
#35468=CARTESIAN_POINT('Ctrl Pts',(39.9126584249495,87.0654278316568,114.260522363569));
#35469=CARTESIAN_POINT('Ctrl Pts',(37.7110496445387,84.4051084012425,114.102573840377));
#35470=CARTESIAN_POINT('Ctrl Pts',(34.3153645284242,84.7902995884757,113.946258570128));
#35471=CARTESIAN_POINT('Ctrl Pts',(33.2790454949687,86.7881792233995,113.84259280761));
#35472=CARTESIAN_POINT('Ctrl Pts',(33.2765252740224,87.769124500281,113.791576552822));
#35473=CARTESIAN_POINT('Origin',(36.3549260746835,87.7685555885722,124.208423447177));
#35474=CARTESIAN_POINT('',(33.2834401666397,87.7660402135948,115.791576552823));
#35475=CARTESIAN_POINT('',(33.2784472978679,87.7706880983643,115.708423447177));
#35476=CARTESIAN_POINT('',(33.2814260746835,87.7685555885726,124.208423447177));
#35477=CARTESIAN_POINT('Ctrl Pts',(33.2784472978679,87.7706880983643,115.708423447178));
#35478=CARTESIAN_POINT('Ctrl Pts',(33.277364762304,87.9071421036308,115.701338556647));
#35479=CARTESIAN_POINT('Ctrl Pts',(33.3473574841613,89.0565012331312,115.641604158386));
#35480=CARTESIAN_POINT('Ctrl Pts',(34.7944081548233,91.0421828204038,115.529220252393));
#35481=CARTESIAN_POINT('Ctrl Pts',(38.2430211478453,90.8648353604754,115.371271729201));
#35482=CARTESIAN_POINT('Ctrl Pts',(39.9797557618474,87.8801852004548,115.213323206008));
#35483=CARTESIAN_POINT('Ctrl Pts',(38.4299675427095,84.7943238664015,115.055374682816));
#35484=CARTESIAN_POINT('Ctrl Pts',(34.9988023340458,84.4051079776717,114.897426159623));
#35485=CARTESIAN_POINT('Ctrl Pts',(33.386777168059,86.353002585266,114.781775747744));
#35486=CARTESIAN_POINT('Ctrl Pts',(33.2784184137796,87.5662617018335,114.718774843595));
#35487=CARTESIAN_POINT('Ctrl Pts',(33.2802200364225,87.76592664843,114.708423447177));
#35488=CARTESIAN_POINT('Ctrl Pts',(33.2834401666397,87.7660402135947,115.791576552823));
#35489=CARTESIAN_POINT('Ctrl Pts',(33.2889737590442,88.472076855709,115.755070725982));
#35490=CARTESIAN_POINT('Ctrl Pts',(33.8805399135678,90.2047528694839,115.665915391411));
#35491=CARTESIAN_POINT('Ctrl Pts',(36.752112807112,91.3732873148253,115.524110549109));
#35492=CARTESIAN_POINT('Ctrl Pts',(39.5904809358262,89.4065521878392,115.366162025916));
#35493=CARTESIAN_POINT('Ctrl Pts',(39.4952698768951,85.954695361712,115.208213502724));
#35494=CARTESIAN_POINT('Ctrl Pts',(36.5528046017381,84.1474104372141,115.050264979531));
#35495=CARTESIAN_POINT('Ctrl Pts',(33.8078411360195,85.4451187391524,114.911385996231));
#35496=CARTESIAN_POINT('Ctrl Pts',(33.2887191893906,87.1204184647656,114.825156520661));
#35497=CARTESIAN_POINT('Ctrl Pts',(33.2847579912934,87.7705715943706,114.791576552823));
#35498=CARTESIAN_POINT('Origin',(36.3549260746835,87.7685555885722,124.208423447177));
#35499=CARTESIAN_POINT('',(33.2764763687653,87.7690073305752,116.791576552823));
#35500=CARTESIAN_POINT('',(33.286148132912,87.7691131822086,116.708423447177));
#35501=CARTESIAN_POINT('',(33.2814260746835,87.7685555885726,124.208423447177));
#35502=CARTESIAN_POINT('Ctrl Pts',(33.286148132912,87.7691131822085,116.708423447177));
#35503=CARTESIAN_POINT('Ctrl Pts',(33.2853698282698,88.2444156975363,116.683902269699));
#35504=CARTESIAN_POINT('Ctrl Pts',(33.6121326413799,89.7392284566303,116.606731584489));
#35505=CARTESIAN_POINT('Ctrl Pts',(35.93460150062,91.3706631221744,116.476911391548));
#35506=CARTESIAN_POINT('Ctrl Pts',(39.1413785773383,90.0896617648689,116.318962868356));
#35507=CARTESIAN_POINT('Ctrl Pts',(39.8217639160215,86.7041840307689,116.161014345163));
#35508=CARTESIAN_POINT('Ctrl Pts',(37.3588728230703,84.2837396167312,116.003065821971));
#35509=CARTESIAN_POINT('Ctrl Pts',(34.1370382392348,84.9897175692517,115.852202189309));
#35510=CARTESIAN_POINT('Ctrl Pts',(33.2854093417222,86.8931199145531,115.753988064378));
#35511=CARTESIAN_POINT('Ctrl Pts',(33.2784472978679,87.7706880983643,115.708423447178));
#35512=CARTESIAN_POINT('Ctrl Pts',(33.2764763687653,87.7690073305752,116.791576552823));
#35513=CARTESIAN_POINT('Ctrl Pts',(33.2764248815123,87.7938606187569,116.790283946765));
#35514=CARTESIAN_POINT('Ctrl Pts',(33.2879103688746,88.830971516364,116.736341832976));
#35515=CARTESIAN_POINT('Ctrl Pts',(34.446988957088,90.8526476873878,116.629750211456));
#35516=CARTESIAN_POINT('Ctrl Pts',(37.894391675665,91.0521350047077,116.471801688264));
#35517=CARTESIAN_POINT('Ctrl Pts',(39.9460077545616,88.2745007309714,116.313853165071));
#35518=CARTESIAN_POINT('Ctrl Pts',(38.7416992921252,85.0381413842478,116.155904641879));
#35519=CARTESIAN_POINT('Ctrl Pts',(35.3733761438603,84.2773655547908,115.997956118686));
#35520=CARTESIAN_POINT('Ctrl Pts',(33.467810029404,86.1261873874685,115.876513422334));
#35521=CARTESIAN_POINT('Ctrl Pts',(33.2809930901675,87.453815255726,115.807720233713));
#35522=CARTESIAN_POINT('Ctrl Pts',(33.2834401666397,87.7660402135947,115.791576552823));
#35523=CARTESIAN_POINT('Origin',(36.3549260746835,87.7685555885722,124.208423447177));
#35524=CARTESIAN_POINT('',(33.2846219536775,87.7706425235964,117.791576552823));
#35525=CARTESIAN_POINT('',(33.2804152395068,87.7658979718733,117.708423447177));
#35526=CARTESIAN_POINT('',(33.2814260746835,87.7685555885726,124.208423447177));
#35527=CARTESIAN_POINT('Ctrl Pts',(33.2804152395068,87.7658979718733,117.708423447177));
#35528=CARTESIAN_POINT('Ctrl Pts',(33.2877456579952,88.5753352182883,117.66646598275));
#35529=CARTESIAN_POINT('Ctrl Pts',(34.029075680634,90.4123622121681,117.571859010592));
#35530=CARTESIAN_POINT('Ctrl Pts',(37.1197916939879,91.3135283692309,117.424602530703));
#35531=CARTESIAN_POINT('Ctrl Pts',(39.7414389614906,89.0660076681044,117.26665400751));
#35532=CARTESIAN_POINT('Ctrl Pts',(39.2926379906584,85.6421266266902,117.108705484318));
#35533=CARTESIAN_POINT('Ctrl Pts',(36.1803029720811,84.1462140525996,116.950756961126));
#35534=CARTESIAN_POINT('Ctrl Pts',(33.6848972085276,85.6569301160522,116.817329615412));
#35535=CARTESIAN_POINT('Ctrl Pts',(33.2870409289463,87.223891969559,116.736551777429));
#35536=CARTESIAN_POINT('Ctrl Pts',(33.286148132912,87.7691131822085,116.708423447177));
#35537=CARTESIAN_POINT('Ctrl Pts',(33.2846219536775,87.7706425235964,117.791576552823));
#35538=CARTESIAN_POINT('Ctrl Pts',(33.282328321745,88.1332185350583,117.772847659816));
#35539=CARTESIAN_POINT('Ctrl Pts',(33.5088046545594,89.5122738095575,117.701469259079));
#35540=CARTESIAN_POINT('Ctrl Pts',(35.5446000364372,91.3034134118094,117.577441350611));
#35541=CARTESIAN_POINT('Ctrl Pts',(38.8718667157924,90.3794669098942,117.419492827418));
#35542=CARTESIAN_POINT('Ctrl Pts',(39.9170998651258,87.0882865202323,117.261544304226));
#35543=CARTESIAN_POINT('Ctrl Pts',(37.7326183772922,84.4138854053773,117.103595781033));
#35544=CARTESIAN_POINT('Ctrl Pts',(34.3271247352706,84.778056850815,116.946939863899));
#35545=CARTESIAN_POINT('Ctrl Pts',(33.2785220235664,86.7815542163916,116.842933454495));
#35546=CARTESIAN_POINT('Ctrl Pts',(33.2764763687653,87.7690073305752,116.791576552823));
#35547=CARTESIAN_POINT('Origin',(36.3549260746835,87.7685555885722,124.208423447177));
#35548=CARTESIAN_POINT('',(33.2836094246712,87.7660847245338,118.791576552823));
#35549=CARTESIAN_POINT('',(33.2782796381252,87.770614382798,118.708423447178));
#35550=CARTESIAN_POINT('',(33.2814260746835,87.7685555885726,124.208423447177));
#35551=CARTESIAN_POINT('Ctrl Pts',(33.2782796381252,87.770614382798,118.708423447178));
#35552=CARTESIAN_POINT('Ctrl Pts',(33.2772752030302,87.9004890602186,118.701679203533));
#35553=CARTESIAN_POINT('Ctrl Pts',(33.3434970062078,89.0432099289289,118.642285452157));
#35554=CARTESIAN_POINT('Ctrl Pts',(34.7734203694599,91.0320952518487,118.53024219305));
#35555=CARTESIAN_POINT('Ctrl Pts',(38.223101017625,90.876894986776,118.372293669858));
#35556=CARTESIAN_POINT('Ctrl Pts',(39.9789642630779,87.9034579247835,118.214345146665));
#35557=CARTESIAN_POINT('Ctrl Pts',(38.4490223032137,84.8077090176302,118.056396623473));
#35558=CARTESIAN_POINT('Ctrl Pts',(35.020426982018,84.3964696461687,117.89844810028));
#35559=CARTESIAN_POINT('Ctrl Pts',(33.3911426763166,86.3396801807466,117.782457041515));
#35560=CARTESIAN_POINT('Ctrl Pts',(33.2785472250074,87.5596286415355,117.719115490481));
#35561=CARTESIAN_POINT('Ctrl Pts',(33.2804152395068,87.7658979718733,117.708423447177));
#35562=CARTESIAN_POINT('Ctrl Pts',(33.2836094246713,87.7660847245338,118.791576552823));
#35563=CARTESIAN_POINT('Ctrl Pts',(33.2889728976556,88.4656306785298,118.755411372868));
#35564=CARTESIAN_POINT('Ctrl Pts',(33.8718280977078,90.1916659326025,118.666596685182));
#35565=CARTESIAN_POINT('Ctrl Pts',(36.7289586417865,91.3757633400502,118.525132489766));
#35566=CARTESIAN_POINT('Ctrl Pts',(39.5798966622645,89.4272939130391,118.367183966573));
#35567=CARTESIAN_POINT('Ctrl Pts',(39.5068519326957,85.9748968968193,118.209235443381));
#35568=CARTESIAN_POINT('Ctrl Pts',(36.5760518898075,84.1487556640973,118.051286920188));
#35569=CARTESIAN_POINT('Ctrl Pts',(33.8160591927152,85.4319515714374,117.912067290002));
#35570=CARTESIAN_POINT('Ctrl Pts',(33.2887760382289,87.1139672364392,117.825497167547));
#35571=CARTESIAN_POINT('Ctrl Pts',(33.2846219536775,87.7706425235964,117.791576552823));
#35572=CARTESIAN_POINT('Origin',(36.3549260746835,87.7685555885722,124.208423447177));
#35573=CARTESIAN_POINT('',(33.2764381388873,87.7688891883613,119.791576552823));
#35574=CARTESIAN_POINT('',(33.2861087598917,87.7692166140277,119.708423447178));
#35575=CARTESIAN_POINT('',(33.2814260746835,87.7685555885726,124.208423447177));
#35576=CARTESIAN_POINT('Ctrl Pts',(33.2861087598917,87.7692166140277,119.708423447178));
#35577=CARTESIAN_POINT('Ctrl Pts',(33.2851982067878,88.237901225937,119.684242916584));
#35578=CARTESIAN_POINT('Ctrl Pts',(33.6056020130081,89.7258962979527,119.60741287826));
#35579=CARTESIAN_POINT('Ctrl Pts',(35.91148104228,91.3678899431996,119.477933332205));
#35580=CARTESIAN_POINT('Ctrl Pts',(39.1264173144016,90.1075057318468,119.319984809013));
#35581=CARTESIAN_POINT('Ctrl Pts',(39.8285267766549,86.7264665283904,119.16203628582));
#35582=CARTESIAN_POINT('Ctrl Pts',(37.3812281242605,84.2902577982121,119.004087762628));
#35583=CARTESIAN_POINT('Ctrl Pts',(34.1476419553814,84.9770811380528,118.85288348308));
#35584=CARTESIAN_POINT('Ctrl Pts',(33.2851164104484,86.8866114198347,118.754328711263));
#35585=CARTESIAN_POINT('Ctrl Pts',(33.2782796381252,87.770614382798,118.708423447178));
#35586=CARTESIAN_POINT('Ctrl Pts',(33.2764381388873,87.7688891883613,119.791576552823));
#35587=CARTESIAN_POINT('Ctrl Pts',(33.2764096940567,87.7871921565167,119.79062459365));
#35588=CARTESIAN_POINT('Ctrl Pts',(33.2848143365715,88.8177409867468,119.737023126747));
#35589=CARTESIAN_POINT('Ctrl Pts',(34.4272254557842,90.8403331303497,119.630772152113));
#35590=CARTESIAN_POINT('Ctrl Pts',(37.873276024629,91.0619522777656,119.47282362892));
#35591=CARTESIAN_POINT('Ctrl Pts',(39.9426850798466,88.2975486028455,119.314875105728));
#35592=CARTESIAN_POINT('Ctrl Pts',(38.7591820609565,85.0535231518079,119.156926582535));
#35593=CARTESIAN_POINT('Ctrl Pts',(35.3958133105107,84.2711349879319,118.998978059343));
#35594=CARTESIAN_POINT('Ctrl Pts',(33.4730368857783,86.1128345972822,118.877194716105));
#35595=CARTESIAN_POINT('Ctrl Pts',(33.2811647182768,87.4472270604913,118.808060880599));
#35596=CARTESIAN_POINT('Ctrl Pts',(33.2836094246713,87.7660847245338,118.791576552823));
#35597=CARTESIAN_POINT('Origin',(36.3549260746835,87.7685555885722,124.208423447177));
#35598=CARTESIAN_POINT('',(33.2844847704405,87.7707064707598,120.791576552823));
#35599=CARTESIAN_POINT('',(33.2806115013714,87.7658718718852,120.708423447177));
#35600=CARTESIAN_POINT('',(33.2814260746835,87.7685555885726,124.208423447177));
#35601=CARTESIAN_POINT('Ctrl Pts',(33.2806115013714,87.7658718718852,120.708423447177));
#35602=CARTESIAN_POINT('Ctrl Pts',(33.2878986300211,88.5688691391512,120.666806629636));
#35603=CARTESIAN_POINT('Ctrl Pts',(34.0192834572627,90.3995065690792,120.572540304363));
#35604=CARTESIAN_POINT('Ctrl Pts',(37.0970139225816,91.3183650716777,120.42562447136));
#35605=CARTESIAN_POINT('Ctrl Pts',(39.7330380846501,89.0877264053273,120.267675948167));
#35606=CARTESIAN_POINT('Ctrl Pts',(39.3062312888321,85.6610331706022,120.109727424975));
#35607=CARTESIAN_POINT('Ctrl Pts',(36.2035655911394,84.1451676350087,119.951778901782));
#35608=CARTESIAN_POINT('Ctrl Pts',(33.6921154687428,85.6436453024385,119.818010909183));
#35609=CARTESIAN_POINT('Ctrl Pts',(33.2871808006975,87.2174102155021,119.736892424315));
#35610=CARTESIAN_POINT('Ctrl Pts',(33.2861087598917,87.7692166140277,119.708423447178));
#35611=CARTESIAN_POINT('Ctrl Pts',(33.2844847704405,87.7707064707598,120.791576552823));
#35612=CARTESIAN_POINT('Ctrl Pts',(33.2821494402512,88.1266499264814,120.773188306702));
#35613=CARTESIAN_POINT('Ctrl Pts',(33.503214227886,89.498930569182,120.70215055285));
#35614=CARTESIAN_POINT('Ctrl Pts',(35.5219282988626,91.2981285259009,120.578463291268));
#35615=CARTESIAN_POINT('Ctrl Pts',(38.8550458568218,90.3955786925481,120.420514768075));
#35616=CARTESIAN_POINT('Ctrl Pts',(39.9213965365604,87.1111711483864,120.262566244883));
#35617=CARTESIAN_POINT('Ctrl Pts',(37.7541292878677,84.4228017462871,120.10461772169));
#35618=CARTESIAN_POINT('Ctrl Pts',(34.3389588652922,84.7658418233948,119.94762115767));
#35619=CARTESIAN_POINT('Ctrl Pts',(33.2779828774206,86.7749194757506,119.843274101381));
#35620=CARTESIAN_POINT('Ctrl Pts',(33.2764381388873,87.7688891883613,119.791576552823));
#35621=CARTESIAN_POINT('Origin',(36.3549260746835,87.7685555885722,124.208423447177));
#35622=CARTESIAN_POINT('',(33.2846474150427,87.7655400361929,121.791576552823));
#35623=CARTESIAN_POINT('',(33.2781263393751,87.7704832126689,121.708423447178));
#35624=CARTESIAN_POINT('',(33.2814260746835,87.7685555885726,124.208423447177));
#35625=CARTESIAN_POINT('',(35.5611267921504,84.7993326348266,122.));
#35626=CARTESIAN_POINT('Ctrl Pts',(35.5611267921505,84.7993326348266,122.));
#35627=CARTESIAN_POINT('Ctrl Pts',(34.5788882023788,85.0619266872043,121.947350492269));
#35628=CARTESIAN_POINT('Ctrl Pts',(33.4791914426982,86.0996627851545,121.877876009877));
#35629=CARTESIAN_POINT('Ctrl Pts',(33.2823062253025,87.4400641803626,121.808401527484));
#35630=CARTESIAN_POINT('Ctrl Pts',(33.2846474150427,87.7655400361928,121.791576552823));
#35631=CARTESIAN_POINT('',(37.1506349127216,84.7942560800323,122.));
#35632=CARTESIAN_POINT('Origin',(36.3549260746835,87.7685555885722,122.));
#35633=CARTESIAN_POINT('Ctrl Pts',(37.1506395481982,84.7942437566139,122.));
#35634=CARTESIAN_POINT('Ctrl Pts',(36.2036733898099,84.5433632815128,121.949053726697));
#35635=CARTESIAN_POINT('Ctrl Pts',(34.1431239694285,84.9982647715874,121.851861542423));
#35636=CARTESIAN_POINT('Ctrl Pts',(33.284789784195,86.880208399197,121.754669358149));
#35637=CARTESIAN_POINT('Ctrl Pts',(33.2781263393751,87.7704832126688,121.708423447178));
#35638=CARTESIAN_POINT('Origin',(87.7685555885722,36.3549260746835,114.));
#35639=CARTESIAN_POINT('',(85.2550451615384,36.3551834992055,107.387416697508));
#35640=CARTESIAN_POINT('',(85.252964853222,36.3513534825213,107.112583302492));
#35641=CARTESIAN_POINT('',(85.2510555885723,36.3549260746835,114.));
#35642=CARTESIAN_POINT('',(85.8550895919076,37.9909132780589,107.));
#35643=CARTESIAN_POINT('Ctrl Pts',(85.252964853222,36.3513534825213,107.112583302492));
#35644=CARTESIAN_POINT('Ctrl Pts',(85.2581102783477,36.9439881062406,107.075055534995));
#35645=CARTESIAN_POINT('Ctrl Pts',(85.4693337604884,37.5397296349884,107.037527767497));
#35646=CARTESIAN_POINT('Ctrl Pts',(85.8550895919077,37.9909132780591,107.));
#35647=CARTESIAN_POINT('',(85.2510555885723,36.3549260746835,107.));
#35648=CARTESIAN_POINT('Origin',(87.7685555885722,36.3549260746835,107.));
#35649=CARTESIAN_POINT('',(85.2510555885723,36.3549260746835,106.));
#35650=CARTESIAN_POINT('',(85.2510555885723,36.3549260746835,114.));
#35651=CARTESIAN_POINT('Origin',(87.7685555885722,36.3549260746835,106.));
#35652=CARTESIAN_POINT('',(89.6856659519484,37.9934540791198,107.));
#35653=CARTESIAN_POINT('Origin',(87.7685555885722,36.3549260746835,107.));
#35654=CARTESIAN_POINT('Ctrl Pts',(89.6856747987073,37.9934602469553,107.));
#35655=CARTESIAN_POINT('Ctrl Pts',(89.1628542734512,38.6021751401191,107.050946273303));
#35656=CARTESIAN_POINT('Ctrl Pts',(88.3231296868319,38.9423518194042,107.101892546605));
#35657=CARTESIAN_POINT('Ctrl Pts',(87.5244587588995,38.8645890944017,107.152838819908));
#35658=CARTESIAN_POINT('Ctrl Pts',(86.6990866861522,38.7842266080846,107.205488327639));
#35659=CARTESIAN_POINT('Ctrl Pts',(85.9175591672441,38.2575125102682,107.25813783537));
#35660=CARTESIAN_POINT('Ctrl Pts',(85.5336745304453,37.5227256538998,107.3107873431));
#35661=CARTESIAN_POINT('Ctrl Pts',(85.3474313716597,37.1662408872642,107.336330461236));
#35662=CARTESIAN_POINT('Ctrl Pts',(85.2547831608045,36.7607811235179,107.361873579372));
#35663=CARTESIAN_POINT('Ctrl Pts',(85.2550451615384,36.3551834992055,107.387416697508));
#35664=CARTESIAN_POINT('Origin',(87.7685555885722,36.3549260746835,114.));
#35665=CARTESIAN_POINT('',(85.249750645845,36.3528305926657,108.387416697508));
#35666=CARTESIAN_POINT('',(85.2471486681112,36.3555923947772,108.112583302492));
#35667=CARTESIAN_POINT('',(85.2510555885723,36.3549260746835,114.));
#35668=CARTESIAN_POINT('Ctrl Pts',(85.2471486681112,36.3555923947772,108.112583302492));
#35669=CARTESIAN_POINT('Ctrl Pts',(85.2470208322483,36.3920495296211,108.110268755777));
#35670=CARTESIAN_POINT('Ctrl Pts',(85.2477437832137,36.4285014277137,108.107954209062));
#35671=CARTESIAN_POINT('Ctrl Pts',(85.2493333996998,36.464915427552,108.105639662347));
#35672=CARTESIAN_POINT('Ctrl Pts',(85.2854927586503,37.2932327622759,108.052990154616));
#35673=CARTESIAN_POINT('Ctrl Pts',(85.7700961483552,38.1019401719081,108.000340646886));
#35674=CARTESIAN_POINT('Ctrl Pts',(86.48347051945,38.5245018294053,107.947691139155));
#35675=CARTESIAN_POINT('Ctrl Pts',(87.1968448905449,38.9470634869024,107.895041631424));
#35676=CARTESIAN_POINT('Ctrl Pts',(88.1389902430297,38.9834793922643,107.842392123693));
#35677=CARTESIAN_POINT('Ctrl Pts',(88.8827694366222,38.6170777029647,107.789742615962));
#35678=CARTESIAN_POINT('Ctrl Pts',(89.6265486302147,38.250676013665,107.737093108232));
#35679=CARTESIAN_POINT('Ctrl Pts',(90.1719616649149,37.4814567297037,107.684443600501));
#35680=CARTESIAN_POINT('Ctrl Pts',(90.2718152971076,36.6584694261649,107.63179409277));
#35681=CARTESIAN_POINT('Ctrl Pts',(90.3716689293003,35.8354821226262,107.579144585039));
#35682=CARTESIAN_POINT('Ctrl Pts',(90.0259631589855,34.9587267995101,107.526495077308));
#35683=CARTESIAN_POINT('Ctrl Pts',(89.3912932551831,34.4249748964641,107.473845569577));
#35684=CARTESIAN_POINT('Ctrl Pts',(88.7566233513807,33.8912229934181,107.421196061847));
#35685=CARTESIAN_POINT('Ctrl Pts',(87.8329893140907,33.7004745104421,107.368546554116));
#35686=CARTESIAN_POINT('Ctrl Pts',(87.0393721878608,33.9406285523688,107.315897046385));
#35687=CARTESIAN_POINT('Ctrl Pts',(86.2457550616309,34.1807825942955,107.263247538654));
#35688=CARTESIAN_POINT('Ctrl Pts',(85.5821548464612,34.8518391611248,107.210598030923));
#35689=CARTESIAN_POINT('Ctrl Pts',(85.3491896324499,35.6461250305103,107.157948523192));
#35690=CARTESIAN_POINT('Ctrl Pts',(85.2822784759824,35.8742560255688,107.142826782959));
#35691=CARTESIAN_POINT('Ctrl Pts',(85.2508915142698,36.1125525244339,107.127705042726));
#35692=CARTESIAN_POINT('Ctrl Pts',(85.252964853222,36.3513534825213,107.112583302492));
#35693=CARTESIAN_POINT('Ctrl Pts',(85.2550451615384,36.3551834992055,107.387416697508));
#35694=CARTESIAN_POINT('Ctrl Pts',(85.2553231970519,35.9247627821685,107.414523087103));
#35695=CARTESIAN_POINT('Ctrl Pts',(85.3602318955731,35.49418681371,107.441629476698));
#35696=CARTESIAN_POINT('Ctrl Pts',(85.5689529493409,35.1218193835969,107.468735866293));
#35697=CARTESIAN_POINT('Ctrl Pts',(85.9743577597246,34.398559584583,107.521385374024));
#35698=CARTESIAN_POINT('Ctrl Pts',(86.7714091351813,33.8948996014755,107.574034881755));
#35699=CARTESIAN_POINT('Ctrl Pts',(87.5986589058312,33.8390486012967,107.626684389485));
#35700=CARTESIAN_POINT('Ctrl Pts',(88.4259086764811,33.7831976011178,107.679333897216));
#35701=CARTESIAN_POINT('Ctrl Pts',(89.2833568423243,34.1751555838677,107.731983404947));
#35702=CARTESIAN_POINT('Ctrl Pts',(89.7823492254361,34.8372914473242,107.784632912678));
#35703=CARTESIAN_POINT('Ctrl Pts',(90.281341608548,35.4994273107807,107.837282420409));
#35704=CARTESIAN_POINT('Ctrl Pts',(90.4218782089285,36.4317410549438,107.889931928139));
#35705=CARTESIAN_POINT('Ctrl Pts',(90.1402212269685,37.2115546649594,107.94258143587));
#35706=CARTESIAN_POINT('Ctrl Pts',(89.8585642450085,37.9913682749749,107.995230943601));
#35707=CARTESIAN_POINT('Ctrl Pts',(89.1547136807079,38.6186817508428,108.047880451332));
#35708=CARTESIAN_POINT('Ctrl Pts',(88.3477629366261,38.8091255628108,108.100529959063));
#35709=CARTESIAN_POINT('Ctrl Pts',(87.5408121925443,38.9995693747789,108.153179466794));
#35710=CARTESIAN_POINT('Ctrl Pts',(86.6307612686814,38.7531435228472,108.205828974524));
#35711=CARTESIAN_POINT('Ctrl Pts',(86.030161371803,38.1815548583619,108.258478482255));
#35712=CARTESIAN_POINT('Ctrl Pts',(85.5398732879433,37.7149495317159,108.301457887339));
#35713=CARTESIAN_POINT('Ctrl Pts',(85.2558020300327,37.0316571131741,108.344437292424));
#35714=CARTESIAN_POINT('Ctrl Pts',(85.249750645845,36.3528305926657,108.387416697508));
#35715=CARTESIAN_POINT('Origin',(87.7685555885722,36.3549260746835,114.));
#35716=CARTESIAN_POINT('',(85.2489004637444,36.356783832747,109.387416697508));
#35717=CARTESIAN_POINT('',(85.2539948967292,36.356454017039,109.112583302492));
#35718=CARTESIAN_POINT('',(85.2510555885723,36.3549260746835,114.));
#35719=CARTESIAN_POINT('Ctrl Pts',(85.2539948967292,36.356454017039,109.112583302492));
#35720=CARTESIAN_POINT('Ctrl Pts',(85.2522386414448,36.6697453263034,109.092832468829));
#35721=CARTESIAN_POINT('Ctrl Pts',(85.3065358325806,36.982449815841,109.073081635165));
#35722=CARTESIAN_POINT('Ctrl Pts',(85.4196754020532,37.2721759899556,109.053330801502));
#35723=CARTESIAN_POINT('Ctrl Pts',(85.7212698936659,38.0444948046395,109.000681293771));
#35724=CARTESIAN_POINT('Ctrl Pts',(86.4409911662098,38.6535325057685,108.94803178604));
#35725=CARTESIAN_POINT('Ctrl Pts',(87.2525647175344,38.8231921626186,108.89538227831));
#35726=CARTESIAN_POINT('Ctrl Pts',(88.064138268859,38.9928518194688,108.842732770579));
#35727=CARTESIAN_POINT('Ctrl Pts',(88.9675640989643,38.7231334320402,108.790083262848));
#35728=CARTESIAN_POINT('Ctrl Pts',(89.5532874509759,38.1363075713555,108.737433755117));
#35729=CARTESIAN_POINT('Ctrl Pts',(90.1390108029874,37.5494817106708,108.684784247386));
#35730=CARTESIAN_POINT('Ctrl Pts',(90.4070316769052,36.64554837673,108.632134739655));
#35731=CARTESIAN_POINT('Ctrl Pts',(90.2358476976249,35.8342964390754,108.579485231925));
#35732=CARTESIAN_POINT('Ctrl Pts',(90.0646637183446,35.0230445014207,108.526835724194));
#35733=CARTESIAN_POINT('Ctrl Pts',(89.4542748858661,34.3044739600521,108.474186216463));
#35734=CARTESIAN_POINT('Ctrl Pts',(88.6813900247885,34.00432871512,108.421536708732));
#35735=CARTESIAN_POINT('Ctrl Pts',(87.9085051637108,33.7041834701879,108.368887201001));
#35736=CARTESIAN_POINT('Ctrl Pts',(86.973124274034,33.8224635216923,108.316237693271));
#35737=CARTESIAN_POINT('Ctrl Pts',(86.2992914932937,34.3055671773523,108.26358818554));
#35738=CARTESIAN_POINT('Ctrl Pts',(85.6550813532253,34.767432914039,108.213253224524));
#35739=CARTESIAN_POINT('Ctrl Pts',(85.249928742989,35.5627509933504,108.162918263508));
#35740=CARTESIAN_POINT('Ctrl Pts',(85.2471486681112,36.3555923947772,108.112583302492));
#35741=CARTESIAN_POINT('Ctrl Pts',(85.249750645845,36.3528305926657,108.387416697508));
#35742=CARTESIAN_POINT('Ctrl Pts',(85.2483891215025,36.2000987872894,108.397086800155));
#35743=CARTESIAN_POINT('Ctrl Pts',(85.2611015862619,36.0475930556804,108.406756902801));
#35744=CARTESIAN_POINT('Ctrl Pts',(85.2887058548593,35.897832262702,108.416427005448));
#35745=CARTESIAN_POINT('Ctrl Pts',(85.4389991046876,35.0824498085661,108.469076513179));
#35746=CARTESIAN_POINT('Ctrl Pts',(86.0307344742379,34.3484363773334,108.521726020909));
#35747=CARTESIAN_POINT('Ctrl Pts',(86.7956561860184,34.0285442450444,108.57437552864));
#35748=CARTESIAN_POINT('Ctrl Pts',(87.5605778977989,33.7086521127554,108.627025036371));
#35749=CARTESIAN_POINT('Ctrl Pts',(88.4986859518095,33.8028812794101,108.679674544102));
#35750=CARTESIAN_POINT('Ctrl Pts',(89.1847040791145,34.2685151393245,108.732324051833));
#35751=CARTESIAN_POINT('Ctrl Pts',(89.8707222064195,34.734148999239,108.784973559563));
#35752=CARTESIAN_POINT('Ctrl Pts',(90.304650407019,35.5711875524131,108.837623067294));
#35753=CARTESIAN_POINT('Ctrl Pts',(90.2897735643535,36.4001717328157,108.890272575025));
#35754=CARTESIAN_POINT('Ctrl Pts',(90.2748967216881,37.2291559132183,108.942922082756));
#35755=CARTESIAN_POINT('Ctrl Pts',(89.8112148357577,38.0500857208495,108.995571590487));
#35756=CARTESIAN_POINT('Ctrl Pts',(89.1089312161219,38.4908052894037,109.048221098218));
#35757=CARTESIAN_POINT('Ctrl Pts',(88.406647596486,38.9315248579579,109.100870605948));
#35758=CARTESIAN_POINT('Ctrl Pts',(87.4657622431447,38.9920341874351,109.153520113679));
#35759=CARTESIAN_POINT('Ctrl Pts',(86.7128111367725,38.6449022068022,109.20616962141));
#35760=CARTESIAN_POINT('Ctrl Pts',(85.9598600304002,38.2977702261693,109.258819129141));
#35761=CARTESIAN_POINT('Ctrl Pts',(85.3948431709971,37.5429969354263,109.311468636872));
#35762=CARTESIAN_POINT('Ctrl Pts',(85.2739024016732,36.7227473703736,109.364118144603));
#35763=CARTESIAN_POINT('Ctrl Pts',(85.2560627609119,36.6017546095624,109.371884328904));
#35764=CARTESIAN_POINT('Ctrl Pts',(85.2478855008807,36.479337190443,109.379650513206));
#35765=CARTESIAN_POINT('Ctrl Pts',(85.2489004637444,36.356783832747,109.387416697508));
#35766=CARTESIAN_POINT('Origin',(87.7685555885722,36.3549260746835,114.));
#35767=CARTESIAN_POINT('',(85.2549713556205,36.3552114621125,110.387416697508));
#35768=CARTESIAN_POINT('',(85.2524195635058,36.3528024297952,110.112583302492));
#35769=CARTESIAN_POINT('',(85.2510555885723,36.3549260746835,114.));
#35770=CARTESIAN_POINT('Ctrl Pts',(85.2524195635058,36.3528024297952,110.112583302492));
#35771=CARTESIAN_POINT('Ctrl Pts',(85.2572190279654,36.9417394717248,110.07539618188));
#35772=CARTESIAN_POINT('Ctrl Pts',(85.4637775213495,37.5337100919753,110.038209061269));
#35773=CARTESIAN_POINT('Ctrl Pts',(85.841473043876,37.9812526944321,110.001021940657));
#35774=CARTESIAN_POINT('Ctrl Pts',(86.3762141855952,38.6148832988006,109.948372432926));
#35775=CARTESIAN_POINT('Ctrl Pts',(87.253997499495,38.9590096316741,109.895722925195));
#35776=CARTESIAN_POINT('Ctrl Pts',(88.0768932710453,38.8576272669864,109.843073417464));
#35777=CARTESIAN_POINT('Ctrl Pts',(88.8997890425955,38.7562449022988,109.790423909734));
#35778=CARTESIAN_POINT('Ctrl Pts',(89.6677972717962,38.2093538400499,109.737774402003));
#35779=CARTESIAN_POINT('Ctrl Pts',(90.0327531016733,37.4648787983024,109.685124894272));
#35780=CARTESIAN_POINT('Ctrl Pts',(90.3977089315504,36.7204037565549,109.632475386541));
#35781=CARTESIAN_POINT('Ctrl Pts',(90.359612362104,35.7783447353088,109.57982587881));
#35782=CARTESIAN_POINT('Ctrl Pts',(89.935733904506,35.0657699248179,109.52717637108));
#35783=CARTESIAN_POINT('Ctrl Pts',(89.511855446908,34.353195114327,109.474526863349));
#35784=CARTESIAN_POINT('Ctrl Pts',(88.7021951011585,33.8701045145914,109.421877355618));
#35785=CARTESIAN_POINT('Ctrl Pts',(87.8738000505619,33.8354997820466,109.369227847887));
#35786=CARTESIAN_POINT('Ctrl Pts',(87.0454049999653,33.8008950495019,109.316578340156));
#35787=CARTESIAN_POINT('Ctrl Pts',(86.1982752445215,34.214776184148,109.263928832425));
#35788=CARTESIAN_POINT('Ctrl Pts',(85.7164442221403,34.8895167155904,109.211279324695));
#35789=CARTESIAN_POINT('Ctrl Pts',(85.4153663499221,35.3111363998153,109.178380650627));
#35790=CARTESIAN_POINT('Ctrl Pts',(85.2569202654081,35.8346092763373,109.14548197656));
#35791=CARTESIAN_POINT('Ctrl Pts',(85.2539948967292,36.356454017039,109.112583302492));
#35792=CARTESIAN_POINT('Ctrl Pts',(85.2489004637444,36.356783832747,109.387416697508));
#35793=CARTESIAN_POINT('Ctrl Pts',(85.254766266655,35.6485078278274,109.432300020937));
#35794=CARTESIAN_POINT('Ctrl Pts',(85.5676580844589,34.9356913891148,109.477183344366));
#35795=CARTESIAN_POINT('Ctrl Pts',(86.0968198597103,34.467100172007,109.522066667795));
#35796=CARTESIAN_POINT('Ctrl Pts',(86.7175427663159,33.9174283780556,109.574716175526));
#35797=CARTESIAN_POINT('Ctrl Pts',(87.6358532587717,33.7038106295153,109.627365683257));
#35798=CARTESIAN_POINT('Ctrl Pts',(88.435449249828,33.9230872942025,109.680015190987));
#35799=CARTESIAN_POINT('Ctrl Pts',(89.2350452408843,34.1423639588897,109.732664698718));
#35800=CARTESIAN_POINT('Ctrl Pts',(89.915926730541,34.7945350368046,109.785314206449));
#35801=CARTESIAN_POINT('Ctrl Pts',(90.1694264446719,35.5839486823747,109.83796371418));
#35802=CARTESIAN_POINT('Ctrl Pts',(90.4229261588028,36.3733623279449,109.890613221911));
#35803=CARTESIAN_POINT('Ctrl Pts',(90.2490440974077,37.3000185411705,109.943262729642));
#35804=CARTESIAN_POINT('Ctrl Pts',(89.7266070511755,37.9438318216275,109.995912237372));
#35805=CARTESIAN_POINT('Ctrl Pts',(89.2041700049433,38.5876451020846,110.048561745103));
#35806=CARTESIAN_POINT('Ctrl Pts',(88.3331779738739,38.9486154497732,110.101211252834));
#35807=CARTESIAN_POINT('Ctrl Pts',(87.5084819490988,38.8631024456324,110.153860760565));
#35808=CARTESIAN_POINT('Ctrl Pts',(86.6837859243238,38.7775894414915,110.206510268296));
#35809=CARTESIAN_POINT('Ctrl Pts',(85.905385905843,38.2455930855212,110.259159776026));
#35810=CARTESIAN_POINT('Ctrl Pts',(85.5261577056066,37.5082858362883,110.311809283757));
#35811=CARTESIAN_POINT('Ctrl Pts',(85.3446272749214,37.1553487329371,110.337011755008));
#35812=CARTESIAN_POINT('Ctrl Pts',(85.2545623833254,36.7553670470907,110.362214226258));
#35813=CARTESIAN_POINT('Ctrl Pts',(85.2549713556205,36.3552114621125,110.387416697508));
#35814=CARTESIAN_POINT('Origin',(87.7685555885722,36.3549260746835,114.));
#35815=CARTESIAN_POINT('',(85.2499086688349,36.3527998632167,111.387416697508));
#35816=CARTESIAN_POINT('',(85.2470898693037,36.3554869991381,111.112583302492));
#35817=CARTESIAN_POINT('',(85.2510555885723,36.3549260746835,114.));
#35818=CARTESIAN_POINT('Ctrl Pts',(85.2470898693037,36.3554869991381,111.112583302492));
#35819=CARTESIAN_POINT('Ctrl Pts',(85.2469951454703,36.3865769470086,111.110609402663));
#35820=CARTESIAN_POINT('Ctrl Pts',(85.2475209470525,36.4176636173667,111.108635502833));
#35821=CARTESIAN_POINT('Ctrl Pts',(85.2486772533794,36.448726817618,111.106661603004));
#35822=CARTESIAN_POINT('Ctrl Pts',(85.2795192231668,37.2772704840766,111.054012095273));
#35823=CARTESIAN_POINT('Ctrl Pts',(85.75892762442,38.0891165727784,111.001362587543));
#35824=CARTESIAN_POINT('Ctrl Pts',(86.4695699486882,38.5162270049124,110.948713079812));
#35825=CARTESIAN_POINT('Ctrl Pts',(87.1802122729565,38.9433374370465,110.896063572081));
#35826=CARTESIAN_POINT('Ctrl Pts',(88.1220885202398,38.9857122126128,110.84341406435));
#35827=CARTESIAN_POINT('Ctrl Pts',(88.8682134168015,38.6241413716773,110.790764556619));
#35828=CARTESIAN_POINT('Ctrl Pts',(89.6143383133631,38.2625705307417,110.738115048888));
#35829=CARTESIAN_POINT('Ctrl Pts',(90.1647118592032,37.4970540733041,110.685465541158));
#35830=CARTESIAN_POINT('Ctrl Pts',(90.2698305766733,36.6746272439013,110.632816033427));
#35831=CARTESIAN_POINT('Ctrl Pts',(90.3749492941434,35.8522004144985,110.580166525696));
#35832=CARTESIAN_POINT('Ctrl Pts',(90.0348131832435,34.9728632131304,110.527517017965));
#35833=CARTESIAN_POINT('Ctrl Pts',(89.4036177776061,34.4352497888972,110.474867510234));
#35834=CARTESIAN_POINT('Ctrl Pts',(88.7724223719687,33.8976363646639,110.422218002503));
#35835=CARTESIAN_POINT('Ctrl Pts',(87.8501676715938,33.7017467175656,110.369568494773));
#35836=CARTESIAN_POINT('Ctrl Pts',(87.0549438200498,33.9363844386613,110.316918987042));
#35837=CARTESIAN_POINT('Ctrl Pts',(86.2597199685058,34.171022159757,110.264269479311));
#35838=CARTESIAN_POINT('Ctrl Pts',(85.5915269657928,34.8361872490467,110.21161997158));
#35839=CARTESIAN_POINT('Ctrl Pts',(85.3532799492055,35.6303372316234,110.158970463849));
#35840=CARTESIAN_POINT('Ctrl Pts',(85.2833102997403,35.8635674172505,110.14350807673));
#35841=CARTESIAN_POINT('Ctrl Pts',(85.250423948459,36.107922686989,110.128045689611));
#35842=CARTESIAN_POINT('Ctrl Pts',(85.2524195635058,36.3528024297952,110.112583302492));
#35843=CARTESIAN_POINT('Ctrl Pts',(85.2549713556205,36.3552114621125,110.387416697508));
#35844=CARTESIAN_POINT('Ctrl Pts',(85.2554167515259,35.9194174945387,110.414863733989));
#35845=CARTESIAN_POINT('Ctrl Pts',(85.3631690851555,35.4834172731087,110.442310770469));
#35846=CARTESIAN_POINT('Ctrl Pts',(85.576947423415,35.107753009214,110.46975780695));
#35847=CARTESIAN_POINT('Ctrl Pts',(85.9870217234522,34.3871455738681,110.522407314681));
#35848=CARTESIAN_POINT('Ctrl Pts',(86.787226705519,33.8885488456719,110.575056822411));
#35849=CARTESIAN_POINT('Ctrl Pts',(87.6148016096937,33.8379940694177,110.627706330142));
#35850=CARTESIAN_POINT('Ctrl Pts',(88.4423765138683,33.7874392931636,110.680355837873));
#35851=CARTESIAN_POINT('Ctrl Pts',(89.2973213401509,34.1849264688513,110.733005345604));
#35852=CARTESIAN_POINT('Ctrl Pts',(89.7920598524681,34.8502608298321,110.785654853335));
#35853=CARTESIAN_POINT('Ctrl Pts',(90.2867983647854,35.5155951908128,110.838304361066));
#35854=CARTESIAN_POINT('Ctrl Pts',(90.4213305631374,36.4487767370866,110.890953868796));
#35855=CARTESIAN_POINT('Ctrl Pts',(90.1346683212381,37.226761805398,110.943603376527));
#35856=CARTESIAN_POINT('Ctrl Pts',(89.8480060793388,38.0047468737095,110.996252884258));
#35857=CARTESIAN_POINT('Ctrl Pts',(89.1401493971882,38.6275354640587,111.048902391989));
#35858=CARTESIAN_POINT('Ctrl Pts',(88.3319943373804,38.812795839625,111.10155189972));
#35859=CARTESIAN_POINT('Ctrl Pts',(87.5238392775726,38.9980562151914,111.15420140745));
#35860=CARTESIAN_POINT('Ctrl Pts',(86.6153858401076,38.745788375975,111.206850915181));
#35861=CARTESIAN_POINT('Ctrl Pts',(86.0184675761862,38.1703541107022,111.259500422912));
#35862=CARTESIAN_POINT('Ctrl Pts',(85.5350470350138,37.704332612047,111.302139181111));
#35863=CARTESIAN_POINT('Ctrl Pts',(85.2559543382204,37.0263546320076,111.344777939309));
#35864=CARTESIAN_POINT('Ctrl Pts',(85.2499086688349,36.3527998632167,111.387416697508));
#35865=CARTESIAN_POINT('Origin',(87.7685555885722,36.3549260746835,114.));
#35866=CARTESIAN_POINT('',(85.2487564810892,36.3567299719253,112.387416697508));
#35867=CARTESIAN_POINT('',(85.2538919790663,36.3565168098445,112.112583302492));
#35868=CARTESIAN_POINT('',(85.2510555885723,36.3549260746835,114.));
#35869=CARTESIAN_POINT('Ctrl Pts',(85.2538919790663,36.3565168098445,112.112583302492));
#35870=CARTESIAN_POINT('Ctrl Pts',(85.2520902264104,36.6643730249807,112.093173115714));
#35871=CARTESIAN_POINT('Ctrl Pts',(85.3044764405676,36.9716374584574,112.073762928937));
#35872=CARTESIAN_POINT('Ctrl Pts',(85.4138341392615,37.2570747873116,112.054352742159));
#35873=CARTESIAN_POINT('Ctrl Pts',(85.710463381873,38.0313143669871,112.001703234428));
#35874=CARTESIAN_POINT('Ctrl Pts',(86.4262592893377,38.6449614200248,111.949053726697));
#35875=CARTESIAN_POINT('Ctrl Pts',(87.2367266719805,38.8198283865448,111.896404218967));
#35876=CARTESIAN_POINT('Ctrl Pts',(88.0471940546233,38.9946953530647,111.843754711236));
#35877=CARTESIAN_POINT('Ctrl Pts',(88.9523329124443,38.7307822330669,111.791105203505));
#35878=CARTESIAN_POINT('Ctrl Pts',(89.5418123085277,38.1477300262273,111.738455695774));
#35879=CARTESIAN_POINT('Ctrl Pts',(90.1312917046111,37.5646778193877,111.685806188043));
#35880=CARTESIAN_POINT('Ctrl Pts',(90.4051116389569,36.6624865257063,111.633156680312));
#35881=CARTESIAN_POINT('Ctrl Pts',(90.239140008257,35.8501508487148,111.580507172582));
#35882=CARTESIAN_POINT('Ctrl Pts',(90.073168377557,35.0378151717233,111.527857664851));
#35883=CARTESIAN_POINT('Ctrl Pts',(89.4674051818114,34.3153351114216,111.47520815712));
#35884=CARTESIAN_POINT('Ctrl Pts',(88.6964639540858,34.0102360165388,111.422558649389));
#35885=CARTESIAN_POINT('Ctrl Pts',(87.9255227263601,33.705136921656,111.369909141658));
#35886=CARTESIAN_POINT('Ctrl Pts',(86.9894034666545,33.8174187921922,111.317259633927));
#35887=CARTESIAN_POINT('Ctrl Pts',(86.3124816059625,34.296180349568,111.264610126197));
#35888=CARTESIAN_POINT('Ctrl Pts',(85.660938443056,34.7569925015818,111.213934518295));
#35889=CARTESIAN_POINT('Ctrl Pts',(85.2495216988075,35.5573198456716,111.163258910394));
#35890=CARTESIAN_POINT('Ctrl Pts',(85.2470898693037,36.3554869991381,111.112583302492));
#35891=CARTESIAN_POINT('Ctrl Pts',(85.2499086688349,36.3527998632167,111.387416697508));
#35892=CARTESIAN_POINT('Ctrl Pts',(85.248489263474,36.19466232893,111.39742744704));
#35893=CARTESIAN_POINT('Ctrl Pts',(85.2621207261532,36.0367686104045,111.407438196572));
#35894=CARTESIAN_POINT('Ctrl Pts',(85.291692389305,35.8819189952726,111.417448946105));
#35895=CARTESIAN_POINT('Ctrl Pts',(85.4472185567229,35.0675188364451,111.470098453835));
#35896=CARTESIAN_POINT('Ctrl Pts',(86.0436539819365,34.3373192101194,111.522747961566));
#35897=CARTESIAN_POINT('Ctrl Pts',(86.8106137348087,34.0223450128831,111.575397469297));
#35898=CARTESIAN_POINT('Ctrl Pts',(87.5775734876809,33.7073708156469,111.628046977028));
#35899=CARTESIAN_POINT('Ctrl Pts',(88.5150575682117,33.8076220475,111.680696484759));
#35900=CARTESIAN_POINT('Ctrl Pts',(89.1980718246363,34.2776513369828,111.73334599249));
#35901=CARTESIAN_POINT('Ctrl Pts',(89.8810860810608,34.7476806264656,111.78599550022));
#35902=CARTESIAN_POINT('Ctrl Pts',(90.3096305133791,35.587487973578,111.838645007951));
#35903=CARTESIAN_POINT('Ctrl Pts',(90.2894310199951,36.4163594883,111.891294515682));
#35904=CARTESIAN_POINT('Ctrl Pts',(90.2692315266111,37.245231003022,111.943944023413));
#35905=CARTESIAN_POINT('Ctrl Pts',(89.8002881075246,38.0631666853536,111.996593531144));
#35906=CARTESIAN_POINT('Ctrl Pts',(89.0951891306436,38.4993678319042,112.049243038874));
#35907=CARTESIAN_POINT('Ctrl Pts',(88.3900901537627,38.9355689784547,112.101892546605));
#35908=CARTESIAN_POINT('Ctrl Pts',(87.4488356190872,38.9900355892243,112.154542054336));
#35909=CARTESIAN_POINT('Ctrl Pts',(86.6981289564312,38.6380760544841,112.207191562067));
#35910=CARTESIAN_POINT('Ctrl Pts',(85.9474222937752,38.2861165197439,112.259841069798));
#35911=CARTESIAN_POINT('Ctrl Pts',(85.3872635031387,37.527730839494,112.312490577529));
#35912=CARTESIAN_POINT('Ctrl Pts',(85.2715920540268,36.7067216292466,112.365140085259));
#35913=CARTESIAN_POINT('Ctrl Pts',(85.2552780805371,36.5909288161227,112.372565622676));
#35914=CARTESIAN_POINT('Ctrl Pts',(85.2478056192164,36.4738903281486,112.379991160092));
#35915=CARTESIAN_POINT('Ctrl Pts',(85.2487564810892,36.3567299719253,112.387416697508));
#35916=CARTESIAN_POINT('Origin',(87.7685555885722,36.3549260746835,114.));
#35917=CARTESIAN_POINT('',(85.2549501597152,36.3552974008805,113.387416697508));
#35918=CARTESIAN_POINT('',(85.2525638004967,36.3528324581658,113.112583302492));
#35919=CARTESIAN_POINT('',(85.2510555885723,36.3549260746835,114.));
#35920=CARTESIAN_POINT('Ctrl Pts',(85.2525638004967,36.3528324581658,113.112583302492));
#35921=CARTESIAN_POINT('Ctrl Pts',(85.2572318872201,36.9364594446687,113.075736828766));
#35922=CARTESIAN_POINT('Ctrl Pts',(85.4596894895625,37.523008588093,113.03889035504));
#35923=CARTESIAN_POINT('Ctrl Pts',(85.8310701294007,37.9688453722444,113.002043881314));
#35924=CARTESIAN_POINT('Ctrl Pts',(86.3617317067771,38.6058964884073,112.949394373583));
#35925=CARTESIAN_POINT('Ctrl Pts',(87.2372872920457,38.9556519800712,112.896744865852));
#35926=CARTESIAN_POINT('Ctrl Pts',(88.0608170750347,38.8595555137566,112.844095358121));
#35927=CARTESIAN_POINT('Ctrl Pts',(88.8843468580237,38.7634590474419,112.79144585039));
#35928=CARTESIAN_POINT('Ctrl Pts',(89.655850838733,38.2215106231487,112.73879634266));
#35929=CARTESIAN_POINT('Ctrl Pts',(90.0255794196246,37.4793943177222,112.686146834929));
#35930=CARTESIAN_POINT('Ctrl Pts',(90.3953080005161,36.7372780122957,112.633497327198));
#35931=CARTESIAN_POINT('Ctrl Pts',(90.3632611815899,35.7949938257358,112.580847819467));
#35932=CARTESIAN_POINT('Ctrl Pts',(89.9439669008761,35.0797119648804,112.528198311736));
#35933=CARTESIAN_POINT('Ctrl Pts',(89.5246726201623,34.364430104025,112.475548804006));
#35934=CARTESIAN_POINT('Ctrl Pts',(88.7181308776611,33.8761505688741,112.422899296275));
#35935=CARTESIAN_POINT('Ctrl Pts',(87.8899751074061,33.836227461513,112.370249788544));
#35936=CARTESIAN_POINT('Ctrl Pts',(87.061819337151,33.796304354152,112.317600280813));
#35937=CARTESIAN_POINT('Ctrl Pts',(86.2120495391423,34.2047376745809,112.264950773082));
#35938=CARTESIAN_POINT('Ctrl Pts',(85.7258959290171,34.8763703879519,112.212301265351));
#35939=CARTESIAN_POINT('Ctrl Pts',(85.4189715801305,35.3003936368778,112.179061944398));
#35940=CARTESIAN_POINT('Ctrl Pts',(85.2569774225757,35.8293229368779,112.145822623445));
#35941=CARTESIAN_POINT('Ctrl Pts',(85.2538919790663,36.3565168098445,112.112583302492));
#35942=CARTESIAN_POINT('Ctrl Pts',(85.2487564810892,36.3567299719253,112.387416697508));
#35943=CARTESIAN_POINT('Ctrl Pts',(85.2545475432976,35.6431847865861,112.432640667823));
#35944=CARTESIAN_POINT('Ctrl Pts',(85.5727774749206,34.9251192501781,112.477864638137));
#35945=CARTESIAN_POINT('Ctrl Pts',(86.1089760466816,34.4564048740649,112.523088608452));
#35946=CARTESIAN_POINT('Ctrl Pts',(86.7332155960355,33.9107300693753,112.575738116183));
#35947=CARTESIAN_POINT('Ctrl Pts',(87.6528788023304,33.7030132002407,112.628387623914));
#35948=CARTESIAN_POINT('Ctrl Pts',(88.4510503361386,33.9274195505719,112.681037131644));
#35949=CARTESIAN_POINT('Ctrl Pts',(89.2492218699467,34.1518259009031,112.733686639375));
#35950=CARTESIAN_POINT('Ctrl Pts',(89.9259017312681,34.8083554706999,112.786336147106));
#35951=CARTESIAN_POINT('Ctrl Pts',(90.1743273951165,35.5993805632173,112.838985654837));
#35952=CARTESIAN_POINT('Ctrl Pts',(90.422753058965,36.3904056557346,112.891635162568));
#35953=CARTESIAN_POINT('Ctrl Pts',(90.2429245253405,37.3159262709724,112.944284670298));
#35954=CARTESIAN_POINT('Ctrl Pts',(89.7163643253429,37.9563717122312,112.996934178029));
#35955=CARTESIAN_POINT('Ctrl Pts',(89.1898041253453,38.5968171534899,113.04958368576));
#35956=CARTESIAN_POINT('Ctrl Pts',(88.3165122589745,38.9521874207695,113.102233193491));
#35957=CARTESIAN_POINT('Ctrl Pts',(87.4923823138641,38.8613808074479,113.154882701222));
#35958=CARTESIAN_POINT('Ctrl Pts',(86.6682523687537,38.7705741941264,113.207532208953));
#35959=CARTESIAN_POINT('Ctrl Pts',(85.8932843449036,38.2335907002035,113.260181716683));
#35960=CARTESIAN_POINT('Ctrl Pts',(85.5187982111328,37.493863626842,113.312831224414));
#35961=CARTESIAN_POINT('Ctrl Pts',(85.3419606890729,37.1445542910419,113.337693048779));
#35962=CARTESIAN_POINT('Ctrl Pts',(85.2544249726597,36.7500360002912,113.362554873143));
#35963=CARTESIAN_POINT('Ctrl Pts',(85.2549501597152,36.3552974008805,113.387416697508));
#35964=CARTESIAN_POINT('Origin',(87.7685555885722,36.3549260746835,114.));
#35965=CARTESIAN_POINT('',(85.2500677241434,36.352772713106,114.387416697508));
#35966=CARTESIAN_POINT('',(85.2470413488897,36.3553920695512,114.112583302492));
#35967=CARTESIAN_POINT('',(85.2510555885723,36.3549260746835,114.));
#35968=CARTESIAN_POINT('Ctrl Pts',(85.2470413488897,36.3553920695512,114.112583302492));
#35969=CARTESIAN_POINT('Ctrl Pts',(85.246975261324,36.3811153243067,114.110950049548));
#35970=CARTESIAN_POINT('Ctrl Pts',(85.2473352048204,36.406836684913,114.109316796605));
#35971=CARTESIAN_POINT('Ctrl Pts',(85.2481269058065,36.4325447491923,114.107683543661));
#35972=CARTESIAN_POINT('Ctrl Pts',(85.2736481622355,37.2612693715961,114.05503403593));
#35973=CARTESIAN_POINT('Ctrl Pts',(85.7478338181264,38.0761770047617,114.002384528199));
#35974=CARTESIAN_POINT('Ctrl Pts',(86.4557190172335,38.507841665341,113.949735020469));
#35975=CARTESIAN_POINT('Ctrl Pts',(87.1636042163406,38.9395063259204,113.897085512738));
#35976=CARTESIAN_POINT('Ctrl Pts',(88.105188958664,38.9879280139136,113.844436005007));
#35977=CARTESIAN_POINT('Ctrl Pts',(88.853620119774,38.6311554934084,113.791786497276));
#35978=CARTESIAN_POINT('Ctrl Pts',(89.6020512808839,38.2743829729033,113.739136989545));
#35979=CARTESIAN_POINT('Ctrl Pts',(90.1573288607805,37.5124162438998,113.686487481815));
#35980=CARTESIAN_POINT('Ctrl Pts',(90.2677262126197,36.6906813359064,113.633837974084));
#35981=CARTESIAN_POINT('Ctrl Pts',(90.3781235644589,35.868946427913,113.581188466353));
#35982=CARTESIAN_POINT('Ctrl Pts',(90.0436406882408,34.9874433409297,113.528538958622));
#35983=CARTESIAN_POINT('Ctrl Pts',(89.4159103094804,34.4457880945882,113.475889450891));
#35984=CARTESIAN_POINT('Ctrl Pts',(88.7881799307199,33.9041328482467,113.42323994316));
#35985=CARTESIAN_POINT('Ctrl Pts',(87.867202049417,33.7023254425469,113.37059043543));
#35986=CARTESIAN_POINT('Ctrl Pts',(87.0704879829226,33.9318521960155,113.317940927699));
#35987=CARTESIAN_POINT('Ctrl Pts',(86.2737739164281,34.1613789494841,113.265291419968));
#35988=CARTESIAN_POINT('Ctrl Pts',(85.6013236647419,34.822239862121,113.212641912237));
#35989=CARTESIAN_POINT('Ctrl Pts',(85.357982323641,35.6148436887704,113.159992404506));
#35990=CARTESIAN_POINT('Ctrl Pts',(85.2849421062881,35.8527480066772,113.144189370502));
#35991=CARTESIAN_POINT('Ctrl Pts',(85.2505617111305,36.1025214736639,113.128386336497));
#35992=CARTESIAN_POINT('Ctrl Pts',(85.2525638004967,36.3528324581658,113.112583302492));
#35993=CARTESIAN_POINT('Ctrl Pts',(85.2549501597152,36.3552974008805,113.387416697508));
#35994=CARTESIAN_POINT('Ctrl Pts',(85.2555371533079,35.914104065589,113.415204380874));
#35995=CARTESIAN_POINT('Ctrl Pts',(85.366131529534,35.4726355164613,113.44299206424));
#35996=CARTESIAN_POINT('Ctrl Pts',(85.5850006992482,35.0937064069138,113.470779747607));
#35997=CARTESIAN_POINT('Ctrl Pts',(85.999693564826,34.3757469131473,113.523429255337));
#35998=CARTESIAN_POINT('Ctrl Pts',(86.8030835396733,33.8822985784145,113.576078763068));
#35999=CARTESIAN_POINT('Ctrl Pts',(87.6309659956938,33.8370587014901,113.628728270799));
#36000=CARTESIAN_POINT('Ctrl Pts',(88.4588484517142,33.7918188245658,113.68137777853));
#36001=CARTESIAN_POINT('Ctrl Pts',(89.3112233889079,34.1947874054499,113.734027286261));
#36002=CARTESIAN_POINT('Ctrl Pts',(89.801679591404,34.8632847658664,113.786676793992));
#36003=CARTESIAN_POINT('Ctrl Pts',(90.2921357939,35.5317821262828,113.839326301722));
#36004=CARTESIAN_POINT('Ctrl Pts',(90.4206732616985,36.4658082662316,113.891975809453));
#36005=CARTESIAN_POINT('Ctrl Pts',(90.129021488418,37.2419366387274,113.944625317184));
#36006=CARTESIAN_POINT('Ctrl Pts',(89.8373697151376,38.0180650112232,113.997274824915));
#36007=CARTESIAN_POINT('Ctrl Pts',(89.1255287007783,38.6362956162661,114.049924332646));
#36008=CARTESIAN_POINT('Ctrl Pts',(88.3162007443671,38.8163630103767,114.102573840377));
#36009=CARTESIAN_POINT('Ctrl Pts',(87.5068727879558,38.9964304044874,114.155223348107));
#36010=CARTESIAN_POINT('Ctrl Pts',(86.6000578894926,38.7383345876658,114.207872855838));
#36011=CARTESIAN_POINT('Ctrl Pts',(86.0068467934315,38.1590793736534,114.260522363569));
#36012=CARTESIAN_POINT('Ctrl Pts',(85.5302666684741,37.6937112709506,114.302820474882));
#36013=CARTESIAN_POINT('Ctrl Pts',(85.2560977910143,37.0210552663375,114.345118586195));
#36014=CARTESIAN_POINT('Ctrl Pts',(85.2500677241434,36.352772713106,114.387416697508));
#36015=CARTESIAN_POINT('Origin',(87.7685555885722,36.3549260746835,114.));
#36016=CARTESIAN_POINT('',(85.2486156762139,36.3566728107829,115.387416697508));
#36017=CARTESIAN_POINT('',(85.2537847572937,36.3565773825072,115.112583302492));
#36018=CARTESIAN_POINT('',(85.2510555885723,36.3549260746835,114.));
#36019=CARTESIAN_POINT('Ctrl Pts',(85.2537847572937,36.3565773825072,115.112583302492));
#36020=CARTESIAN_POINT('Ctrl Pts',(85.2519421925275,36.6589983217697,115.0935137626));
#36021=CARTESIAN_POINT('Ctrl Pts',(85.30245434637,36.9608245141166,115.074444222708));
#36022=CARTESIAN_POINT('Ctrl Pts',(85.4080899859888,37.2419365270239,115.055374682816));
#36023=CARTESIAN_POINT('Ctrl Pts',(85.6997417225407,38.0180648017789,115.002725175085));
#36024=CARTESIAN_POINT('Ctrl Pts',(86.4115826472556,38.6362953289655,114.950075667354));
#36025=CARTESIAN_POINT('Ctrl Pts',(87.2209105017453,38.8163627003993,114.897426159623));
#36026=CARTESIAN_POINT('Ctrl Pts',(88.030238356235,38.9964300718331,114.844776651893));
#36027=CARTESIAN_POINT('Ctrl Pts',(88.9370531404997,38.7383342875141,114.792127144162));
#36028=CARTESIAN_POINT('Ctrl Pts',(89.5302641618553,38.1590791464492,114.739477636431));
#36029=CARTESIAN_POINT('Ctrl Pts',(90.123475183211,37.5798240053843,114.6868281287));
#36030=CARTESIAN_POINT('Ctrl Pts',(90.4030824416578,36.6794095075733,114.634178620969));
#36031=CARTESIAN_POINT('Ctrl Pts',(90.2423302385139,35.8660248731645,114.581529113238));
#36032=CARTESIAN_POINT('Ctrl Pts',(90.0815780353701,35.0526402387556,114.528879605508));
#36033=CARTESIAN_POINT('Ctrl Pts',(89.4804663706356,34.3262854677489,114.476230097777));
#36034=CARTESIAN_POINT('Ctrl Pts',(88.7115000765254,34.0162424500392,114.423580590046));
#36035=CARTESIAN_POINT('Ctrl Pts',(87.9425337824152,33.7061994323295,114.370931082315));
#36036=CARTESIAN_POINT('Ctrl Pts',(87.0057128589294,33.812468167917,114.318281574584));
#36037=CARTESIAN_POINT('Ctrl Pts',(86.3257308256699,34.2868733415318,114.265632066854));
#36038=CARTESIAN_POINT('Ctrl Pts',(85.6668426773359,34.7465618790433,114.214615812066));
#36039=CARTESIAN_POINT('Ctrl Pts',(85.24910565871,35.5519010220325,114.163599557279));
#36040=CARTESIAN_POINT('Ctrl Pts',(85.2470413488897,36.3553920695512,114.112583302492));
#36041=CARTESIAN_POINT('Ctrl Pts',(85.2500677241434,36.352772713106,114.387416697508));
#36042=CARTESIAN_POINT('Ctrl Pts',(85.2485920172934,36.189227405458,114.397768093926));
#36043=CARTESIAN_POINT('Ctrl Pts',(85.2631752035907,36.0259440247882,114.408119490344));
#36044=CARTESIAN_POINT('Ctrl Pts',(85.294780627099,35.8660248115963,114.418470886761));
#36045=CARTESIAN_POINT('Ctrl Pts',(85.4555328504867,35.0526400747549,114.471120394492));
#36046=CARTESIAN_POINT('Ctrl Pts',(86.0566445909211,34.3262852122755,114.523769902223));
#36047=CARTESIAN_POINT('Ctrl Pts',(86.8256109818699,34.0162421555207,114.576419409954));
#36048=CARTESIAN_POINT('Ctrl Pts',(87.5945773728186,33.7061990987659,114.629068917685));
#36049=CARTESIAN_POINT('Ctrl Pts',(88.5313984142817,33.8124678477358,114.681718425416));
#36050=CARTESIAN_POINT('Ctrl Pts',(89.2113805331739,34.2868730810938,114.734367933146));
#36051=CARTESIAN_POINT('Ctrl Pts',(89.8913626520661,34.7612783144519,114.787017440877));
#36052=CARTESIAN_POINT('Ctrl Pts',(90.3145058483874,35.6038200321981,114.839666948608));
#36053=CARTESIAN_POINT('Ctrl Pts',(90.2889845887447,36.4325447589662,114.892316456339));
#36054=CARTESIAN_POINT('Ctrl Pts',(90.2634633291021,37.2612694857343,114.94496596407));
#36055=CARTESIAN_POINT('Ctrl Pts',(89.7892776134956,38.0761772215243,114.997615471801));
#36056=CARTESIAN_POINT('Ctrl Pts',(89.0813923252421,38.507841936465,115.050264979531));
#36057=CARTESIAN_POINT('Ctrl Pts',(88.3735070369886,38.9395066514057,115.102914487262));
#36058=CARTESIAN_POINT('Ctrl Pts',(87.4319221760881,38.9879283454972,115.155563994993));
#36059=CARTESIAN_POINT('Ctrl Pts',(86.6834909207253,38.6311557800627,115.208213502724));
#36060=CARTESIAN_POINT('Ctrl Pts',(85.9350596653626,38.2743832146282,115.260863010455));
#36061=CARTESIAN_POINT('Ctrl Pts',(85.3797820155375,37.5124163896676,115.313512518185));
#36062=CARTESIAN_POINT('Ctrl Pts',(85.2693846497952,36.6906813781902,115.366162025916));
#36063=CARTESIAN_POINT('Ctrl Pts',(85.2545287986229,36.5801028969778,115.373246916447));
#36064=CARTESIAN_POINT('Ctrl Pts',(85.2477289726895,36.4684421155685,115.380331806977));
#36065=CARTESIAN_POINT('Ctrl Pts',(85.2486156762139,36.3566728107829,115.387416697508));
#36066=CARTESIAN_POINT('Origin',(87.7685555885722,36.3549260746835,114.));
#36067=CARTESIAN_POINT('',(85.2549234205521,36.3553827989325,116.387416697508));
#36068=CARTESIAN_POINT('',(85.2527053287706,36.35286573419,116.112583302492));
#36069=CARTESIAN_POINT('',(85.2510555885723,36.3549260746835,114.));
#36070=CARTESIAN_POINT('Ctrl Pts',(85.2527053287706,36.35286573419,116.112583302492));
#36071=CARTESIAN_POINT('Ctrl Pts',(85.2572378873775,36.9311794633336,116.076077475652));
#36072=CARTESIAN_POINT('Ctrl Pts',(85.455643720258,37.5123030198393,116.039571648811));
#36073=CARTESIAN_POINT('Ctrl Pts',(85.8207470970968,37.9563715105561,116.003065821971));
#36074=CARTESIAN_POINT('Ctrl Pts',(86.3473072307831,38.596816871161,115.95041631424));
#36075=CARTESIAN_POINT('Ctrl Pts',(87.2205989871771,38.9521870936872,115.897766806509));
#36076=CARTESIAN_POINT('Ctrl Pts',(88.0447288285018,38.861380491801,115.845117298778));
#36077=CARTESIAN_POINT('Ctrl Pts',(88.8688586698266,38.7705738899147,115.792467791047));
#36078=CARTESIAN_POINT('Ctrl Pts',(89.6438265960819,38.2335904636158,115.739818283317));
#36079=CARTESIAN_POINT('Ctrl Pts',(90.0183126826921,37.4938634834107,115.687168775586));
#36080=CARTESIAN_POINT('Ctrl Pts',(90.3927987693023,36.7541365032055,115.634519267855));
#36081=CARTESIAN_POINT('Ctrl Pts',(90.3668030162672,35.8116659690941,115.581869760124));
#36082=CARTESIAN_POINT('Ctrl Pts',(89.9521102029129,35.093706565743,115.529220252393));
#36083=CARTESIAN_POINT('Ctrl Pts',(89.5374173895586,34.3757471623918,115.476570744662));
#36084=CARTESIAN_POINT('Ctrl Pts',(88.7340275158849,33.8822988898011,115.423921236932));
#36085=CARTESIAN_POINT('Ctrl Pts',(87.9061451641227,33.8370590185742,115.371271729201));
#36086=CARTESIAN_POINT('Ctrl Pts',(87.0782628123604,33.7918191473474,115.31862222147));
#36087=CARTESIAN_POINT('Ctrl Pts',(86.2258879825096,34.1947876774846,115.265972713739));
#36088=CARTESIAN_POINT('Ctrl Pts',(85.7354318417787,34.8632849537149,115.213323206008));
#36089=CARTESIAN_POINT('Ctrl Pts',(85.4226178736733,35.2896539361353,115.17974323817));
#36090=CARTESIAN_POINT('Ctrl Pts',(85.2570293696933,35.8240377684581,115.146163270331));
#36091=CARTESIAN_POINT('Ctrl Pts',(85.2537847572937,36.3565773825072,115.112583302492));
#36092=CARTESIAN_POINT('Ctrl Pts',(85.2486156762139,36.3566728107829,115.387416697508));
#36093=CARTESIAN_POINT('Ctrl Pts',(85.254318277614,35.6378578107033,115.432981314708));
#36094=CARTESIAN_POINT('Ctrl Pts',(85.577942057269,34.9145541945511,115.478545931909));
#36095=CARTESIAN_POINT('Ctrl Pts',(86.1212006602061,34.4457878541641,115.524110549109));
#36096=CARTESIAN_POINT('Ctrl Pts',(86.7489311180187,33.9041325396098,115.57676005684));
#36097=CARTESIAN_POINT('Ctrl Pts',(87.6699091153034,33.7023251084953,115.62940956457));
#36098=CARTESIAN_POINT('Ctrl Pts',(88.4666232821311,33.9318518908688,115.682059072301));
#36099=CARTESIAN_POINT('Ctrl Pts',(89.2633374489588,34.1613786732422,115.734708580032));
#36100=CARTESIAN_POINT('Ctrl Pts',(89.9357877853295,34.8222396691035,115.787358087763));
#36101=CARTESIAN_POINT('Ctrl Pts',(90.1791291570756,35.6148435955682,115.840007595494));
#36102=CARTESIAN_POINT('Ctrl Pts',(90.4224705288217,36.407447522033,115.892657103225));
#36103=CARTESIAN_POINT('Ctrl Pts',(90.2367029359434,37.3317943791011,115.945306610955));
#36104=CARTESIAN_POINT('Ctrl Pts',(89.706041291739,37.9688455754904,115.997956118686));
#36105=CARTESIAN_POINT('Ctrl Pts',(89.1753796475346,38.6058967718796,116.050605626417));
#36106=CARTESIAN_POINT('Ctrl Pts',(88.2998239520043,38.9556523075899,116.103255134148));
#36107=CARTESIAN_POINT('Ctrl Pts',(87.4762940653052,38.8595558291738,116.155904641879));
#36108=CARTESIAN_POINT('Ctrl Pts',(86.6527641786061,38.7634593507577,116.20855414961));
#36109=CARTESIAN_POINT('Ctrl Pts',(85.8812601007382,38.2215108582152,116.26120365734));
#36110=CARTESIAN_POINT('Ctrl Pts',(85.5115314732851,37.4793944593314,116.313853165071));
#36111=CARTESIAN_POINT('Ctrl Pts',(85.3393326877013,37.1337584085611,116.33837434255));
#36112=CARTESIAN_POINT('Ctrl Pts',(85.2542859121947,36.7447024938529,116.362895520029));
#36113=CARTESIAN_POINT('Ctrl Pts',(85.2549234205521,36.3553827989325,116.387416697508));
#36114=CARTESIAN_POINT('Origin',(87.7685555885722,36.3549260746835,114.));
#36115=CARTESIAN_POINT('',(85.2502276147452,36.3527492241744,117.387416697508));
#36116=CARTESIAN_POINT('',(85.2470012906549,36.3552960959922,117.112583302492));
#36117=CARTESIAN_POINT('',(85.2510555885723,36.3549260746835,114.));
#36118=CARTESIAN_POINT('Ctrl Pts',(85.2470012906549,36.3552960959922,117.112583302492));
#36119=CARTESIAN_POINT('Ctrl Pts',(85.2469591175104,36.3756533932096,117.111290696434));
#36120=CARTESIAN_POINT('Ctrl Pts',(85.2471845538459,36.3960097327226,117.109998090376));
#36121=CARTESIAN_POINT('Ctrl Pts',(85.2476804746124,36.4163594805645,117.108705484318));
#36122=CARTESIAN_POINT('Ctrl Pts',(85.2678799654529,37.2452308909037,117.056055976587));
#36123=CARTESIAN_POINT('Ctrl Pts',(85.736823325484,38.0631664702294,117.003406468856));
#36124=CARTESIAN_POINT('Ctrl Pts',(86.4419222135695,38.4993675618474,116.950756961125));
#36125=CARTESIAN_POINT('Ctrl Pts',(87.1470211016549,38.9355686534653,116.898107453395));
#36126=CARTESIAN_POINT('Ctrl Pts',(88.0882755177948,38.9900352573753,116.845457945664));
#36127=CARTESIAN_POINT('Ctrl Pts',(88.8389820859114,38.6380757669584,116.792808437933));
#36128=CARTESIAN_POINT('Ctrl Pts',(89.5896886540281,38.2861162765415,116.740158930202));
#36129=CARTESIAN_POINT('Ctrl Pts',(90.1498473741216,37.5277306917976,116.687509422471));
#36130=CARTESIAN_POINT('Ctrl Pts',(90.2655188086662,36.7067215849428,116.634859914741));
#36131=CARTESIAN_POINT('Ctrl Pts',(90.3811902432109,35.8857124780881,116.58221040701));
#36132=CARTESIAN_POINT('Ctrl Pts',(90.0523743922067,35.0020798491225,116.529560899279));
#36133=CARTESIAN_POINT('Ctrl Pts',(89.4281349214653,34.4564051131519,116.476911391548));
#36134=CARTESIAN_POINT('Ctrl Pts',(88.803895450724,33.9107303771813,116.424261883817));
#36135=CARTESIAN_POINT('Ctrl Pts',(87.8842323602454,33.7030135342056,116.371612376086));
#36136=CARTESIAN_POINT('Ctrl Pts',(87.086060926954,33.9274198562768,116.318962868356));
#36137=CARTESIAN_POINT('Ctrl Pts',(86.2878894936626,34.151826178348,116.266313360625));
#36138=CARTESIAN_POINT('Ctrl Pts',(85.6112097175582,34.808355665466,116.213663852894));
#36139=CARTESIAN_POINT('Ctrl Pts',(85.3627840849953,35.5993806583668,116.161014345163));
#36140=CARTESIAN_POINT('Ctrl Pts',(85.2866104547005,35.8419290811744,116.144870664273));
#36141=CARTESIAN_POINT('Ctrl Pts',(85.2507009314977,36.0971226623065,116.128726983382));
#36142=CARTESIAN_POINT('Ctrl Pts',(85.2527053287706,36.35286573419,116.112583302492));
#36143=CARTESIAN_POINT('Ctrl Pts',(85.2549234205521,36.3553827989325,116.387416697508));
#36144=CARTESIAN_POINT('Ctrl Pts',(85.2556547086655,35.9087927866191,116.41554502776));
#36145=CARTESIAN_POINT('Ctrl Pts',(85.3691333706026,35.4618556800097,116.443673358012));
#36146=CARTESIAN_POINT('Ctrl Pts',(85.5931440023105,35.0797118042889,116.471801688264));
#36147=CARTESIAN_POINT('Ctrl Pts',(86.0124383358272,34.3644298533553,116.524451195994));
#36148=CARTESIAN_POINT('Ctrl Pts',(86.8189801798991,33.8761502567132,116.577100703725));
#36149=CARTESIAN_POINT('Ctrl Pts',(87.6471360544467,33.8362271443242,116.629750211456));
#36150=CARTESIAN_POINT('Ctrl Pts',(88.4752919289944,33.7963040319352,116.682399719187));
#36151=CARTESIAN_POINT('Ctrl Pts',(89.3250618340178,34.2047374037992,116.735049226918));
#36152=CARTESIAN_POINT('Ctrl Pts',(89.8112155053664,34.8763702017512,116.787698734649));
#36153=CARTESIAN_POINT('Ctrl Pts',(90.297369176715,35.5480029997032,116.840348242379));
#36154=CARTESIAN_POINT('Ctrl Pts',(90.4199066143887,36.4828352237432,116.89299775011));
#36155=CARTESIAN_POINT('Ctrl Pts',(90.1232773344219,37.2570749009216,116.945647257841));
#36156=CARTESIAN_POINT('Ctrl Pts',(89.8266480544551,38.0313145781,116.998296765572));
#36157=CARTESIAN_POINT('Ctrl Pts',(89.1108520568479,38.6449617084168,117.050946273303));
#36158=CARTESIAN_POINT('Ctrl Pts',(88.30038457214,38.8198286969587,117.103595781033));
#36159=CARTESIAN_POINT('Ctrl Pts',(87.4899170874322,38.9946956855005,117.156245288764));
#36160=CARTESIAN_POINT('Ctrl Pts',(86.5847781156238,38.7307825322675,117.208894796495));
#36161=CARTESIAN_POINT('Ctrl Pts',(85.995298645305,38.1477302520023,117.261544304226));
#36162=CARTESIAN_POINT('Ctrl Pts',(85.5255304561508,37.6830840214317,117.303501768653));
#36163=CARTESIAN_POINT('Ctrl Pts',(85.2562319513466,37.0157582587766,117.345459233081));
#36164=CARTESIAN_POINT('Ctrl Pts',(85.2502276147452,36.3527492241744,117.387416697508));
#36165=CARTESIAN_POINT('Origin',(87.7685555885722,36.3549260746835,114.));
#36166=CARTESIAN_POINT('',(85.2484783463287,36.3566124304548,118.387416697508));
#36167=CARTESIAN_POINT('',(85.2536733290529,36.3566354805472,118.112583302492));
#36168=CARTESIAN_POINT('',(85.2510555885723,36.3549260746835,114.));
#36169=CARTESIAN_POINT('Ctrl Pts',(85.2536733290529,36.3566354805472,118.112583302492));
#36170=CARTESIAN_POINT('Ctrl Pts',(85.25179461801,36.6536210373574,118.093854409486));
#36171=CARTESIAN_POINT('Ctrl Pts',(85.300469441061,36.950010821798,118.075125516479));
#36172=CARTESIAN_POINT('Ctrl Pts',(85.4024431538798,37.2267616956054,118.056396623473));
#36173=CARTESIAN_POINT('Ctrl Pts',(85.689105359679,38.0047466659423,118.003747115742));
#36174=CARTESIAN_POINT('Ctrl Pts',(86.3969619526868,38.6275351778612,117.951097608011));
#36175=CARTESIAN_POINT('Ctrl Pts',(87.2051169107208,38.8127955300968,117.89844810028));
#36176=CARTESIAN_POINT('Ctrl Pts',(88.0132718687548,38.9980558823324,117.845798592549));
#36177=CARTESIAN_POINT('Ctrl Pts',(88.921725191815,38.7457880748847,117.793149084819));
#36178=CARTESIAN_POINT('Ctrl Pts',(89.5186433805641,38.1703538820781,117.740499577088));
#36179=CARTESIAN_POINT('Ctrl Pts',(90.1155615693133,37.5949196892716,117.687850069357));
#36180=CARTESIAN_POINT('Ctrl Pts',(90.4009446237513,36.6963191111062,117.635200561626));
#36181=CARTESIAN_POINT('Ctrl Pts',(90.245418475919,35.8819190548391,117.582551053895));
#36182=CARTESIAN_POINT('Ctrl Pts',(90.0898923280867,35.0675189985721,117.529901546165));
#36183=CARTESIAN_POINT('Ctrl Pts',(89.4934569779841,34.3373194642033,117.477252038434));
#36184=CARTESIAN_POINT('Ctrl Pts',(88.7264973216978,34.0223453066331,117.424602530703));
#36185=CARTESIAN_POINT('Ctrl Pts',(87.9595376654115,33.707371149063,117.371953022972));
#36186=CARTESIAN_POINT('Ctrl Pts',(87.0220537029416,33.8076223682915,117.319303515241));
#36187=CARTESIAN_POINT('Ctrl Pts',(86.3390395325317,34.277651598582,117.266654007511));
#36188=CARTESIAN_POINT('Ctrl Pts',(85.6727941467207,34.7361410698757,117.215297105838));
#36189=CARTESIAN_POINT('Ctrl Pts',(85.24867688394,35.5464744870913,117.163940204165));
#36190=CARTESIAN_POINT('Ctrl Pts',(85.2470012906549,36.3552960959922,117.112583302492));
#36191=CARTESIAN_POINT('Ctrl Pts',(85.2502276147452,36.3527492241744,117.387416697508));
#36192=CARTESIAN_POINT('Ctrl Pts',(85.2486975264086,36.1837942740767,117.398108740812));
#36193=CARTESIAN_POINT('Ctrl Pts',(85.2642653937837,36.0151196462724,117.408800784115));
#36194=CARTESIAN_POINT('Ctrl Pts',(85.2979708577576,35.8501507851476,117.419492827418));
#36195=CARTESIAN_POINT('Ctrl Pts',(85.4639425093587,35.0378150058556,117.472142335149));
#36196=CARTESIAN_POINT('Ctrl Pts',(86.0697057813901,34.3153348545691,117.52479184288));
#36197=CARTESIAN_POINT('Ctrl Pts',(86.8406471062031,34.0102357212638,117.577441350611));
#36198=CARTESIAN_POINT('Ctrl Pts',(87.611588431016,33.7051365879585,117.630090858342));
#36199=CARTESIAN_POINT('Ctrl Pts',(88.5477078086104,33.8174184726344,117.682740366072));
#36200=CARTESIAN_POINT('Ctrl Pts',(89.2246297545498,34.2961800903021,117.735389873803));
#36201=CARTESIAN_POINT('Ctrl Pts',(89.9015517004892,34.7749417079699,117.788039381534));
#36202=CARTESIAN_POINT('Ctrl Pts',(90.3192762147736,35.6201830586296,117.840688889265));
#36203=CARTESIAN_POINT('Ctrl Pts',(90.2884342411026,36.4487268294297,117.893338396996));
#36204=CARTESIAN_POINT('Ctrl Pts',(90.2575922674315,37.2772706002298,117.945987904727));
#36205=CARTESIAN_POINT('Ctrl Pts',(89.778183805805,38.0891167911703,117.998637412457));
#36206=CARTESIAN_POINT('Ctrl Pts',(89.0675413920431,38.5162272770923,118.051286920188));
#36207=CARTESIAN_POINT('Ctrl Pts',(88.3568989782812,38.9433377630143,118.103936427919));
#36208=CARTESIAN_POINT('Ctrl Pts',(87.415022612384,38.9857125439178,118.15658593565));
#36209=CARTESIAN_POINT('Ctrl Pts',(86.66889762186,38.6241416574484,118.209235443381));
#36210=CARTESIAN_POINT('Ctrl Pts',(85.922772631336,38.262570770979,118.261884951112));
#36211=CARTESIAN_POINT('Ctrl Pts',(85.3723990161852,37.4970542171365,118.314534458842));
#36212=CARTESIAN_POINT('Ctrl Pts',(85.2672802854768,36.674627284163,118.367183966573));
#36213=CARTESIAN_POINT('Ctrl Pts',(85.2538148921218,36.569276866748,118.373928210218));
#36214=CARTESIAN_POINT('Ctrl Pts',(85.2476556148006,36.4629926160435,118.380672453863));
#36215=CARTESIAN_POINT('Ctrl Pts',(85.2484783463287,36.3566124304548,118.387416697508));
#36216=CARTESIAN_POINT('Origin',(87.7685555885722,36.3549260746835,114.));
#36217=CARTESIAN_POINT('',(85.2548911701606,36.3554675198059,119.387416697508));
#36218=CARTESIAN_POINT('',(85.2528439678122,36.3529021930443,119.112583302492));
#36219=CARTESIAN_POINT('',(85.2510555885723,36.3549260746835,114.));
#36220=CARTESIAN_POINT('Ctrl Pts',(85.2528439678122,36.3529021930443,119.112583302492));
#36221=CARTESIAN_POINT('Ctrl Pts',(85.2572371818151,36.925899407681,119.076418122537));
#36222=CARTESIAN_POINT('Ctrl Pts',(85.4516400977114,37.5015934845315,119.040252942582));
#36223=CARTESIAN_POINT('Ctrl Pts',(85.8105043725551,37.9438316215303,119.004087762628));
#36224=CARTESIAN_POINT('Ctrl Pts',(86.332941352996,38.5876448209081,118.951438254897));
#36225=CARTESIAN_POINT('Ctrl Pts',(87.2039332743765,38.9486151231408,118.898788747166));
#36226=CARTESIAN_POINT('Ctrl Pts',(88.0286291952941,38.8631021297693,118.846139239435));
#36227=CARTESIAN_POINT('Ctrl Pts',(88.8533251162117,38.7775891363977,118.793489731704));
#36228=CARTESIAN_POINT('Ctrl Pts',(89.6317250366665,38.245592847422,118.740840223974));
#36229=CARTESIAN_POINT('Ctrl Pts',(90.0109531891454,37.5082856910403,118.688190716243));
#36230=CARTESIAN_POINT('Ctrl Pts',(90.3901813416243,36.7709785346587,118.635541208512));
#36231=CARTESIAN_POINT('Ctrl Pts',(90.3702377261273,35.8283605108711,118.582891700781));
#36232=CARTESIAN_POINT('Ctrl Pts',(89.9601634777318,35.1077531662743,118.53024219305));
#36233=CARTESIAN_POINT('Ctrl Pts',(89.5500892293363,34.3871458216774,118.477592685319));
#36234=CARTESIAN_POINT('Ctrl Pts',(88.7498843480423,33.8885491562713,118.424943177589));
#36235=CARTESIAN_POINT('Ctrl Pts',(87.9223095480872,33.8379943863839,118.372293669858));
#36236=CARTESIAN_POINT('Ctrl Pts',(87.094734748132,33.7874396164965,118.319644162127));
#36237=CARTESIAN_POINT('Ctrl Pts',(86.2397900295158,34.1849267421278,118.266994654396));
#36238=CARTESIAN_POINT('Ctrl Pts',(85.745051579503,34.8502610193208,118.214345146665));
#36239=CARTESIAN_POINT('Ctrl Pts',(85.4263053447227,35.2789174047707,118.180424531941));
#36240=CARTESIAN_POINT('Ctrl Pts',(85.2570759345055,35.818753575417,118.146503917216));
#36241=CARTESIAN_POINT('Ctrl Pts',(85.2536733290529,36.3566354805472,118.112583302492));
#36242=CARTESIAN_POINT('Ctrl Pts',(85.2484783463287,36.3566124304548,118.387416697508));
#36243=CARTESIAN_POINT('Ctrl Pts',(85.2540783379746,35.6325267108323,118.433321961594));
#36244=CARTESIAN_POINT('Ctrl Pts',(85.5831519524022,34.9039963671497,118.47922722568));
#36245=CARTESIAN_POINT('Ctrl Pts',(86.1334931936283,34.4352495471468,118.525132489766));
#36246=CARTESIAN_POINT('Ctrl Pts',(86.7646886787542,33.8976360552089,118.577781997497));
#36247=CARTESIAN_POINT('Ctrl Pts',(87.686943495272,33.7017463834379,118.630431505227));
#36248=CARTESIAN_POINT('Ctrl Pts',(88.4821674469615,33.9363841340836,118.683081012958));
#36249=CARTESIAN_POINT('Ctrl Pts',(89.277391398651,34.1710218847294,118.735730520689));
#36250=CARTESIAN_POINT('Ctrl Pts',(89.9455844855122,34.836187057792,118.78838002842));
#36251=CARTESIAN_POINT('Ctrl Pts',(90.183831532103,35.6303371403756,118.841029536151));
#36252=CARTESIAN_POINT('Ctrl Pts',(90.4220785786939,36.4244872229593,118.893679043881));
#36253=CARTESIAN_POINT('Ctrl Pts',(90.2303795850143,37.347622215064,118.946328551612));
#36254=CARTESIAN_POINT('Ctrl Pts',(89.6956383759536,37.9812528992341,118.998978059343));
#36255=CARTESIAN_POINT('Ctrl Pts',(89.160897166893,38.6148835834043,119.051627567074));
#36256=CARTESIAN_POINT('Ctrl Pts',(88.2831137424512,38.9590099596401,119.104277074805));
#36257=CARTESIAN_POINT('Ctrl Pts',(87.4602178672702,38.8576275821734,119.156926582536));
#36258=CARTESIAN_POINT('Ctrl Pts',(86.6373219920892,38.7562452047068,119.209576090266));
#36259=CARTESIAN_POINT('Ctrl Pts',(85.8693136661691,38.2093540735378,119.262225597997));
#36260=CARTESIAN_POINT('Ctrl Pts',(85.5043577903326,37.4648789380589,119.314875105728));
#36261=CARTESIAN_POINT('Ctrl Pts',(85.3367431800309,37.1229611392932,119.339055636321));
#36262=CARTESIAN_POINT('Ctrl Pts',(85.2541453372537,36.7393664983262,119.363236166915));
#36263=CARTESIAN_POINT('Ctrl Pts',(85.2548911701606,36.3554675198059,119.387416697508));
#36264=CARTESIAN_POINT('Origin',(87.7685555885722,36.3549260746835,114.));
#36265=CARTESIAN_POINT('',(85.2503883725927,36.3527278457068,120.387416697508));
#36266=CARTESIAN_POINT('',(85.2469699766098,36.3551993258525,120.112583302492));
#36267=CARTESIAN_POINT('',(85.2510555885723,36.3549260746835,114.));
#36268=CARTESIAN_POINT('Ctrl Pts',(85.2469699766098,36.3551993258525,120.112583302492));
#36269=CARTESIAN_POINT('Ctrl Pts',(85.2469466774846,36.3701912641417,120.11163134332));
#36270=CARTESIAN_POINT('Ctrl Pts',(85.2470689410778,36.3851828122953,120.110679384147));
#36271=CARTESIAN_POINT('Ctrl Pts',(85.247337930202,36.400171727274,120.109727424975));
#36272=CARTESIAN_POINT('Ctrl Pts',(85.2622147709145,37.2291558034242,120.057077917244));
#36273=CARTESIAN_POINT('Ctrl Pts',(85.7258965986341,38.0500855073677,120.004428409513));
#36274=CARTESIAN_POINT('Ctrl Pts',(86.4281801298719,38.4908050203458,119.951778901782));
#36275=CARTESIAN_POINT('Ctrl Pts',(87.1304636611096,38.9315245333239,119.899129394052));
#36276=CARTESIAN_POINT('Ctrl Pts',(88.0713488958655,38.9920338553367,119.846479886321));
#36277=CARTESIAN_POINT('Ctrl Pts',(88.8242999073929,38.6449019184573,119.79383037859));
#36278=CARTESIAN_POINT('Ctrl Pts',(89.5772509189203,38.2977699815779,119.741180870859));
#36279=CARTESIAN_POINT('Ctrl Pts',(90.1422677072192,37.5429967858063,119.688531363128));
#36280=CARTESIAN_POINT('Ctrl Pts',(90.2632084613244,36.722747324031,119.635881855397));
#36281=CARTESIAN_POINT('Ctrl Pts',(90.3841492154295,35.9024978622557,119.583232347667));
#36282=CARTESIAN_POINT('Ctrl Pts',(90.061013935341,35.0167721344767,119.530582839936));
#36283=CARTESIAN_POINT('Ctrl Pts',(89.4402911068987,34.4671004097576,119.477933332205));
#36284=CARTESIAN_POINT('Ctrl Pts',(88.8195682784564,33.9174286850386,119.425283824474));
#36285=CARTESIAN_POINT('Ctrl Pts',(87.9012579016605,33.7038109633795,119.372634316743));
#36286=CARTESIAN_POINT('Ctrl Pts',(87.1016620113036,33.9230876004477,119.319984809013));
#36287=CARTESIAN_POINT('Ctrl Pts',(86.3020661209467,34.1423642375158,119.267335301282));
#36288=CARTESIAN_POINT('Ctrl Pts',(85.6211847170289,34.7945352333111,119.214685793551));
#36289=CARTESIAN_POINT('Ctrl Pts',(85.3676850348207,35.5839487794703,119.16203628582));
#36290=CARTESIAN_POINT('Ctrl Pts',(85.2883154066373,35.831110665812,119.145551958044));
#36291=CARTESIAN_POINT('Ctrl Pts',(85.2508415118669,36.0917262798423,119.129067630268));
#36292=CARTESIAN_POINT('Ctrl Pts',(85.2528439678122,36.3529021930443,119.112583302492));
#36293=CARTESIAN_POINT('Ctrl Pts',(85.2548911701606,36.3554675198059,119.387416697508));
#36294=CARTESIAN_POINT('Ctrl Pts',(85.2557692774417,35.9034835899905,119.415885674646));
#36295=CARTESIAN_POINT('Ctrl Pts',(85.3721747116417,35.4510778008831,119.444354651783));
#36296=CARTESIAN_POINT('Ctrl Pts',(85.6013769997188,35.0657697625188,119.472823628921));
#36297=CARTESIAN_POINT('Ctrl Pts',(86.0252555106942,34.3531948622462,119.525473136651));
#36298=CARTESIAN_POINT('Ctrl Pts',(86.8349159583979,33.8701042014898,119.578122644382));
#36299=CARTESIAN_POINT('Ctrl Pts',(87.6633111133241,33.8354994646724,119.630772152113));
#36300=CARTESIAN_POINT('Ctrl Pts',(88.4917062682503,33.800894727855,119.683421659844));
#36301=CARTESIAN_POINT('Ctrl Pts',(89.338836130399,34.2147759149767,119.736071167575));
#36302=CARTESIAN_POINT('Ctrl Pts',(89.820667213443,34.8895165312273,119.788720675305));
#36303=CARTESIAN_POINT('Ctrl Pts',(90.302498296487,35.5642571474778,119.841370183036));
#36304=CARTESIAN_POINT('Ctrl Pts',(90.4190306004264,36.4998571928572,119.894019690767));
#36305=CARTESIAN_POINT('Ctrl Pts',(90.1174360708708,37.2721761051156,119.946669198498));
#36306=CARTESIAN_POINT('Ctrl Pts',(89.8158415413152,38.0444950173741,119.999318706229));
#36307=CARTESIAN_POINT('Ctrl Pts',(89.0961201782648,38.6535327965116,120.05196821396));
#36308=CARTESIAN_POINT('Ctrl Pts',(88.2845465246492,38.823192474133,120.10461772169));
#36309=CARTESIAN_POINT('Ctrl Pts',(87.4729728710336,38.9928521517545,120.157267229421));
#36310=CARTESIAN_POINT('Ctrl Pts',(86.5695469268528,38.7231337278599,120.209916737152));
#36311=CARTESIAN_POINT('Ctrl Pts',(85.9838235012758,38.1363077943951,120.262566244883));
#36312=CARTESIAN_POINT('Ctrl Pts',(85.5208382620447,37.6724510775078,120.304183062425));
#36313=CARTESIAN_POINT('Ctrl Pts',(85.2563572505414,37.0104619014552,120.345799879966));
#36314=CARTESIAN_POINT('Ctrl Pts',(85.2503883725927,36.3527278457068,120.387416697508));
#36315=CARTESIAN_POINT('Origin',(87.7685555885722,36.3549260746835,114.));
#36316=CARTESIAN_POINT('',(85.2483527795145,36.3565049891663,121.387416697508));
#36317=CARTESIAN_POINT('',(85.2535609624353,36.356687859589,121.112583302492));
#36318=CARTESIAN_POINT('',(85.2510555885723,36.3549260746835,114.));
#36319=CARTESIAN_POINT('',(89.6820215852375,37.9909132780583,122.));
#36320=CARTESIAN_POINT('Ctrl Pts',(85.2483527795145,36.3565049891663,121.387416697508));
#36321=CARTESIAN_POINT('Ctrl Pts',(85.2538107988196,35.6272820046487,121.43366260848));
#36322=CARTESIAN_POINT('Ctrl Pts',(85.5883404885854,34.8938077603138,121.479908519451));
#36323=CARTESIAN_POINT('Ctrl Pts',(86.1458176141296,34.424974468788,121.526154430423));
#36324=CARTESIAN_POINT('Ctrl Pts',(86.7804876987815,33.8912225869868,121.578803938153));
#36325=CARTESIAN_POINT('Ctrl Pts',(87.7041222448919,33.7004745623117,121.631453445884));
#36326=CARTESIAN_POINT('Ctrl Pts',(88.4977390693866,33.9406283069268,121.684102953615));
#36327=CARTESIAN_POINT('Ctrl Pts',(89.2913558938813,34.1807820515418,121.736752461346));
#36328=CARTESIAN_POINT('Ctrl Pts',(89.9549549967602,34.8518375654471,121.789401969077));
#36329=CARTESIAN_POINT('Ctrl Pts',(90.1879202661796,35.6461235705208,121.842051476808));
#36330=CARTESIAN_POINT('Ctrl Pts',(90.420885535599,36.4404095755945,121.894700984538));
#36331=CARTESIAN_POINT('Ctrl Pts',(90.223216971559,37.3579260718367,121.947350492269));
#36332=CARTESIAN_POINT('Ctrl Pts',(89.6820215852375,37.9909132780583,122.));
#36333=CARTESIAN_POINT('',(85.851445435845,37.9934539601853,122.));
#36334=CARTESIAN_POINT('Origin',(87.7685555885722,36.3549260746835,122.));
#36335=CARTESIAN_POINT('Ctrl Pts',(85.8514365905238,37.9934601270861,122.));
#36336=CARTESIAN_POINT('Ctrl Pts',(86.3742571786771,38.6021753566418,121.949053726697));
#36337=CARTESIAN_POINT('Ctrl Pts',(87.2139816114554,38.9423514086554,121.898107453395));
#36338=CARTESIAN_POINT('Ctrl Pts',(88.0126524068155,38.8645885675841,121.847161180092));
#36339=CARTESIAN_POINT('Ctrl Pts',(88.8380243425583,38.7842259613178,121.794511672361));
#36340=CARTESIAN_POINT('Ctrl Pts',(89.6195517471766,38.2575122895073,121.74186216463));
#36341=CARTESIAN_POINT('Ctrl Pts',(90.0034363424997,37.5227256081353,121.6892126569));
#36342=CARTESIAN_POINT('Ctrl Pts',(90.3873209378227,36.7879389267633,121.636563149169));
#36343=CARTESIAN_POINT('Ctrl Pts',(90.3735627238505,35.8450792358298,121.583913641438));
#36344=CARTESIAN_POINT('Ctrl Pts',(89.968157966865,35.1218194832123,121.531264133707));
#36345=CARTESIAN_POINT('Ctrl Pts',(89.5627532098795,34.3985597305948,121.478614625976));
#36346=CARTESIAN_POINT('Ctrl Pts',(88.7657019098808,33.8948999162933,121.425965118245));
#36347=CARTESIAN_POINT('Ctrl Pts',(87.9384522395737,33.839048947649,121.373315610515));
#36348=CARTESIAN_POINT('Ctrl Pts',(87.1112025692666,33.7831979790047,121.320666102784));
#36349=CARTESIAN_POINT('Ctrl Pts',(86.2537545286512,34.1751558560176,121.268016595053));
#36350=CARTESIAN_POINT('Ctrl Pts',(85.7547622115628,34.837291622859,121.215367087322));
#36351=CARTESIAN_POINT('Ctrl Pts',(85.4300468048286,35.2681713728674,121.181105825712));
#36352=CARTESIAN_POINT('Ctrl Pts',(85.2571250437046,35.8134621481951,121.146844564102));
#36353=CARTESIAN_POINT('Ctrl Pts',(85.2535609624353,36.356687859589,121.112583302492));
#36354=CARTESIAN_POINT('Origin',(87.7685555885722,36.3549260746835,124.208423447177));
#36355=CARTESIAN_POINT('',(84.6902858090144,36.3557395542501,107.791576552823));
#36356=CARTESIAN_POINT('',(84.6999262747735,36.3552403524466,107.708423447177));
#36357=CARTESIAN_POINT('',(84.6950555885722,36.3549260746838,124.208423447177));
#36358=CARTESIAN_POINT('',(88.5623548711046,33.3857031209377,107.));
#36359=CARTESIAN_POINT('Ctrl Pts',(84.6999262747735,36.3552403524466,107.708423447177));
#36360=CARTESIAN_POINT('Ctrl Pts',(84.6996064101237,36.85041584334,107.682880329042));
#36361=CARTESIAN_POINT('Ctrl Pts',(85.0458587055101,38.3657324650862,107.604687703175));
#36362=CARTESIAN_POINT('Ctrl Pts',(87.4170211924556,39.9637884258442,107.473845569577));
#36363=CARTESIAN_POINT('Ctrl Pts',(90.6005810357291,38.6233305395511,107.315897046385));
#36364=CARTESIAN_POINT('Ctrl Pts',(91.2113484819485,35.2211464889414,107.157948523192));
#36365=CARTESIAN_POINT('Ctrl Pts',(89.5445934608762,33.6482971733151,107.052649507731));
#36366=CARTESIAN_POINT('Ctrl Pts',(88.5623548711045,33.3857031209377,107.));
#36367=CARTESIAN_POINT('',(86.9747563060389,33.385703120938,107.));
#36368=CARTESIAN_POINT('Origin',(87.7685555885722,36.3549260746835,107.));
#36369=CARTESIAN_POINT('Ctrl Pts',(84.6902858090144,36.3557395542501,107.791576552823));
#36370=CARTESIAN_POINT('Ctrl Pts',(84.690129740087,36.4002483939492,107.789262006108));
#36371=CARTESIAN_POINT('Ctrl Pts',(84.7110894559424,37.4570578636397,107.734297951662));
#36372=CARTESIAN_POINT('Ctrl Pts',(85.920358340807,39.4750889550508,107.626684389485));
#36373=CARTESIAN_POINT('Ctrl Pts',(89.3710241690437,39.6084644686119,107.468735866293));
#36374=CARTESIAN_POINT('Ctrl Pts',(91.3686332599885,36.7911510990924,107.3107873431));
#36375=CARTESIAN_POINT('Ctrl Pts',(90.1161181236528,33.6146079014889,107.154542054336));
#36376=CARTESIAN_POINT('Ctrl Pts',(87.9198086998421,33.1297337399419,107.050946273303));
#36377=CARTESIAN_POINT('Ctrl Pts',(86.9728422455434,33.3806145099939,107.));
#36378=CARTESIAN_POINT('Origin',(87.7685555885722,36.3549260746835,124.208423447177));
#36379=CARTESIAN_POINT('',(84.6986440547572,36.3567914692534,108.791576552823));
#36380=CARTESIAN_POINT('',(84.6934624439954,36.3523677970343,108.708423447177));
#36381=CARTESIAN_POINT('',(84.6950555885722,36.3549260746838,124.208423447177));
#36382=CARTESIAN_POINT('Ctrl Pts',(84.6934624439954,36.3523677970344,108.708423447177));
#36383=CARTESIAN_POINT('Ctrl Pts',(84.7008503007187,37.1811158847336,108.665444042093));
#36384=CARTESIAN_POINT('Ctrl Pts',(85.4724993959125,39.0372064318679,108.569815129278));
#36385=CARTESIAN_POINT('Ctrl Pts',(88.6015534780661,39.8844994763739,108.421536708732));
#36386=CARTESIAN_POINT('Ctrl Pts',(91.1794498546833,37.5869249364573,108.26358818554));
#36387=CARTESIAN_POINT('Ctrl Pts',(90.6647258333095,34.1722679839027,108.105639662347));
#36388=CARTESIAN_POINT('Ctrl Pts',(87.5242687079243,32.736697544997,107.947691139155));
#36389=CARTESIAN_POINT('Ctrl Pts',(85.0771138477131,34.2830645841973,107.815285734098));
#36390=CARTESIAN_POINT('Ctrl Pts',(84.7002657155484,35.8297594889657,107.735529836772));
#36391=CARTESIAN_POINT('Ctrl Pts',(84.6999262747735,36.3552403524466,107.708423447177));
#36392=CARTESIAN_POINT('Ctrl Pts',(84.6986440547572,36.3567914692533,108.791576552823));
#36393=CARTESIAN_POINT('Ctrl Pts',(84.6964999234298,36.7392744241785,108.771825719159));
#36394=CARTESIAN_POINT('Ctrl Pts',(84.939494334228,38.1387104097186,108.699425377765));
#36395=CARTESIAN_POINT('Ctrl Pts',(87.0264678344641,39.9047351075969,108.57437552864));
#36396=CARTESIAN_POINT('Ctrl Pts',(90.3353210088379,38.9168747734219,108.416427005448));
#36397=CARTESIAN_POINT('Ctrl Pts',(91.3169640944224,35.6061628347523,108.258478482255));
#36398=CARTESIAN_POINT('Ctrl Pts',(89.0813771113567,32.9743536285202,108.100529959063));
#36399=CARTESIAN_POINT('Ctrl Pts',(85.7056888771381,33.401213512673,107.944895982585));
#36400=CARTESIAN_POINT('Ctrl Pts',(84.6936798746098,35.3877959406313,107.841911513838));
#36401=CARTESIAN_POINT('Ctrl Pts',(84.6902858090144,36.3557395542501,107.791576552823));
#36402=CARTESIAN_POINT('Origin',(87.7685555885722,36.3549260746835,124.208423447177));
#36403=CARTESIAN_POINT('',(84.6967208028556,36.352333414281,109.791576552823));
#36404=CARTESIAN_POINT('',(84.6924244957587,36.3571941260871,109.708423447177));
#36405=CARTESIAN_POINT('',(84.6950555885722,36.3549260746838,124.208423447177));
#36406=CARTESIAN_POINT('Ctrl Pts',(84.6924244957587,36.3571941260872,109.708423447177));
#36407=CARTESIAN_POINT('Ctrl Pts',(84.6911853742644,36.5068138857211,109.700657262876));
#36408=CARTESIAN_POINT('Ctrl Pts',(84.7688482751212,37.6694639479526,109.640241570843));
#36409=CARTESIAN_POINT('Ctrl Pts',(86.2502054472947,39.6483231784334,109.527176371079));
#36410=CARTESIAN_POINT('Ctrl Pts',(89.696256450466,39.4267040036787,109.369227847887));
#36411=CARTESIAN_POINT('Ctrl Pts',(91.3945201363532,36.4199976317768,109.211279324695));
#36412=CARTESIAN_POINT('Ctrl Pts',(89.805231169669,33.3542919795258,109.053330801502));
#36413=CARTESIAN_POINT('Ctrl Pts',(86.3693521976711,33.0091718082685,108.89538227831));
#36414=CARTESIAN_POINT('Ctrl Pts',(84.7918202895625,34.9660087126265,108.780413160201));
#36415=CARTESIAN_POINT('Ctrl Pts',(84.691800221526,36.1659045581767,108.718093549824));
#36416=CARTESIAN_POINT('Ctrl Pts',(84.6934624439954,36.3523677970344,108.708423447177));
#36417=CARTESIAN_POINT('Ctrl Pts',(84.6967208028556,36.352333414281,109.791576552823));
#36418=CARTESIAN_POINT('Ctrl Pts',(84.7025802483439,37.0713395705354,109.754389432211));
#36419=CARTESIAN_POINT('Ctrl Pts',(85.3117911792528,38.8172613514562,109.664552803868));
#36420=CARTESIAN_POINT('Ctrl Pts',(88.2120005651333,39.9542599759734,109.522066667795));
#36421=CARTESIAN_POINT('Ctrl Pts',(91.0248783714271,37.9512375173972,109.364118144602));
#36422=CARTESIAN_POINT('Ctrl Pts',(90.8853473213453,34.5008878826802,109.20616962141));
#36423=CARTESIAN_POINT('Ctrl Pts',(87.9199160530301,32.731538577869,109.048221098218));
#36424=CARTESIAN_POINT('Ctrl Pts',(85.2052266838201,34.0578509982748,108.910023408688));
#36425=CARTESIAN_POINT('Ctrl Pts',(84.7022155028742,35.719695218788,108.82447522689));
#36426=CARTESIAN_POINT('Ctrl Pts',(84.6986440547572,36.3567914692533,108.791576552823));
#36427=CARTESIAN_POINT('Origin',(87.7685555885722,36.3549260746835,124.208423447177));
#36428=CARTESIAN_POINT('',(84.6902140242538,36.3556108815602,110.791576552823));
#36429=CARTESIAN_POINT('',(84.6998361685216,36.3552744910741,110.708423447177));
#36430=CARTESIAN_POINT('',(84.6950555885722,36.3549260746838,124.208423447177));
#36431=CARTESIAN_POINT('Ctrl Pts',(84.6998361685216,36.3552744910741,110.708423447177));
#36432=CARTESIAN_POINT('Ctrl Pts',(84.6993368730504,36.8438060463592,110.683220975927));
#36433=CARTESIAN_POINT('Ctrl Pts',(85.0389979619791,38.3522541503725,110.605368996946));
#36434=CARTESIAN_POINT('Ctrl Pts',(87.3945229743647,39.962134280427,110.474867510234));
#36435=CARTESIAN_POINT('Ctrl Pts',(90.5845853467483,38.6400579781975,110.316918987042));
#36436=CARTESIAN_POINT('Ctrl Pts',(91.2214391886919,35.2461220838395,110.158970463849));
#36437=CARTESIAN_POINT('Ctrl Pts',(88.7276684735458,32.8575050336255,110.001021940657));
#36438=CARTESIAN_POINT('Ctrl Pts',(85.529673083003,33.6014239812827,109.850839601766));
#36439=CARTESIAN_POINT('Ctrl Pts',(84.6995857848333,35.4924925169032,109.753306770606));
#36440=CARTESIAN_POINT('Ctrl Pts',(84.6924244957587,36.3571941260872,109.708423447177));
#36441=CARTESIAN_POINT('Ctrl Pts',(84.6902140242538,36.3556108815602,110.791576552823));
#36442=CARTESIAN_POINT('Ctrl Pts',(84.6900983802807,36.3935671694569,110.789602652993));
#36443=CARTESIAN_POINT('Ctrl Pts',(84.7078623206447,37.4438145955638,110.734979245433));
#36444=CARTESIAN_POINT('Ctrl Pts',(85.9003808808979,39.463265081444,110.627706330142));
#36445=CARTESIAN_POINT('Ctrl Pts',(89.3500610946321,39.6184653269691,110.46975780695));
#36446=CARTESIAN_POINT('Ctrl Pts',(91.365838365503,36.8147137894109,110.311809283757));
#36447=CARTESIAN_POINT('Ctrl Pts',(90.1200687486007,33.5940867128609,110.153860760565));
#36448=CARTESIAN_POINT('Ctrl Pts',(86.7422536682402,32.8766287223663,109.995912237372));
#36449=CARTESIAN_POINT('Ctrl Pts',(84.8711429126263,34.7392605484639,109.875150834792));
#36450=CARTESIAN_POINT('Ctrl Pts',(84.6942844481997,36.0533709954071,109.807038939942));
#36451=CARTESIAN_POINT('Ctrl Pts',(84.6967208028556,36.352333414281,109.791576552823));
#36452=CARTESIAN_POINT('Origin',(87.7685555885722,36.3549260746835,124.208423447177));
#36453=CARTESIAN_POINT('',(84.6985184073145,36.356868130103,111.791576552823));
#36454=CARTESIAN_POINT('',(84.6936553669982,36.3523302808631,111.708423447177));
#36455=CARTESIAN_POINT('',(84.6950555885722,36.3549260746838,124.208423447177));
#36456=CARTESIAN_POINT('Ctrl Pts',(84.6936553669982,36.3523302808631,111.708423447177));
#36457=CARTESIAN_POINT('Ctrl Pts',(84.7010362467823,37.1746423292757,111.665784688979));
#36458=CARTESIAN_POINT('Ctrl Pts',(85.4624962321431,39.0243972984566,111.570496423049));
#36459=CARTESIAN_POINT('Ctrl Pts',(88.5788817288668,39.8897843430778,111.422558649389));
#36460=CARTESIAN_POINT('Ctrl Pts',(91.1714507607514,37.608782477213,111.264610126197));
#36461=CARTESIAN_POINT('Ctrl Pts',(90.6787182344735,34.1909471455679,111.106661603004));
#36462=CARTESIAN_POINT('Ctrl Pts',(87.5474297456003,32.7351256943546,110.948713079812));
#36463=CARTESIAN_POINT('Ctrl Pts',(85.0842716491725,34.2698856564043,110.81596702787));
#36464=CARTESIAN_POINT('Ctrl Pts',(84.7003799319041,35.8232336730648,110.735870483658));
#36465=CARTESIAN_POINT('Ctrl Pts',(84.6998361685216,36.3552744910741,110.708423447177));
#36466=CARTESIAN_POINT('Ctrl Pts',(84.6985184073145,36.356868130103,111.791576552823));
#36467=CARTESIAN_POINT('Ctrl Pts',(84.6963187303381,36.7327156285024,111.772166366045));
#36468=CARTESIAN_POINT('Ctrl Pts',(84.9337530284994,38.1253552052707,111.700106671536));
#36469=CARTESIAN_POINT('Ctrl Pts',(87.0036900655912,39.8998984089112,111.575397469297));
#36470=CARTESIAN_POINT('Ctrl Pts',(90.3188173102936,38.9333002270083,111.417448946105));
#36471=CARTESIAN_POINT('Ctrl Pts',(91.3216998146175,35.6289686189096,111.259500422912));
#36472=CARTESIAN_POINT('Ctrl Pts',(89.1030545131784,32.9828405569386,111.10155189972));
#36473=CARTESIAN_POINT('Ctrl Pts',(85.7173071460403,33.3889405742214,110.945577276356));
#36474=CARTESIAN_POINT('Ctrl Pts',(84.6931829330837,35.3811653021443,110.842252160724));
#36475=CARTESIAN_POINT('Ctrl Pts',(84.6902140242538,36.3556108815602,110.791576552823));
#36476=CARTESIAN_POINT('Origin',(87.7685555885722,36.3549260746835,124.208423447177));
#36477=CARTESIAN_POINT('',(84.6968968951659,36.3523700745377,112.791576552823));
#36478=CARTESIAN_POINT('',(84.6922487139548,36.3571283698866,112.708423447177));
#36479=CARTESIAN_POINT('',(84.6950555885722,36.3549260746838,124.208423447177));
#36480=CARTESIAN_POINT('Ctrl Pts',(84.6922487139549,36.3571283698866,112.708423447177));
#36481=CARTESIAN_POINT('Ctrl Pts',(84.6910878504133,36.5001640619827,112.700997909761));
#36482=CARTESIAN_POINT('Ctrl Pts',(84.7648941835271,37.6561662491889,112.640922864614));
#36483=CARTESIAN_POINT('Ctrl Pts',(86.2290897937213,39.6385059043325,112.528198311736));
#36484=CARTESIAN_POINT('Ctrl Pts',(89.6764929464422,39.4390185618894,112.370249788544));
#36485=CARTESIAN_POINT('Ctrl Pts',(91.3940273240736,36.4432783597291,112.212301265351));
#36486=CARTESIAN_POINT('Ctrl Pts',(89.8244567428654,33.3674318278324,112.054352742159));
#36487=CARTESIAN_POINT('Ctrl Pts',(86.3908631124647,33.0002554690232,111.896404218966));
#36488=CARTESIAN_POINT('Ctrl Pts',(84.7960898684621,34.9526928622712,111.781094453973));
#36489=CARTESIAN_POINT('Ctrl Pts',(84.6919224802546,36.1592674361242,111.71843419671));
#36490=CARTESIAN_POINT('Ctrl Pts',(84.6936553669982,36.3523302808631,111.708423447177));
#36491=CARTESIAN_POINT('Ctrl Pts',(84.696896895166,36.3523700745377,112.791576552823));
#36492=CARTESIAN_POINT('Ctrl Pts',(84.7025959476166,37.0648934282683,112.754730079097));
#36493=CARTESIAN_POINT('Ctrl Pts',(85.3029472141711,38.8041984337469,112.66523409764));
#36494=CARTESIAN_POINT('Ctrl Pts',(88.188880109704,39.957033154659,112.523088608452));
#36495=CARTESIAN_POINT('Ctrl Pts',(91.0145613228638,37.9721134143629,112.365140085259));
#36496=CARTESIAN_POINT('Ctrl Pts',(90.8971878595435,34.5209390977093,112.207191562067));
#36497=CARTESIAN_POINT('Ctrl Pts',(87.9431786691826,32.7325849948854,112.049243038874));
#36498=CARTESIAN_POINT('Ctrl Pts',(85.2133167317337,34.0446657231455,111.91070470246));
#36499=CARTESIAN_POINT('Ctrl Pts',(84.702285283432,35.7132413699984,111.824815873776));
#36500=CARTESIAN_POINT('Ctrl Pts',(84.6985184073145,36.356868130103,111.791576552823));
#36501=CARTESIAN_POINT('Origin',(87.7685555885722,36.3549260746835,124.208423447177));
#36502=CARTESIAN_POINT('',(84.6901547879111,36.3554949863923,113.791576552823));
#36503=CARTESIAN_POINT('',(84.6998102914154,36.3553794097646,113.708423447177));
#36504=CARTESIAN_POINT('',(84.6950555885722,36.3549260746838,124.208423447177));
#36505=CARTESIAN_POINT('Ctrl Pts',(84.6998102914154,36.3553794097646,113.708423447177));
#36506=CARTESIAN_POINT('Ctrl Pts',(84.6991691146865,36.8372976164334,113.683561622813));
#36507=CARTESIAN_POINT('Ctrl Pts',(85.0323508879597,38.3389281403725,113.606050290717));
#36508=CARTESIAN_POINT('Ctrl Pts',(87.3713688061258,39.9596582548938,113.475889450891));
#36509=CARTESIAN_POINT('Ctrl Pts',(90.5698544680408,38.6580925947341,113.317940927699));
#36510=CARTESIAN_POINT('Ctrl Pts',(91.2284876335959,35.2683158984878,113.159992404506));
#36511=CARTESIAN_POINT('Ctrl Pts',(88.7501056430045,32.8637356012436,113.002043881314));
#36512=CARTESIAN_POINT('Ctrl Pts',(85.5401350086611,33.5887456327592,112.851520895538));
#36513=CARTESIAN_POINT('Ctrl Pts',(84.6993187555426,35.4859938605954,112.753647417492));
#36514=CARTESIAN_POINT('Ctrl Pts',(84.6922487139549,36.3571283698866,112.708423447177));
#36515=CARTESIAN_POINT('Ctrl Pts',(84.6901547879111,36.3554949863923,113.791576552823));
#36516=CARTESIAN_POINT('Ctrl Pts',(84.6900741046407,36.3868993254153,113.789943299879));
#36517=CARTESIAN_POINT('Ctrl Pts',(84.7046792722822,37.4305764228221,113.735660539204));
#36518=CARTESIAN_POINT('Ctrl Pts',(85.880460753186,39.4512054566615,113.628728270799));
#36519=CARTESIAN_POINT('Ctrl Pts',(89.3290733119119,39.6285528942548,113.470779747607));
#36520=CARTESIAN_POINT('Ctrl Pts',(91.3628119118867,36.837802457402,113.312831224414));
#36521=CARTESIAN_POINT('Ctrl Pts',(90.1377476178771,33.6092426903596,113.154882701222));
#36522=CARTESIAN_POINT('Ctrl Pts',(86.7646089666149,32.8701105416984,112.996934178029));
#36523=CARTESIAN_POINT('Ctrl Pts',(84.8762651228155,34.7259097370386,112.875832128563));
#36524=CARTESIAN_POINT('Ctrl Pts',(84.6944526363112,36.046776902396,112.807379586827));
#36525=CARTESIAN_POINT('Ctrl Pts',(84.696896895166,36.3523700745377,112.791576552823));
#36526=CARTESIAN_POINT('Origin',(87.7685555885722,36.3549260746835,124.208423447177));
#36527=CARTESIAN_POINT('',(84.6983875051821,36.3569420804818,114.791576552823));
#36528=CARTESIAN_POINT('',(84.6938495503113,36.3522971345412,114.708423447178));
#36529=CARTESIAN_POINT('',(84.6950555885722,36.3549260746838,124.208423447177));
#36530=CARTESIAN_POINT('Ctrl Pts',(84.6938495503113,36.3522971345412,114.708423447177));
#36531=CARTESIAN_POINT('Ctrl Pts',(84.7012113817027,37.1681725773841,114.666125335864));
#36532=CARTESIAN_POINT('Ctrl Pts',(85.4525660601554,39.0115737713416,114.571177716821));
#36533=CARTESIAN_POINT('Ctrl Pts',(88.5561677048511,39.8949145754395,114.423580590046));
#36534=CARTESIAN_POINT('Ctrl Pts',(91.1633296007399,37.630606613653,114.265632066854));
#36535=CARTESIAN_POINT('Ctrl Pts',(90.6925531471805,34.2096779052527,114.107683543661));
#36536=CARTESIAN_POINT('Ctrl Pts',(87.5706770365969,32.7337804673015,113.949735020469));
#36537=CARTESIAN_POINT('Ctrl Pts',(85.0913690235364,34.2565906200758,113.816648321641));
#36538=CARTESIAN_POINT('Ctrl Pts',(84.7005269249039,35.8167467519618,113.736211130544));
#36539=CARTESIAN_POINT('Ctrl Pts',(84.6998102914154,36.3553794097646,113.708423447177));
#36540=CARTESIAN_POINT('Ctrl Pts',(84.6983875051821,36.3569420804818,114.791576552823));
#36541=CARTESIAN_POINT('Ctrl Pts',(84.6961380025769,36.726153900471,114.772507012931));
#36542=CARTESIAN_POINT('Ctrl Pts',(84.9280663987333,38.1119998679058,114.700787965308));
#36543=CARTESIAN_POINT('Ctrl Pts',(86.9809435714815,39.8949141296362,114.576419409954));
#36544=CARTESIAN_POINT('Ctrl Pts',(90.3022090008012,38.9496223007136,114.418470886762));
#36545=CARTESIAN_POINT('Ctrl Pts',(91.3262879388381,35.6517983177679,114.260522363569));
#36546=CARTESIAN_POINT('Ctrl Pts',(89.1246791584273,32.9914788873536,114.102573840377));
#36547=CARTESIAN_POINT('Ctrl Pts',(85.7289940423128,33.376670074587,113.946258570128));
#36548=CARTESIAN_POINT('Ctrl Pts',(84.6926750088575,35.3745497095108,113.84259280761));
#36549=CARTESIAN_POINT('Ctrl Pts',(84.6901547879111,36.3554949863923,113.791576552823));
#36550=CARTESIAN_POINT('Origin',(87.7685555885722,36.3549260746835,124.208423447177));
#36551=CARTESIAN_POINT('',(84.6970696805284,36.352410699706,115.791576552823));
#36552=CARTESIAN_POINT('',(84.6920768117566,36.3570585844756,115.708423447177));
#36553=CARTESIAN_POINT('',(84.6950555885722,36.3549260746838,124.208423447177));
#36554=CARTESIAN_POINT('Ctrl Pts',(84.6920768117566,36.3570585844756,115.708423447177));
#36555=CARTESIAN_POINT('Ctrl Pts',(84.6909942761927,36.4935125897422,115.701338556647));
#36556=CARTESIAN_POINT('Ctrl Pts',(84.76098699805,37.6428717192427,115.641604158385));
#36557=CARTESIAN_POINT('Ctrl Pts',(86.2080376687123,39.6285533065152,115.529220252393));
#36558=CARTESIAN_POINT('Ctrl Pts',(89.6566506617342,39.4512058465864,115.371271729201));
#36559=CARTESIAN_POINT('Ctrl Pts',(91.3933852757362,36.4665556865659,115.213323206008));
#36560=CARTESIAN_POINT('Ctrl Pts',(89.843597056598,33.3806943525127,115.055374682816));
#36561=CARTESIAN_POINT('Ctrl Pts',(86.4124318479345,32.9914784637831,114.897426159623));
#36562=CARTESIAN_POINT('Ctrl Pts',(84.8004066819477,34.9393730713774,114.781775747744));
#36563=CARTESIAN_POINT('Ctrl Pts',(84.6920479276683,36.1526321879448,114.718774843595));
#36564=CARTESIAN_POINT('Ctrl Pts',(84.6938495503113,36.3522971345412,114.708423447177));
#36565=CARTESIAN_POINT('Ctrl Pts',(84.6970696805284,36.352410699706,115.791576552823));
#36566=CARTESIAN_POINT('Ctrl Pts',(84.7026032729329,37.0584473418203,115.755070725982));
#36567=CARTESIAN_POINT('Ctrl Pts',(85.2941694274566,38.7911233555952,115.665915391411));
#36568=CARTESIAN_POINT('Ctrl Pts',(88.1657423210009,39.9596578009367,115.524110549109));
#36569=CARTESIAN_POINT('Ctrl Pts',(91.0041104497151,37.9929226739502,115.366162025916));
#36570=CARTESIAN_POINT('Ctrl Pts',(90.9088993907837,34.5410658478232,115.208213502724));
#36571=CARTESIAN_POINT('Ctrl Pts',(87.9664341156267,32.7337809233254,115.050264979531));
#36572=CARTESIAN_POINT('Ctrl Pts',(85.2214706499081,34.0314892252637,114.911385996231));
#36573=CARTESIAN_POINT('Ctrl Pts',(84.7023487032794,35.7067889508769,114.825156520661));
#36574=CARTESIAN_POINT('Ctrl Pts',(84.6983875051821,36.3569420804818,114.791576552823));
#36575=CARTESIAN_POINT('Origin',(87.7685555885722,36.3549260746835,124.208423447177));
#36576=CARTESIAN_POINT('',(84.690105882654,36.3553778166865,116.791576552823));
#36577=CARTESIAN_POINT('',(84.6997776468007,36.3554836683198,116.708423447177));
#36578=CARTESIAN_POINT('',(84.6950555885722,36.3549260746838,124.208423447177));
#36579=CARTESIAN_POINT('Ctrl Pts',(84.6997776468007,36.3554836683198,116.708423447177));
#36580=CARTESIAN_POINT('Ctrl Pts',(84.6989993421585,36.8307861836476,116.683902269698));
#36581=CARTESIAN_POINT('Ctrl Pts',(85.0257621552687,38.3255989427417,116.606731584489));
#36582=CARTESIAN_POINT('Ctrl Pts',(87.3482310145089,39.9570336082856,116.476911391548));
#36583=CARTESIAN_POINT('Ctrl Pts',(90.5550080912271,38.6760322509801,116.318962868356));
#36584=CARTESIAN_POINT('Ctrl Pts',(91.2353934299102,35.2905545168799,116.161014345163));
#36585=CARTESIAN_POINT('Ctrl Pts',(88.7725023369588,32.8701101028426,116.003065821971));
#36586=CARTESIAN_POINT('Ctrl Pts',(85.5506677531235,33.576088055363,115.852202189309));
#36587=CARTESIAN_POINT('Ctrl Pts',(84.6990388556109,35.4794904006645,115.753988064378));
#36588=CARTESIAN_POINT('Ctrl Pts',(84.6920768117566,36.3570585844756,115.708423447177));
#36589=CARTESIAN_POINT('Ctrl Pts',(84.690105882654,36.3553778166865,116.791576552823));
#36590=CARTESIAN_POINT('Ctrl Pts',(84.690054395401,36.3802311048682,116.790283946765));
#36591=CARTESIAN_POINT('Ctrl Pts',(84.7015398827634,37.4173420024755,116.736341832976));
#36592=CARTESIAN_POINT('Ctrl Pts',(85.8606184709768,39.4390181734991,116.629750211456));
#36593=CARTESIAN_POINT('Ctrl Pts',(89.3080211895539,39.6385054908189,116.471801688264));
#36594=CARTESIAN_POINT('Ctrl Pts',(91.3596372684504,36.8608712170826,116.313853165071));
#36595=CARTESIAN_POINT('Ctrl Pts',(90.1553288060137,33.6245118703589,116.155904641879));
#36596=CARTESIAN_POINT('Ctrl Pts',(86.7870056577489,32.8637360409022,115.997956118686));
#36597=CARTESIAN_POINT('Ctrl Pts',(84.8814395432927,34.71255787358,115.876513422334));
#36598=CARTESIAN_POINT('Ctrl Pts',(84.6946226040563,36.0401857418374,115.807720233713));
#36599=CARTESIAN_POINT('Ctrl Pts',(84.6970696805284,36.352410699706,115.791576552823));
#36600=CARTESIAN_POINT('Origin',(87.7685555885722,36.3549260746835,124.208423447177));
#36601=CARTESIAN_POINT('',(84.6982514675662,36.3570130097076,117.791576552823));
#36602=CARTESIAN_POINT('',(84.6940447533955,36.3522684579846,117.708423447177));
#36603=CARTESIAN_POINT('',(84.6950555885722,36.3549260746838,124.208423447177));
#36604=CARTESIAN_POINT('Ctrl Pts',(84.6940447533956,36.3522684579846,117.708423447177));
#36605=CARTESIAN_POINT('Ctrl Pts',(84.7013751718839,37.1617057043996,117.66646598275));
#36606=CARTESIAN_POINT('Ctrl Pts',(85.4427051945229,38.9987326982796,117.571859010592));
#36607=CARTESIAN_POINT('Ctrl Pts',(88.5334212078769,39.8998988553421,117.424602530703));
#36608=CARTESIAN_POINT('Ctrl Pts',(91.1550684753794,37.6523781542154,117.266654007511));
#36609=CARTESIAN_POINT('Ctrl Pts',(90.7062675045469,34.2284971128012,117.108705484318));
#36610=CARTESIAN_POINT('Ctrl Pts',(87.5939324859696,32.7325845387109,116.950756961126));
#36611=CARTESIAN_POINT('Ctrl Pts',(85.0985267224163,34.2433006021635,116.817329615412));
#36612=CARTESIAN_POINT('Ctrl Pts',(84.700670442835,35.8102624556703,116.736551777429));
#36613=CARTESIAN_POINT('Ctrl Pts',(84.6997776468007,36.3554836683198,116.708423447177));
#36614=CARTESIAN_POINT('Ctrl Pts',(84.6982514675662,36.3570130097076,117.791576552823));
#36615=CARTESIAN_POINT('Ctrl Pts',(84.6959578356337,36.7195890211696,117.772847659816));
#36616=CARTESIAN_POINT('Ctrl Pts',(84.9224341684481,38.0986442956688,117.701469259079));
#36617=CARTESIAN_POINT('Ctrl Pts',(86.9582295503262,39.8897838979207,117.577441350611));
#36618=CARTESIAN_POINT('Ctrl Pts',(90.2854962296813,38.9658373960053,117.419492827418));
#36619=CARTESIAN_POINT('Ctrl Pts',(91.3307293790144,35.6746570063435,117.261544304226));
#36620=CARTESIAN_POINT('Ctrl Pts',(89.1462478911809,33.0002558914885,117.103595781033));
#36621=CARTESIAN_POINT('Ctrl Pts',(85.7407542491592,33.3644273369264,116.946939863899));
#36622=CARTESIAN_POINT('Ctrl Pts',(84.6921515374552,35.367924702503,116.842933454495));
#36623=CARTESIAN_POINT('Ctrl Pts',(84.690105882654,36.3553778166865,116.791576552823));
#36624=CARTESIAN_POINT('Origin',(87.7685555885722,36.3549260746835,124.208423447177));
#36625=CARTESIAN_POINT('',(84.69723893856,36.352455210645,118.791576552823));
#36626=CARTESIAN_POINT('',(84.6919091520139,36.3569848689092,118.708423447178));
#36627=CARTESIAN_POINT('',(84.6950555885722,36.3549260746838,124.208423447177));
#36628=CARTESIAN_POINT('Ctrl Pts',(84.6919091520139,36.3569848689092,118.708423447178));
#36629=CARTESIAN_POINT('Ctrl Pts',(84.690904716919,36.48685954633,118.701679203533));
#36630=CARTESIAN_POINT('Ctrl Pts',(84.7571265200965,37.6295804150404,118.642285452157));
#36631=CARTESIAN_POINT('Ctrl Pts',(86.1870498833489,39.6184657379601,118.53024219305));
#36632=CARTESIAN_POINT('Ctrl Pts',(89.6367305315139,39.4632654728871,118.372293669858));
#36633=CARTESIAN_POINT('Ctrl Pts',(91.3925937769666,36.4898284108945,118.214345146665));
#36634=CARTESIAN_POINT('Ctrl Pts',(89.8626518171021,33.3940795037413,118.056396623473));
#36635=CARTESIAN_POINT('Ctrl Pts',(86.4340564959065,32.9828401322801,117.89844810028));
#36636=CARTESIAN_POINT('Ctrl Pts',(84.8047721902053,34.926050666858,117.782457041515));
#36637=CARTESIAN_POINT('Ctrl Pts',(84.6921767388961,36.1459991276468,117.719115490481));
#36638=CARTESIAN_POINT('Ctrl Pts',(84.6940447533956,36.3522684579846,117.708423447177));
#36639=CARTESIAN_POINT('Ctrl Pts',(84.69723893856,36.352455210645,118.791576552823));
#36640=CARTESIAN_POINT('Ctrl Pts',(84.7026024115443,37.0520011646411,118.755411372868));
#36641=CARTESIAN_POINT('Ctrl Pts',(85.2854576115966,38.7780364187139,118.666596685182));
#36642=CARTESIAN_POINT('Ctrl Pts',(88.1425881556754,39.9621338261614,118.525132489766));
#36643=CARTESIAN_POINT('Ctrl Pts',(90.9935261761534,38.0136643991501,118.367183966573));
#36644=CARTESIAN_POINT('Ctrl Pts',(90.9204814465843,34.5612673829304,118.209235443381));
#36645=CARTESIAN_POINT('Ctrl Pts',(87.989681403696,32.7351261502086,118.051286920188));
#36646=CARTESIAN_POINT('Ctrl Pts',(85.2296887066039,34.0183220575488,117.912067290002));
#36647=CARTESIAN_POINT('Ctrl Pts',(84.7024055521176,35.7003377225505,117.825497167547));
#36648=CARTESIAN_POINT('Ctrl Pts',(84.6982514675662,36.3570130097076,117.791576552823));
#36649=CARTESIAN_POINT('Origin',(87.7685555885722,36.3549260746835,124.208423447177));
#36650=CARTESIAN_POINT('',(84.6900676527761,36.3552596744725,119.791576552823));
#36651=CARTESIAN_POINT('',(84.6997382737804,36.3555871001389,119.708423447177));
#36652=CARTESIAN_POINT('',(84.6950555885722,36.3549260746838,124.208423447177));
#36653=CARTESIAN_POINT('Ctrl Pts',(84.6997382737804,36.3555871001389,119.708423447177));
#36654=CARTESIAN_POINT('Ctrl Pts',(84.6988277206765,36.8242717120483,119.684242916584));
#36655=CARTESIAN_POINT('Ctrl Pts',(85.0192315268969,38.3122667840641,119.60741287826));
#36656=CARTESIAN_POINT('Ctrl Pts',(87.325110556169,39.9542604293109,119.477933332205));
#36657=CARTESIAN_POINT('Ctrl Pts',(90.5400468282905,38.6938762179578,119.319984809012));
#36658=CARTESIAN_POINT('Ctrl Pts',(91.2421562905436,35.3128370145015,119.16203628582));
#36659=CARTESIAN_POINT('Ctrl Pts',(88.7948576381488,32.8766282843233,119.004087762628));
#36660=CARTESIAN_POINT('Ctrl Pts',(85.5612714692701,33.5634516241642,118.85288348308));
#36661=CARTESIAN_POINT('Ctrl Pts',(84.6987459243371,35.472981905946,118.754328711263));
#36662=CARTESIAN_POINT('Ctrl Pts',(84.6919091520139,36.3569848689092,118.708423447178));
#36663=CARTESIAN_POINT('Ctrl Pts',(84.6900676527761,36.3552596744725,119.791576552823));
#36664=CARTESIAN_POINT('Ctrl Pts',(84.6900392079454,36.373562642628,119.79062459365));
#36665=CARTESIAN_POINT('Ctrl Pts',(84.6984438504603,37.4041114728583,119.737023126747));
#36666=CARTESIAN_POINT('Ctrl Pts',(85.8408549696731,39.426703616461,119.630772152113));
#36667=CARTESIAN_POINT('Ctrl Pts',(89.286905538518,39.6483227638767,119.472823628921));
#36668=CARTESIAN_POINT('Ctrl Pts',(91.3563145937352,36.8839190889564,119.314875105728));
#36669=CARTESIAN_POINT('Ctrl Pts',(90.1728115748451,33.639893637919,119.156926582536));
#36670=CARTESIAN_POINT('Ctrl Pts',(86.8094428243991,32.8575054740432,118.998978059343));
#36671=CARTESIAN_POINT('Ctrl Pts',(84.886666399667,34.6992050833937,118.877194716105));
#36672=CARTESIAN_POINT('Ctrl Pts',(84.6947942321655,36.0335975466026,118.808060880599));
#36673=CARTESIAN_POINT('Ctrl Pts',(84.69723893856,36.352455210645,118.791576552823));
#36674=CARTESIAN_POINT('Origin',(87.7685555885722,36.3549260746835,124.208423447177));
#36675=CARTESIAN_POINT('',(84.6981142843292,36.357076956871,120.791576552823));
#36676=CARTESIAN_POINT('',(84.6942410152602,36.3522423579964,120.708423447177));
#36677=CARTESIAN_POINT('',(84.6950555885722,36.3549260746838,124.208423447177));
#36678=CARTESIAN_POINT('Ctrl Pts',(84.6942410152602,36.3522423579965,120.708423447177));
#36679=CARTESIAN_POINT('Ctrl Pts',(84.7015281439098,37.1552396252626,120.666806629636));
#36680=CARTESIAN_POINT('Ctrl Pts',(85.4329129711515,38.9858770551906,120.572540304363));
#36681=CARTESIAN_POINT('Ctrl Pts',(88.5106434364707,39.9047355577889,120.42562447136));
#36682=CARTESIAN_POINT('Ctrl Pts',(91.146667598539,37.6740968914383,120.267675948167));
#36683=CARTESIAN_POINT('Ctrl Pts',(90.7198608027206,34.2474036567132,120.109727424975));
#36684=CARTESIAN_POINT('Ctrl Pts',(87.6171951050278,32.7315381211201,119.951778901782));
#36685=CARTESIAN_POINT('Ctrl Pts',(85.1057449826314,34.2300157885499,119.818010909183));
#36686=CARTESIAN_POINT('Ctrl Pts',(84.7008103145862,35.8037807016134,119.736892424315));
#36687=CARTESIAN_POINT('Ctrl Pts',(84.6997382737804,36.3555871001389,119.708423447177));
#36688=CARTESIAN_POINT('Ctrl Pts',(84.6981142843292,36.357076956871,120.791576552823));
#36689=CARTESIAN_POINT('Ctrl Pts',(84.6957789541399,36.7130204125928,120.773188306702));
#36690=CARTESIAN_POINT('Ctrl Pts',(84.9168437417748,38.0853010552934,120.70215055285));
#36691=CARTESIAN_POINT('Ctrl Pts',(86.9355578127517,39.8844990120122,120.578463291268));
#36692=CARTESIAN_POINT('Ctrl Pts',(90.2686753707106,38.9819491786592,120.420514768075));
#36693=CARTESIAN_POINT('Ctrl Pts',(91.3350260504491,35.6975416344974,120.262566244883));
#36694=CARTESIAN_POINT('Ctrl Pts',(89.1677588017562,33.0091722323982,120.10461772169));
#36695=CARTESIAN_POINT('Ctrl Pts',(85.7525883791808,33.3522123095062,119.94762115767));
#36696=CARTESIAN_POINT('Ctrl Pts',(84.6916123913094,35.361289961862,119.843274101381));
#36697=CARTESIAN_POINT('Ctrl Pts',(84.6900676527761,36.3552596744725,119.791576552823));
#36698=CARTESIAN_POINT('Origin',(87.7685555885722,36.3549260746835,124.208423447177));
#36699=CARTESIAN_POINT('',(84.6982769289314,36.3519105223041,121.791576552823));
#36700=CARTESIAN_POINT('',(84.6917558532639,36.3568536987801,121.708423447177));
#36701=CARTESIAN_POINT('',(84.6950555885722,36.3549260746838,124.208423447177));
#36702=CARTESIAN_POINT('',(86.9747563060389,33.385703120938,122.));
#36703=CARTESIAN_POINT('Ctrl Pts',(86.9747563060389,33.385703120938,122.));
#36704=CARTESIAN_POINT('Ctrl Pts',(85.9925177162673,33.6482971733158,121.947350492269));
#36705=CARTESIAN_POINT('Ctrl Pts',(84.8928209565869,34.686033271266,121.877876009877));
#36706=CARTESIAN_POINT('Ctrl Pts',(84.6959357391912,36.0264346664739,121.808401527484));
#36707=CARTESIAN_POINT('Ctrl Pts',(84.6982769289315,36.3519105223041,121.791576552823));
#36708=CARTESIAN_POINT('',(88.5642644266099,33.3806265661435,122.));
#36709=CARTESIAN_POINT('Origin',(87.7685555885722,36.3549260746835,122.));
#36710=CARTESIAN_POINT('Ctrl Pts',(88.5642690620867,33.3806142427251,122.));
#36711=CARTESIAN_POINT('Ctrl Pts',(87.6173029036983,33.1297337676241,121.949053726697));
#36712=CARTESIAN_POINT('Ctrl Pts',(85.556753483317,33.5846352576989,121.851861542423));
#36713=CARTESIAN_POINT('Ctrl Pts',(84.6984192980838,35.4665788853084,121.754669358149));
#36714=CARTESIAN_POINT('Ctrl Pts',(84.6917558532639,36.3568536987801,121.708423447177));
#36715=CARTESIAN_POINT('Origin',(-36.3549260746835,-87.7685555885722,114.));
#36716=CARTESIAN_POINT('',(-38.8684363400902,-87.7682981264136,107.387416697508));
#36717=CARTESIAN_POINT('',(-38.8705162236156,-87.7721288317432,107.112583302492));
#36718=CARTESIAN_POINT('',(-38.8724260746835,-87.7685555885722,114.));
#36719=CARTESIAN_POINT('',(-38.2683920713482,-86.1325683851969,107.));
#36720=CARTESIAN_POINT('Ctrl Pts',(-38.8705162236156,-87.7721288317432,
107.112583302492));
#36721=CARTESIAN_POINT('Ctrl Pts',(-38.8653710199197,-87.1794939521863,
107.075055534995));
#36722=CARTESIAN_POINT('Ctrl Pts',(-38.6541479027674,-86.5837520282675,
107.037527767497));
#36723=CARTESIAN_POINT('Ctrl Pts',(-38.2683920713482,-86.1325683851969,
107.));
#36724=CARTESIAN_POINT('',(-38.8724260746835,-87.7685555885722,107.));
#36725=CARTESIAN_POINT('Origin',(-36.3549260746835,-87.7685555885722,107.));
#36726=CARTESIAN_POINT('',(-38.8724260746835,-87.7685555885722,106.));
#36727=CARTESIAN_POINT('',(-38.8724260746835,-87.7685555885722,114.));
#36728=CARTESIAN_POINT('Origin',(-36.3549260746835,-87.7685555885722,106.));
#36729=CARTESIAN_POINT('',(-34.4378158180085,-86.1300276446784,107.));
#36730=CARTESIAN_POINT('Origin',(-36.3549260746835,-87.7685555885722,107.));
#36731=CARTESIAN_POINT('Ctrl Pts',(-34.4378069719681,-86.1300214773102,
107.));
#36732=CARTESIAN_POINT('Ctrl Pts',(-34.9606275290818,-85.5213064137174,
107.050946273303));
#36733=CARTESIAN_POINT('Ctrl Pts',(-35.8003520377837,-85.1811300520207,
107.101892546605));
#36734=CARTESIAN_POINT('Ctrl Pts',(-36.5990228985553,-85.2588928357685,
107.152838819908));
#36735=CARTESIAN_POINT('Ctrl Pts',(-37.4243949018965,-85.3392553827949,
107.205488327639));
#36736=CARTESIAN_POINT('Ctrl Pts',(-38.2059223628864,-85.865969264881,107.25813783537));
#36737=CARTESIAN_POINT('Ctrl Pts',(-38.589806978663,-86.6007560325992,107.3107873431));
#36738=CARTESIAN_POINT('Ctrl Pts',(-38.7760501272496,-86.9572407562258,
107.336330461236));
#36739=CARTESIAN_POINT('Ctrl Pts',(-38.8686983365902,-87.3627005068745,
107.361873579372));
#36740=CARTESIAN_POINT('Ctrl Pts',(-38.8684363400902,-87.7682981264136,
107.387416697508));
#36741=CARTESIAN_POINT('Origin',(-36.3549260746835,-87.7685555885722,114.));
#36742=CARTESIAN_POINT('',(-38.8737308567828,-87.7706510706098,108.387416697508));
#36743=CARTESIAN_POINT('',(-38.8763331790899,-87.7678892788988,108.112583302492));
#36744=CARTESIAN_POINT('',(-38.8724260746835,-87.7685555885722,114.));
#36745=CARTESIAN_POINT('Ctrl Pts',(-38.8763331790899,-87.7678892788988,
108.112583302492));
#36746=CARTESIAN_POINT('Ctrl Pts',(-38.8764610150598,-87.7314321411263,
108.110268755777));
#36747=CARTESIAN_POINT('Ctrl Pts',(-38.8757380641522,-87.6949802400596,
108.107954209062));
#36748=CARTESIAN_POINT('Ctrl Pts',(-38.8741484476744,-87.6585662372005,
108.105639662347));
#36749=CARTESIAN_POINT('Ctrl Pts',(-38.8379890889129,-86.8302488337614,
108.052990154616));
#36750=CARTESIAN_POINT('Ctrl Pts',(-38.3533856737909,-86.021541331288,108.000340646886));
#36751=CARTESIAN_POINT('Ctrl Pts',(-37.6400112436482,-85.5989796556856,
107.947691139155));
#36752=CARTESIAN_POINT('Ctrl Pts',(-36.9266368135056,-85.1764179800833,
107.895041631424));
#36753=CARTESIAN_POINT('Ctrl Pts',(-35.9844913683424,-85.140002131352,107.842392123693));
#36754=CARTESIAN_POINT('Ctrl Pts',(-35.2407121334911,-85.5064038253269,
107.789742615962));
#36755=CARTESIAN_POINT('Ctrl Pts',(-34.4969328986398,-85.8728055193019,
107.737093108232));
#36756=CARTESIAN_POINT('Ctrl Pts',(-33.9515198741004,-86.6420247559832,
107.684443600501));
#36757=CARTESIAN_POINT('Ctrl Pts',(-33.8516662037545,-87.465012158015,107.63179409277));
#36758=CARTESIAN_POINT('Ctrl Pts',(-33.7518125334087,-88.2879995600469,
107.579144585039));
#36759=CARTESIAN_POINT('Ctrl Pts',(-34.0975182172564,-89.1647551274293,
107.526495077308));
#36760=CARTESIAN_POINT('Ctrl Pts',(-34.7321882273048,-89.6985070179526,
107.473845569577));
#36761=CARTESIAN_POINT('Ctrl Pts',(-35.3668582373533,-90.232258908476,107.421196061847));
#36762=CARTESIAN_POINT('Ctrl Pts',(-36.2904925736025,-90.4230071221403,
107.368546554116));
#36763=CARTESIAN_POINT('Ctrl Pts',(-37.0841095226148,-90.1828532548222,
107.315897046385));
#36764=CARTESIAN_POINT('Ctrl Pts',(-37.8777264716271,-89.9426993875041,
107.263247538654));
#36765=CARTESIAN_POINT('Ctrl Pts',(-38.5413260334026,-89.2716434392036,
107.210598030923));
#36766=CARTESIAN_POINT('Ctrl Pts',(-38.7742912799133,-88.4773574901821,
107.157948523192));
#36767=CARTESIAN_POINT('Ctrl Pts',(-38.8412024457151,-88.249226472251,107.142826782959));
#36768=CARTESIAN_POINT('Ctrl Pts',(-38.8725894733431,-88.0109298929199,
107.127705042726));
#36769=CARTESIAN_POINT('Ctrl Pts',(-38.8705162236156,-87.7721288317432,
107.112583302492));
#36770=CARTESIAN_POINT('Ctrl Pts',(-38.8684363400902,-87.7682981264136,
107.387416697508));
#36771=CARTESIAN_POINT('Ctrl Pts',(-38.8681583090697,-88.1987188383852,
107.414523087103));
#36772=CARTESIAN_POINT('Ctrl Pts',(-38.7632496215152,-88.6292948111527,
107.441629476698));
#36773=CARTESIAN_POINT('Ctrl Pts',(-38.5545285816793,-89.0016622291512,
107.468735866293));
#36774=CARTESIAN_POINT('Ctrl Pts',(-38.1491237983557,-89.7249220046346,
107.521385374024));
#36775=CARTESIAN_POINT('Ctrl Pts',(-37.3520724611453,-90.2285819022512,
107.574034881755));
#36776=CARTESIAN_POINT('Ctrl Pts',(-36.5248227413449,-90.2844328864611,
107.626684389485));
#36777=CARTESIAN_POINT('Ctrl Pts',(-35.6975730215444,-90.3402838706711,
107.679333897216));
#36778=CARTESIAN_POINT('Ctrl Pts',(-34.8401249191538,-89.9483259414745,
107.731983404947));
#36779=CARTESIAN_POINT('Ctrl Pts',(-34.3411325694982,-89.2861901269712,
107.784632912678));
#36780=CARTESIAN_POINT('Ctrl Pts',(-33.8421402198425,-88.624054312468,107.837282420409));
#36781=CARTESIAN_POINT('Ctrl Pts',(-33.7016036229218,-87.6917406126582,
107.889931928139));
#36782=CARTESIAN_POINT('Ctrl Pts',(-33.9832605857992,-86.9119270488255,
107.94258143587));
#36783=CARTESIAN_POINT('Ctrl Pts',(-34.2649175486767,-86.1321134849928,
107.995230943601));
#36784=CARTESIAN_POINT('Ctrl Pts',(-34.9687680713523,-85.5048000571372,
108.047880451332));
#36785=CARTESIAN_POINT('Ctrl Pts',(-35.7757187646338,-85.3143562592227,
108.100529959063));
#36786=CARTESIAN_POINT('Ctrl Pts',(-36.5826694579152,-85.1239124613082,
108.153179466794));
#36787=CARTESIAN_POINT('Ctrl Pts',(-37.4927203218023,-85.3703382933347,
108.205828974524));
#36788=CARTESIAN_POINT('Ctrl Pts',(-38.093320179937,-85.9419269203423,108.258478482255));
#36789=CARTESIAN_POINT('Ctrl Pts',(-38.583608232169,-86.4085322163941,108.30145788734));
#36790=CARTESIAN_POINT('Ctrl Pts',(-38.8676794726009,-87.0918245926314,
108.344437292424));
#36791=CARTESIAN_POINT('Ctrl Pts',(-38.8737308567828,-87.7706510706098,
108.387416697508));
#36792=CARTESIAN_POINT('Origin',(-36.3549260746835,-87.7685555885722,114.));
#36793=CARTESIAN_POINT('',(-38.8745810387237,-87.7666978306399,109.387416697508));
#36794=CARTESIAN_POINT('',(-38.8694869524425,-87.7670276463177,109.112583302492));
#36795=CARTESIAN_POINT('',(-38.8724260746835,-87.7685555885722,114.));
#36796=CARTESIAN_POINT('Ctrl Pts',(-38.8694869524425,-87.7670276463177,
109.112583302492));
#36797=CARTESIAN_POINT('Ctrl Pts',(-38.8712432078539,-87.4537363139361,
109.092832468829));
#36798=CARTESIAN_POINT('Ctrl Pts',(-38.8169460127038,-87.1410318012893,
109.073081635165));
#36799=CARTESIAN_POINT('Ctrl Pts',(-38.7038064348735,-86.8513056056821,
109.053330801502));
#36800=CARTESIAN_POINT('Ctrl Pts',(-38.402211920982,-86.0789867337058,109.000681293771));
#36801=CARTESIAN_POINT('Ctrl Pts',(-37.6824905952959,-85.4699489867722,
108.94803178604));
#36802=CARTESIAN_POINT('Ctrl Pts',(-36.8709169839095,-85.3002893177264,
108.89538227831));
#36803=CARTESIAN_POINT('Ctrl Pts',(-36.0593433725232,-85.1306296486805,
108.842732770579));
#36804=CARTESIAN_POINT('Ctrl Pts',(-35.1559174754367,-85.4003480575224,
108.790083262848));
#36805=CARTESIAN_POINT('Ctrl Pts',(-34.5701940802303,-85.9871739609405,
108.737433755117));
#36806=CARTESIAN_POINT('Ctrl Pts',(-33.984470685024,-86.5739998643585,108.684784247386));
#36807=CARTESIAN_POINT('Ctrl Pts',(-33.716449791698,-87.4779332623528,108.632134739655));
#36808=CARTESIAN_POINT('Ctrl Pts',(-33.8876337833753,-88.2891852612251,
108.579485231925));
#36809=CARTESIAN_POINT('Ctrl Pts',(-34.0588177750527,-89.1004372600974,
108.526835724194));
#36810=CARTESIAN_POINT('Ctrl Pts',(-34.6692066517334,-89.8190078598478,
108.474186216463));
#36811=CARTESIAN_POINT('Ctrl Pts',(-35.4420915705444,-90.1191531246981,
108.421536708732));
#36812=CARTESIAN_POINT('Ctrl Pts',(-36.2149764893555,-90.4192983895484,
108.368887201001));
#36813=CARTESIAN_POINT('Ctrl Pts',(-37.1503574502968,-90.3010183194988,
108.316237693271));
#36814=CARTESIAN_POINT('Ctrl Pts',(-37.8241902795669,-89.8179146322715,
108.26358818554));
#36815=CARTESIAN_POINT('Ctrl Pts',(-38.4684004660316,-89.3560488654054,
108.213253224524));
#36816=CARTESIAN_POINT('Ctrl Pts',(-38.8735531018844,-88.5607307440123,
108.162918263508));
#36817=CARTESIAN_POINT('Ctrl Pts',(-38.8763331790899,-87.7678892788988,
108.112583302492));
#36818=CARTESIAN_POINT('Ctrl Pts',(-38.8737308567828,-87.7706510706098,
108.387416697508));
#36819=CARTESIAN_POINT('Ctrl Pts',(-38.875092381124,-87.9233828664173,108.397086800155));
#36820=CARTESIAN_POINT('Ctrl Pts',(-38.8623799172478,-88.0758885884459,
108.406756902801));
#36821=CARTESIAN_POINT('Ctrl Pts',(-38.8347756504559,-88.2256493719635,
108.416427005448));
#36822=CARTESIAN_POINT('Ctrl Pts',(-38.684482410458,-89.0410317745883,108.469076513179));
#36823=CARTESIAN_POINT('Ctrl Pts',(-38.0927470780801,-89.7750451578491,
108.521726020909));
#36824=CARTESIAN_POINT('Ctrl Pts',(-37.32782541498,-90.0949372694507,108.57437552864));
#36825=CARTESIAN_POINT('Ctrl Pts',(-36.5629037518798,-90.4148293810522,
108.627025036371));
#36826=CARTESIAN_POINT('Ctrl Pts',(-35.6247957580574,-90.3206002209945,
108.679674544102));
#36827=CARTESIAN_POINT('Ctrl Pts',(-34.938777674606,-89.8549663909368,108.732324051833));
#36828=CARTESIAN_POINT('Ctrl Pts',(-34.2527595911546,-89.3893325608792,
108.784973559563));
#36829=CARTESIAN_POINT('Ctrl Pts',(-33.8188314180741,-88.5522940608215,
108.837623067294));
#36830=CARTESIAN_POINT('Ctrl Pts',(-33.8337082597499,-87.7233099332487,
108.890272575025));
#36831=CARTESIAN_POINT('Ctrl Pts',(-33.8485851014256,-86.894325805676,108.942922082756));
#36832=CARTESIAN_POINT('Ctrl Pts',(-34.3122669578576,-86.0733960505882,
108.995571590487));
#36833=CARTESIAN_POINT('Ctrl Pts',(-35.0145505326977,-85.632676510197,109.048221098218));
#36834=CARTESIAN_POINT('Ctrl Pts',(-35.7168341075378,-85.1919569698057,
109.100870605948));
#36835=CARTESIAN_POINT('Ctrl Pts',(-36.6577194007862,-85.1314476441111,
109.153520113679));
#36836=CARTESIAN_POINT('Ctrl Pts',(-37.410670459096,-85.4785796025718,109.20616962141));
#36837=CARTESIAN_POINT('Ctrl Pts',(-38.1636215174058,-85.8257115610326,
109.258819129141));
#36838=CARTESIAN_POINT('Ctrl Pts',(-38.728638340777,-86.5804848036488,109.311468636872));
#36839=CARTESIAN_POINT('Ctrl Pts',(-38.8495791023889,-87.4007343163658,
109.364118144603));
#36840=CARTESIAN_POINT('Ctrl Pts',(-38.8674187420126,-87.521727069457,109.371884328904));
#36841=CARTESIAN_POINT('Ctrl Pts',(-38.8755960015225,-87.6441444807647,
109.379650513206));
#36842=CARTESIAN_POINT('Ctrl Pts',(-38.8745810387237,-87.7666978306399,
109.387416697508));
#36843=CARTESIAN_POINT('Origin',(-36.3549260746835,-87.7685555885722,114.));
#36844=CARTESIAN_POINT('',(-38.8685101472268,-87.7682702011617,110.387416697508));
#36845=CARTESIAN_POINT('',(-38.8710622858024,-87.7706792336182,110.112583302492));
#36846=CARTESIAN_POINT('',(-38.8724260746835,-87.7685555885722,114.));
#36847=CARTESIAN_POINT('Ctrl Pts',(-38.8710622858024,-87.7706792336182,
110.112583302492));
#36848=CARTESIAN_POINT('Ctrl Pts',(-38.8662628209879,-87.1817421481431,
110.07539618188));
#36849=CARTESIAN_POINT('Ctrl Pts',(-38.6597043123301,-86.5897714841231,
110.038209061269));
#36850=CARTESIAN_POINT('Ctrl Pts',(-38.2820087618755,-86.1422288485708,
110.001021940657));
#36851=CARTESIAN_POINT('Ctrl Pts',(-37.7472675806157,-85.5085981973457,
109.948372432926));
#36852=CARTESIAN_POINT('Ctrl Pts',(-36.8694842018095,-85.1644718390116,
109.895722925195));
#36853=CARTESIAN_POINT('Ctrl Pts',(-36.046588369411,-85.2658542112028,109.843073417464));
#36854=CARTESIAN_POINT('Ctrl Pts',(-35.2236925370125,-85.367236583394,109.790423909734));
#36855=CARTESIAN_POINT('Ctrl Pts',(-34.4556842510217,-85.9141276861104,
109.737774402003));
#36856=CARTESIAN_POINT('Ctrl Pts',(-34.090728394159,-86.6586027828937,109.685124894272));
#36857=CARTESIAN_POINT('Ctrl Pts',(-33.7257725372963,-87.403077879677,109.632475386541));
#36858=CARTESIAN_POINT('Ctrl Pts',(-33.7638691095618,-88.345136970527,109.57982587881));
#36859=CARTESIAN_POINT('Ctrl Pts',(-34.1877475985013,-89.0577118337345,
109.527176371079));
#36860=CARTESIAN_POINT('Ctrl Pts',(-34.6116260874407,-89.770286696942,109.474526863349));
#36861=CARTESIAN_POINT('Ctrl Pts',(-35.4212864930542,-90.2533773325069,
109.421877355618));
#36862=CARTESIAN_POINT('Ctrl Pts',(-36.2496816049095,-90.2879820675602,
109.369227847887));
#36863=CARTESIAN_POINT('Ctrl Pts',(-37.0780767167647,-90.3225868026134,
109.316578340156));
#36864=CARTESIAN_POINT('Ctrl Pts',(-37.9252065348617,-89.908705637155,109.263928832425));
#36865=CARTESIAN_POINT('Ctrl Pts',(-38.4070375928618,-89.2339650559163,
109.211279324695));
#36866=CARTESIAN_POINT('Ctrl Pts',(-38.708115487337,-88.8123453405756,109.178380650627));
#36867=CARTESIAN_POINT('Ctrl Pts',(-38.8665615835522,-88.2888724255255,
109.145481976559));
#36868=CARTESIAN_POINT('Ctrl Pts',(-38.8694869524425,-87.7670276463177,
109.112583302492));
#36869=CARTESIAN_POINT('Ctrl Pts',(-38.8745810387237,-87.7666978306399,
109.387416697508));
#36870=CARTESIAN_POINT('Ctrl Pts',(-38.8687152361884,-88.4749737903615,
109.432300020937));
#36871=CARTESIAN_POINT('Ctrl Pts',(-38.5558234383421,-89.1877901835691,
109.477183344366));
#36872=CARTESIAN_POINT('Ctrl Pts',(-38.0266616968572,-89.6563813707687,
109.522066667795));
#36873=CARTESIAN_POINT('Ctrl Pts',(-37.4059388298609,-90.2060531296368,
109.574716175526));
#36874=CARTESIAN_POINT('Ctrl Pts',(-36.4876283960155,-90.4196708645552,
109.627365683257));
#36875=CARTESIAN_POINT('Ctrl Pts',(-35.6880324559884,-90.200394213864,109.680015190987));
#36876=CARTESIAN_POINT('Ctrl Pts',(-34.8884365159614,-89.9811175631728,
109.732664698718));
#36877=CARTESIAN_POINT('Ctrl Pts',(-34.2075550697527,-89.3289465268721,
109.785314206449));
#36878=CARTESIAN_POINT('Ctrl Pts',(-33.9540553717985,-88.5395329316783,
109.83796371418));
#36879=CARTESIAN_POINT('Ctrl Pts',(-33.7005556738443,-87.7501193364846,
109.890613221911));
#36880=CARTESIAN_POINT('Ctrl Pts',(-33.8744377241447,-86.8234631823979,
109.943262729642));
#36881=CARTESIAN_POINT('Ctrl Pts',(-34.3968747370372,-86.1796499430275,
109.995912237372));
#36882=CARTESIAN_POINT('Ctrl Pts',(-34.9193117499297,-85.5358367036571,
110.048561745103));
#36883=CARTESIAN_POINT('Ctrl Pts',(-35.7903037254143,-85.1748663790032,
110.101211252834));
#36884=CARTESIAN_POINT('Ctrl Pts',(-36.6149996975598,-85.2603793776866,
110.153860760565));
#36885=CARTESIAN_POINT('Ctrl Pts',(-37.4396956697052,-85.34589237637,110.206510268296));
#36886=CARTESIAN_POINT('Ctrl Pts',(-38.2180956385115,-85.8778886983908,
110.259159776027));
#36887=CARTESIAN_POINT('Ctrl Pts',(-38.597323814547,-86.6151959005714,110.311809283757));
#36888=CARTESIAN_POINT('Ctrl Pts',(-38.7788542336475,-86.9681329813994,
110.337011755008));
#36889=CARTESIAN_POINT('Ctrl Pts',(-38.8689191194958,-87.3681146417202,
110.362214226258));
#36890=CARTESIAN_POINT('Ctrl Pts',(-38.8685101472268,-87.7682702011617,
110.387416697508));
#36891=CARTESIAN_POINT('Origin',(-36.3549260746835,-87.7685555885722,114.));
#36892=CARTESIAN_POINT('',(-38.8735728336891,-87.7706817999035,111.387416697508));
#36893=CARTESIAN_POINT('',(-38.8763919803986,-87.7679946640762,111.112583302492));
#36894=CARTESIAN_POINT('',(-38.8724260746835,-87.7685555885722,114.));
#36895=CARTESIAN_POINT('Ctrl Pts',(-38.8763919803986,-87.7679946640762,
111.112583302492));
#36896=CARTESIAN_POINT('Ctrl Pts',(-38.8764867042391,-87.7369047139068,
111.110609402663));
#36897=CARTESIAN_POINT('Ctrl Pts',(-38.875960902618,-87.7058180412501,111.108635502833));
#36898=CARTESIAN_POINT('Ctrl Pts',(-38.8748045962056,-87.6747548387019,
111.106661603004));
#36899=CARTESIAN_POINT('Ctrl Pts',(-38.8439626241377,-86.8462111109777,
111.054012095273));
#36900=CARTESIAN_POINT('Ctrl Pts',(-38.3645541874353,-86.034364962245,111.001362587542));
#36901=CARTESIAN_POINT('Ctrl Pts',(-37.6539118106195,-85.6072544985287,
110.948713079812));
#36902=CARTESIAN_POINT('Ctrl Pts',(-36.9432694338037,-85.1801440348125,
110.896063572081));
#36903=CARTESIAN_POINT('Ctrl Pts',(-36.0013931168745,-85.1377692561125,
110.84341406435));
#36904=CARTESIAN_POINT('Ctrl Pts',(-35.2552681651416,-85.499340123784,110.790764556619));
#36905=CARTESIAN_POINT('Ctrl Pts',(-34.5091432134086,-85.8609109914556,
110.738115048888));
#36906=CARTESIAN_POINT('Ctrl Pts',(-33.9587696268719,-86.6264275054988,
110.685465541158));
#36907=CARTESIAN_POINT('Ctrl Pts',(-33.8536509016289,-87.4488543957147,
110.632816033427));
#36908=CARTESIAN_POINT('Ctrl Pts',(-33.7485321763859,-88.2712812859306,
110.580166525696));
#36909=CARTESIAN_POINT('Ctrl Pts',(-34.0886683124366,-89.1506185523193,
110.527517017965));
#36910=CARTESIAN_POINT('Ctrl Pts',(-34.719863764747,-89.6882320163061,110.474867510234));
#36911=CARTESIAN_POINT('Ctrl Pts',(-35.3510592170573,-90.225845480293,110.422218002503));
#36912=CARTESIAN_POINT('Ctrl Pts',(-36.2733139856272,-90.4217351418781,
110.369568494773));
#36913=CARTESIAN_POINT('Ctrl Pts',(-37.068537895973,-90.1870974034315,110.316918987042));
#36914=CARTESIAN_POINT('Ctrl Pts',(-37.8637618063188,-89.9524596649849,
110.264269479311));
#36915=CARTESIAN_POINT('Ctrl Pts',(-38.5319548584405,-89.2872945265066,
110.21161997158));
#36916=CARTESIAN_POINT('Ctrl Pts',(-38.7702018926446,-88.4931444852094,
110.158970463849));
#36917=CARTESIAN_POINT('Ctrl Pts',(-38.8401715472838,-88.2599142823368,
110.14350807673));
#36918=CARTESIAN_POINT('Ctrl Pts',(-38.8730579009968,-88.0155589945307,
110.128045689611));
#36919=CARTESIAN_POINT('Ctrl Pts',(-38.8710622858024,-87.7706792336182,
110.112583302492));
#36920=CARTESIAN_POINT('Ctrl Pts',(-38.8685101472268,-87.7682702011617,
110.387416697508));
#36921=CARTESIAN_POINT('Ctrl Pts',(-38.8680647513497,-88.2040641409246,
110.414863733989));
#36922=CARTESIAN_POINT('Ctrl Pts',(-38.7603124245963,-88.6400643345304,
110.442310770469));
#36923=CARTESIAN_POINT('Ctrl Pts',(-38.5465340999794,-89.0157285744514,
110.46975780695));
#36924=CARTESIAN_POINT('Ctrl Pts',(-38.1364598261117,-89.7363359638104,
110.522407314681));
#36925=CARTESIAN_POINT('Ctrl Pts',(-37.3362548951114,-90.2349326601879,
110.575056822411));
#36926=CARTESIAN_POINT('Ctrl Pts',(-36.5086800437499,-90.2854874332158,
110.627706330142));
#36927=CARTESIAN_POINT('Ctrl Pts',(-35.6811051923884,-90.3360422062437,
110.680355837873));
#36928=CARTESIAN_POINT('Ctrl Pts',(-34.8261604206655,-89.9385550559221,
110.733005345604));
#36929=CARTESIAN_POINT('Ctrl Pts',(-34.3314219399208,-89.2732207374008,
110.785654853335));
#36930=CARTESIAN_POINT('Ctrl Pts',(-33.8366834591761,-88.6078864188794,
110.838304361066));
#36931=CARTESIAN_POINT('Ctrl Pts',(-33.7021512694097,-87.6747049321583,
110.890953868796));
#36932=CARTESIAN_POINT('Ctrl Pts',(-33.9888134930152,-86.8967199134953,
110.943603376527));
#36933=CARTESIAN_POINT('Ctrl Pts',(-34.2754757166207,-86.1187348948324,
110.996252884258));
#36934=CARTESIAN_POINT('Ctrl Pts',(-34.9833323535982,-85.4959463442275,
111.048902391989));
#36935=CARTESIAN_POINT('Ctrl Pts',(-35.7914873618322,-85.3106859804839,
111.10155189972));
#36936=CARTESIAN_POINT('Ctrl Pts',(-36.5996423700663,-85.1254256167402,
111.154201407451));
#36937=CARTESIAN_POINT('Ctrl Pts',(-37.5080957495568,-85.3776934398577,
111.206850915181));
#36938=CARTESIAN_POINT('Ctrl Pts',(-38.1050139753849,-85.9531276684082,
111.259500422912));
#36939=CARTESIAN_POINT('Ctrl Pts',(-38.5884344857069,-86.4191491373235,
111.302139181111));
#36940=CARTESIAN_POINT('Ctrl Pts',(-38.8675271646894,-87.0971270740966,
111.344777939309));
#36941=CARTESIAN_POINT('Ctrl Pts',(-38.8735728336891,-87.7706817999035,
111.387416697508));
#36942=CARTESIAN_POINT('Origin',(-36.3549260746835,-87.7685555885722,114.));
#36943=CARTESIAN_POINT('',(-38.8747250213613,-87.7667516914454,112.387416697508));
#36944=CARTESIAN_POINT('',(-38.869589870133,-87.7669648532936,112.112583302492));
#36945=CARTESIAN_POINT('',(-38.8724260746835,-87.7685555885722,114.));
#36946=CARTESIAN_POINT('Ctrl Pts',(-38.869589870133,-87.7669648532936,112.112583302492));
#36947=CARTESIAN_POINT('Ctrl Pts',(-38.8713916229222,-87.4591086153934,
112.093173115714));
#36948=CARTESIAN_POINT('Ctrl Pts',(-38.8190054048914,-87.1518441591964,
112.073762928937));
#36949=CARTESIAN_POINT('Ctrl Pts',(-38.7096476981112,-86.866406809236,112.054352742159));
#36950=CARTESIAN_POINT('Ctrl Pts',(-38.4130184335659,-86.0921671723103,
112.001703234428));
#36951=CARTESIAN_POINT('Ctrl Pts',(-37.6972224731726,-85.4785200738972,
111.949053726697));
#36952=CARTESIAN_POINT('Ctrl Pts',(-36.8867550306008,-85.3036530944469,
111.896404218966));
#36953=CARTESIAN_POINT('Ctrl Pts',(-36.076287588029,-85.1287861149966,111.843754711236));
#36954=CARTESIAN_POINT('Ctrl Pts',(-35.1711486632787,-85.3926992545092,
111.791105203505));
#36955=CARTESIAN_POINT('Ctrl Pts',(-34.5816692236069,-85.9757515044618,
111.738455695774));
#36956=CARTESIAN_POINT('Ctrl Pts',(-33.9921897839352,-86.5588037544144,
111.685806188043));
#36957=CARTESIAN_POINT('Ctrl Pts',(-33.7183698293421,-87.4609951148072,
111.633156680312));
#36958=CARTESIAN_POINT('Ctrl Pts',(-33.8843414723145,-88.2733308518658,
111.580507172582));
#36959=CARTESIAN_POINT('Ctrl Pts',(-34.050313115287,-89.0856665889245,111.527857664851));
#36960=CARTESIAN_POINT('Ctrl Pts',(-34.656076355825,-89.808146702649,111.47520815712));
#36961=CARTESIAN_POINT('Ctrl Pts',(-35.4270176405568,-90.113245820092,111.422558649389));
#36962=CARTESIAN_POINT('Ctrl Pts',(-36.1979589252887,-90.418344937535,111.369909141658));
#36963=CARTESIAN_POINT('Ctrl Pts',(-37.1340782542145,-90.3060630586964,
111.317259633927));
#36964=CARTESIAN_POINT('Ctrl Pts',(-37.8110001649606,-89.8273014659192,
111.264610126197));
#36965=CARTESIAN_POINT('Ctrl Pts',(-38.4625433760447,-89.3664892798312,
111.213934518295));
#36966=CARTESIAN_POINT('Ctrl Pts',(-38.8739601507151,-88.5661618765622,
111.163258910394));
#36967=CARTESIAN_POINT('Ctrl Pts',(-38.8763919803986,-87.7679946640762,
111.112583302492));
#36968=CARTESIAN_POINT('Ctrl Pts',(-38.8735728336891,-87.7706817999035,
111.387416697508));
#36969=CARTESIAN_POINT('Ctrl Pts',(-38.8749922389595,-87.9288193240984,
111.39742744704));
#36970=CARTESIAN_POINT('Ctrl Pts',(-38.8613607771502,-88.0867130325477,
111.407438196572));
#36971=CARTESIAN_POINT('Ctrl Pts',(-38.8317891158855,-88.2415626377976,
111.417448946105));
#36972=CARTESIAN_POINT('Ctrl Pts',(-38.6762629583927,-89.0559627446527,
111.470098453835));
#36973=CARTESIAN_POINT('Ctrl Pts',(-38.0798275712416,-89.7861623243795,
111.522747961566));
#36974=CARTESIAN_POINT('Ctrl Pts',(-37.3128678673142,-90.1011365015151,
111.575397469297));
#36975=CARTESIAN_POINT('Ctrl Pts',(-36.5459081633868,-90.4161106786507,
111.628046977028));
#36976=CARTESIAN_POINT('Ctrl Pts',(-35.6084241426832,-90.3158594531952,
111.680696484759));
#36977=CARTESIAN_POINT('Ctrl Pts',(-34.9254099298464,-89.8458301937081,
111.733345992489));
#36978=CARTESIAN_POINT('Ctrl Pts',(-34.2423957170096,-89.3758009342209,
111.78599550022));
#36979=CARTESIAN_POINT('Ctrl Pts',(-33.8138513120396,-88.5359936407022,
111.838645007951));
#36980=CARTESIAN_POINT('Ctrl Pts',(-33.8340508041346,-87.7071221788761,
111.891294515682));
#36981=CARTESIAN_POINT('Ctrl Pts',(-33.8542502962297,-86.8782507170499,
111.943944023413));
#36982=CARTESIAN_POINT('Ctrl Pts',(-34.3231936853898,-86.0603150869163,
111.996593531144));
#36983=CARTESIAN_POINT('Ctrl Pts',(-35.0282926172737,-85.6241139682027,
112.049243038875));
#36984=CARTESIAN_POINT('Ctrl Pts',(-35.7333915491576,-85.1879128494891,
112.101892546605));
#36985=CARTESIAN_POINT('Ctrl Pts',(-36.6746460237652,-85.1334462421954,
112.154542054336));
#36986=CARTESIAN_POINT('Ctrl Pts',(-37.4253526385136,-85.4854057544748,
112.207191562067));
#36987=CARTESIAN_POINT('Ctrl Pts',(-38.1760592532619,-85.8373652667541,
112.259841069798));
#36988=CARTESIAN_POINT('Ctrl Pts',(-38.736218008151,-86.5957508986065,112.312490577529));
#36989=CARTESIAN_POINT('Ctrl Pts',(-38.851889449881,-87.4167600564597,112.365140085259));
#36990=CARTESIAN_POINT('Ctrl Pts',(-38.8682034223296,-87.5325528621941,
112.372565622676));
#36991=CARTESIAN_POINT('Ctrl Pts',(-38.8756758831734,-87.649591342699,112.379991160092));
#36992=CARTESIAN_POINT('Ctrl Pts',(-38.8747250213613,-87.7667516914454,
112.387416697508));
#36993=CARTESIAN_POINT('Origin',(-36.3549260746835,-87.7685555885722,114.));
#36994=CARTESIAN_POINT('',(-38.8685313431306,-87.768184262399,113.387416697508));
#36995=CARTESIAN_POINT('',(-38.8709180488009,-87.7706492052449,113.112583302492));
#36996=CARTESIAN_POINT('',(-38.8724260746835,-87.7685555885722,114.));
#36997=CARTESIAN_POINT('Ctrl Pts',(-38.8709180488009,-87.7706492052449,
113.112583302492));
#36998=CARTESIAN_POINT('Ctrl Pts',(-38.8662499617323,-87.1870221755863,
113.075736828766));
#36999=CARTESIAN_POINT('Ctrl Pts',(-38.6637923444195,-86.6004729887904,
113.03889035504));
#37000=CARTESIAN_POINT('Ctrl Pts',(-38.2924116771201,-86.1546361716722,
113.002043881314));
#37001=CARTESIAN_POINT('Ctrl Pts',(-37.7617500605046,-85.5175850084034,
112.949394373583));
#37002=CARTESIAN_POINT('Ctrl Pts',(-36.8861944104941,-85.1678294908771,
112.896744865852));
#37003=CARTESIAN_POINT('Ctrl Pts',(-36.0626645666103,-85.2639259642975,
112.844095358121));
#37004=CARTESIAN_POINT('Ctrl Pts',(-35.2391347227264,-85.3600224377178,
112.791445850391));
#37005=CARTESIAN_POINT('Ctrl Pts',(-34.4676306849692,-85.9019709020846,
112.73879634266));
#37006=CARTESIAN_POINT('Ctrl Pts',(-34.0979020767385,-86.644087262386,112.686146834929));
#37007=CARTESIAN_POINT('Ctrl Pts',(-33.7281734685077,-87.3862036226874,
112.633497327198));
#37008=CARTESIAN_POINT('Ctrl Pts',(-33.7602202898036,-88.3284878789233,
112.580847819467));
#37009=CARTESIAN_POINT('Ctrl Pts',(-34.1795146015215,-89.0437697926693,
112.528198311736));
#37010=CARTESIAN_POINT('Ctrl Pts',(-34.5988089132394,-89.7590517064154,
112.475548804006));
#37011=CARTESIAN_POINT('Ctrl Pts',(-35.4053507153794,-90.2473312776716,
112.422899296275));
#37012=CARTESIAN_POINT('Ctrl Pts',(-36.2335065468714,-90.2872543879847,
112.370249788544));
#37013=CARTESIAN_POINT('Ctrl Pts',(-37.0616623783633,-90.3271774982979,
112.317600280813));
#37014=CARTESIAN_POINT('Ctrl Pts',(-37.9114322392072,-89.918744147668,112.264950773082));
#37015=CARTESIAN_POINT('Ctrl Pts',(-38.3975858852805,-89.2471113846339,
112.212301265351));
#37016=CARTESIAN_POINT('Ctrl Pts',(-38.7045102568622,-88.8230881043542,
112.179061944398));
#37017=CARTESIAN_POINT('Ctrl Pts',(-38.8665044263955,-88.294158765243,112.145822623445));
#37018=CARTESIAN_POINT('Ctrl Pts',(-38.869589870133,-87.7669648532936,112.112583302492));
#37019=CARTESIAN_POINT('Ctrl Pts',(-38.8747250213613,-87.7667516914454,
112.387416697508));
#37020=CARTESIAN_POINT('Ctrl Pts',(-38.8689339595225,-88.4802968312487,
112.432640667823));
#37021=CARTESIAN_POINT('Ctrl Pts',(-38.5507040482079,-89.1983623218322,
112.477864638137));
#37022=CARTESIAN_POINT('Ctrl Pts',(-38.0145055106651,-89.6670766680336,
112.523088608452));
#37023=CARTESIAN_POINT('Ctrl Pts',(-37.3902660011481,-90.2127514379001,
112.575738116183));
#37024=CARTESIAN_POINT('Ctrl Pts',(-36.4706028535431,-90.4204682937787,
112.628387623914));
#37025=CARTESIAN_POINT('Ctrl Pts',(-35.6724313706716,-90.1960619577684,
112.681037131644));
#37026=CARTESIAN_POINT('Ctrl Pts',(-34.8742598878001,-89.971655621758,112.733686639375));
#37027=CARTESIAN_POINT('Ctrl Pts',(-34.1975800696622,-89.3151260938587,
112.786336147106));
#37028=CARTESIAN_POINT('Ctrl Pts',(-33.9491544216676,-88.5241010518219,
112.838985654837));
#37029=CARTESIAN_POINT('Ctrl Pts',(-33.7007287736729,-87.7330760097852,
112.891635162568));
#37030=CARTESIAN_POINT('Ctrl Pts',(-33.8805572958214,-86.8075554536111,
112.944284670298));
#37031=CARTESIAN_POINT('Ctrl Pts',(-34.4071174622157,-86.1671100532235,
112.996934178029));
#37032=CARTESIAN_POINT('Ctrl Pts',(-34.9336776286101,-85.5266646528359,
113.04958368576));
#37033=CARTESIAN_POINT('Ctrl Pts',(-35.8069694392502,-85.1712944082348,
113.102233193491));
#37034=CARTESIAN_POINT('Ctrl Pts',(-36.6310993317674,-85.2621010157615,
113.154882701222));
#37035=CARTESIAN_POINT('Ctrl Pts',(-37.4552292242845,-85.3529076232882,
113.207532208953));
#37036=CARTESIAN_POINT('Ctrl Pts',(-38.2301971986787,-85.8898910829425,
113.260181716683));
#37037=CARTESIAN_POINT('Ctrl Pts',(-38.604683308551,-86.6296181090971,113.312831224414));
#37038=CARTESIAN_POINT('Ctrl Pts',(-38.7815208193256,-86.9789274226054,
113.337693048779));
#37039=CARTESIAN_POINT('Ctrl Pts',(-38.8690565301526,-87.3734456881792,
113.362554873143));
#37040=CARTESIAN_POINT('Ctrl Pts',(-38.8685313431306,-87.768184262399,113.387416697508));
#37041=CARTESIAN_POINT('Origin',(-36.3549260746835,-87.7685555885722,114.));
#37042=CARTESIAN_POINT('',(-38.8734137783908,-87.7707089500124,114.387416697508));
#37043=CARTESIAN_POINT('',(-38.8764405008163,-87.7680895936699,114.112583302492));
#37044=CARTESIAN_POINT('',(-38.8724260746835,-87.7685555885722,114.));
#37045=CARTESIAN_POINT('Ctrl Pts',(-38.8764405008163,-87.7680895936699,
114.112583302492));
#37046=CARTESIAN_POINT('Ctrl Pts',(-38.8765065883869,-87.7423663370125,
114.110950049548));
#37047=CARTESIAN_POINT('Ctrl Pts',(-38.8761466448638,-87.7166449745044,
114.109316796605));
#37048=CARTESIAN_POINT('Ctrl Pts',(-38.8753549438192,-87.6909369083243,
114.107683543661));
#37049=CARTESIAN_POINT('Ctrl Pts',(-38.8498336855031,-86.8622122246415,
114.05503403593));
#37050=CARTESIAN_POINT('Ctrl Pts',(-38.3756479945492,-86.0473045312185,
114.002384528199));
#37051=CARTESIAN_POINT('Ctrl Pts',(-37.6677627430985,-85.6156398387202,
113.949735020469));
#37052=CARTESIAN_POINT('Ctrl Pts',(-36.9598774916477,-85.1839751462218,
113.897085512738));
#37053=CARTESIAN_POINT('Ctrl Pts',(-36.0182926797001,-85.1355534546481,
113.844436005007));
#37054=CARTESIAN_POINT('Ctrl Pts',(-35.2698614632483,-85.4923260015343,
113.791786497276));
#37055=CARTESIAN_POINT('Ctrl Pts',(-34.5214302467965,-85.8490985484205,
113.739136989545));
#37056=CARTESIAN_POINT('Ctrl Pts',(-33.9661526258405,-86.6110653337667,
113.686487481815));
#37057=CARTESIAN_POINT('Ctrl Pts',(-33.855755265838,-87.4328003025223,113.633837974084));
#37058=CARTESIAN_POINT('Ctrl Pts',(-33.7453579058355,-88.2545352712778,
113.581188466353));
#37059=CARTESIAN_POINT('Ctrl Pts',(-34.0798408067865,-89.1360384234427,
113.528538958622));
#37060=CARTESIAN_POINT('Ctrl Pts',(-34.7075712319637,-89.6776937098362,
113.475889450891));
#37061=CARTESIAN_POINT('Ctrl Pts',(-35.3353016571408,-90.2193489962298,
113.42323994316));
#37062=CARTESIAN_POINT('Ctrl Pts',(-36.2562796065442,-90.421156416852,113.37059043543));
#37063=CARTESIAN_POINT('Ctrl Pts',(-37.0529937319507,-90.1916296464115,
113.317940927699));
#37064=CARTESIAN_POINT('Ctrl Pts',(-37.8497078573572,-89.9621028759709,
113.265291419968));
#37065=CARTESIAN_POINT('Ctrl Pts',(-38.522158158767,-89.3012419144675,113.212641912237));
#37066=CARTESIAN_POINT('Ctrl Pts',(-38.7654995178616,-88.50863802921,113.159992404506));
#37067=CARTESIAN_POINT('Ctrl Pts',(-38.8385397406153,-88.2707336937116,
113.144189370502));
#37068=CARTESIAN_POINT('Ctrl Pts',(-38.8729201383152,-88.0209602082557,
113.128386336497));
#37069=CARTESIAN_POINT('Ctrl Pts',(-38.8709180488009,-87.7706492052449,
113.112583302492));
#37070=CARTESIAN_POINT('Ctrl Pts',(-38.8685313431306,-87.768184262399,113.387416697508));
#37071=CARTESIAN_POINT('Ctrl Pts',(-38.8679443495754,-88.2093775695351,
113.415204380874));
#37072=CARTESIAN_POINT('Ctrl Pts',(-38.757349980407,-88.6508460904898,113.442992064241));
#37073=CARTESIAN_POINT('Ctrl Pts',(-38.5384808246602,-89.0297751758553,
113.470779747607));
#37074=CARTESIAN_POINT('Ctrl Pts',(-38.1237879855467,-89.747734623804,113.523429255338));
#37075=CARTESIAN_POINT('Ctrl Pts',(-37.3203980619691,-90.2411829270465,
113.576078763068));
#37076=CARTESIAN_POINT('Ctrl Pts',(-36.4925156587813,-90.2864228010837,
113.628728270799));
#37077=CARTESIAN_POINT('Ctrl Pts',(-35.6646332555936,-90.3316626751209,
113.68137777853));
#37078=CARTESIAN_POINT('Ctrl Pts',(-34.8122583727957,-89.9286941199529,
113.734027286261));
#37079=CARTESIAN_POINT('Ctrl Pts',(-34.321802201599,-89.2601968021977,113.786676793992));
#37080=CARTESIAN_POINT('Ctrl Pts',(-33.8313460304022,-88.5916994844425,
113.839326301723));
#37081=CARTESIAN_POINT('Ctrl Pts',(-33.7028085708067,-87.6576734041001,
113.891975809453));
#37082=CARTESIAN_POINT('Ctrl Pts',(-33.9944603254749,-86.8815450811342,
113.944625317184));
#37083=CARTESIAN_POINT('Ctrl Pts',(-34.2861120801431,-86.1054167581684,
113.997274824915));
#37084=CARTESIAN_POINT('Ctrl Pts',(-34.9979530490751,-85.4871861925791,
114.049924332646));
#37085=CARTESIAN_POINT('Ctrl Pts',(-35.8072809538378,-85.3071188099598,
114.102573840377));
#37086=CARTESIAN_POINT('Ctrl Pts',(-36.6166088586004,-85.1270514273405,
114.155223348107));
#37087=CARTESIAN_POINT('Ctrl Pts',(-37.5234236991937,-85.3851472276913,
114.207872855838));
#37088=CARTESIAN_POINT('Ctrl Pts',(-38.116634757398,-85.9644024047377,114.260522363569));
#37089=CARTESIAN_POINT('Ctrl Pts',(-38.5932148519415,-86.4297704777422,
114.302820474882));
#37090=CARTESIAN_POINT('Ctrl Pts',(-38.8673837119047,-87.1024264394285,
114.345118586195));
#37091=CARTESIAN_POINT('Ctrl Pts',(-38.8734137783908,-87.7707089500124,
114.387416697508));
#37092=CARTESIAN_POINT('Origin',(-36.3549260746835,-87.7685555885722,114.));
#37093=CARTESIAN_POINT('',(-38.8748658262276,-87.7668088525845,115.387416697508));
#37094=CARTESIAN_POINT('',(-38.8696970919136,-87.7669042806264,115.112583302492));
#37095=CARTESIAN_POINT('',(-38.8724260746835,-87.7685555885722,114.));
#37096=CARTESIAN_POINT('Ctrl Pts',(-38.8696970919136,-87.7669042806264,
115.112583302492));
#37097=CARTESIAN_POINT('Ctrl Pts',(-38.871539656816,-87.4644833190019,115.0935137626));
#37098=CARTESIAN_POINT('Ctrl Pts',(-38.8210274992386,-87.1626571043369,
115.074444222708));
#37099=CARTESIAN_POINT('Ctrl Pts',(-38.7153918518087,-86.8815450706432,
115.055374682816));
#37100=CARTESIAN_POINT('Ctrl Pts',(-38.423740093691,-86.1054167384983,115.002725175085));
#37101=CARTESIAN_POINT('Ctrl Pts',(-37.7118991163401,-85.4871861655974,
114.950075667354));
#37102=CARTESIAN_POINT('Ctrl Pts',(-36.9025712020056,-85.3071187808487,
114.897426159623));
#37103=CARTESIAN_POINT('Ctrl Pts',(-36.0932432876712,-85.1270513961,114.844776651893));
#37104=CARTESIAN_POINT('Ctrl Pts',(-35.1864284363532,-85.3851471995034,
114.792127144162));
#37105=CARTESIAN_POINT('Ctrl Pts',(-34.5932173711332,-85.9644023834006,
114.739477636431));
#37106=CARTESIAN_POINT('Ctrl Pts',(-34.0000063059132,-86.5436575672978,
114.6868281287));
#37107=CARTESIAN_POINT('Ctrl Pts',(-33.7203990267912,-87.4440721316887,
114.634178620969));
#37108=CARTESIAN_POINT('Ctrl Pts',(-33.8811512418217,-88.2574568262423,
114.581529113239));
#37109=CARTESIAN_POINT('Ctrl Pts',(-34.0419034568521,-89.0708415207959,
114.528879605508));
#37110=CARTESIAN_POINT('Ctrl Pts',(-34.643015166035,-89.797196345512,114.476230097777));
#37111=CARTESIAN_POINT('Ctrl Pts',(-35.4119815170054,-90.1072393861475,
114.423580590046));
#37112=CARTESIAN_POINT('Ctrl Pts',(-36.1809478679757,-90.417282426783,114.370931082315));
#37113=CARTESIAN_POINT('Ctrl Pts',(-37.1177688607336,-90.3110136833377,
114.318281574584));
#37114=CARTESIAN_POINT('Ctrl Pts',(-37.7977509442735,-89.8366084746437,
114.265632066854));
#37115=CARTESIAN_POINT('Ctrl Pts',(-38.4566391413284,-89.3769199031411,
114.214615812066));
#37116=CARTESIAN_POINT('Ctrl Pts',(-38.8743761908434,-88.5715807006019,
114.163599557279));
#37117=CARTESIAN_POINT('Ctrl Pts',(-38.8764405008163,-87.7680895936699,
114.112583302492));
#37118=CARTESIAN_POINT('Ctrl Pts',(-38.8734137783908,-87.7707089500124,
114.387416697508));
#37119=CARTESIAN_POINT('Ctrl Pts',(-38.8748894851466,-87.9342542472236,
114.397768093926));
#37120=CARTESIAN_POINT('Ctrl Pts',(-38.8603062997799,-88.0975376174732,
114.408119490344));
#37121=CARTESIAN_POINT('Ctrl Pts',(-38.8287008782886,-88.2574568204596,
114.418470886762));
#37122=CARTESIAN_POINT('Ctrl Pts',(-38.6679486651595,-89.0708415053934,
114.471120394492));
#37123=CARTESIAN_POINT('Ctrl Pts',(-38.066836963086,-89.7971963215193,114.523769902223));
#37124=CARTESIAN_POINT('Ctrl Pts',(-37.2978706212101,-90.1072393584882,
114.576419409954));
#37125=CARTESIAN_POINT('Ctrl Pts',(-36.5289042793342,-90.417282395457,114.629068917685));
#37126=CARTESIAN_POINT('Ctrl Pts',(-35.5920832976559,-90.3110136532687,
114.681718425416));
#37127=CARTESIAN_POINT('Ctrl Pts',(-34.912101222158,-89.8366084501855,114.734367933147));
#37128=CARTESIAN_POINT('Ctrl Pts',(-34.2321191466601,-89.3622032471024,
114.787017440877));
#37129=CARTESIAN_POINT('Ctrl Pts',(-33.8089759773425,-88.5196615831244,
114.839666948608));
#37130=CARTESIAN_POINT('Ctrl Pts',(-33.8344972353565,-87.6909369092428,
114.892316456339));
#37131=CARTESIAN_POINT('Ctrl Pts',(-33.8600184933705,-86.8622122353612,
114.94496596407));
#37132=CARTESIAN_POINT('Ctrl Pts',(-34.3342041787161,-86.0473045515759,
114.997615471801));
#37133=CARTESIAN_POINT('Ctrl Pts',(-35.0420894217948,-85.6156398641826,
115.050264979531));
#37134=CARTESIAN_POINT('Ctrl Pts',(-35.7499746648734,-85.1839751767894,
115.102914487262));
#37135=CARTESIAN_POINT('Ctrl Pts',(-36.6915594656851,-85.1355534857881,
115.155563994993));
#37136=CARTESIAN_POINT('Ctrl Pts',(-37.4399906732854,-85.4923260284547,
115.208213502724));
#37137=CARTESIAN_POINT('Ctrl Pts',(-38.1884218808857,-85.8490985711212,
115.260863010455));
#37138=CARTESIAN_POINT('Ctrl Pts',(-38.7436994952747,-86.6110653474556,
115.313512518185));
#37139=CARTESIAN_POINT('Ctrl Pts',(-38.8540968539717,-87.4328003064926,
115.366162025916));
#37140=CARTESIAN_POINT('Ctrl Pts',(-38.868952704196,-87.5433787806482,115.373246916447));
#37141=CARTESIAN_POINT('Ctrl Pts',(-38.8757525296954,-87.6550395549316,
115.380331806977));
#37142=CARTESIAN_POINT('Ctrl Pts',(-38.8748658262276,-87.7668088525845,
115.387416697508));
#37143=CARTESIAN_POINT('Origin',(-36.3549260746835,-87.7685555885722,114.));
#37144=CARTESIAN_POINT('',(-38.868558082292,-87.7680988643522,116.387416697508));
#37145=CARTESIAN_POINT('',(-38.8707765205166,-87.7706159292182,116.112583302492));
#37146=CARTESIAN_POINT('',(-38.8724260746835,-87.7685555885722,114.));
#37147=CARTESIAN_POINT('Ctrl Pts',(-38.8707765205166,-87.7706159292182,
116.112583302492));
#37148=CARTESIAN_POINT('Ctrl Pts',(-38.8662439615746,-87.1923021573119,
116.076077475652));
#37149=CARTESIAN_POINT('Ctrl Pts',(-38.6678381140232,-86.6111785578358,
116.039571648811));
#37150=CARTESIAN_POINT('Ctrl Pts',(-38.3027347101873,-86.167110034283,116.003065821971));
#37151=CARTESIAN_POINT('Ctrl Pts',(-37.7761745375653,-85.5266646263211,
115.95041631424));
#37152=CARTESIAN_POINT('Ctrl Pts',(-36.9028827165968,-85.1712943775174,
115.897766806509));
#37153=CARTESIAN_POINT('Ctrl Pts',(-36.0787528143328,-85.2621009861182,
115.845117298778));
#37154=CARTESIAN_POINT('Ctrl Pts',(-35.2546229120689,-85.352907594719,115.792467791047));
#37155=CARTESIAN_POINT('Ctrl Pts',(-34.4796549285094,-85.8898910607243,
115.739818283317));
#37156=CARTESIAN_POINT('Ctrl Pts',(-34.1051688142083,-86.6296180956276,
115.687168775586));
#37157=CARTESIAN_POINT('Ctrl Pts',(-33.7306826999072,-87.3693451305309,
115.634519267855));
#37158=CARTESIAN_POINT('Ctrl Pts',(-33.7566784548643,-88.3118157343321,
115.581869760124));
#37159=CARTESIAN_POINT('Ctrl Pts',(-34.1713712988825,-89.0297751907719,
115.529220252393));
#37160=CARTESIAN_POINT('Ctrl Pts',(-34.5860641429007,-89.7477346472117,
115.476570744662));
#37161=CARTESIAN_POINT('Ctrl Pts',(-35.38945407598,-90.2411829562899,115.423921236932));
#37162=CARTESIAN_POINT('Ctrl Pts',(-36.217336488959,-90.2864228308621,115.371271729201));
#37163=CARTESIAN_POINT('Ctrl Pts',(-37.045218901938,-90.3316627054341,115.31862222147));
#37164=CARTESIAN_POINT('Ctrl Pts',(-37.8975937948167,-89.9286941455001,
115.265972713739));
#37165=CARTESIAN_POINT('Ctrl Pts',(-38.3880499718138,-89.2601968198386,
115.213323206008));
#37166=CARTESIAN_POINT('Ctrl Pts',(-38.7008639630498,-88.8338278058908,
115.17974323817));
#37167=CARTESIAN_POINT('Ctrl Pts',(-38.8664524792742,-88.2994439340536,
115.146163270331));
#37168=CARTESIAN_POINT('Ctrl Pts',(-38.8696970919136,-87.7669042806264,
115.112583302492));
#37169=CARTESIAN_POINT('Ctrl Pts',(-38.8748658262276,-87.7668088525845,
115.387416697508));
#37170=CARTESIAN_POINT('Ctrl Pts',(-38.8691632251914,-88.4856238067917,
115.432981314708));
#37171=CARTESIAN_POINT('Ctrl Pts',(-38.5455394661889,-89.2089273767851,
115.478545931909));
#37172=CARTESIAN_POINT('Ctrl Pts',(-38.0022808979207,-89.6776936872569,
115.524110549109));
#37173=CARTESIAN_POINT('Ctrl Pts',(-37.3745504801678,-90.2193489672445,
115.57676005684));
#37174=CARTESIAN_POINT('Ctrl Pts',(-36.4535725416567,-90.4211563854802,
115.62940956457));
#37175=CARTESIAN_POINT('Ctrl Pts',(-35.6568584256728,-90.1916296177544,
115.682059072301));
#37176=CARTESIAN_POINT('Ctrl Pts',(-34.8601443096888,-89.9621028500285,
115.734708580032));
#37177=CARTESIAN_POINT('Ctrl Pts',(-34.1876940162318,-89.3012418963412,
115.787358087763));
#37178=CARTESIAN_POINT('Ctrl Pts',(-33.944352660015,-88.5086380204578,115.840007595494));
#37179=CARTESIAN_POINT('Ctrl Pts',(-33.7010113037982,-87.7160341445744,
115.892657103225));
#37180=CARTESIAN_POINT('Ctrl Pts',(-33.8867788848215,-86.7916873464949,
115.945306610955));
#37181=CARTESIAN_POINT('Ctrl Pts',(-34.4174404951608,-86.1546361907602,
115.997956118686));
#37182=CARTESIAN_POINT('Ctrl Pts',(-34.9481021055002,-85.5175850350255,
116.050605626417));
#37183=CARTESIAN_POINT('Ctrl Pts',(-35.8236577451555,-85.1678295216356,
116.103255134148));
#37184=CARTESIAN_POINT('Ctrl Pts',(-36.6471875792997,-85.2639259939193,
116.155904641879));
#37185=CARTESIAN_POINT('Ctrl Pts',(-37.4707174134438,-85.3600224662028,
116.208554149609));
#37186=CARTESIAN_POINT('Ctrl Pts',(-38.2422214420767,-85.90197092416,116.26120365734));
#37187=CARTESIAN_POINT('Ctrl Pts',(-38.6119500459349,-86.6440872756844,
116.313853165071));
#37188=CARTESIAN_POINT('Ctrl Pts',(-38.7841488205295,-86.9897233043973,
116.33837434255));
#37189=CARTESIAN_POINT('Ctrl Pts',(-38.8691955906087,-87.3787791942771,
116.362895520029));
#37190=CARTESIAN_POINT('Ctrl Pts',(-38.868558082292,-87.7680988643522,116.387416697508));
#37191=CARTESIAN_POINT('Origin',(-36.3549260746835,-87.7685555885722,114.));
#37192=CARTESIAN_POINT('',(-38.8732538877992,-87.7707324389422,117.387416697508));
#37193=CARTESIAN_POINT('',(-38.8764805590541,-87.7681855672363,117.112583302492));
#37194=CARTESIAN_POINT('',(-38.8724260746835,-87.7685555885722,114.));
#37195=CARTESIAN_POINT('Ctrl Pts',(-38.8764805590541,-87.7681855672363,
117.112583302492));
#37196=CARTESIAN_POINT('Ctrl Pts',(-38.8765227322016,-87.7478282685136,
117.111290696434));
#37197=CARTESIAN_POINT('Ctrl Pts',(-38.8762972958495,-87.7274719274955,
117.109998090376));
#37198=CARTESIAN_POINT('Ctrl Pts',(-38.8758013750463,-87.707122178149,117.108705484318));
#37199=CARTESIAN_POINT('Ctrl Pts',(-38.8556018827122,-86.8782507065199,
117.056055976587));
#37200=CARTESIAN_POINT('Ctrl Pts',(-38.3866584880058,-86.0603150667128,
117.003406468856));
#37201=CARTESIAN_POINT('Ctrl Pts',(-37.6815595477827,-85.6241139428405,
116.950756961126));
#37202=CARTESIAN_POINT('Ctrl Pts',(-36.9764606075597,-85.1879128189682,
116.898107453395));
#37203=CARTESIAN_POINT('Ctrl Pts',(-36.0352061218199,-85.1334462110306,
116.845457945664));
#37204=CARTESIAN_POINT('Ctrl Pts',(-35.2844994981932,-85.4854057274726,
116.792808437933));
#37205=CARTESIAN_POINT('Ctrl Pts',(-34.5337928745664,-85.8373652439147,
116.740158930202));
#37206=CARTESIAN_POINT('Ctrl Pts',(-33.9736341130527,-86.5957508847365,
116.687509422471));
#37207=CARTESIAN_POINT('Ctrl Pts',(-33.8579626699548,-87.4167600522997,
116.634859914741));
#37208=CARTESIAN_POINT('Ctrl Pts',(-33.7422912268569,-88.2377692198629,
116.58221040701));
#37209=CARTESIAN_POINT('Ctrl Pts',(-34.0711071021749,-89.1214019141675,
116.529560899279));
#37210=CARTESIAN_POINT('Ctrl Pts',(-34.6953466190748,-89.6670766904874,
116.476911391548));
#37211=CARTESIAN_POINT('Ctrl Pts',(-35.3195861359746,-90.2127514668073,
116.424261883817));
#37212=CARTESIAN_POINT('Ctrl Pts',(-36.2392492944564,-90.4204683251425,
116.371612376086));
#37213=CARTESIAN_POINT('Ctrl Pts',(-37.0374207867677,-90.1960619864779,
116.318962868356));
#37214=CARTESIAN_POINT('Ctrl Pts',(-37.8355922790789,-89.9716556478134,
116.266313360625));
#37215=CARTESIAN_POINT('Ctrl Pts',(-38.5122721052197,-89.3151261121492,
116.213663852894));
#37216=CARTESIAN_POINT('Ctrl Pts',(-38.7606977561522,-88.5241010607571,
116.161014345163));
#37217=CARTESIAN_POINT('Ctrl Pts',(-38.8368713920796,-88.2815526200145,
116.144870664273));
#37218=CARTESIAN_POINT('Ctrl Pts',(-38.8727809179377,-88.0263590200123,
116.128726983382));
#37219=CARTESIAN_POINT('Ctrl Pts',(-38.8707765205166,-87.7706159292182,
116.112583302492));
#37220=CARTESIAN_POINT('Ctrl Pts',(-38.868558082292,-87.7680988643522,116.387416697508));
#37221=CARTESIAN_POINT('Ctrl Pts',(-38.8678267942253,-88.2146888481658,
116.41554502776));
#37222=CARTESIAN_POINT('Ctrl Pts',(-38.7543481395299,-88.6616259262534,
116.443673358012));
#37223=CARTESIAN_POINT('Ctrl Pts',(-38.5303375221176,-89.0437697775872,
116.471801688264));
#37224=CARTESIAN_POINT('Ctrl Pts',(-38.1110432153587,-89.7590516828738,
116.524451195994));
#37225=CARTESIAN_POINT('Ctrl Pts',(-37.3045014227577,-90.2473312483554,
116.577100703725));
#37226=CARTESIAN_POINT('Ctrl Pts',(-36.4763456010602,-90.2872543581965,
116.629750211456));
#37227=CARTESIAN_POINT('Ctrl Pts',(-35.6481897793627,-90.3271774680377,
116.682399719187));
#37228=CARTESIAN_POINT('Ctrl Pts',(-34.7984199285688,-89.9187441222385,
116.735049226918));
#37229=CARTESIAN_POINT('Ctrl Pts',(-34.312266288245,-89.2471113671478,116.787698734649));
#37230=CARTESIAN_POINT('Ctrl Pts',(-33.8261126479212,-88.5754786120571,
116.840348242379));
#37231=CARTESIAN_POINT('Ctrl Pts',(-33.7035752180675,-87.640646447675,116.89299775011));
#37232=CARTESIAN_POINT('Ctrl Pts',(-34.0002044791045,-86.8664068199061,
116.945647257841));
#37233=CARTESIAN_POINT('Ctrl Pts',(-34.2968337401414,-86.0921671921372,
116.998296765572));
#37234=CARTESIAN_POINT('Ctrl Pts',(-35.012629692069,-85.4785201009814,117.050946273303));
#37235=CARTESIAN_POINT('Ctrl Pts',(-35.8230971250555,-85.303653123599,117.103595781034));
#37236=CARTESIAN_POINT('Ctrl Pts',(-36.633564558042,-85.1287861462166,117.156245288764));
#37237=CARTESIAN_POINT('Ctrl Pts',(-37.5387034720875,-85.3926992826077,
117.208894796495));
#37238=CARTESIAN_POINT('Ctrl Pts',(-38.1281829047877,-85.9757515256646,
117.261544304226));
#37239=CARTESIAN_POINT('Ctrl Pts',(-38.5979510639627,-86.4403977265829,
117.303501768653));
#37240=CARTESIAN_POINT('Ctrl Pts',(-38.8672495515809,-87.1077234466512,
117.345459233081));
#37241=CARTESIAN_POINT('Ctrl Pts',(-38.8732538877992,-87.7707324389422,
117.387416697508));
#37242=CARTESIAN_POINT('Origin',(-36.3549260746835,-87.7685555885722,114.));
#37243=CARTESIAN_POINT('',(-38.8750031561041,-87.7668692329086,118.387416697508));
#37244=CARTESIAN_POINT('',(-38.8698085201626,-87.7668461825819,118.112583302492));
#37245=CARTESIAN_POINT('',(-38.8724260746835,-87.7685555885722,114.));
#37246=CARTESIAN_POINT('Ctrl Pts',(-38.8698085201626,-87.7668461825819,
118.112583302492));
#37247=CARTESIAN_POINT('Ctrl Pts',(-38.8716872313444,-87.4698606038117,
118.093854409486));
#37248=CARTESIAN_POINT('Ctrl Pts',(-38.8230124046943,-87.1734707974551,
118.075125516479));
#37249=CARTESIAN_POINT('Ctrl Pts',(-38.7210386843352,-86.8967199031838,
118.056396623473));
#37250=CARTESIAN_POINT('Ctrl Pts',(-38.4343764573392,-86.1187348753197,
118.003747115742));
#37251=CARTESIAN_POINT('Ctrl Pts',(-37.7265198119899,-85.4959463173494,
117.951097608011));
#37252=CARTESIAN_POINT('Ctrl Pts',(-36.9183647941979,-85.3106859514149,
117.89844810028));
#37253=CARTESIAN_POINT('Ctrl Pts',(-36.110209776406,-85.1254255854804,117.845798592549));
#37254=CARTESIAN_POINT('Ctrl Pts',(-35.2017563861714,-85.3776934115817,
117.793149084819));
#37255=CARTESIAN_POINT('Ctrl Pts',(-34.6048381532838,-85.9531276469379,
117.740499577088));
#37256=CARTESIAN_POINT('Ctrl Pts',(-34.0079199203962,-86.5285618822942,
117.687850069357));
#37257=CARTESIAN_POINT('Ctrl Pts',(-33.7225368448558,-87.4271625269054,
117.635200561626));
#37258=CARTESIAN_POINT('Ctrl Pts',(-33.8780630041881,-88.2415626433923,
117.582551053895));
#37259=CARTESIAN_POINT('Ctrl Pts',(-34.0335891635205,-89.0559627598792,
117.529901546165));
#37260=CARTESIAN_POINT('Ctrl Pts',(-34.6300245577258,-89.7861623482417,
117.477252038434));
#37261=CARTESIAN_POINT('Ctrl Pts',(-35.3969842707239,-90.1011365291023,
117.424602530703));
#37262=CARTESIAN_POINT('Ctrl Pts',(-36.163943983722,-90.4161107099629,117.371953022972));
#37263=CARTESIAN_POINT('Ctrl Pts',(-37.1014280155131,-90.3158594833215,
117.319303515241));
#37264=CARTESIAN_POINT('Ctrl Pts',(-37.7844422364276,-89.8458302182753,
117.26665400751));
#37265=CARTESIAN_POINT('Ctrl Pts',(-38.4506876715034,-89.3873407130792,
117.215297105838));
#37266=CARTESIAN_POINT('Ctrl Pts',(-38.874804965645,-88.5770072359445,117.163940204165));
#37267=CARTESIAN_POINT('Ctrl Pts',(-38.8764805590541,-87.7681855672363,
117.112583302492));
#37268=CARTESIAN_POINT('Ctrl Pts',(-38.8732538877992,-87.7707324389422,
117.387416697508));
#37269=CARTESIAN_POINT('Ctrl Pts',(-38.8747839760381,-87.9396873782579,
117.398108740812));
#37270=CARTESIAN_POINT('Ctrl Pts',(-38.8592161096564,-88.1083619952982,
117.408800784115));
#37271=CARTESIAN_POINT('Ctrl Pts',(-38.8255106478334,-88.2733308458954,
117.419492827418));
#37272=CARTESIAN_POINT('Ctrl Pts',(-38.6595390068241,-89.0856665733467,
117.472142335149));
#37273=CARTESIAN_POINT('Ctrl Pts',(-38.0537757734505,-89.8081466785269,
117.52479184288));
#37274=CARTESIAN_POINT('Ctrl Pts',(-37.2828344978364,-90.1132457923617,
117.577441350611));
#37275=CARTESIAN_POINT('Ctrl Pts',(-36.5118932222224,-90.4183449061965,
117.630090858342));
#37276=CARTESIAN_POINT('Ctrl Pts',(-35.5757739043679,-90.3060630286859,
117.682740366073));
#37277=CARTESIAN_POINT('Ctrl Pts',(-34.8988520016275,-89.8273014415711,
117.735389873803));
#37278=CARTESIAN_POINT('Ctrl Pts',(-34.2219300988871,-89.3485398544562,
117.788039381534));
#37279=CARTESIAN_POINT('Ctrl Pts',(-33.8042056112606,-88.5032985577371,
117.840688889265));
#37280=CARTESIAN_POINT('Ctrl Pts',(-33.8350475829636,-87.6747548398119,
117.893338396996));
#37281=CARTESIAN_POINT('Ctrl Pts',(-33.8658895546665,-86.8462111218867,
117.945987904727));
#37282=CARTESIAN_POINT('Ctrl Pts',(-34.3452979856988,-86.0343649827555,
117.998637412457));
#37283=CARTESIAN_POINT('Ctrl Pts',(-35.0559403541099,-85.6072545240904,
118.051286920188));
#37284=CARTESIAN_POINT('Ctrl Pts',(-35.766582722521,-85.1801440654253,118.103936427919));
#37285=CARTESIAN_POINT('Ctrl Pts',(-36.7084590283107,-85.1377692872263,
118.15658593565));
#37286=CARTESIAN_POINT('Ctrl Pts',(-37.4545839712195,-85.4993401506215,
118.209235443381));
#37287=CARTESIAN_POINT('Ctrl Pts',(-38.2007089141282,-85.8609110140166,
118.261884951112));
#37288=CARTESIAN_POINT('Ctrl Pts',(-38.751082494156,-86.626427519006,118.314534458842));
#37289=CARTESIAN_POINT('Ctrl Pts',(-38.8562012181559,-87.4488543994952,
118.367183966573));
#37290=CARTESIAN_POINT('Ctrl Pts',(-38.8696666106516,-87.554204810187,118.373928210218));
#37291=CARTESIAN_POINT('Ctrl Pts',(-38.8758258875797,-87.6604890541088,
118.380672453863));
#37292=CARTESIAN_POINT('Ctrl Pts',(-38.8750031561041,-87.7668692329086,
118.387416697508));
#37293=CARTESIAN_POINT('Origin',(-36.3549260746835,-87.7685555885722,114.));
#37294=CARTESIAN_POINT('',(-38.8685903326823,-87.7680141435005,119.387416697508));
#37295=CARTESIAN_POINT('',(-38.8706378814634,-87.770579470363,119.112583302492));
#37296=CARTESIAN_POINT('',(-38.8724260746835,-87.7685555885722,114.));
#37297=CARTESIAN_POINT('Ctrl Pts',(-38.8706378814634,-87.770579470363,119.112583302492));
#37298=CARTESIAN_POINT('Ctrl Pts',(-38.866244667136,-87.1975822133564,119.076418122537));
#37299=CARTESIAN_POINT('Ctrl Pts',(-38.671841736866,-86.6218880939353,119.040252942582));
#37300=CARTESIAN_POINT('Ctrl Pts',(-38.3129774354871,-86.1796499242353,
119.004087762628));
#37301=CARTESIAN_POINT('Ctrl Pts',(-37.7905404164158,-85.5358366772506,
118.951438254897));
#37302=CARTESIAN_POINT('Ctrl Pts',(-36.9195484306298,-85.174866348328,118.898788747166));
#37303=CARTESIAN_POINT('Ctrl Pts',(-36.0948524487308,-85.260379348023,118.846139239435));
#37304=CARTESIAN_POINT('Ctrl Pts',(-35.2701564668318,-85.345892347718,118.793489731704));
#37305=CARTESIAN_POINT('Ctrl Pts',(-34.4917564888197,-85.8778886760306,
118.740840223973));
#37306=CARTESIAN_POINT('Ctrl Pts',(-34.1125283082994,-86.6151958869313,
118.688190716243));
#37307=CARTESIAN_POINT('Ctrl Pts',(-33.733300127779,-87.352503097832,118.635541208512));
#37308=CARTESIAN_POINT('Ctrl Pts',(-33.7532437447503,-88.2951211913206,
118.582891700781));
#37309=CARTESIAN_POINT('Ctrl Pts',(-34.1633180234681,-89.015728589202,118.53024219305));
#37310=CARTESIAN_POINT('Ctrl Pts',(-34.5733923021859,-89.7363359870834,
118.477592685319));
#37311=CARTESIAN_POINT('Ctrl Pts',(-35.3735972426501,-90.2349326893574,
118.424943177588));
#37312=CARTESIAN_POINT('Ctrl Pts',(-36.2011721037992,-90.2854874629831,
118.372293669858));
#37313=CARTESIAN_POINT('Ctrl Pts',(-37.0287469649484,-90.3360422366088,
118.319644162127));
#37314=CARTESIAN_POINT('Ctrl Pts',(-37.8836917467824,-89.938555081586,118.266994654396));
#37315=CARTESIAN_POINT('Ctrl Pts',(-38.3784302333781,-89.2732207551958,
118.214345146665));
#37316=CARTESIAN_POINT('Ctrl Pts',(-38.6971764917278,-88.8445643380494,
118.180424531941));
#37317=CARTESIAN_POINT('Ctrl Pts',(-38.8664059144585,-88.3047281274853,
118.146503917216));
#37318=CARTESIAN_POINT('Ctrl Pts',(-38.8698085201626,-87.7668461825819,
118.112583302492));
#37319=CARTESIAN_POINT('Ctrl Pts',(-38.8750031561041,-87.7668692329086,
118.387416697508));
#37320=CARTESIAN_POINT('Ctrl Pts',(-38.8694031648155,-88.4909549063227,
118.433321961594));
#37321=CARTESIAN_POINT('Ctrl Pts',(-38.5403295713882,-89.2194852035135,
118.47922722568));
#37322=CARTESIAN_POINT('Ctrl Pts',(-37.9899883652829,-89.6882319936022,
118.525132489766));
#37323=CARTESIAN_POINT('Ctrl Pts',(-37.3587929204378,-90.2258454512309,
118.577781997497));
#37324=CARTESIAN_POINT('Ctrl Pts',(-36.4365381627752,-90.4217351104991,
118.630431505227));
#37325=CARTESIAN_POINT('Ctrl Pts',(-35.6413142618343,-90.1870973748279,
118.683081012958));
#37326=CARTESIAN_POINT('Ctrl Pts',(-34.8460903608934,-89.9524596391566,
118.735730520689));
#37327=CARTESIAN_POINT('Ctrl Pts',(-34.1778973166741,-89.2872945085458,
118.78838002842));
#37328=CARTESIAN_POINT('Ctrl Pts',(-33.9396502852875,-88.4931444766406,
118.841029536151));
#37329=CARTESIAN_POINT('Ctrl Pts',(-33.7014032539009,-87.6989944447354,
118.893679043881));
#37330=CARTESIAN_POINT('Ctrl Pts',(-33.8931022353469,-86.7758595115357,
118.946328551612));
#37331=CARTESIAN_POINT('Ctrl Pts',(-34.4278434102823,-86.1422288678049,
118.998978059343));
#37332=CARTESIAN_POINT('Ctrl Pts',(-34.9625845852178,-85.5085982240741,
119.051627567074));
#37333=CARTESIAN_POINT('Ctrl Pts',(-35.8403679536426,-85.164471869812,119.104277074805));
#37334=CARTESIAN_POINT('Ctrl Pts',(-36.6632637763088,-85.2658542408029,
119.156926582536));
#37335=CARTESIAN_POINT('Ctrl Pts',(-37.4861595989751,-85.3672366117938,
119.209576090266));
#37336=CARTESIAN_POINT('Ctrl Pts',(-38.2541678758828,-85.9141277080375,
119.262225597997));
#37337=CARTESIAN_POINT('Ctrl Pts',(-38.6191237284295,-86.6586027960181,
119.314875105728));
#37338=CARTESIAN_POINT('Ctrl Pts',(-38.7867383280348,-87.000520572969,119.339055636321));
#37339=CARTESIAN_POINT('Ctrl Pts',(-38.8693361655413,-87.3841151894692,
119.363236166915));
#37340=CARTESIAN_POINT('Ctrl Pts',(-38.8685903326823,-87.7680141435005,
119.387416697508));
#37341=CARTESIAN_POINT('Origin',(-36.3549260746835,-87.7685555885722,114.));
#37342=CARTESIAN_POINT('',(-38.873093130194,-87.7707538189189,120.387416697508));
#37343=CARTESIAN_POINT('',(-38.8765118730483,-87.7682823374696,120.112583302492));
#37344=CARTESIAN_POINT('',(-38.8724260746835,-87.7685555885722,114.));
#37345=CARTESIAN_POINT('Ctrl Pts',(-38.8765118730483,-87.7682823374696,
120.112583302492));
#37346=CARTESIAN_POINT('Ctrl Pts',(-38.8765351721742,-87.7532903980737,
120.11163134332));
#37347=CARTESIAN_POINT('Ctrl Pts',(-38.8764129085711,-87.7382988488132,
120.110679384147));
#37348=CARTESIAN_POINT('Ctrl Pts',(-38.8761439194262,-87.7233099327277,
120.109727424975));
#37349=CARTESIAN_POINT('Ctrl Pts',(-38.8612670775668,-86.8943257953643,
120.057077917244));
#37350=CARTESIAN_POINT('Ctrl Pts',(-38.3975852156679,-86.0733960305389,
120.004428409513));
#37351=CARTESIAN_POINT('Ctrl Pts',(-37.6953016325259,-85.6326764849286,
119.951778901782));
#37352=CARTESIAN_POINT('Ctrl Pts',(-36.9930180493839,-85.1919569393182,
119.899129394052));
#37353=CARTESIAN_POINT('Ctrl Pts',(-36.0521327449989,-85.1314476129227,
119.846479886321));
#37354=CARTESIAN_POINT('Ctrl Pts',(-35.299181677782,-85.4785795754927,119.79383037859));
#37355=CARTESIAN_POINT('Ctrl Pts',(-34.5462306105651,-85.8257115380627,
119.741180870859));
#37356=CARTESIAN_POINT('Ctrl Pts',(-33.9812137805165,-86.5804847895982,
119.688531363128));
#37357=CARTESIAN_POINT('Ctrl Pts',(-33.8602730174755,-87.4007343120143,
119.635881855397));
#37358=CARTESIAN_POINT('Ctrl Pts',(-33.7393322544345,-88.2209838344304,
119.583232347667));
#37359=CARTESIAN_POINT('Ctrl Pts',(-34.0624675584012,-89.1067096277273,
119.530582839936));
#37360=CARTESIAN_POINT('Ctrl Pts',(-34.6831904327383,-89.656381393097,119.477933332205));
#37361=CARTESIAN_POINT('Ctrl Pts',(-35.3039133070753,-90.2060531584668,
119.425283824474));
#37362=CARTESIAN_POINT('Ctrl Pts',(-36.2222237517827,-90.4196708959094,
119.372634316743));
#37363=CARTESIAN_POINT('Ctrl Pts',(-37.0218197012666,-90.2003942426243,
119.319984809013));
#37364=CARTESIAN_POINT('Ctrl Pts',(-37.8214156507506,-89.9811175893391,
119.267335301282));
#37365=CARTESIAN_POINT('Ctrl Pts',(-38.5022971050112,-89.328946545326,119.214685793551));
#37366=CARTESIAN_POINT('Ctrl Pts',(-38.7557968059632,-88.5395329407962,
119.16203628582));
#37367=CARTESIAN_POINT('Ctrl Pts',(-38.8351664400152,-88.2923710361789,
119.145551958044));
#37368=CARTESIAN_POINT('Ctrl Pts',(-38.8726403375566,-88.0317554028776,
119.129067630268));
#37369=CARTESIAN_POINT('Ctrl Pts',(-38.8706378814634,-87.770579470363,119.112583302492));
#37370=CARTESIAN_POINT('Ctrl Pts',(-38.8685903326823,-87.7680141435005,
119.387416697508));
#37371=CARTESIAN_POINT('Ctrl Pts',(-38.8677122254576,-88.219998044484,119.415885674646));
#37372=CARTESIAN_POINT('Ctrl Pts',(-38.7513067986863,-88.6724038047288,
119.444354651783));
#37373=CARTESIAN_POINT('Ctrl Pts',(-38.5221045252354,-89.0577118184919,
119.472823628921));
#37374=CARTESIAN_POINT('Ctrl Pts',(-38.0982260413089,-89.7702866732678,
119.525473136651));
#37375=CARTESIAN_POINT('Ctrl Pts',(-37.2885656452704,-90.2533773031023,
119.578122644382));
#37376=CARTESIAN_POINT('Ctrl Pts',(-36.4601705432131,-90.2879820377545,
119.630772152113));
#37377=CARTESIAN_POINT('Ctrl Pts',(-35.6317754411557,-90.3225867724067,
119.683421659844));
#37378=CARTESIAN_POINT('Ctrl Pts',(-34.7846456330796,-89.9087056118767,
119.736071167575));
#37379=CARTESIAN_POINT('Ctrl Pts',(-34.3028145807763,-89.2339650386027,
119.788720675305));
#37380=CARTESIAN_POINT('Ctrl Pts',(-33.8209835284731,-88.5592244653287,
119.841370183036));
#37381=CARTESIAN_POINT('Ctrl Pts',(-33.7044512319429,-87.6236244793106,
119.894019690767));
#37382=CARTESIAN_POINT('Ctrl Pts',(-34.0060457422708,-86.8513056164977,
119.946669198498));
#37383=CARTESIAN_POINT('Ctrl Pts',(-34.3076402525988,-86.0789867536849,
119.999318706229));
#37384=CARTESIAN_POINT('Ctrl Pts',(-35.027361569785,-85.4699490140772,120.05196821396));
#37385=CARTESIAN_POINT('Ctrl Pts',(-35.8389351715648,-85.3002893469818,
120.10461772169));
#37386=CARTESIAN_POINT('Ctrl Pts',(-36.6505087733447,-85.1306296798865,
120.157267229421));
#37387=CARTESIAN_POINT('Ctrl Pts',(-37.5539346597181,-85.4003480853034,
120.209916737152));
#37388=CARTESIAN_POINT('Ctrl Pts',(-38.1396580480158,-85.9871739818863,
120.262566244883));
#37389=CARTESIAN_POINT('Ctrl Pts',(-38.6026432577794,-86.4510306696204,
120.304183062425));
#37390=CARTESIAN_POINT('Ctrl Pts',(-38.8671242526413,-87.1130198050204,
120.345799879966));
#37391=CARTESIAN_POINT('Ctrl Pts',(-38.873093130194,-87.7707538189189,120.387416697508));
#37392=CARTESIAN_POINT('Origin',(-36.3549260746835,-87.7685555885722,114.));
#37393=CARTESIAN_POINT('',(-38.8751287300693,-87.7669767062971,121.387416697508));
#37394=CARTESIAN_POINT('',(-38.8699208872996,-87.7667938007243,121.112583302492));
#37395=CARTESIAN_POINT('',(-38.8724260746835,-87.7685555885722,114.));
#37396=CARTESIAN_POINT('',(-34.4414600780185,-86.1325683851973,122.));
#37397=CARTESIAN_POINT('Ctrl Pts',(-38.8751287300693,-87.7669767062971,
121.387416697508));
#37398=CARTESIAN_POINT('Ctrl Pts',(-38.8696706756881,-88.49619959385,121.43366260848));
#37399=CARTESIAN_POINT('Ctrl Pts',(-38.5351409382516,-89.2296736768507,
121.479908519451));
#37400=CARTESIAN_POINT('Ctrl Pts',(-37.9776638931539,-89.6985069777893,
121.526154430423));
#37401=CARTESIAN_POINT('Ctrl Pts',(-37.3429939000879,-90.2322588703065,
121.578803938153));
#37402=CARTESIAN_POINT('Ctrl Pts',(-36.4193596116175,-90.4230071270047,
121.631453445884));
#37403=CARTESIAN_POINT('Ctrl Pts',(-35.6257426342697,-90.1828532317666,
121.684102953615));
#37404=CARTESIAN_POINT('Ctrl Pts',(-34.832125656922,-89.9426993365284,121.736752461346));
#37405=CARTESIAN_POINT('Ctrl Pts',(-34.168525990697,-89.2716432893538,121.789401969077));
#37406=CARTESIAN_POINT('Ctrl Pts',(-33.9355607493907,-88.4773573530763,
121.842051476808));
#37407=CARTESIAN_POINT('Ctrl Pts',(-33.7025955080844,-87.6830714167989,
121.894700984538));
#37408=CARTESIAN_POINT('Ctrl Pts',(-33.9002646916969,-86.7655555914187,
121.947350492269));
#37409=CARTESIAN_POINT('Ctrl Pts',(-34.4414600780185,-86.1325683851972,
122.));
#37410=CARTESIAN_POINT('',(-38.2720363511395,-86.1300276335002,122.));
#37411=CARTESIAN_POINT('Origin',(-36.3549260746835,-87.7685555885722,122.));
#37412=CARTESIAN_POINT('Ctrl Pts',(-38.2720451973147,-86.1300214660444,
122.));
#37413=CARTESIAN_POINT('Ctrl Pts',(-37.7492246461072,-85.5213064340422,
121.949053726697));
#37414=CARTESIAN_POINT('Ctrl Pts',(-36.9095001229587,-85.1811300134451,
121.898107453395));
#37415=CARTESIAN_POINT('Ctrl Pts',(-36.1108292497374,-85.258892786295,121.847161180092));
#37416=CARTESIAN_POINT('Ctrl Pts',(-35.2854572335304,-85.3392553220591,
121.794511672361));
#37417=CARTESIAN_POINT('Ctrl Pts',(-34.5039297618072,-85.8659692441484,
121.74186216463));
#37418=CARTESIAN_POINT('Ctrl Pts',(-34.1200451421356,-86.6007560283003,
121.6892126569));
#37419=CARTESIAN_POINT('Ctrl Pts',(-33.7361605224639,-87.3355428124522,
121.636563149169));
#37420=CARTESIAN_POINT('Ctrl Pts',(-33.7499187548438,-88.2784024586666,
121.583913641438));
#37421=CARTESIAN_POINT('Ctrl Pts',(-34.1553235431823,-89.0016622385077,
121.531264133707));
#37422=CARTESIAN_POINT('Ctrl Pts',(-34.5607283315209,-89.7249220183489,
121.478614625976));
#37423=CARTESIAN_POINT('Ctrl Pts',(-35.3577796758181,-90.2285819318168,
121.425965118245));
#37424=CARTESIAN_POINT('Ctrl Pts',(-36.1850294050421,-90.2844329189877,
121.373315610515));
#37425=CARTESIAN_POINT('Ctrl Pts',(-37.0122791342662,-90.3402839061586,
121.320666102784));
#37426=CARTESIAN_POINT('Ctrl Pts',(-37.8697272484169,-89.9483259670326,
121.268016595053));
#37427=CARTESIAN_POINT('Ctrl Pts',(-38.3687196042729,-89.286190143456,121.215367087322));
#37428=CARTESIAN_POINT('Ctrl Pts',(-38.6934350362348,-88.8553103565275,
121.181105825712));
#37429=CARTESIAN_POINT('Ctrl Pts',(-38.8663568078635,-88.310019546557,121.146844564102));
#37430=CARTESIAN_POINT('Ctrl Pts',(-38.8699208872996,-87.7667938007243,
121.112583302492));
#37431=CARTESIAN_POINT('Origin',(-36.3549260746835,-87.7685555885722,124.208423447177));
#37432=CARTESIAN_POINT('',(-39.4331960788118,-87.7677421217272,107.791576552823));
#37433=CARTESIAN_POINT('',(-39.4235551911591,-87.7682412648602,107.708423447177));
#37434=CARTESIAN_POINT('',(-39.4284260746835,-87.768555588572,124.208423447177));
#37435=CARTESIAN_POINT('',(-35.5611267921511,-90.7377785423181,107.));
#37436=CARTESIAN_POINT('Ctrl Pts',(-39.4235551911591,-87.7682412648602,
107.708423447177));
#37437=CARTESIAN_POINT('Ctrl Pts',(-39.4238750506399,-87.2730657797943,
107.682880329042));
#37438=CARTESIAN_POINT('Ctrl Pts',(-39.077622760914,-85.7577492069975,107.604687703175));
#37439=CARTESIAN_POINT('Ctrl Pts',(-36.7064604496932,-84.1596939007676,
107.473845569577));
#37440=CARTESIAN_POINT('Ctrl Pts',(-33.5229009026989,-85.5001505522318,
107.315897046385));
#37441=CARTESIAN_POINT('Ctrl Pts',(-32.9121328624527,-88.9023373811549,
107.157948523192));
#37442=CARTESIAN_POINT('Ctrl Pts',(-34.5788882023795,-90.4751844899406,
107.052649507731));
#37443=CARTESIAN_POINT('Ctrl Pts',(-35.5611267921512,-90.7377785423181,
107.));
#37444=CARTESIAN_POINT('',(-37.1487253572168,-90.7377785423178,107.));
#37445=CARTESIAN_POINT('Origin',(-36.3549260746835,-87.7685555885722,107.));
#37446=CARTESIAN_POINT('Ctrl Pts',(-39.4331960788118,-87.7677421217272,
107.791576552823));
#37447=CARTESIAN_POINT('Ctrl Pts',(-39.4333521478699,-87.7232332784528,
107.789262006108));
#37448=CARTESIAN_POINT('Ctrl Pts',(-39.4123924336899,-86.666423722535,107.734297951662));
#37449=CARTESIAN_POINT('Ctrl Pts',(-38.2031234854001,-84.6483923994501,
107.626684389485));
#37450=CARTESIAN_POINT('Ctrl Pts',(-34.7524573177229,-84.5150170933021,
107.468735866293));
#37451=CARTESIAN_POINT('Ctrl Pts',(-32.7548482639927,-87.3323302896557,
107.3107873431));
#37452=CARTESIAN_POINT('Ctrl Pts',(-34.0073630870521,-90.5088743722522,
107.154542054336));
#37453=CARTESIAN_POINT('Ctrl Pts',(-36.2036732140504,-90.9937479068112,
107.050946273303));
#37454=CARTESIAN_POINT('Ctrl Pts',(-37.1506394945612,-90.7428673099699,
107.));
#37455=CARTESIAN_POINT('Origin',(-36.3549260746835,-87.7685555885722,124.208423447177));
#37456=CARTESIAN_POINT('',(-39.4248378354749,-87.7666901941256,108.791576552823));
#37457=CARTESIAN_POINT('',(-39.4300190231571,-87.7711138662458,108.708423447177));
#37458=CARTESIAN_POINT('',(-39.4284260746835,-87.768555588572,124.208423447177));
#37459=CARTESIAN_POINT('Ctrl Pts',(-39.4300190231571,-87.7711138662458,
108.708423447177));
#37460=CARTESIAN_POINT('Ctrl Pts',(-39.422631166441,-86.9423658304694,108.665444042093));
#37461=CARTESIAN_POINT('Ctrl Pts',(-38.6509821187261,-85.0862753982503,
108.569815129278));
#37462=CARTESIAN_POINT('Ctrl Pts',(-35.5219282427889,-84.238982422185,108.421536708732));
#37463=CARTESIAN_POINT('Ctrl Pts',(-32.9440320186257,-86.5365567862535,
108.26358818554));
#37464=CARTESIAN_POINT('Ctrl Pts',(-33.4587560273279,-89.9512135763613,
108.105639662347));
#37465=CARTESIAN_POINT('Ctrl Pts',(-36.5992129203138,-91.3867838191251,
107.947691139155));
#37466=CARTESIAN_POINT('Ctrl Pts',(-39.0463676630991,-89.8404170424041,
107.815285734098));
#37467=CARTESIAN_POINT('Ctrl Pts',(-39.4232157558696,-88.293722122157,107.735529836772));
#37468=CARTESIAN_POINT('Ctrl Pts',(-39.4235551911591,-87.7682412648602,
107.708423447177));
#37469=CARTESIAN_POINT('Ctrl Pts',(-39.4248378354749,-87.7666901941256,
108.791576552823));
#37470=CARTESIAN_POINT('Ctrl Pts',(-39.4269819669572,-87.3842072109777,
108.771825719159));
#37471=CARTESIAN_POINT('Ctrl Pts',(-39.183987538194,-85.9847711220175,108.699425377765));
#37472=CARTESIAN_POINT('Ctrl Pts',(-37.0970138838616,-84.2187462913202,
108.57437552864));
#37473=CARTESIAN_POINT('Ctrl Pts',(-33.7881604641648,-85.2066067039222,
108.416427005448));
#37474=CARTESIAN_POINT('Ctrl Pts',(-32.8065173074963,-88.517318877192,108.258478482255));
#37475=CARTESIAN_POINT('Ctrl Pts',(-35.0421044524555,-91.1491282972506,
108.100529959063));
#37476=CARTESIAN_POINT('Ctrl Pts',(-38.4177929438602,-90.72226834617,107.944895982585));
#37477=CARTESIAN_POINT('Ctrl Pts',(-39.4298020103746,-88.7356858130984,
107.841911513838));
#37478=CARTESIAN_POINT('Ctrl Pts',(-39.4331960788118,-87.7677421217272,
107.791576552823));
#37479=CARTESIAN_POINT('Origin',(-36.3549260746835,-87.7685555885722,124.208423447177));
#37480=CARTESIAN_POINT('',(-39.4267610875431,-87.7711482491674,109.791576552823));
#37481=CARTESIAN_POINT('',(-39.4310569711989,-87.7662875373292,109.708423447177));
#37482=CARTESIAN_POINT('',(-39.4284260746835,-87.768555588572,124.208423447177));
#37483=CARTESIAN_POINT('Ctrl Pts',(-39.4310569711989,-87.7662875373292,
109.708423447177));
#37484=CARTESIAN_POINT('Ctrl Pts',(-39.4322960926139,-87.6166677872432,
109.700657262876));
#37485=CARTESIAN_POINT('Ctrl Pts',(-39.3546331967087,-86.4540177992007,
109.640241570843));
#37486=CARTESIAN_POINT('Ctrl Pts',(-37.8732761190034,-84.4751586948984,
109.52717637108));
#37487=CARTESIAN_POINT('Ctrl Pts',(-34.4272253359264,-84.6967778557991,
109.369227847887));
#37488=CARTESIAN_POINT('Ctrl Pts',(-32.728961758079,-87.7034840352579,109.211279324695));
#37489=CARTESIAN_POINT('Ctrl Pts',(-34.3182506239731,-90.7691894929664,
109.053330801502));
#37490=CARTESIAN_POINT('Ctrl Pts',(-37.754129375528,-91.1143096400617,108.89538227831));
#37491=CARTESIAN_POINT('Ctrl Pts',(-39.3316611845371,-89.1574728635941,
108.780413160201));
#37492=CARTESIAN_POINT('Ctrl Pts',(-39.4316812456249,-87.9575770934212,
108.718093549824));
#37493=CARTESIAN_POINT('Ctrl Pts',(-39.4300190231571,-87.7711138662458,
108.708423447177));
#37494=CARTESIAN_POINT('Ctrl Pts',(-39.4267610875431,-87.7711482491674,
109.791576552823));
#37495=CARTESIAN_POINT('Ctrl Pts',(-39.4209016416215,-87.0521420397502,
109.754389432211));
#37496=CARTESIAN_POINT('Ctrl Pts',(-38.8116906656652,-85.3062201297381,
109.664552803868));
#37497=CARTESIAN_POINT('Ctrl Pts',(-35.9114810653333,-84.1692214210988,
109.522066667795));
#37498=CARTESIAN_POINT('Ctrl Pts',(-33.098603051042,-86.1722440278901,109.364118144602));
#37499=CARTESIAN_POINT('Ctrl Pts',(-33.2381341114487,-89.6225939175359,
109.20616962141));
#37500=CARTESIAN_POINT('Ctrl Pts',(-36.2035655990193,-91.3919433535738,
109.048221098218));
#37501=CARTESIAN_POINT('Ctrl Pts',(-38.9182551690064,-90.0656308344281,
108.910023408688));
#37502=CARTESIAN_POINT('Ctrl Pts',(-39.4212663870998,-88.4037864916013,
108.82447522689));
#37503=CARTESIAN_POINT('Ctrl Pts',(-39.4248378354749,-87.7666901941256,
108.791576552823));
#37504=CARTESIAN_POINT('Origin',(-36.3549260746835,-87.7685555885722,124.208423447177));
#37505=CARTESIAN_POINT('',(-39.4332678666261,-87.7678707816449,110.791576552823));
#37506=CARTESIAN_POINT('',(-39.4236452988987,-87.7682071722042,110.708423447177));
#37507=CARTESIAN_POINT('',(-39.4284260746835,-87.768555588572,124.208423447177));
#37508=CARTESIAN_POINT('Ctrl Pts',(-39.4236452988987,-87.7682071722042,
110.708423447177));
#37509=CARTESIAN_POINT('Ctrl Pts',(-39.4241445943381,-87.2796756480956,
110.683220975927));
#37510=CARTESIAN_POINT('Ctrl Pts',(-39.0844835270856,-85.7712276403467,
110.605368996946));
#37511=CARTESIAN_POINT('Ctrl Pts',(-36.7289586650204,-84.1613476130271,
110.474867510234));
#37512=CARTESIAN_POINT('Ctrl Pts',(-33.5388964962196,-85.4834238308911,
110.316918987042));
#37513=CARTESIAN_POINT('Ctrl Pts',(-32.9020426949109,-88.8773595086493,
110.158970463849));
#37514=CARTESIAN_POINT('Ctrl Pts',(-35.3958132509259,-91.2659764064493,
110.001021940657));
#37515=CARTESIAN_POINT('Ctrl Pts',(-38.5938084373591,-90.5220575062303,
109.850839601766));
#37516=CARTESIAN_POINT('Ctrl Pts',(-39.4238956825823,-88.6309890913328,
109.753306770606));
#37517=CARTESIAN_POINT('Ctrl Pts',(-39.4310569711989,-87.7662875373292,
109.708423447177));
#37518=CARTESIAN_POINT('Ctrl Pts',(-39.4332678666261,-87.7678707816449,
110.791576552823));
#37519=CARTESIAN_POINT('Ctrl Pts',(-39.4333835106076,-87.7299144909416,
110.789602652993));
#37520=CARTESIAN_POINT('Ctrl Pts',(-39.4156195689302,-86.6796669871756,
110.734979245433));
#37521=CARTESIAN_POINT('Ctrl Pts',(-38.2231009204979,-84.66021635197,110.627706330142));
#37522=CARTESIAN_POINT('Ctrl Pts',(-34.7734204516813,-84.5050160949677,
110.46975780695));
#37523=CARTESIAN_POINT('Ctrl Pts',(-32.7576430317562,-87.3087678398475,
110.311809283757));
#37524=CARTESIAN_POINT('Ctrl Pts',(-34.0034127407753,-90.5293951545392,
110.153860760565));
#37525=CARTESIAN_POINT('Ctrl Pts',(-37.381228070904,-91.2468531980925,109.995912237372));
#37526=CARTESIAN_POINT('Ctrl Pts',(-39.252338964875,-89.3842212342544,109.875150834792));
#37527=CARTESIAN_POINT('Ctrl Pts',(-39.4291974423792,-88.0701106901465,
109.807038939942));
#37528=CARTESIAN_POINT('Ctrl Pts',(-39.4267610875431,-87.7711482491674,
109.791576552823));
#37529=CARTESIAN_POINT('Origin',(-36.3549260746835,-87.7685555885722,124.208423447177));
#37530=CARTESIAN_POINT('',(-39.4249634829513,-87.7666135330092,111.791576552823));
#37531=CARTESIAN_POINT('',(-39.4298261000276,-87.7711513822271,111.708423447177));
#37532=CARTESIAN_POINT('',(-39.4284260746835,-87.768555588572,124.208423447177));
#37533=CARTESIAN_POINT('Ctrl Pts',(-39.4298261000276,-87.7711513822271,
111.708423447177));
#37534=CARTESIAN_POINT('Ctrl Pts',(-39.4224452207145,-86.9488393862918,
111.665784688979));
#37535=CARTESIAN_POINT('Ctrl Pts',(-38.6609852839478,-85.0990845351561,
111.570496423049));
#37536=CARTESIAN_POINT('Ctrl Pts',(-35.5445999861014,-84.2336975457609,
111.422558649389));
#37537=CARTESIAN_POINT('Ctrl Pts',(-32.9520311196661,-86.5146992660596,
111.264610126197));
#37538=CARTESIAN_POINT('Ctrl Pts',(-33.444763614499,-89.9325343795896,111.106661603004));
#37539=CARTESIAN_POINT('Ctrl Pts',(-36.5760519035439,-91.3883557378978,
110.948713079812));
#37540=CARTESIAN_POINT('Ctrl Pts',(-39.0392098427808,-89.8535958737908,
110.815967027869));
#37541=CARTESIAN_POINT('Ctrl Pts',(-39.4231015355509,-88.3002479562603,
110.735870483658));
#37542=CARTESIAN_POINT('Ctrl Pts',(-39.4236452988987,-87.7682071722042,
110.708423447177));
#37543=CARTESIAN_POINT('Ctrl Pts',(-39.4249634829513,-87.7666135330092,
111.791576552823));
#37544=CARTESIAN_POINT('Ctrl Pts',(-39.4271631600903,-87.3907660068182,
111.772166366045));
#37545=CARTESIAN_POINT('Ctrl Pts',(-39.1897288443723,-85.998126327073,111.700106671536));
#37546=CARTESIAN_POINT('Ctrl Pts',(-37.1197916542217,-84.2235829922162,
111.575397469297));
#37547=CARTESIAN_POINT('Ctrl Pts',(-33.8046641643864,-85.1901812455926,
111.417448946105));
#37548=CARTESIAN_POINT('Ctrl Pts',(-32.8017815859054,-88.494513098026,111.259500422912));
#37549=CARTESIAN_POINT('Ctrl Pts',(-35.0204270513993,-91.1406413556617,
111.10155189972));
#37550=CARTESIAN_POINT('Ctrl Pts',(-38.4061746688924,-90.7345413083506,
110.945577276357));
#37551=CARTESIAN_POINT('Ctrl Pts',(-39.4302989575766,-88.742316433115,110.842252160724));
#37552=CARTESIAN_POINT('Ctrl Pts',(-39.4332678666261,-87.7678707816449,
110.791576552823));
#37553=CARTESIAN_POINT('Origin',(-36.3549260746835,-87.7685555885722,124.208423447177));
#37554=CARTESIAN_POINT('',(-39.4265849952197,-87.7711115889072,112.791576552823));
#37555=CARTESIAN_POINT('',(-39.4312327529812,-87.7663532935098,112.708423447177));
#37556=CARTESIAN_POINT('',(-39.4284260746835,-87.768555588572,124.208423447177));
#37557=CARTESIAN_POINT('Ctrl Pts',(-39.4312327529812,-87.7663532935098,
112.708423447177));
#37558=CARTESIAN_POINT('Ctrl Pts',(-39.4323936164487,-87.6233176105418,
112.700997909761));
#37559=CARTESIAN_POINT('Ctrl Pts',(-39.358587288045,-86.4673154971078,112.640922864614));
#37560=CARTESIAN_POINT('Ctrl Pts',(-37.8943917712909,-84.4849759684705,
112.528198311736));
#37561=CARTESIAN_POINT('Ctrl Pts',(-34.446988838572,-84.684463298183,112.370249788544));
#37562=CARTESIAN_POINT('Ctrl Pts',(-32.7294545705478,-87.6802033091648,
112.212301265352));
#37563=CARTESIAN_POINT('Ctrl Pts',(-34.299025051591,-90.7560496447713,112.054352742159));
#37564=CARTESIAN_POINT('Ctrl Pts',(-37.7326184628711,-91.1232259801486,
111.896404218966));
#37565=CARTESIAN_POINT('Ctrl Pts',(-39.3273916051006,-89.1707887114988,
111.781094453973));
#37566=CARTESIAN_POINT('Ctrl Pts',(-39.4315589866606,-87.9642142146455,
111.71843419671));
#37567=CARTESIAN_POINT('Ctrl Pts',(-39.4298261000276,-87.7711513822271,
111.708423447177));
#37568=CARTESIAN_POINT('Ctrl Pts',(-39.4265849952197,-87.7711115889072,
112.791576552823));
#37569=CARTESIAN_POINT('Ctrl Pts',(-39.4208859423477,-87.05858818249,112.754730079096));
#37570=CARTESIAN_POINT('Ctrl Pts',(-38.820534631401,-85.3192830484007,112.66523409764));
#37571=CARTESIAN_POINT('Ctrl Pts',(-35.9346015224717,-84.1664482422435,
112.523088608452));
#37572=CARTESIAN_POINT('Ctrl Pts',(-33.1089201003701,-86.1513681293118,
112.365140085259));
#37573=CARTESIAN_POINT('Ctrl Pts',(-33.2262935723694,-89.6025427011582,
112.207191562067));
#37574=CARTESIAN_POINT('Ctrl Pts',(-36.1803029811607,-91.3908969362198,
112.049243038874));
#37575=CARTESIAN_POINT('Ctrl Pts',(-38.9101651204659,-90.0788161109398,
111.91070470246));
#37576=CARTESIAN_POINT('Ctrl Pts',(-39.4211966065552,-88.4102403407061,
111.824815873776));
#37577=CARTESIAN_POINT('Ctrl Pts',(-39.4249634829513,-87.7666135330092,
111.791576552823));
#37578=CARTESIAN_POINT('Origin',(-36.3549260746835,-87.7685555885722,124.208423447177));
#37579=CARTESIAN_POINT('',(-39.4333271029731,-87.7679866768215,113.791576552823));
#37580=CARTESIAN_POINT('',(-39.4236711760032,-87.7681022535202,113.708423447177));
#37581=CARTESIAN_POINT('',(-39.4284260746835,-87.768555588572,124.208423447177));
#37582=CARTESIAN_POINT('Ctrl Pts',(-39.4236711760032,-87.7681022535202,
113.708423447178));
#37583=CARTESIAN_POINT('Ctrl Pts',(-39.4243123526912,-87.2861840776058,
113.683561622813));
#37584=CARTESIAN_POINT('Ctrl Pts',(-39.0911306006805,-85.7845536494958,
113.606050290717));
#37585=CARTESIAN_POINT('Ctrl Pts',(-36.7521128317831,-84.1638236384041,
113.475889450891));
#37586=CARTESIAN_POINT('Ctrl Pts',(-33.5536273739847,-85.4653892155019,
113.317940927699));
#37587=CARTESIAN_POINT('Ctrl Pts',(-32.8949942504612,-88.8551656954239,
113.159992404506));
#37588=CARTESIAN_POINT('Ctrl Pts',(-35.3733760828904,-91.2597458392159,
113.002043881314));
#37589=CARTESIAN_POINT('Ctrl Pts',(-38.5833465123841,-90.5347358539682,
112.851520895538));
#37590=CARTESIAN_POINT('Ctrl Pts',(-39.4241627118446,-88.6374877472081,
112.753647417492));
#37591=CARTESIAN_POINT('Ctrl Pts',(-39.4312327529812,-87.7663532935098,
112.708423447177));
#37592=CARTESIAN_POINT('Ctrl Pts',(-39.4333271029731,-87.7679866768215,
113.791576552823));
#37593=CARTESIAN_POINT('Ctrl Pts',(-39.4334077862495,-87.7365823354763,
113.789943299879));
#37594=CARTESIAN_POINT('Ctrl Pts',(-39.4188026175281,-86.6929051608962,
113.735660539204));
#37595=CARTESIAN_POINT('Ctrl Pts',(-38.2430210496827,-84.672275977644,113.628728270799));
#37596=CARTESIAN_POINT('Ctrl Pts',(-34.7944082359535,-84.4949285269366,
113.470779747607));
#37597=CARTESIAN_POINT('Ctrl Pts',(-32.7606694855963,-87.2856791701479,
113.312831224414));
#37598=CARTESIAN_POINT('Ctrl Pts',(-33.9857338701916,-90.514239175922,113.154882701222));
#37599=CARTESIAN_POINT('Ctrl Pts',(-37.3588727708761,-91.2533713792378,
112.996934178029));
#37600=CARTESIAN_POINT('Ctrl Pts',(-39.247216754307,-89.3975720466728,112.875832128563));
#37601=CARTESIAN_POINT('Ctrl Pts',(-39.4290292542553,-88.0767047836455,
112.807379586827));
#37602=CARTESIAN_POINT('Ctrl Pts',(-39.4265849952197,-87.7711115889072,
112.791576552823));
#37603=CARTESIAN_POINT('Origin',(-36.3549260746835,-87.7685555885722,124.208423447177));
#37604=CARTESIAN_POINT('',(-39.4250943850934,-87.7665395826249,114.791576552823));
#37605=CARTESIAN_POINT('',(-39.4296319167269,-87.7711845285468,114.708423447178));
#37606=CARTESIAN_POINT('',(-39.4284260746835,-87.768555588572,124.208423447177));
#37607=CARTESIAN_POINT('Ctrl Pts',(-39.4296319167269,-87.7711845285468,
114.708423447177));
#37608=CARTESIAN_POINT('Ctrl Pts',(-39.4222700858053,-86.9553091377705,
114.666125335865));
#37609=CARTESIAN_POINT('Ctrl Pts',(-38.6709154553017,-85.1119080614529,
114.571177716821));
#37610=CARTESIAN_POINT('Ctrl Pts',(-35.5673140086676,-84.2285673137265,
114.423580590046));
#37611=CARTESIAN_POINT('Ctrl Pts',(-32.9601522791593,-86.4928751310124,
114.265632066854));
#37612=CARTESIAN_POINT('Ctrl Pts',(-33.4309287026749,-89.9138036211001,
114.107683543661));
#37613=CARTESIAN_POINT('Ctrl Pts',(-36.5528046140307,-91.3897009648648,
113.949735020469));
#37614=CARTESIAN_POINT('Ctrl Pts',(-39.0321124688702,-89.8668909092713,
113.816648321641));
#37615=CARTESIAN_POINT('Ctrl Pts',(-39.4229545425604,-88.3067348769492,
113.736211130544));
#37616=CARTESIAN_POINT('Ctrl Pts',(-39.4236711760032,-87.7681022535202,
113.708423447178));
#37617=CARTESIAN_POINT('Ctrl Pts',(-39.4250943850934,-87.7665395826249,
114.791576552823));
#37618=CARTESIAN_POINT('Ctrl Pts',(-39.4273438878649,-87.3973277353349,
114.772507012931));
#37619=CARTESIAN_POINT('Ctrl Pts',(-39.195415474559,-86.0114816654255,114.700787965308));
#37620=CARTESIAN_POINT('Ctrl Pts',(-37.1425381500136,-84.2285672718597,
114.576419409954));
#37621=CARTESIAN_POINT('Ctrl Pts',(-33.821272475107,-85.1738591706804,114.418470886761));
#37622=CARTESIAN_POINT('Ctrl Pts',(-32.7971934613455,-88.4716833974796,
114.260522363569));
#37623=CARTESIAN_POINT('Ctrl Pts',(-34.9988024045514,-91.1320030246078,
114.102573840377));
#37624=CARTESIAN_POINT('Ctrl Pts',(-38.3944877717556,-90.7468118088923,
113.946258570128));
#37625=CARTESIAN_POINT('Ctrl Pts',(-39.4308068818404,-88.7489320262378,
113.84259280761));
#37626=CARTESIAN_POINT('Ctrl Pts',(-39.4333271029731,-87.7679866768215,
113.791576552823));
#37627=CARTESIAN_POINT('Origin',(-36.3549260746835,-87.7685555885722,124.208423447177));
#37628=CARTESIAN_POINT('',(-39.4264122098445,-87.7710709637358,115.791576552823));
#37629=CARTESIAN_POINT('',(-39.4314046551684,-87.7664230789163,115.708423447177));
#37630=CARTESIAN_POINT('',(-39.4284260746835,-87.768555588572,124.208423447177));
#37631=CARTESIAN_POINT('Ctrl Pts',(-39.4314046551684,-87.7664230789163,
115.708423447177));
#37632=CARTESIAN_POINT('Ctrl Pts',(-39.4324871906633,-87.6299690823578,
115.701338556647));
#37633=CARTESIAN_POINT('Ctrl Pts',(-39.3624944732727,-86.4806100262057,
115.641604158386));
#37634=CARTESIAN_POINT('Ctrl Pts',(-37.9154438949567,-84.494928565653,115.529220252393));
#37635=CARTESIAN_POINT('Ctrl Pts',(-34.4668311220138,-84.6722760142634,
115.371271729201));
#37636=CARTESIAN_POINT('Ctrl Pts',(-32.7300966188443,-87.6569259838135,
115.213323206008));
#37637=CARTESIAN_POINT('Ctrl Pts',(-34.2798847390797,-90.7427871209372,
115.055374682816));
#37638=CARTESIAN_POINT('Ctrl Pts',(-37.7110497287778,-91.1320029848287,
114.897426159623));
#37639=CARTESIAN_POINT('Ctrl Pts',(-39.3230747918906,-89.1841085015426,
114.781775747744));
#37640=CARTESIAN_POINT('Ctrl Pts',(-39.4314335392548,-87.9708494624013,
114.718774843595));
#37641=CARTESIAN_POINT('Ctrl Pts',(-39.4296319167269,-87.7711845285468,
114.708423447177));
#37642=CARTESIAN_POINT('Ctrl Pts',(-39.4264122098445,-87.7710709637358,
115.791576552823));
#37643=CARTESIAN_POINT('Ctrl Pts',(-39.4208786170309,-87.0650342694146,
115.755070725982));
#37644=CARTESIAN_POINT('Ctrl Pts',(-38.8293124187647,-85.3323581275192,
115.665915391411));
#37645=CARTESIAN_POINT('Ctrl Pts',(-35.9577393128856,-84.1638235957717,
115.524110549109));
#37646=CARTESIAN_POINT('Ctrl Pts',(-33.1193709742919,-86.1305588681857,
115.366162025916));
#37647=CARTESIAN_POINT('Ctrl Pts',(-33.2145820402631,-89.5824159495559,
115.208213502724));
#37648=CARTESIAN_POINT('Ctrl Pts',(-36.1570475329969,-91.3897010076914,
115.050264979531));
#37649=CARTESIAN_POINT('Ctrl Pts',(-38.9020112016885,-90.0919926097959,
114.911385996231));
#37650=CARTESIAN_POINT('Ctrl Pts',(-39.4211331867032,-88.4166927603047,
114.825156520661));
#37651=CARTESIAN_POINT('Ctrl Pts',(-39.4250943850934,-87.7665395826249,
114.791576552823));
#37652=CARTESIAN_POINT('Origin',(-36.3549260746835,-87.7685555885722,124.208423447177));
#37653=CARTESIAN_POINT('',(-39.4333760082338,-87.768103846536,116.791576552823));
#37654=CARTESIAN_POINT('',(-39.4237038206158,-87.7679979949716,116.708423447177));
#37655=CARTESIAN_POINT('',(-39.4284260746835,-87.768555588572,124.208423447177));
#37656=CARTESIAN_POINT('Ctrl Pts',(-39.4237038206158,-87.7679979949716,
116.708423447177));
#37657=CARTESIAN_POINT('Ctrl Pts',(-39.4244821252083,-87.2926955099761,
116.683902269698));
#37658=CARTESIAN_POINT('Ctrl Pts',(-39.0977193329511,-85.7978828462761,
116.606731584489));
#37659=CARTESIAN_POINT('Ctrl Pts',(-36.7752506219235,-84.1664482848449,
116.476911391548));
#37660=CARTESIAN_POINT('Ctrl Pts',(-33.568473749851,-85.4474495604007,116.318962868356));
#37661=CARTESIAN_POINT('Ctrl Pts',(-32.8880884545876,-88.8329270784509,
116.161014345163));
#37662=CARTESIAN_POINT('Ctrl Pts',(-35.3509793903652,-91.2533713380237,
116.003065821971));
#37663=CARTESIAN_POINT('Ctrl Pts',(-38.5728137685938,-90.5473934305567,
115.852202189309));
#37664=CARTESIAN_POINT('Ctrl Pts',(-39.4244426117584,-88.643991206724,115.753988064378));
#37665=CARTESIAN_POINT('Ctrl Pts',(-39.4314046551684,-87.7664230789163,
115.708423447177));
#37666=CARTESIAN_POINT('Ctrl Pts',(-39.4333760082338,-87.768103846536,116.791576552823));
#37667=CARTESIAN_POINT('Ctrl Pts',(-39.4334274954906,-87.7432505565165,
116.790283946765));
#37668=CARTESIAN_POINT('Ctrl Pts',(-39.421942007279,-86.7061395822215,116.736341832976));
#37669=CARTESIAN_POINT('Ctrl Pts',(-38.2628633333592,-84.6844632617075,
116.629750211456));
#37670=CARTESIAN_POINT('Ctrl Pts',(-34.8154603598683,-84.4849759296366,
116.471801688264));
#37671=CARTESIAN_POINT('Ctrl Pts',(-32.7638441292674,-87.2626104087614,
116.313853165071));
#37672=CARTESIAN_POINT('Ctrl Pts',(-33.9681526807548,-90.4989699947938,
116.155904641879));
#37673=CARTESIAN_POINT('Ctrl Pts',(-37.336476078086,-91.2597458805054,115.997956118686));
#37674=CARTESIAN_POINT('Ctrl Pts',(-39.2420423334472,-89.4109239111188,
115.876513422334));
#37675=CARTESIAN_POINT('Ctrl Pts',(-39.4288592864976,-88.0832959446915,
115.807720233713));
#37676=CARTESIAN_POINT('Ctrl Pts',(-39.4264122098445,-87.7710709637358,
115.791576552823));
#37677=CARTESIAN_POINT('Origin',(-36.3549260746835,-87.7685555885722,124.208423447177));
#37678=CARTESIAN_POINT('',(-39.4252304227193,-87.7664686533939,117.791576552823));
#37679=CARTESIAN_POINT('',(-39.4294367136551,-87.7712132051017,117.708423447177));
#37680=CARTESIAN_POINT('',(-39.4284260746835,-87.768555588572,124.208423447177));
#37681=CARTESIAN_POINT('Ctrl Pts',(-39.4294367136551,-87.7712132051017,
117.708423447177));
#37682=CARTESIAN_POINT('Ctrl Pts',(-39.4221062956345,-86.9617760103423,
117.66646598275));
#37683=CARTESIAN_POINT('Ctrl Pts',(-38.680776320305,-85.1247491336954,117.571859010592));
#37684=CARTESIAN_POINT('Ctrl Pts',(-35.5900605041904,-84.2235830341421,
117.424602530703));
#37685=CARTESIAN_POINT('Ctrl Pts',(-32.9684134039925,-86.4711035918391,
117.26665400751));
#37686=CARTESIAN_POINT('Ctrl Pts',(-33.4172143461837,-89.8949844147526,
117.108705484318));
#37687=CARTESIAN_POINT('Ctrl Pts',(-36.5295491661419,-91.390896893379,116.950756961125));
#37688=CARTESIAN_POINT('Ctrl Pts',(-39.0249547704469,-89.8801809263355,
116.817329615412));
#37689=CARTESIAN_POINT('Ctrl Pts',(-39.4228110246384,-88.313219172827,116.736551777429));
#37690=CARTESIAN_POINT('Ctrl Pts',(-39.4237038206158,-87.7679979949716,
116.708423447177));
#37691=CARTESIAN_POINT('Ctrl Pts',(-39.4252304227193,-87.7664686533939,
117.791576552823));
#37692=CARTESIAN_POINT('Ctrl Pts',(-39.4275240548214,-87.4038926151218,
117.772847659816));
#37693=CARTESIAN_POINT('Ctrl Pts',(-39.2010477052606,-86.0248372386501,
117.701469259079));
#37694=CARTESIAN_POINT('Ctrl Pts',(-37.1652521728484,-84.2336975039545,
117.577441350611));
#37695=CARTESIAN_POINT('Ctrl Pts',(-33.8379852474627,-85.1576440741897,
117.419492827418));
#37696=CARTESIAN_POINT('Ctrl Pts',(-32.7927520208408,-88.4488247072137,
117.261544304226));
#37697=CARTESIAN_POINT('Ctrl Pts',(-34.9772336702029,-91.123226019824,117.103595781034));
#37698=CARTESIAN_POINT('Ctrl Pts',(-38.3827275640396,-90.7590545474582,
116.946939863899));
#37699=CARTESIAN_POINT('Ctrl Pts',(-39.4313303532814,-88.7555570337355,
116.842933454495));
#37700=CARTESIAN_POINT('Ctrl Pts',(-39.4333760082338,-87.768103846536,116.791576552823));
#37701=CARTESIAN_POINT('Origin',(-36.3549260746835,-87.7685555885722,124.208423447177));
#37702=CARTESIAN_POINT('',(-39.4262429517989,-87.7710264527958,118.791576552823));
#37703=CARTESIAN_POINT('',(-39.4315723149004,-87.7664967944779,118.708423447177));
#37704=CARTESIAN_POINT('',(-39.4284260746835,-87.768555588572,124.208423447177));
#37705=CARTESIAN_POINT('Ctrl Pts',(-39.4315723149004,-87.7664967944779,
118.708423447177));
#37706=CARTESIAN_POINT('Ctrl Pts',(-39.4325767499313,-87.6366221253453,
118.701679203533));
#37707=CARTESIAN_POINT('Ctrl Pts',(-39.3663549509798,-86.4939013295593,
118.642285452157));
#37708=CARTESIAN_POINT('Ctrl Pts',(-37.9364316789807,-84.5050161335647,
118.53024219305));
#37709=CARTESIAN_POINT('Ctrl Pts',(-34.4867512509629,-84.6602163887321,
118.372293669858));
#37710=CARTESIAN_POINT('Ctrl Pts',(-32.7308881175633,-87.6336532609701,
118.214345146665));
#37711=CARTESIAN_POINT('Ctrl Pts',(-34.2608299797916,-90.7294019705626,
118.056396623473));
#37712=CARTESIAN_POINT('Ctrl Pts',(-37.6894250821856,-91.1406413157804,
117.89844810028));
#37713=CARTESIAN_POINT('Ctrl Pts',(-39.3187092839115,-89.197430905212,117.782457041515));
#37714=CARTESIAN_POINT('Ctrl Pts',(-39.4313047280353,-87.9774825222761,
117.719115490481));
#37715=CARTESIAN_POINT('Ctrl Pts',(-39.4294367136551,-87.7712132051017,
117.708423447177));
#37716=CARTESIAN_POINT('Ctrl Pts',(-39.4262429517989,-87.7710264527958,
118.791576552823));
#37717=CARTESIAN_POINT('Ctrl Pts',(-39.4208794784184,-87.0714804470721,
118.755411372868));
#37718=CARTESIAN_POINT('Ctrl Pts',(-38.8380242352711,-85.345445065365,118.666596685182));
#37719=CARTESIAN_POINT('Ctrl Pts',(-35.980893479922,-84.1613475703659,118.525132489766));
#37720=CARTESIAN_POINT('Ctrl Pts',(-33.1299552486368,-86.109817141451,118.367183966573));
#37721=CARTESIAN_POINT('Ctrl Pts',(-33.2029999836058,-89.5622144129554,
118.209235443381));
#37722=CARTESIAN_POINT('Ctrl Pts',(-36.1338002432087,-91.3883557807084,
118.051286920188));
#37723=CARTESIAN_POINT('Ctrl Pts',(-38.893793144385,-90.1051597784844,117.912067290002));
#37724=CARTESIAN_POINT('Ctrl Pts',(-39.4210763378607,-88.4231439891081,
117.825497167547));
#37725=CARTESIAN_POINT('Ctrl Pts',(-39.4252304227193,-87.7664686533939,
117.791576552823));
#37726=CARTESIAN_POINT('Origin',(-36.3549260746835,-87.7685555885722,124.208423447177));
#37727=CARTESIAN_POINT('',(-39.4334142380496,-87.7682219888642,119.791576552823));
#37728=CARTESIAN_POINT('',(-39.4237431936346,-87.7678945631787,119.708423447177));
#37729=CARTESIAN_POINT('',(-39.4284260746835,-87.768555588572,124.208423447177));
#37730=CARTESIAN_POINT('Ctrl Pts',(-39.4237431936346,-87.7678945631786,
119.708423447177));
#37731=CARTESIAN_POINT('Ctrl Pts',(-39.4246537466801,-87.2992099811667,
119.684242916584));
#37732=CARTESIAN_POINT('Ctrl Pts',(-39.1042499609049,-85.8112150040598,
119.60741287826));
#37733=CARTESIAN_POINT('Ctrl Pts',(-36.7983710787885,-84.169221463673,119.477933332205));
#37734=CARTESIAN_POINT('Ctrl Pts',(-33.5834350118328,-85.4296055945461,
119.319984809013));
#37735=CARTESIAN_POINT('Ctrl Pts',(-32.8813255943857,-88.8106445822591,
119.16203628582));
#37736=CARTESIAN_POINT('Ctrl Pts',(-35.3286240906017,-91.2468531569549,
119.004087762628));
#37737=CARTESIAN_POINT('Ctrl Pts',(-38.5622100531239,-90.5600298609509,
118.85288348308));
#37738=CARTESIAN_POINT('Ctrl Pts',(-39.4247355430135,-88.6504997010273,
118.754328711263));
#37739=CARTESIAN_POINT('Ctrl Pts',(-39.4315723149004,-87.7664967944779,
118.708423447177));
#37740=CARTESIAN_POINT('Ctrl Pts',(-39.4334142380496,-87.7682219888642,
119.791576552823));
#37741=CARTESIAN_POINT('Ctrl Pts',(-39.4334426828812,-87.7499190193576,
119.79062459365));
#37742=CARTESIAN_POINT('Ctrl Pts',(-39.4250380396833,-86.7193701130363,
119.737023126747));
#37743=CARTESIAN_POINT('Ctrl Pts',(-38.2826268362602,-84.6967778194338,
119.630772152113));
#37744=CARTESIAN_POINT('Ctrl Pts',(-34.8365760123942,-84.4751586559665,
119.472823628921));
#37745=CARTESIAN_POINT('Ctrl Pts',(-32.7671668042656,-87.2395625351253,
119.314875105728));
#37746=CARTESIAN_POINT('Ctrl Pts',(-33.9506699106112,-90.4835882261257,
119.156926582536));
#37747=CARTESIAN_POINT('Ctrl Pts',(-37.3140389097867,-91.26597644781,118.998978059343));
#37748=CARTESIAN_POINT('Ctrl Pts',(-39.2368154766846,-89.424276702295,118.877194716105));
#37749=CARTESIAN_POINT('Ctrl Pts',(-39.4286876583739,-88.0898841404161,
118.808060880599));
#37750=CARTESIAN_POINT('Ctrl Pts',(-39.4262429517989,-87.7710264527958,
118.791576552823));
#37751=CARTESIAN_POINT('Origin',(-36.3549260746835,-87.7685555885722,124.208423447177));
#37752=CARTESIAN_POINT('',(-39.4253676065904,-87.7664047027925,120.791576552823));
#37753=CARTESIAN_POINT('',(-39.4292404520863,-87.7712393069318,120.708423447177));
#37754=CARTESIAN_POINT('',(-39.4284260746835,-87.768555588572,124.208423447177));
#37755=CARTESIAN_POINT('Ctrl Pts',(-39.4292404520863,-87.7712393069318,
120.708423447177));
#37756=CARTESIAN_POINT('Ctrl Pts',(-39.4219533239201,-86.9682420907583,
120.666806629636));
#37757=CARTESIAN_POINT('Ctrl Pts',(-38.6905685426978,-85.137604773249,120.572540304363));
#37758=CARTESIAN_POINT('Ctrl Pts',(-35.6128382743126,-84.2187463335991,
120.42562447136));
#37759=CARTESIAN_POINT('Ctrl Pts',(-32.976814280225,-86.4493848551693,120.267675948167));
#37760=CARTESIAN_POINT('Ctrl Pts',(-33.4036210489072,-89.8760778724798,
120.109727424975));
#37761=CARTESIAN_POINT('Ctrl Pts',(-36.5062865485562,-91.3919433106791,
119.951778901783));
#37762=CARTESIAN_POINT('Ctrl Pts',(-39.0177365106944,-89.8934657391649,
119.818010909183));
#37763=CARTESIAN_POINT('Ctrl Pts',(-39.4226711528978,-88.3197009265046,
119.736892424315));
#37764=CARTESIAN_POINT('Ctrl Pts',(-39.4237431936346,-87.7678945631786,
119.708423447177));
#37765=CARTESIAN_POINT('Ctrl Pts',(-39.4253676065904,-87.7664047027925,
120.791576552823));
#37766=CARTESIAN_POINT('Ctrl Pts',(-39.4277029355786,-87.4104612245052,
120.773188306702));
#37767=CARTESIAN_POINT('Ctrl Pts',(-39.2066381265416,-86.0381804949055,
120.70215055285));
#37768=CARTESIAN_POINT('Ctrl Pts',(-37.1879239172525,-84.2389823785756,
120.578463291268));
#37769=CARTESIAN_POINT('Ctrl Pts',(-33.8548061047563,-85.1415322964398,
120.420514768075));
#37770=CARTESIAN_POINT('Ctrl Pts',(-32.7884553507106,-88.4259400742007,
120.262566244883));
#37771=CARTESIAN_POINT('Ctrl Pts',(-34.9557227571499,-91.1143096798933,
120.10461772169));
#37772=CARTESIAN_POINT('Ctrl Pts',(-38.3708934336136,-90.771269574952,119.94762115767));
#37773=CARTESIAN_POINT('Ctrl Pts',(-39.4318694994647,-88.7621917748598,
119.843274101381));
#37774=CARTESIAN_POINT('Ctrl Pts',(-39.4334142380496,-87.7682219888642,
119.791576552823));
#37775=CARTESIAN_POINT('Origin',(-36.3549260746835,-87.7685555885722,124.208423447177));
#37776=CARTESIAN_POINT('',(-39.4252046443693,-87.771569957437,121.791576552823));
#37777=CARTESIAN_POINT('',(-39.4317256223809,-87.7666280037969,121.708423447177));
#37778=CARTESIAN_POINT('',(-39.4284260746835,-87.768555588572,124.208423447177));
#37779=CARTESIAN_POINT('',(-37.1487253572165,-90.7377785423179,122.));
#37780=CARTESIAN_POINT('Ctrl Pts',(-37.1487253572165,-90.7377785423179,
122.));
#37781=CARTESIAN_POINT('Ctrl Pts',(-38.1309639469881,-90.4751844899402,
121.947350492269));
#37782=CARTESIAN_POINT('Ctrl Pts',(-39.2306604626821,-89.4374467038025,
121.877876009877));
#37783=CARTESIAN_POINT('Ctrl Pts',(-39.427545797006,-88.0970456694337,121.808401527484));
#37784=CARTESIAN_POINT('Ctrl Pts',(-39.4252046443693,-87.771569957437,121.791576552823));
#37785=CARTESIAN_POINT('',(-35.5592173021306,-90.7428549624115,122.));
#37786=CARTESIAN_POINT('Origin',(-36.3549260746835,-87.7685555885722,122.));
#37787=CARTESIAN_POINT('Ctrl Pts',(-35.5592126670536,-90.7428672848631,
122.));
#37788=CARTESIAN_POINT('Ctrl Pts',(-36.5061789753531,-90.9937479094032,
121.949053726697));
#37789=CARTESIAN_POINT('Ctrl Pts',(-38.5667278271917,-90.5388459125472,
121.851861542423));
#37790=CARTESIAN_POINT('Ctrl Pts',(-39.4250621347381,-88.6569026988886,
121.754669358149));
#37791=CARTESIAN_POINT('Ctrl Pts',(-39.4317256223809,-87.7666280037969,
121.708423447177));
#37792=CARTESIAN_POINT('Origin',(-87.7685555885722,-36.3549260746835,114.));
#37793=CARTESIAN_POINT('',(-90.2820658539789,-36.3546686125247,107.387416697508));
#37794=CARTESIAN_POINT('',(-90.2841457375043,-36.3584993178544,107.112583302492));
#37795=CARTESIAN_POINT('',(-90.2860555885722,-36.3549260746835,114.));
#37796=CARTESIAN_POINT('',(-89.6820215852369,-34.7189388713081,107.));
#37797=CARTESIAN_POINT('Ctrl Pts',(-90.2841457375043,-36.3584993178544,
107.112583302492));
#37798=CARTESIAN_POINT('Ctrl Pts',(-90.2790005338084,-35.7658644382975,
107.075055534995));
#37799=CARTESIAN_POINT('Ctrl Pts',(-90.0677774166561,-35.1701225143786,
107.037527767497));
#37800=CARTESIAN_POINT('Ctrl Pts',(-89.6820215852368,-34.718938871308,107.));
#37801=CARTESIAN_POINT('',(-90.2860555885722,-36.3549260746835,107.));
#37802=CARTESIAN_POINT('Origin',(-87.7685555885722,-36.3549260746835,107.));
#37803=CARTESIAN_POINT('',(-90.2860555885722,-36.3549260746835,106.));
#37804=CARTESIAN_POINT('',(-90.2860555885722,-36.3549260746835,114.));
#37805=CARTESIAN_POINT('Origin',(-87.7685555885722,-36.3549260746835,106.));
#37806=CARTESIAN_POINT('',(-85.8514453318972,-34.7163981307897,107.));
#37807=CARTESIAN_POINT('Origin',(-87.7685555885722,-36.3549260746835,107.));
#37808=CARTESIAN_POINT('Ctrl Pts',(-85.8514364858568,-34.7163919634214,
107.));
#37809=CARTESIAN_POINT('Ctrl Pts',(-86.3742570429706,-34.1076768998287,
107.050946273303));
#37810=CARTESIAN_POINT('Ctrl Pts',(-87.2139815516724,-33.767500538132,107.101892546605));
#37811=CARTESIAN_POINT('Ctrl Pts',(-88.012652412444,-33.8452633218798,107.152838819908));
#37812=CARTESIAN_POINT('Ctrl Pts',(-88.8380244157852,-33.9256258689062,
107.205488327639));
#37813=CARTESIAN_POINT('Ctrl Pts',(-89.6195518767751,-34.4523397509922,
107.25813783537));
#37814=CARTESIAN_POINT('Ctrl Pts',(-90.0034364925517,-35.1871265187104,
107.3107873431));
#37815=CARTESIAN_POINT('Ctrl Pts',(-90.1896796411383,-35.543611242337,107.336330461236));
#37816=CARTESIAN_POINT('Ctrl Pts',(-90.2823278504789,-35.9490709929857,
107.361873579372));
#37817=CARTESIAN_POINT('Ctrl Pts',(-90.2820658539789,-36.3546686125247,
107.387416697508));
#37818=CARTESIAN_POINT('Origin',(-87.7685555885722,-36.3549260746835,114.));
#37819=CARTESIAN_POINT('',(-90.2873603706715,-36.3570215567213,108.387416697508));
#37820=CARTESIAN_POINT('',(-90.2899626929787,-36.35425976501,108.112583302492));
#37821=CARTESIAN_POINT('',(-90.2860555885722,-36.3549260746835,114.));
#37822=CARTESIAN_POINT('Ctrl Pts',(-90.2899626929787,-36.35425976501,108.112583302492));
#37823=CARTESIAN_POINT('Ctrl Pts',(-90.2900905289486,-36.3178026272376,
108.110268755777));
#37824=CARTESIAN_POINT('Ctrl Pts',(-90.289367578041,-36.2813507261708,108.107954209062));
#37825=CARTESIAN_POINT('Ctrl Pts',(-90.2877779615632,-36.2449367233117,
108.105639662347));
#37826=CARTESIAN_POINT('Ctrl Pts',(-90.2516186028016,-35.4166193198727,
108.052990154616));
#37827=CARTESIAN_POINT('Ctrl Pts',(-89.7670151876795,-34.6079118173993,
108.000340646886));
#37828=CARTESIAN_POINT('Ctrl Pts',(-89.0536407575369,-34.1853501417969,
107.947691139155));
#37829=CARTESIAN_POINT('Ctrl Pts',(-88.3402663273943,-33.7627884661946,
107.895041631424));
#37830=CARTESIAN_POINT('Ctrl Pts',(-87.3981208822312,-33.7263726174632,
107.842392123693));
#37831=CARTESIAN_POINT('Ctrl Pts',(-86.6543416473799,-34.0927743114382,
107.789742615962));
#37832=CARTESIAN_POINT('Ctrl Pts',(-85.9105624125286,-34.4591760054132,
107.737093108232));
#37833=CARTESIAN_POINT('Ctrl Pts',(-85.3651493879892,-35.2283952420945,
107.684443600501));
#37834=CARTESIAN_POINT('Ctrl Pts',(-85.2652957176433,-36.0513826441264,
107.63179409277));
#37835=CARTESIAN_POINT('Ctrl Pts',(-85.1654420472974,-36.8743700461582,
107.579144585039));
#37836=CARTESIAN_POINT('Ctrl Pts',(-85.5111477311451,-37.7511256135406,
107.526495077308));
#37837=CARTESIAN_POINT('Ctrl Pts',(-86.1458177411936,-38.284877504064,107.473845569577));
#37838=CARTESIAN_POINT('Ctrl Pts',(-86.7804877512421,-38.8186293945873,
107.421196061847));
#37839=CARTESIAN_POINT('Ctrl Pts',(-87.7041220874913,-39.0093776082516,
107.368546554116));
#37840=CARTESIAN_POINT('Ctrl Pts',(-88.4977390365037,-38.7692237409335,
107.315897046385));
#37841=CARTESIAN_POINT('Ctrl Pts',(-89.291355985516,-38.5290698736153,107.263247538654));
#37842=CARTESIAN_POINT('Ctrl Pts',(-89.9549555472913,-37.8580139253148,
107.210598030923));
#37843=CARTESIAN_POINT('Ctrl Pts',(-90.187920793802,-37.0637279762933,107.157948523192));
#37844=CARTESIAN_POINT('Ctrl Pts',(-90.2548319596038,-36.8355969583622,
107.142826782959));
#37845=CARTESIAN_POINT('Ctrl Pts',(-90.2862189872318,-36.597300379031,107.127705042726));
#37846=CARTESIAN_POINT('Ctrl Pts',(-90.2841457375043,-36.3584993178544,
107.112583302492));
#37847=CARTESIAN_POINT('Ctrl Pts',(-90.2820658539789,-36.3546686125247,
107.387416697508));
#37848=CARTESIAN_POINT('Ctrl Pts',(-90.2817878229584,-36.7850893244963,
107.414523087103));
#37849=CARTESIAN_POINT('Ctrl Pts',(-90.1768791354039,-37.2156652972639,
107.441629476698));
#37850=CARTESIAN_POINT('Ctrl Pts',(-89.968158095568,-37.5880327152623,107.468735866293));
#37851=CARTESIAN_POINT('Ctrl Pts',(-89.5627533122445,-38.3112924907458,
107.521385374024));
#37852=CARTESIAN_POINT('Ctrl Pts',(-88.7657019750341,-38.8149523883624,
107.574034881755));
#37853=CARTESIAN_POINT('Ctrl Pts',(-87.9384522552337,-38.8708033725724,
107.626684389485));
#37854=CARTESIAN_POINT('Ctrl Pts',(-87.1112025354333,-38.9266543567824,
107.679333897216));
#37855=CARTESIAN_POINT('Ctrl Pts',(-86.2537544330426,-38.5346964275858,
107.731983404947));
#37856=CARTESIAN_POINT('Ctrl Pts',(-85.754762083387,-37.8725606130825,107.784632912678));
#37857=CARTESIAN_POINT('Ctrl Pts',(-85.2557697337313,-37.2104247985793,
107.837282420409));
#37858=CARTESIAN_POINT('Ctrl Pts',(-85.1152331368106,-36.2781110987695,
107.889931928139));
#37859=CARTESIAN_POINT('Ctrl Pts',(-85.396890099688,-35.4982975349368,107.94258143587));
#37860=CARTESIAN_POINT('Ctrl Pts',(-85.6785470625655,-34.7184839711041,
107.995230943601));
#37861=CARTESIAN_POINT('Ctrl Pts',(-86.3823975852411,-34.0911705432485,
108.047880451332));
#37862=CARTESIAN_POINT('Ctrl Pts',(-87.1893482785224,-33.900726745334,108.100529959063));
#37863=CARTESIAN_POINT('Ctrl Pts',(-87.9962989718038,-33.7102829474194,
108.153179466794));
#37864=CARTESIAN_POINT('Ctrl Pts',(-88.9063498356909,-33.9567087794459,
108.205828974524));
#37865=CARTESIAN_POINT('Ctrl Pts',(-89.5069496938256,-34.5282974064535,
108.258478482255));
#37866=CARTESIAN_POINT('Ctrl Pts',(-89.9972377460577,-34.9949027025053,
108.301457887339));
#37867=CARTESIAN_POINT('Ctrl Pts',(-90.2813089864897,-35.6781950787427,
108.344437292424));
#37868=CARTESIAN_POINT('Ctrl Pts',(-90.2873603706715,-36.3570215567213,
108.387416697508));
#37869=CARTESIAN_POINT('Origin',(-87.7685555885722,-36.3549260746835,114.));
#37870=CARTESIAN_POINT('',(-90.2882105526124,-36.3530683167515,109.387416697508));
#37871=CARTESIAN_POINT('',(-90.2831164663313,-36.3533981324289,109.112583302492));
#37872=CARTESIAN_POINT('',(-90.2860555885722,-36.3549260746835,114.));
#37873=CARTESIAN_POINT('Ctrl Pts',(-90.2831164663313,-36.3533981324289,
109.112583302492));
#37874=CARTESIAN_POINT('Ctrl Pts',(-90.2848727217426,-36.0401068000473,
109.092832468829));
#37875=CARTESIAN_POINT('Ctrl Pts',(-90.2305755265925,-35.7274022874004,
109.073081635165));
#37876=CARTESIAN_POINT('Ctrl Pts',(-90.1174359487622,-35.4376760917933,
109.053330801502));
#37877=CARTESIAN_POINT('Ctrl Pts',(-89.8158414348707,-34.665357219817,109.000681293771));
#37878=CARTESIAN_POINT('Ctrl Pts',(-89.0961201091845,-34.0563194728835,
108.94803178604));
#37879=CARTESIAN_POINT('Ctrl Pts',(-88.2845464977982,-33.8866598038377,
108.89538227831));
#37880=CARTESIAN_POINT('Ctrl Pts',(-87.4729728864118,-33.7170001347919,
108.842732770579));
#37881=CARTESIAN_POINT('Ctrl Pts',(-86.5695469893253,-33.9867185436337,
108.790083262848));
#37882=CARTESIAN_POINT('Ctrl Pts',(-85.983823594119,-34.5735444470518,108.737433755117));
#37883=CARTESIAN_POINT('Ctrl Pts',(-85.3981001989128,-35.1603703504699,
108.684784247386));
#37884=CARTESIAN_POINT('Ctrl Pts',(-85.1300793055867,-36.0643037484642,
108.632134739655));
#37885=CARTESIAN_POINT('Ctrl Pts',(-85.301263297264,-36.8755557473365,108.579485231925));
#37886=CARTESIAN_POINT('Ctrl Pts',(-85.4724472889414,-37.6868077462088,
108.526835724194));
#37887=CARTESIAN_POINT('Ctrl Pts',(-86.0828361656222,-38.4053783459591,
108.474186216463));
#37888=CARTESIAN_POINT('Ctrl Pts',(-86.8557210844333,-38.7055236108094,
108.421536708732));
#37889=CARTESIAN_POINT('Ctrl Pts',(-87.6286060032443,-39.0056688756597,
108.368887201001));
#37890=CARTESIAN_POINT('Ctrl Pts',(-88.5639869641856,-38.88738880561,108.316237693271));
#37891=CARTESIAN_POINT('Ctrl Pts',(-89.2378197934557,-38.4042851183828,
108.26358818554));
#37892=CARTESIAN_POINT('Ctrl Pts',(-89.8820299799204,-37.9424193515166,
108.213253224524));
#37893=CARTESIAN_POINT('Ctrl Pts',(-90.2871826157732,-37.1471012301236,
108.162918263508));
#37894=CARTESIAN_POINT('Ctrl Pts',(-90.2899626929787,-36.35425976501,108.112583302492));
#37895=CARTESIAN_POINT('Ctrl Pts',(-90.2873603706715,-36.3570215567213,
108.387416697508));
#37896=CARTESIAN_POINT('Ctrl Pts',(-90.2887218950127,-36.5097533525287,
108.397086800155));
#37897=CARTESIAN_POINT('Ctrl Pts',(-90.2760094311365,-36.6622590745572,
108.406756902801));
#37898=CARTESIAN_POINT('Ctrl Pts',(-90.2484051643446,-36.8120198580747,
108.416427005448));
#37899=CARTESIAN_POINT('Ctrl Pts',(-90.0981119243468,-37.6274022606995,
108.469076513179));
#37900=CARTESIAN_POINT('Ctrl Pts',(-89.5063765919689,-38.3614156439603,
108.521726020909));
#37901=CARTESIAN_POINT('Ctrl Pts',(-88.7414549288688,-38.6813077555619,
108.57437552864));
#37902=CARTESIAN_POINT('Ctrl Pts',(-87.9765332657687,-39.0011998671635,
108.627025036371));
#37903=CARTESIAN_POINT('Ctrl Pts',(-87.0384252719463,-38.9069707071058,
108.679674544102));
#37904=CARTESIAN_POINT('Ctrl Pts',(-86.3524071884949,-38.4413368770482,
108.732324051833));
#37905=CARTESIAN_POINT('Ctrl Pts',(-85.6663891050434,-37.9757030469905,
108.784973559563));
#37906=CARTESIAN_POINT('Ctrl Pts',(-85.2324609319629,-37.1386645469329,
108.837623067294));
#37907=CARTESIAN_POINT('Ctrl Pts',(-85.2473377736386,-36.3096804193602,
108.890272575025));
#37908=CARTESIAN_POINT('Ctrl Pts',(-85.2622146153143,-35.4806962917874,
108.942922082756));
#37909=CARTESIAN_POINT('Ctrl Pts',(-85.7258964717462,-34.6597665366996,
108.995571590487));
#37910=CARTESIAN_POINT('Ctrl Pts',(-86.4281800465863,-34.2190469963083,
109.048221098218));
#37911=CARTESIAN_POINT('Ctrl Pts',(-87.1304636214265,-33.778327455917,109.100870605948));
#37912=CARTESIAN_POINT('Ctrl Pts',(-88.0713489146749,-33.7178181302223,
109.153520113679));
#37913=CARTESIAN_POINT('Ctrl Pts',(-88.8242999729847,-34.0649500886831,
109.20616962141));
#37914=CARTESIAN_POINT('Ctrl Pts',(-89.5772510312945,-34.4120820471438,
109.258819129141));
#37915=CARTESIAN_POINT('Ctrl Pts',(-90.1422678546657,-35.16685528976,109.311468636872));
#37916=CARTESIAN_POINT('Ctrl Pts',(-90.2632086162776,-35.987104802477,109.364118144603));
#37917=CARTESIAN_POINT('Ctrl Pts',(-90.2810482559013,-36.1080975555683,
109.371884328904));
#37918=CARTESIAN_POINT('Ctrl Pts',(-90.2892255154112,-36.2305149668762,
109.379650513206));
#37919=CARTESIAN_POINT('Ctrl Pts',(-90.2882105526124,-36.3530683167515,
109.387416697508));
#37920=CARTESIAN_POINT('Origin',(-87.7685555885722,-36.3549260746835,114.));
#37921=CARTESIAN_POINT('',(-90.2821396611156,-36.3546406872729,110.387416697508));
#37922=CARTESIAN_POINT('',(-90.2846917996912,-36.3570497197296,110.112583302492));
#37923=CARTESIAN_POINT('',(-90.2860555885722,-36.3549260746835,114.));
#37924=CARTESIAN_POINT('Ctrl Pts',(-90.2846917996912,-36.3570497197296,
110.112583302492));
#37925=CARTESIAN_POINT('Ctrl Pts',(-90.2798923348767,-35.7681126342544,
110.07539618188));
#37926=CARTESIAN_POINT('Ctrl Pts',(-90.0733338262189,-35.1761419702344,
110.038209061269));
#37927=CARTESIAN_POINT('Ctrl Pts',(-89.6956382757642,-34.728599334682,110.001021940657));
#37928=CARTESIAN_POINT('Ctrl Pts',(-89.1608970945044,-34.0949686834569,
109.948372432926));
#37929=CARTESIAN_POINT('Ctrl Pts',(-88.2831137156981,-33.7508423251229,
109.895722925195));
#37930=CARTESIAN_POINT('Ctrl Pts',(-87.4602178832996,-33.8522246973141,
109.843073417464));
#37931=CARTESIAN_POINT('Ctrl Pts',(-86.6373220509011,-33.9536070695053,
109.790423909734));
#37932=CARTESIAN_POINT('Ctrl Pts',(-85.8693137649103,-34.5004981722218,
109.737774402003));
#37933=CARTESIAN_POINT('Ctrl Pts',(-85.5043579080477,-35.2449732690051,
109.685124894272));
#37934=CARTESIAN_POINT('Ctrl Pts',(-85.139402051185,-35.9894483657884,109.632475386541));
#37935=CARTESIAN_POINT('Ctrl Pts',(-85.1774986234505,-36.9315074566384,
109.57982587881));
#37936=CARTESIAN_POINT('Ctrl Pts',(-85.60137711239,-37.6440823198458,109.52717637108));
#37937=CARTESIAN_POINT('Ctrl Pts',(-86.0252556013295,-38.3566571830533,
109.474526863349));
#37938=CARTESIAN_POINT('Ctrl Pts',(-86.834916006943,-38.8397478186181,109.421877355618));
#37939=CARTESIAN_POINT('Ctrl Pts',(-87.6633111187983,-38.8743525536714,
109.369227847887));
#37940=CARTESIAN_POINT('Ctrl Pts',(-88.4917062306535,-38.9089572887246,
109.316578340156));
#37941=CARTESIAN_POINT('Ctrl Pts',(-89.3388360487506,-38.4950761232663,
109.263928832425));
#37942=CARTESIAN_POINT('Ctrl Pts',(-89.8206671067506,-37.8203355420275,
109.211279324695));
#37943=CARTESIAN_POINT('Ctrl Pts',(-90.1217450012257,-37.3987158266868,
109.178380650627));
#37944=CARTESIAN_POINT('Ctrl Pts',(-90.280191097441,-36.8752429116366,109.14548197656));
#37945=CARTESIAN_POINT('Ctrl Pts',(-90.2831164663313,-36.3533981324289,
109.112583302492));
#37946=CARTESIAN_POINT('Ctrl Pts',(-90.2882105526124,-36.3530683167515,
109.387416697508));
#37947=CARTESIAN_POINT('Ctrl Pts',(-90.2823447500771,-37.061344276473,109.432300020937));
#37948=CARTESIAN_POINT('Ctrl Pts',(-89.9694529522308,-37.7741606696804,
109.477183344366));
#37949=CARTESIAN_POINT('Ctrl Pts',(-89.440291210746,-38.2427518568799,109.522066667795));
#37950=CARTESIAN_POINT('Ctrl Pts',(-88.8195683437496,-38.792423615748,109.574716175526));
#37951=CARTESIAN_POINT('Ctrl Pts',(-87.9012579099043,-39.0060413506665,
109.627365683257));
#37952=CARTESIAN_POINT('Ctrl Pts',(-87.1016619698773,-38.7867646999753,
109.680015190987));
#37953=CARTESIAN_POINT('Ctrl Pts',(-86.3020660298503,-38.5674880492842,
109.732664698718));
#37954=CARTESIAN_POINT('Ctrl Pts',(-85.6211845836416,-37.9153170129834,
109.785314206449));
#37955=CARTESIAN_POINT('Ctrl Pts',(-85.3676848856873,-37.1259034177897,
109.83796371418));
#37956=CARTESIAN_POINT('Ctrl Pts',(-85.1141851877331,-36.336489822596,109.890613221911));
#37957=CARTESIAN_POINT('Ctrl Pts',(-85.2880672380334,-35.4098336685093,
109.943262729642));
#37958=CARTESIAN_POINT('Ctrl Pts',(-85.8105042509258,-34.7660204291389,
109.995912237372));
#37959=CARTESIAN_POINT('Ctrl Pts',(-86.3329412638183,-34.1222071897685,
110.048561745103));
#37960=CARTESIAN_POINT('Ctrl Pts',(-87.203933239303,-33.7612368651145,110.101211252834));
#37961=CARTESIAN_POINT('Ctrl Pts',(-88.0286292114484,-33.8467498637978,
110.153860760565));
#37962=CARTESIAN_POINT('Ctrl Pts',(-88.8533251835939,-33.9322628624812,
110.206510268296));
#37963=CARTESIAN_POINT('Ctrl Pts',(-89.6317251524002,-34.464259184502,110.259159776027));
#37964=CARTESIAN_POINT('Ctrl Pts',(-90.0109533284357,-35.2015663866826,
110.311809283757));
#37965=CARTESIAN_POINT('Ctrl Pts',(-90.1924837475362,-35.5545034675106,
110.337011755008));
#37966=CARTESIAN_POINT('Ctrl Pts',(-90.2825486333846,-35.9544851278314,
110.362214226258));
#37967=CARTESIAN_POINT('Ctrl Pts',(-90.2821396611156,-36.3546406872729,
110.387416697508));
#37968=CARTESIAN_POINT('Origin',(-87.7685555885722,-36.3549260746835,114.));
#37969=CARTESIAN_POINT('',(-90.2872023475779,-36.3570522860146,111.387416697508));
#37970=CARTESIAN_POINT('',(-90.2900214942874,-36.3543651501874,111.112583302492));
#37971=CARTESIAN_POINT('',(-90.2860555885722,-36.3549260746835,114.));
#37972=CARTESIAN_POINT('Ctrl Pts',(-90.2900214942874,-36.3543651501874,
111.112583302492));
#37973=CARTESIAN_POINT('Ctrl Pts',(-90.2901162181278,-36.323275200018,111.110609402663));
#37974=CARTESIAN_POINT('Ctrl Pts',(-90.2895904165067,-36.2921885273613,
111.108635502833));
#37975=CARTESIAN_POINT('Ctrl Pts',(-90.2884341100943,-36.261125324813,111.106661603004));
#37976=CARTESIAN_POINT('Ctrl Pts',(-90.2575921380264,-35.4325815970888,
111.054012095273));
#37977=CARTESIAN_POINT('Ctrl Pts',(-89.7781837013239,-34.6207354483563,
111.001362587542));
#37978=CARTESIAN_POINT('Ctrl Pts',(-89.0675413245081,-34.19362498464,110.948713079812));
#37979=CARTESIAN_POINT('Ctrl Pts',(-88.3568989476923,-33.7665145209237,
110.896063572081));
#37980=CARTESIAN_POINT('Ctrl Pts',(-87.4150226307631,-33.7241397422238,
110.84341406435));
#37981=CARTESIAN_POINT('Ctrl Pts',(-86.6688976790302,-34.0857106098954,
110.790764556619));
#37982=CARTESIAN_POINT('Ctrl Pts',(-85.9227727272973,-34.447281477567,110.738115048888));
#37983=CARTESIAN_POINT('Ctrl Pts',(-85.3723991407606,-35.2127979916102,
110.685465541158));
#37984=CARTESIAN_POINT('Ctrl Pts',(-85.2672804155176,-36.0352248818261,
110.632816033427));
#37985=CARTESIAN_POINT('Ctrl Pts',(-85.1621616902746,-36.857651772042,110.580166525696));
#37986=CARTESIAN_POINT('Ctrl Pts',(-85.5022978263254,-37.7369890384306,
110.527517017965));
#37987=CARTESIAN_POINT('Ctrl Pts',(-86.1334932786358,-38.2746025024174,
110.474867510234));
#37988=CARTESIAN_POINT('Ctrl Pts',(-86.7646887309461,-38.8122159664043,
110.422218002503));
#37989=CARTESIAN_POINT('Ctrl Pts',(-87.686943499516,-39.0081056279894,110.369568494773));
#37990=CARTESIAN_POINT('Ctrl Pts',(-88.4821674098618,-38.7734678895427,
110.316918987042));
#37991=CARTESIAN_POINT('Ctrl Pts',(-89.2773913202076,-38.5388301510961,
110.264269479311));
#37992=CARTESIAN_POINT('Ctrl Pts',(-89.9455843723293,-37.8736650126178,
110.21161997158));
#37993=CARTESIAN_POINT('Ctrl Pts',(-90.1838314065334,-37.0795149713205,
110.158970463849));
#37994=CARTESIAN_POINT('Ctrl Pts',(-90.2538010611725,-36.8462847684481,
110.14350807673));
#37995=CARTESIAN_POINT('Ctrl Pts',(-90.2866874148855,-36.6019294806421,
110.128045689611));
#37996=CARTESIAN_POINT('Ctrl Pts',(-90.2846917996912,-36.3570497197296,
110.112583302492));
#37997=CARTESIAN_POINT('Ctrl Pts',(-90.2821396611156,-36.3546406872729,
110.387416697508));
#37998=CARTESIAN_POINT('Ctrl Pts',(-90.2816942652385,-36.7904346270357,
110.414863733989));
#37999=CARTESIAN_POINT('Ctrl Pts',(-90.1739419384852,-37.2264348206415,
110.442310770469));
#38000=CARTESIAN_POINT('Ctrl Pts',(-89.9601636138683,-37.6020990605625,
110.46975780695));
#38001=CARTESIAN_POINT('Ctrl Pts',(-89.5500893400006,-38.3227064499215,
110.522407314681));
#38002=CARTESIAN_POINT('Ctrl Pts',(-88.7498844090003,-38.8213031462991,
110.575056822411));
#38003=CARTESIAN_POINT('Ctrl Pts',(-87.9223095576387,-38.8718579193271,
110.627706330142));
#38004=CARTESIAN_POINT('Ctrl Pts',(-87.0947347062772,-38.9224126923551,
110.680355837873));
#38005=CARTESIAN_POINT('Ctrl Pts',(-86.2397899345544,-38.5249255420335,
110.733005345604));
#38006=CARTESIAN_POINT('Ctrl Pts',(-85.7450514538097,-37.8595912235122,
110.785654853335));
#38007=CARTESIAN_POINT('Ctrl Pts',(-85.250312973065,-37.1942569049909,110.838304361066));
#38008=CARTESIAN_POINT('Ctrl Pts',(-85.1157807832985,-36.2610754182697,
110.890953868796));
#38009=CARTESIAN_POINT('Ctrl Pts',(-85.402443006904,-35.4830903996067,110.943603376527));
#38010=CARTESIAN_POINT('Ctrl Pts',(-85.6891052305094,-34.7051053809437,
110.996252884258));
#38011=CARTESIAN_POINT('Ctrl Pts',(-86.3969618674869,-34.0823168303388,
111.048902391989));
#38012=CARTESIAN_POINT('Ctrl Pts',(-87.2051168757209,-33.8970564665951,
111.10155189972));
#38013=CARTESIAN_POINT('Ctrl Pts',(-88.0132718839549,-33.7117961028514,
111.154201407451));
#38014=CARTESIAN_POINT('Ctrl Pts',(-88.9217252634454,-33.964063925969,111.206850915181));
#38015=CARTESIAN_POINT('Ctrl Pts',(-89.5186434892735,-34.5394981545195,
111.259500422912));
#38016=CARTESIAN_POINT('Ctrl Pts',(-90.0020639995955,-35.0055196234347,
111.302139181111));
#38017=CARTESIAN_POINT('Ctrl Pts',(-90.2811566785782,-35.6834975602078,
111.344777939309));
#38018=CARTESIAN_POINT('Ctrl Pts',(-90.2872023475779,-36.3570522860146,
111.387416697508));
#38019=CARTESIAN_POINT('Origin',(-87.7685555885722,-36.3549260746835,114.));
#38020=CARTESIAN_POINT('',(-90.2883545352501,-36.3531221775569,112.387416697508));
#38021=CARTESIAN_POINT('',(-90.2832193840218,-36.3533353394049,112.112583302492));
#38022=CARTESIAN_POINT('',(-90.2860555885722,-36.3549260746835,114.));
#38023=CARTESIAN_POINT('Ctrl Pts',(-90.2832193840218,-36.3533353394049,
112.112583302492));
#38024=CARTESIAN_POINT('Ctrl Pts',(-90.285021136811,-36.0454791015047,112.093173115714));
#38025=CARTESIAN_POINT('Ctrl Pts',(-90.2326349187801,-35.7382146453077,
112.073762928937));
#38026=CARTESIAN_POINT('Ctrl Pts',(-90.1232772119999,-35.4527772953472,
112.054352742159));
#38027=CARTESIAN_POINT('Ctrl Pts',(-89.8266479474545,-34.6785376584215,
112.001703234428));
#38028=CARTESIAN_POINT('Ctrl Pts',(-89.1108519870612,-34.0648905600084,
111.949053726697));
#38029=CARTESIAN_POINT('Ctrl Pts',(-88.3003845444894,-33.8900235805582,
111.896404218967));
#38030=CARTESIAN_POINT('Ctrl Pts',(-87.4899171019176,-33.7151566011079,
111.843754711236));
#38031=CARTESIAN_POINT('Ctrl Pts',(-86.5847781771673,-33.9790697406205,
111.791105203505));
#38032=CARTESIAN_POINT('Ctrl Pts',(-85.9952987374956,-34.5621219905731,
111.738455695774));
#38033=CARTESIAN_POINT('Ctrl Pts',(-85.4058192978239,-35.1451742405258,
111.685806188043));
#38034=CARTESIAN_POINT('Ctrl Pts',(-85.1319993432308,-36.0473656009185,
111.633156680312));
#38035=CARTESIAN_POINT('Ctrl Pts',(-85.2979709862033,-36.8597013379772,
111.580507172582));
#38036=CARTESIAN_POINT('Ctrl Pts',(-85.4639426291757,-37.6720370750359,
111.527857664851));
#38037=CARTESIAN_POINT('Ctrl Pts',(-86.0697058697138,-38.3945171887604,
111.47520815712));
#38038=CARTESIAN_POINT('Ctrl Pts',(-86.8406471544457,-38.6996163062034,
111.422558649389));
#38039=CARTESIAN_POINT('Ctrl Pts',(-87.6115884391776,-39.0047154236463,
111.369909141658));
#38040=CARTESIAN_POINT('Ctrl Pts',(-88.5477077681033,-38.8924335448076,
111.317259633927));
#38041=CARTESIAN_POINT('Ctrl Pts',(-89.2246296788495,-38.4136719520304,
111.264610126197));
#38042=CARTESIAN_POINT('Ctrl Pts',(-89.8761728899335,-37.9528597659424,
111.213934518295));
#38043=CARTESIAN_POINT('Ctrl Pts',(-90.2875896646038,-37.1525323626734,
111.163258910394));
#38044=CARTESIAN_POINT('Ctrl Pts',(-90.2900214942874,-36.3543651501874,
111.112583302492));
#38045=CARTESIAN_POINT('Ctrl Pts',(-90.2872023475779,-36.3570522860146,
111.387416697508));
#38046=CARTESIAN_POINT('Ctrl Pts',(-90.2886217528483,-36.5151898102095,
111.39742744704));
#38047=CARTESIAN_POINT('Ctrl Pts',(-90.274990291039,-36.6730835186588,111.407438196572));
#38048=CARTESIAN_POINT('Ctrl Pts',(-90.2454186297744,-36.8279331239087,
111.417448946105));
#38049=CARTESIAN_POINT('Ctrl Pts',(-90.0898924722816,-37.6423332307638,
111.470098453835));
#38050=CARTESIAN_POINT('Ctrl Pts',(-89.4934570851304,-38.3725328104906,
111.522747961566));
#38051=CARTESIAN_POINT('Ctrl Pts',(-88.7264973812031,-38.6875069876263,
111.575397469297));
#38052=CARTESIAN_POINT('Ctrl Pts',(-87.9595376772757,-39.0024811647619,
111.628046977028));
#38053=CARTESIAN_POINT('Ctrl Pts',(-87.0220536565721,-38.9022299393065,
111.680696484759));
#38054=CARTESIAN_POINT('Ctrl Pts',(-86.3390394437353,-38.4322006798194,
111.73334599249));
#38055=CARTESIAN_POINT('Ctrl Pts',(-85.6560252308984,-37.9621714203324,
111.78599550022));
#38056=CARTESIAN_POINT('Ctrl Pts',(-85.2274808259284,-37.1223641268137,
111.838645007951));
#38057=CARTESIAN_POINT('Ctrl Pts',(-85.2476803180234,-36.2934926649875,
111.891294515682));
#38058=CARTESIAN_POINT('Ctrl Pts',(-85.2678798101183,-35.4646212031613,
111.943944023413));
#38059=CARTESIAN_POINT('Ctrl Pts',(-85.7368231992784,-34.6466855730277,
111.996593531144));
#38060=CARTESIAN_POINT('Ctrl Pts',(-86.4419221311623,-34.210484454314,112.049243038874));
#38061=CARTESIAN_POINT('Ctrl Pts',(-87.1470210630461,-33.7742833356004,
112.101892546605));
#38062=CARTESIAN_POINT('Ctrl Pts',(-88.0882755376538,-33.7198167283067,
112.154542054336));
#38063=CARTESIAN_POINT('Ctrl Pts',(-88.8389821524022,-34.071776240586,112.207191562067));
#38064=CARTESIAN_POINT('Ctrl Pts',(-89.5896887671506,-34.4237357528653,
112.259841069798));
#38065=CARTESIAN_POINT('Ctrl Pts',(-90.1498475220396,-35.1821213847176,
112.312490577529));
#38066=CARTESIAN_POINT('Ctrl Pts',(-90.2655189637697,-36.0031305425708,
112.365140085259));
#38067=CARTESIAN_POINT('Ctrl Pts',(-90.2818329362183,-36.1189233483053,
112.372565622676));
#38068=CARTESIAN_POINT('Ctrl Pts',(-90.2893053970622,-36.2359618288104,
112.379991160092));
#38069=CARTESIAN_POINT('Ctrl Pts',(-90.2883545352501,-36.3531221775569,
112.387416697508));
#38070=CARTESIAN_POINT('Origin',(-87.7685555885722,-36.3549260746835,114.));
#38071=CARTESIAN_POINT('',(-90.2821608570194,-36.3545547485103,113.387416697508));
#38072=CARTESIAN_POINT('',(-90.2845475626897,-36.3570196913561,113.112583302492));
#38073=CARTESIAN_POINT('',(-90.2860555885722,-36.3549260746835,114.));
#38074=CARTESIAN_POINT('Ctrl Pts',(-90.2845475626897,-36.3570196913561,
113.112583302492));
#38075=CARTESIAN_POINT('Ctrl Pts',(-90.279879475621,-35.7733926616976,113.075736828766));
#38076=CARTESIAN_POINT('Ctrl Pts',(-90.0774218583082,-35.1868434749016,
113.03889035504));
#38077=CARTESIAN_POINT('Ctrl Pts',(-89.7060411910088,-34.7410066577834,
113.002043881314));
#38078=CARTESIAN_POINT('Ctrl Pts',(-89.1753795743932,-34.1039554945146,
112.949394373583));
#38079=CARTESIAN_POINT('Ctrl Pts',(-88.2998239243827,-33.7541999769884,
112.896744865852));
#38080=CARTESIAN_POINT('Ctrl Pts',(-87.4762940804989,-33.8502964504088,
112.844095358121));
#38081=CARTESIAN_POINT('Ctrl Pts',(-86.652764236615,-33.9463929238291,112.791445850391));
#38082=CARTESIAN_POINT('Ctrl Pts',(-85.8812601988578,-34.4883413881961,
112.73879634266));
#38083=CARTESIAN_POINT('Ctrl Pts',(-85.5115315906271,-35.2304577484975,
112.686146834929));
#38084=CARTESIAN_POINT('Ctrl Pts',(-85.1418029823965,-35.9725741087989,
112.633497327198));
#38085=CARTESIAN_POINT('Ctrl Pts',(-85.1738498036924,-36.9148583650348,
112.580847819467));
#38086=CARTESIAN_POINT('Ctrl Pts',(-85.5931441154104,-37.6301402787808,
112.528198311736));
#38087=CARTESIAN_POINT('Ctrl Pts',(-86.0124384271283,-38.3454221925268,
112.475548804006));
#38088=CARTESIAN_POINT('Ctrl Pts',(-86.8189802292683,-38.8337017637829,
112.422899296275));
#38089=CARTESIAN_POINT('Ctrl Pts',(-87.6471360607603,-38.873624874096,112.370249788544));
#38090=CARTESIAN_POINT('Ctrl Pts',(-88.4752918922522,-38.9135479844091,
112.317600280813));
#38091=CARTESIAN_POINT('Ctrl Pts',(-89.325061753096,-38.5051146337791,112.264950773082));
#38092=CARTESIAN_POINT('Ctrl Pts',(-89.8112153991693,-37.833481870745,112.212301265351));
#38093=CARTESIAN_POINT('Ctrl Pts',(-90.118139770751,-37.4094585904653,112.179061944398));
#38094=CARTESIAN_POINT('Ctrl Pts',(-90.2801339402842,-36.8805292513542,
112.145822623445));
#38095=CARTESIAN_POINT('Ctrl Pts',(-90.2832193840218,-36.3533353394049,
112.112583302492));
#38096=CARTESIAN_POINT('Ctrl Pts',(-90.2883545352501,-36.3531221775569,
112.387416697508));
#38097=CARTESIAN_POINT('Ctrl Pts',(-90.2825634734112,-37.06666731736,112.432640667823));
#38098=CARTESIAN_POINT('Ctrl Pts',(-89.9643335620966,-37.7847328079434,
112.477864638137));
#38099=CARTESIAN_POINT('Ctrl Pts',(-89.4281350245541,-38.2534471541448,
112.523088608452));
#38100=CARTESIAN_POINT('Ctrl Pts',(-88.8038955150371,-38.7991219240113,
112.575738116183));
#38101=CARTESIAN_POINT('Ctrl Pts',(-87.884232367432,-39.00683877989,112.628387623914));
#38102=CARTESIAN_POINT('Ctrl Pts',(-87.0860608845605,-38.7824324438797,
112.681037131644));
#38103=CARTESIAN_POINT('Ctrl Pts',(-86.287889401689,-38.5580261078694,112.733686639375));
#38104=CARTESIAN_POINT('Ctrl Pts',(-85.6112095835511,-37.9014965799701,
112.786336147106));
#38105=CARTESIAN_POINT('Ctrl Pts',(-85.3627839355564,-37.1104715379333,
112.838985654837));
#38106=CARTESIAN_POINT('Ctrl Pts',(-85.1143582875617,-36.3194464958966,
112.891635162568));
#38107=CARTESIAN_POINT('Ctrl Pts',(-85.2941868097101,-35.3939259397225,
112.944284670298));
#38108=CARTESIAN_POINT('Ctrl Pts',(-85.8207469761043,-34.7534805393349,
112.996934178029));
#38109=CARTESIAN_POINT('Ctrl Pts',(-86.3473071424986,-34.1130351389473,
113.04958368576));
#38110=CARTESIAN_POINT('Ctrl Pts',(-87.2205989531388,-33.7576648943461,
113.102233193491));
#38111=CARTESIAN_POINT('Ctrl Pts',(-88.044728845656,-33.8484715018728,113.154882701222));
#38112=CARTESIAN_POINT('Ctrl Pts',(-88.8688587381731,-33.9392781093994,
113.207532208953));
#38113=CARTESIAN_POINT('Ctrl Pts',(-89.6438267125673,-34.4762615690537,
113.260181716683));
#38114=CARTESIAN_POINT('Ctrl Pts',(-90.0183128224397,-35.2159885952083,
113.312831224414));
#38115=CARTESIAN_POINT('Ctrl Pts',(-90.1951503332143,-35.5652979087166,
113.337693048779));
#38116=CARTESIAN_POINT('Ctrl Pts',(-90.2826860440414,-35.9598161742905,
113.362554873143));
#38117=CARTESIAN_POINT('Ctrl Pts',(-90.2821608570194,-36.3545547485103,
113.387416697508));
#38118=CARTESIAN_POINT('Origin',(-87.7685555885722,-36.3549260746835,114.));
#38119=CARTESIAN_POINT('',(-90.2870432922795,-36.3570794361236,114.387416697508));
#38120=CARTESIAN_POINT('',(-90.290070014705,-36.3544600797813,114.112583302492));
#38121=CARTESIAN_POINT('',(-90.2860555885722,-36.3549260746835,114.));
#38122=CARTESIAN_POINT('Ctrl Pts',(-90.290070014705,-36.3544600797813,114.112583302492));
#38123=CARTESIAN_POINT('Ctrl Pts',(-90.2901361022756,-36.3287368231238,
114.110950049548));
#38124=CARTESIAN_POINT('Ctrl Pts',(-90.2897761587525,-36.3030154606156,
114.109316796605));
#38125=CARTESIAN_POINT('Ctrl Pts',(-90.2889844577079,-36.2773073944353,
114.107683543661));
#38126=CARTESIAN_POINT('Ctrl Pts',(-90.2634631993918,-35.4485827107525,
114.05503403593));
#38127=CARTESIAN_POINT('Ctrl Pts',(-89.7892775084378,-34.6336750173297,
114.002384528199));
#38128=CARTESIAN_POINT('Ctrl Pts',(-89.081392256987,-34.2020103248314,113.949735020469));
#38129=CARTESIAN_POINT('Ctrl Pts',(-88.3735070055363,-33.7703456323331,
113.897085512738));
#38130=CARTESIAN_POINT('Ctrl Pts',(-87.4319221935886,-33.7219239407594,
113.844436005007));
#38131=CARTESIAN_POINT('Ctrl Pts',(-86.6834909771368,-34.0786964876457,
113.791786497276));
#38132=CARTESIAN_POINT('Ctrl Pts',(-85.9350597606851,-34.4354690345319,
113.739136989545));
#38133=CARTESIAN_POINT('Ctrl Pts',(-85.3797821397292,-35.1974358198782,
113.686487481814));
#38134=CARTESIAN_POINT('Ctrl Pts',(-85.2693847797268,-36.0191707886337,
113.633837974084));
#38135=CARTESIAN_POINT('Ctrl Pts',(-85.1589874197243,-36.8409057573892,
113.581188466353));
#38136=CARTESIAN_POINT('Ctrl Pts',(-85.4934703206754,-37.7224089095541,
113.528538958622));
#38137=CARTESIAN_POINT('Ctrl Pts',(-86.1212007458526,-38.2640641959476,
113.475889450891));
#38138=CARTESIAN_POINT('Ctrl Pts',(-86.7489311710298,-38.8057194823412,
113.42323994316));
#38139=CARTESIAN_POINT('Ctrl Pts',(-87.6699091204331,-39.0075269029633,
113.37059043543));
#38140=CARTESIAN_POINT('Ctrl Pts',(-88.4666232458397,-38.7780001325227,
113.317940927699));
#38141=CARTESIAN_POINT('Ctrl Pts',(-89.2633373712462,-38.548473362082,113.265291419968));
#38142=CARTESIAN_POINT('Ctrl Pts',(-89.9357876726559,-37.8876124005786,
113.212641912237));
#38143=CARTESIAN_POINT('Ctrl Pts',(-90.1791290317504,-37.0950085153211,
113.159992404506));
#38144=CARTESIAN_POINT('Ctrl Pts',(-90.2521692545041,-36.8571041798227,
113.144189370502));
#38145=CARTESIAN_POINT('Ctrl Pts',(-90.2865496522039,-36.6073306943669,
113.128386336497));
#38146=CARTESIAN_POINT('Ctrl Pts',(-90.2845475626897,-36.3570196913561,
113.112583302492));
#38147=CARTESIAN_POINT('Ctrl Pts',(-90.2821608570194,-36.3545547485103,
113.387416697508));
#38148=CARTESIAN_POINT('Ctrl Pts',(-90.2815738634642,-36.7957480556462,
113.415204380874));
#38149=CARTESIAN_POINT('Ctrl Pts',(-90.1709794942958,-37.2372165766009,
113.442992064241));
#38150=CARTESIAN_POINT('Ctrl Pts',(-89.9521103385491,-37.6161456619663,
113.470779747607));
#38151=CARTESIAN_POINT('Ctrl Pts',(-89.5374174994356,-38.3341051099151,
113.523429255338));
#38152=CARTESIAN_POINT('Ctrl Pts',(-88.7340275758579,-38.8275534131576,
113.576078763068));
#38153=CARTESIAN_POINT('Ctrl Pts',(-87.9061451726702,-38.8727932871949,
113.628728270799));
#38154=CARTESIAN_POINT('Ctrl Pts',(-87.0782627694825,-38.9180331612322,
113.68137777853));
#38155=CARTESIAN_POINT('Ctrl Pts',(-86.2258878866846,-38.5150646060642,
113.734027286261));
#38156=CARTESIAN_POINT('Ctrl Pts',(-85.7354317154879,-37.8465672883091,
113.786676793992));
#38157=CARTESIAN_POINT('Ctrl Pts',(-85.2449755442911,-37.1780699705539,
113.839326301722));
#38158=CARTESIAN_POINT('Ctrl Pts',(-85.1164380846954,-36.2440438902116,
113.891975809453));
#38159=CARTESIAN_POINT('Ctrl Pts',(-85.4080898393636,-35.4679155672457,
113.944625317184));
#38160=CARTESIAN_POINT('Ctrl Pts',(-85.6997415940317,-34.6917872442799,
113.997274824915));
#38161=CARTESIAN_POINT('Ctrl Pts',(-86.4115825629637,-34.0735566786905,
114.049924332646));
#38162=CARTESIAN_POINT('Ctrl Pts',(-87.2209104677263,-33.8934892960711,
114.102573840377));
#38163=CARTESIAN_POINT('Ctrl Pts',(-88.0302383724889,-33.7134219134518,
114.155223348107));
#38164=CARTESIAN_POINT('Ctrl Pts',(-88.9370532130822,-33.9715177138025,
114.207872855838));
#38165=CARTESIAN_POINT('Ctrl Pts',(-89.5302642712866,-34.5507728908488,
114.260522363569));
#38166=CARTESIAN_POINT('Ctrl Pts',(-90.0068443658301,-35.0161409638533,
114.302820474882));
#38167=CARTESIAN_POINT('Ctrl Pts',(-90.2810132257934,-35.6887969255397,
114.345118586195));
#38168=CARTESIAN_POINT('Ctrl Pts',(-90.2870432922795,-36.3570794361236,
114.387416697508));
#38169=CARTESIAN_POINT('Origin',(-87.7685555885722,-36.3549260746835,114.));
#38170=CARTESIAN_POINT('',(-90.2884953401163,-36.3531793386956,115.387416697508));
#38171=CARTESIAN_POINT('',(-90.2833266058024,-36.3532747667377,115.112583302492));
#38172=CARTESIAN_POINT('',(-90.2860555885722,-36.3549260746835,114.));
#38173=CARTESIAN_POINT('Ctrl Pts',(-90.2833266058024,-36.3532747667377,
115.112583302492));
#38174=CARTESIAN_POINT('Ctrl Pts',(-90.2851691707048,-36.0508538051131,
115.0935137626));
#38175=CARTESIAN_POINT('Ctrl Pts',(-90.2346570131273,-35.749027590448,115.074444222708));
#38176=CARTESIAN_POINT('Ctrl Pts',(-90.1290213656974,-35.4679155567543,
115.055374682816));
#38177=CARTESIAN_POINT('Ctrl Pts',(-89.8373696075796,-34.6917872246094,
115.002725175085));
#38178=CARTESIAN_POINT('Ctrl Pts',(-89.1255286302286,-34.0735566517086,
114.950075667354));
#38179=CARTESIAN_POINT('Ctrl Pts',(-88.3162007158942,-33.89348926696,114.897426159623));
#38180=CARTESIAN_POINT('Ctrl Pts',(-87.5068728015597,-33.7134218822113,
114.844776651893));
#38181=CARTESIAN_POINT('Ctrl Pts',(-86.6000579502418,-33.9715176856148,
114.792127144162));
#38182=CARTESIAN_POINT('Ctrl Pts',(-86.0068468850218,-34.550772869512,114.739477636431));
#38183=CARTESIAN_POINT('Ctrl Pts',(-85.4136358198019,-35.1300280534093,
114.6868281287));
#38184=CARTESIAN_POINT('Ctrl Pts',(-85.13402854068,-36.0304426178002,114.634178620969));
#38185=CARTESIAN_POINT('Ctrl Pts',(-85.2947807557105,-36.8438273123537,
114.581529113239));
#38186=CARTESIAN_POINT('Ctrl Pts',(-85.4555329707409,-37.6572120069073,
114.528879605508));
#38187=CARTESIAN_POINT('Ctrl Pts',(-86.0566446799239,-38.3835668316234,
114.476230097777));
#38188=CARTESIAN_POINT('Ctrl Pts',(-86.8256110308943,-38.6936098722588,
114.423580590046));
#38189=CARTESIAN_POINT('Ctrl Pts',(-87.5945773818647,-39.0036529128942,
114.370931082315));
#38190=CARTESIAN_POINT('Ctrl Pts',(-88.5313983746226,-38.8973841694489,
114.318281574584));
#38191=CARTESIAN_POINT('Ctrl Pts',(-89.2113804581624,-38.4229789607549,
114.265632066854));
#38192=CARTESIAN_POINT('Ctrl Pts',(-89.8702686552171,-37.9632903892523,
114.214615812066));
#38193=CARTESIAN_POINT('Ctrl Pts',(-90.288005704732,-37.1579511867132,114.163599557279));
#38194=CARTESIAN_POINT('Ctrl Pts',(-90.290070014705,-36.3544600797813,114.112583302492));
#38195=CARTESIAN_POINT('Ctrl Pts',(-90.2870432922795,-36.3570794361236,
114.387416697508));
#38196=CARTESIAN_POINT('Ctrl Pts',(-90.2885189990354,-36.5206247333347,
114.397768093926));
#38197=CARTESIAN_POINT('Ctrl Pts',(-90.2739358136687,-36.6839081035843,
114.408119490344));
#38198=CARTESIAN_POINT('Ctrl Pts',(-90.2423303921774,-36.8438273065707,
114.418470886762));
#38199=CARTESIAN_POINT('Ctrl Pts',(-90.0815781790484,-37.6572119915045,
114.471120394492));
#38200=CARTESIAN_POINT('Ctrl Pts',(-89.4804664769749,-38.3835668076304,
114.523769902223));
#38201=CARTESIAN_POINT('Ctrl Pts',(-88.711500135099,-38.6936098445993,114.576419409954));
#38202=CARTESIAN_POINT('Ctrl Pts',(-87.9425337932232,-39.0036528815682,
114.629068917685));
#38203=CARTESIAN_POINT('Ctrl Pts',(-87.0057128115448,-38.89738413938,114.681718425416));
#38204=CARTESIAN_POINT('Ctrl Pts',(-86.3257307360469,-38.4229789362969,
114.734367933146));
#38205=CARTESIAN_POINT('Ctrl Pts',(-85.6457486605489,-37.9485737332138,
114.787017440877));
#38206=CARTESIAN_POINT('Ctrl Pts',(-85.2226054912313,-37.1060320692359,
114.839666948608));
#38207=CARTESIAN_POINT('Ctrl Pts',(-85.2481267492453,-36.2773073953543,
114.892316456339));
#38208=CARTESIAN_POINT('Ctrl Pts',(-85.2736480072592,-35.4485827214727,
114.94496596407));
#38209=CARTESIAN_POINT('Ctrl Pts',(-85.7478336926047,-34.6336750376873,
114.997615471801));
#38210=CARTESIAN_POINT('Ctrl Pts',(-86.4557189356833,-34.202010350294,115.050264979531));
#38211=CARTESIAN_POINT('Ctrl Pts',(-87.1636041787619,-33.7703456629007,
115.102914487262));
#38212=CARTESIAN_POINT('Ctrl Pts',(-88.1051889795735,-33.7219239718993,
115.155563994993));
#38213=CARTESIAN_POINT('Ctrl Pts',(-88.8536201871739,-34.0786965145658,
115.208213502724));
#38214=CARTESIAN_POINT('Ctrl Pts',(-89.6020513947743,-34.4354690572323,
115.260863010455));
#38215=CARTESIAN_POINT('Ctrl Pts',(-90.1573290091633,-35.1974358335667,
115.313512518185));
#38216=CARTESIAN_POINT('Ctrl Pts',(-90.2677263678604,-36.0191707926036,
115.366162025916));
#38217=CARTESIAN_POINT('Ctrl Pts',(-90.2825822180847,-36.1297492667593,
115.373246916447));
#38218=CARTESIAN_POINT('Ctrl Pts',(-90.2893820435841,-36.2414100410428,
115.380331806977));
#38219=CARTESIAN_POINT('Ctrl Pts',(-90.2884953401163,-36.3531793386956,
115.387416697508));
#38220=CARTESIAN_POINT('Origin',(-87.7685555885722,-36.3549260746835,114.));
#38221=CARTESIAN_POINT('',(-90.2821875961807,-36.3544693504637,116.387416697508));
#38222=CARTESIAN_POINT('',(-90.2844060344053,-36.3569864153294,116.112583302492));
#38223=CARTESIAN_POINT('',(-90.2860555885722,-36.3549260746835,114.));
#38224=CARTESIAN_POINT('Ctrl Pts',(-90.2844060344053,-36.3569864153294,
116.112583302492));
#38225=CARTESIAN_POINT('Ctrl Pts',(-90.2798734754633,-35.7786726434231,
116.076077475652));
#38226=CARTESIAN_POINT('Ctrl Pts',(-90.0814676279119,-35.197549043947,116.039571648811));
#38227=CARTESIAN_POINT('Ctrl Pts',(-89.7163642240759,-34.7534805203941,
116.003065821971));
#38228=CARTESIAN_POINT('Ctrl Pts',(-89.1898040514538,-34.1130351124323,
115.95041631424));
#38229=CARTESIAN_POINT('Ctrl Pts',(-88.3165122304853,-33.7576648636286,
115.897766806509));
#38230=CARTESIAN_POINT('Ctrl Pts',(-87.4923823282214,-33.8484714722295,
115.845117298778));
#38231=CARTESIAN_POINT('Ctrl Pts',(-86.6682524259574,-33.9392780808303,
115.792467791047));
#38232=CARTESIAN_POINT('Ctrl Pts',(-85.893284442398,-34.4762615468358,115.739818283317));
#38233=CARTESIAN_POINT('Ctrl Pts',(-85.5187983280969,-35.2159885817391,
115.687168775586));
#38234=CARTESIAN_POINT('Ctrl Pts',(-85.1443122137959,-35.9557156166424,
115.634519267855));
#38235=CARTESIAN_POINT('Ctrl Pts',(-85.1703079687531,-36.8981862204437,
115.581869760124));
#38236=CARTESIAN_POINT('Ctrl Pts',(-85.5850008127714,-37.6161456768834,
115.529220252393));
#38237=CARTESIAN_POINT('Ctrl Pts',(-85.9996936567897,-38.3341051333231,
115.476570744662));
#38238=CARTESIAN_POINT('Ctrl Pts',(-86.8030835898689,-38.8275534424013,
115.423921236932));
#38239=CARTESIAN_POINT('Ctrl Pts',(-87.6309660028479,-38.8727933169733,
115.371271729201));
#38240=CARTESIAN_POINT('Ctrl Pts',(-88.4588484158269,-38.9180331915453,
115.31862222147));
#38241=CARTESIAN_POINT('Ctrl Pts',(-89.3112233087056,-38.5150646316112,
115.265972713739));
#38242=CARTESIAN_POINT('Ctrl Pts',(-89.8016794857027,-37.8465673059497,
115.213323206008));
#38243=CARTESIAN_POINT('Ctrl Pts',(-90.1144934769387,-37.420198292002,115.17974323817));
#38244=CARTESIAN_POINT('Ctrl Pts',(-90.2800819931629,-36.8858144201648,
115.146163270331));
#38245=CARTESIAN_POINT('Ctrl Pts',(-90.2833266058024,-36.3532747667377,
115.112583302492));
#38246=CARTESIAN_POINT('Ctrl Pts',(-90.2884953401163,-36.3531793386956,
115.387416697508));
#38247=CARTESIAN_POINT('Ctrl Pts',(-90.2827927390801,-37.0719942929028,
115.432981314708));
#38248=CARTESIAN_POINT('Ctrl Pts',(-89.9591689800778,-37.7952978628962,
115.478545931909));
#38249=CARTESIAN_POINT('Ctrl Pts',(-89.4159104118097,-38.264064173368,115.524110549109));
#38250=CARTESIAN_POINT('Ctrl Pts',(-88.7881799940568,-38.8057194533557,
115.57676005684));
#38251=CARTESIAN_POINT('Ctrl Pts',(-87.8672020555458,-39.0075268715915,
115.62940956457));
#38252=CARTESIAN_POINT('Ctrl Pts',(-87.0704879395618,-38.7780001038657,
115.682059072301));
#38253=CARTESIAN_POINT('Ctrl Pts',(-86.2737738235778,-38.5484733361399,
115.734708580032));
#38254=CARTESIAN_POINT('Ctrl Pts',(-85.6013235301207,-37.8876123824526,
115.787358087763));
#38255=CARTESIAN_POINT('Ctrl Pts',(-85.3579821739038,-37.0950085065692,
115.840007595494));
#38256=CARTESIAN_POINT('Ctrl Pts',(-85.1146408176869,-36.3024046306858,
115.892657103225));
#38257=CARTESIAN_POINT('Ctrl Pts',(-85.3004083987102,-35.3780578326064,
115.945306610955));
#38258=CARTESIAN_POINT('Ctrl Pts',(-85.8310700090495,-34.7410066768717,
115.997956118686));
#38259=CARTESIAN_POINT('Ctrl Pts',(-86.3617316193887,-34.103955521137,116.050605626417));
#38260=CARTESIAN_POINT('Ctrl Pts',(-87.237287259044,-33.754200007747,116.103255134148));
#38261=CARTESIAN_POINT('Ctrl Pts',(-88.0608170931881,-33.8502964800305,
116.155904641879));
#38262=CARTESIAN_POINT('Ctrl Pts',(-88.8843469273323,-33.946392952314,116.208554149609));
#38263=CARTESIAN_POINT('Ctrl Pts',(-89.6558509559653,-34.4883414102711,
116.26120365734));
#38264=CARTESIAN_POINT('Ctrl Pts',(-90.0255795598235,-35.2304577617955,
116.313853165071));
#38265=CARTESIAN_POINT('Ctrl Pts',(-90.1977783344182,-35.5760937905085,
116.33837434255));
#38266=CARTESIAN_POINT('Ctrl Pts',(-90.2828251044975,-35.9651496803884,
116.362895520029));
#38267=CARTESIAN_POINT('Ctrl Pts',(-90.2821875961807,-36.3544693504637,
116.387416697508));
#38268=CARTESIAN_POINT('Origin',(-87.7685555885722,-36.3549260746835,114.));
#38269=CARTESIAN_POINT('',(-90.2868834016879,-36.3571029250538,117.387416697508));
#38270=CARTESIAN_POINT('',(-90.2901100729428,-36.3545560533475,117.112583302492));
#38271=CARTESIAN_POINT('',(-90.2860555885722,-36.3549260746835,114.));
#38272=CARTESIAN_POINT('Ctrl Pts',(-90.2901100729428,-36.3545560533475,
117.112583302492));
#38273=CARTESIAN_POINT('Ctrl Pts',(-90.2901522460903,-36.3341987546248,
117.111290696434));
#38274=CARTESIAN_POINT('Ctrl Pts',(-90.2899268097382,-36.3138424136066,
117.109998090376));
#38275=CARTESIAN_POINT('Ctrl Pts',(-90.2894308889351,-36.29349266426,117.108705484318));
#38276=CARTESIAN_POINT('Ctrl Pts',(-90.2692313966009,-35.4646211926309,
117.056055976587));
#38277=CARTESIAN_POINT('Ctrl Pts',(-89.8002880018944,-34.6466855528239,
117.003406468856));
#38278=CARTESIAN_POINT('Ctrl Pts',(-89.0951890616713,-34.2104844289517,
116.950756961126));
#38279=CARTESIAN_POINT('Ctrl Pts',(-88.3900901214482,-33.7742833050794,
116.898107453395));
#38280=CARTESIAN_POINT('Ctrl Pts',(-87.4488356357085,-33.7198166971419,
116.845457945664));
#38281=CARTESIAN_POINT('Ctrl Pts',(-86.6981290120818,-34.071776213584,116.792808437933));
#38282=CARTESIAN_POINT('Ctrl Pts',(-85.947422388455,-34.4237357300261,116.740158930202));
#38283=CARTESIAN_POINT('Ctrl Pts',(-85.3872636269413,-35.1821213708479,
116.687509422471));
#38284=CARTESIAN_POINT('Ctrl Pts',(-85.2715921838434,-36.0031305384112,
116.634859914741));
#38285=CARTESIAN_POINT('Ctrl Pts',(-85.1559207407456,-36.8241397059744,
116.58221040701));
#38286=CARTESIAN_POINT('Ctrl Pts',(-85.4847366160637,-37.707772400279,116.529560899279));
#38287=CARTESIAN_POINT('Ctrl Pts',(-86.1089761329637,-38.2534471765989,
116.476911391548));
#38288=CARTESIAN_POINT('Ctrl Pts',(-86.7332156498636,-38.7991219529187,
116.424261883817));
#38289=CARTESIAN_POINT('Ctrl Pts',(-87.6528788083454,-39.0068388112537,
116.371612376086));
#38290=CARTESIAN_POINT('Ctrl Pts',(-88.4510503006566,-38.7824324725891,
116.318962868356));
#38291=CARTESIAN_POINT('Ctrl Pts',(-89.2492217929678,-38.5580261339245,
116.266313360625));
#38292=CARTESIAN_POINT('Ctrl Pts',(-89.9259016191085,-37.9014965982603,
116.213663852894));
#38293=CARTESIAN_POINT('Ctrl Pts',(-90.174327270041,-37.1104715468681,116.161014345163));
#38294=CARTESIAN_POINT('Ctrl Pts',(-90.2505009059684,-36.8679231061256,
116.144870664273));
#38295=CARTESIAN_POINT('Ctrl Pts',(-90.2864104318265,-36.6127295061235,
116.128726983382));
#38296=CARTESIAN_POINT('Ctrl Pts',(-90.2844060344053,-36.3569864153294,
116.112583302492));
#38297=CARTESIAN_POINT('Ctrl Pts',(-90.2821875961807,-36.3544693504637,
116.387416697508));
#38298=CARTESIAN_POINT('Ctrl Pts',(-90.281456308114,-36.8010593342772,116.41554502776));
#38299=CARTESIAN_POINT('Ctrl Pts',(-90.1679776534187,-37.2479964123646,
116.443673358012));
#38300=CARTESIAN_POINT('Ctrl Pts',(-89.9439670360065,-37.6301402636982,
116.471801688264));
#38301=CARTESIAN_POINT('Ctrl Pts',(-89.5246727292477,-38.3454221689849,
116.524451195994));
#38302=CARTESIAN_POINT('Ctrl Pts',(-88.7181309366466,-38.8337017344665,
116.577100703725));
#38303=CARTESIAN_POINT('Ctrl Pts',(-87.8899751149491,-38.8736248443078,
116.629750211456));
#38304=CARTESIAN_POINT('Ctrl Pts',(-87.0618192932517,-38.913547954149,116.682399719187));
#38305=CARTESIAN_POINT('Ctrl Pts',(-86.2120494424578,-38.5051146083499,
116.735049226918));
#38306=CARTESIAN_POINT('Ctrl Pts',(-85.7258958021339,-37.8334818532593,
116.787698734649));
#38307=CARTESIAN_POINT('Ctrl Pts',(-85.2397421618101,-37.1618490981687,
116.840348242379));
#38308=CARTESIAN_POINT('Ctrl Pts',(-85.1172047319563,-36.2270169337866,
116.89299775011));
#38309=CARTESIAN_POINT('Ctrl Pts',(-85.4138339929931,-35.4527773060176,
116.945647257841));
#38310=CARTESIAN_POINT('Ctrl Pts',(-85.71046325403,-34.6785376782487,116.998296765572));
#38311=CARTESIAN_POINT('Ctrl Pts',(-86.4262592059575,-34.0648905870928,
117.050946273303));
#38312=CARTESIAN_POINT('Ctrl Pts',(-87.236726638944,-33.8900236097103,117.103595781033));
#38313=CARTESIAN_POINT('Ctrl Pts',(-88.0471940719305,-33.7151566323279,
117.156245288764));
#38314=CARTESIAN_POINT('Ctrl Pts',(-88.952332985976,-33.9790697687189,117.208894796495));
#38315=CARTESIAN_POINT('Ctrl Pts',(-89.5418124186763,-34.5621220117756,
117.261544304226));
#38316=CARTESIAN_POINT('Ctrl Pts',(-90.0115805778514,-35.026768212694,117.303501768653));
#38317=CARTESIAN_POINT('Ctrl Pts',(-90.2808790654697,-35.6940939327625,
117.345459233081));
#38318=CARTESIAN_POINT('Ctrl Pts',(-90.2868834016879,-36.3571029250538,
117.387416697508));
#38319=CARTESIAN_POINT('Origin',(-87.7685555885722,-36.3549260746835,114.));
#38320=CARTESIAN_POINT('',(-90.2886326699929,-36.3532397190198,118.387416697508));
#38321=CARTESIAN_POINT('',(-90.2834380340513,-36.3532166686934,118.112583302492));
#38322=CARTESIAN_POINT('',(-90.2860555885722,-36.3549260746835,114.));
#38323=CARTESIAN_POINT('Ctrl Pts',(-90.2834380340513,-36.3532166686934,
118.112583302492));
#38324=CARTESIAN_POINT('Ctrl Pts',(-90.2853167452331,-36.0562310899231,
118.093854409486));
#38325=CARTESIAN_POINT('Ctrl Pts',(-90.236641918583,-35.7598412835663,118.075125516479));
#38326=CARTESIAN_POINT('Ctrl Pts',(-90.1346681982238,-35.4830903892948,
118.056396623473));
#38327=CARTESIAN_POINT('Ctrl Pts',(-89.8480059712278,-34.7051053614309,
118.003747115742));
#38328=CARTESIAN_POINT('Ctrl Pts',(-89.1401493258784,-34.0823168034606,
117.951097608011));
#38329=CARTESIAN_POINT('Ctrl Pts',(-88.3319943080865,-33.8970564375262,
117.89844810028));
#38330=CARTESIAN_POINT('Ctrl Pts',(-87.5238392902945,-33.7117960715917,
117.845798592549));
#38331=CARTESIAN_POINT('Ctrl Pts',(-86.6153859000598,-33.9640638976931,
117.793149084819));
#38332=CARTESIAN_POINT('Ctrl Pts',(-86.0184676671723,-34.5394981330494,
117.740499577088));
#38333=CARTESIAN_POINT('Ctrl Pts',(-85.4215494342849,-35.1149323684057,
117.687850069357));
#38334=CARTESIAN_POINT('Ctrl Pts',(-85.1361663587445,-36.013533013017,117.635200561626));
#38335=CARTESIAN_POINT('Ctrl Pts',(-85.291692518077,-36.8279331295038,117.582551053895));
#38336=CARTESIAN_POINT('Ctrl Pts',(-85.4472186774094,-37.6423332459907,
117.529901546165));
#38337=CARTESIAN_POINT('Ctrl Pts',(-86.0436540716147,-38.3725328343531,
117.477252038434));
#38338=CARTESIAN_POINT('Ctrl Pts',(-86.8106137846128,-38.6875070152136,
117.424602530703));
#38339=CARTESIAN_POINT('Ctrl Pts',(-87.577573497611,-39.0024811960742,117.371953022972));
#38340=CARTESIAN_POINT('Ctrl Pts',(-88.515057529402,-38.9022299694327,117.319303515241));
#38341=CARTESIAN_POINT('Ctrl Pts',(-89.1980717503166,-38.4322007043864,
117.26665400751));
#38342=CARTESIAN_POINT('Ctrl Pts',(-89.8643171853922,-37.9737111991903,
117.215297105838));
#38343=CARTESIAN_POINT('Ctrl Pts',(-90.2884344795338,-37.1633777220556,
117.163940204165));
#38344=CARTESIAN_POINT('Ctrl Pts',(-90.2901100729428,-36.3545560533475,
117.112583302492));
#38345=CARTESIAN_POINT('Ctrl Pts',(-90.2868834016879,-36.3571029250538,
117.387416697508));
#38346=CARTESIAN_POINT('Ctrl Pts',(-90.2884134899268,-36.5260578643693,
117.398108740811));
#38347=CARTESIAN_POINT('Ctrl Pts',(-90.2728456235452,-36.6947324814093,
117.408800784115));
#38348=CARTESIAN_POINT('Ctrl Pts',(-90.2391401617222,-36.8597013320064,
117.419492827418));
#38349=CARTESIAN_POINT('Ctrl Pts',(-90.073168520713,-37.6720370594578,117.472142335149));
#38350=CARTESIAN_POINT('Ctrl Pts',(-89.4674052873395,-38.394517164638,117.52479184288));
#38351=CARTESIAN_POINT('Ctrl Pts',(-88.6964640117255,-38.6996162784728,
117.577441350611));
#38352=CARTESIAN_POINT('Ctrl Pts',(-87.9255227361115,-39.0047153923077,
117.630090858342));
#38353=CARTESIAN_POINT('Ctrl Pts',(-86.989403418257,-38.8924335147973,117.682740366073));
#38354=CARTESIAN_POINT('Ctrl Pts',(-86.3124815155165,-38.4136719276825,
117.735389873803));
#38355=CARTESIAN_POINT('Ctrl Pts',(-85.6355596127759,-37.9349103405677,
117.788039381534));
#38356=CARTESIAN_POINT('Ctrl Pts',(-85.2178351251494,-37.0896690438486,
117.840688889265));
#38357=CARTESIAN_POINT('Ctrl Pts',(-85.2486770968523,-36.2611253259234,
117.893338396996));
#38358=CARTESIAN_POINT('Ctrl Pts',(-85.2795190685552,-35.4325816079982,
117.945987904727));
#38359=CARTESIAN_POINT('Ctrl Pts',(-85.7589274995874,-34.620735468867,117.998637412457));
#38360=CARTESIAN_POINT('Ctrl Pts',(-86.4695698679984,-34.1936250102018,
118.051286920188));
#38361=CARTESIAN_POINT('Ctrl Pts',(-87.1802122364094,-33.7665145515366,
118.103936427919));
#38362=CARTESIAN_POINT('Ctrl Pts',(-88.1220885421992,-33.7241397733375,
118.15658593565));
#38363=CARTESIAN_POINT('Ctrl Pts',(-88.868213485108,-34.0857106367326,118.209235443381));
#38364=CARTESIAN_POINT('Ctrl Pts',(-89.6143384280168,-34.4472815001277,
118.261884951112));
#38365=CARTESIAN_POINT('Ctrl Pts',(-90.1647120080446,-35.212798005117,118.314534458842));
#38366=CARTESIAN_POINT('Ctrl Pts',(-90.2698307320447,-36.0352248856062,
118.367183966573));
#38367=CARTESIAN_POINT('Ctrl Pts',(-90.2832961245404,-36.140575296298,118.373928210218));
#38368=CARTESIAN_POINT('Ctrl Pts',(-90.2894554014685,-36.2468595402199,
118.380672453863));
#38369=CARTESIAN_POINT('Ctrl Pts',(-90.2886326699929,-36.3532397190198,
118.387416697508));
#38370=CARTESIAN_POINT('Origin',(-87.7685555885722,-36.3549260746835,114.));
#38371=CARTESIAN_POINT('',(-90.2822198465711,-36.3543846296117,119.387416697508));
#38372=CARTESIAN_POINT('',(-90.2842673953521,-36.3569499564742,119.112583302492));
#38373=CARTESIAN_POINT('',(-90.2860555885722,-36.3549260746835,114.));
#38374=CARTESIAN_POINT('Ctrl Pts',(-90.2842673953521,-36.3569499564742,
119.112583302492));
#38375=CARTESIAN_POINT('Ctrl Pts',(-90.2798741810248,-35.7839526994676,
119.076418122537));
#38376=CARTESIAN_POINT('Ctrl Pts',(-90.0854712507547,-35.2082585800464,
119.040252942582));
#38377=CARTESIAN_POINT('Ctrl Pts',(-89.7266069493757,-34.7660204103463,
119.004087762628));
#38378=CARTESIAN_POINT('Ctrl Pts',(-89.2041699303043,-34.1222071633618,
118.951438254897));
#38379=CARTESIAN_POINT('Ctrl Pts',(-88.3331779445183,-33.7612368344392,
118.898788747166));
#38380=CARTESIAN_POINT('Ctrl Pts',(-87.5084819626193,-33.8467498341343,
118.846139239435));
#38381=CARTESIAN_POINT('Ctrl Pts',(-86.6837859807203,-33.9322628338293,
118.793489731704));
#38382=CARTESIAN_POINT('Ctrl Pts',(-85.9053860027083,-34.4642591621421,
118.740840223973));
#38383=CARTESIAN_POINT('Ctrl Pts',(-85.526157822188,-35.2015663730428,118.688190716243));
#38384=CARTESIAN_POINT('Ctrl Pts',(-85.1469296416677,-35.9388735839435,
118.635541208512));
#38385=CARTESIAN_POINT('Ctrl Pts',(-85.1668732586391,-36.8814916774321,
118.582891700781));
#38386=CARTESIAN_POINT('Ctrl Pts',(-85.576947537357,-37.6020990753135,118.53024219305));
#38387=CARTESIAN_POINT('Ctrl Pts',(-85.9870218160749,-38.3227064731948,
118.477592685319));
#38388=CARTESIAN_POINT('Ctrl Pts',(-86.7872267565391,-38.8213031754689,
118.424943177589));
#38389=CARTESIAN_POINT('Ctrl Pts',(-87.6148016176882,-38.8718579490944,
118.372293669858));
#38390=CARTESIAN_POINT('Ctrl Pts',(-88.4423764788374,-38.92241272272,118.319644162127));
#38391=CARTESIAN_POINT('Ctrl Pts',(-89.2973212606714,-38.5249255676971,
118.266994654396));
#38392=CARTESIAN_POINT('Ctrl Pts',(-89.792059747267,-37.8595912413068,118.214345146665));
#38393=CARTESIAN_POINT('Ctrl Pts',(-90.1108060056166,-37.4309348241605,
118.180424531941));
#38394=CARTESIAN_POINT('Ctrl Pts',(-90.2800354283472,-36.8910986135966,
118.146503917216));
#38395=CARTESIAN_POINT('Ctrl Pts',(-90.2834380340513,-36.3532166686934,
118.112583302492));
#38396=CARTESIAN_POINT('Ctrl Pts',(-90.2886326699929,-36.3532397190198,
118.387416697508));
#38397=CARTESIAN_POINT('Ctrl Pts',(-90.2830326787043,-37.0773253924338,
118.433321961594));
#38398=CARTESIAN_POINT('Ctrl Pts',(-89.953959085277,-37.8058556896245,118.47922722568));
#38399=CARTESIAN_POINT('Ctrl Pts',(-89.4036178791718,-38.2746024797132,
118.525132489766));
#38400=CARTESIAN_POINT('Ctrl Pts',(-88.7724224343267,-38.812215937342,118.577781997496));
#38401=CARTESIAN_POINT('Ctrl Pts',(-87.8501676766643,-39.0081055966104,
118.630431505227));
#38402=CARTESIAN_POINT('Ctrl Pts',(-87.0549437757234,-38.7734678609392,
118.683081012958));
#38403=CARTESIAN_POINT('Ctrl Pts',(-86.2597198747824,-38.538830125268,118.735730520689));
#38404=CARTESIAN_POINT('Ctrl Pts',(-85.5915268305631,-37.8736649946574,
118.78838002842));
#38405=CARTESIAN_POINT('Ctrl Pts',(-85.3532797991764,-37.0795149627522,
118.841029536151));
#38406=CARTESIAN_POINT('Ctrl Pts',(-85.1150327677896,-36.285364930847,118.893679043881));
#38407=CARTESIAN_POINT('Ctrl Pts',(-85.3067317492356,-35.3622299976473,
118.946328551612));
#38408=CARTESIAN_POINT('Ctrl Pts',(-85.8414729241709,-34.7285993539164,
118.998978059343));
#38409=CARTESIAN_POINT('Ctrl Pts',(-86.3762140991062,-34.0949687101855,
119.051627567074));
#38410=CARTESIAN_POINT('Ctrl Pts',(-87.253997467531,-33.7508423559234,119.104277074805));
#38411=CARTESIAN_POINT('Ctrl Pts',(-88.0768932901973,-33.8522247269142,
119.156926582536));
#38412=CARTESIAN_POINT('Ctrl Pts',(-88.8997891128635,-33.9536070979049,
119.209576090266));
#38413=CARTESIAN_POINT('Ctrl Pts',(-89.6677973897713,-34.5004981941486,
119.262225597997));
#38414=CARTESIAN_POINT('Ctrl Pts',(-90.0327532423181,-35.2449732821291,
119.314875105728));
#38415=CARTESIAN_POINT('Ctrl Pts',(-90.2003678419235,-35.5868910590801,
119.339055636321));
#38416=CARTESIAN_POINT('Ctrl Pts',(-90.28296567943,-35.9704856755803,119.363236166915));
#38417=CARTESIAN_POINT('Ctrl Pts',(-90.2822198465711,-36.3543846296117,
119.387416697508));
#38418=CARTESIAN_POINT('Origin',(-87.7685555885722,-36.3549260746835,114.));
#38419=CARTESIAN_POINT('',(-90.2867226440827,-36.3571243050301,120.387416697508));
#38420=CARTESIAN_POINT('',(-90.290141386937,-36.3546528235808,120.112583302492));
#38421=CARTESIAN_POINT('',(-90.2860555885722,-36.3549260746835,114.));
#38422=CARTESIAN_POINT('Ctrl Pts',(-90.290141386937,-36.3546528235808,120.112583302492));
#38423=CARTESIAN_POINT('Ctrl Pts',(-90.290164686063,-36.3396608841848,120.11163134332));
#38424=CARTESIAN_POINT('Ctrl Pts',(-90.2900424224598,-36.3246693349243,
120.110679384147));
#38425=CARTESIAN_POINT('Ctrl Pts',(-90.2897734333149,-36.3096804188387,
120.109727424975));
#38426=CARTESIAN_POINT('Ctrl Pts',(-90.2748965914554,-35.4806962814753,
120.057077917244));
#38427=CARTESIAN_POINT('Ctrl Pts',(-89.8112147295564,-34.65976651665,120.004428409513));
#38428=CARTESIAN_POINT('Ctrl Pts',(-89.1089311464144,-34.2190469710397,
119.951778901782));
#38429=CARTESIAN_POINT('Ctrl Pts',(-88.4066475632724,-33.7783274254294,
119.899129394052));
#38430=CARTESIAN_POINT('Ctrl Pts',(-87.4657622588873,-33.7178180990341,
119.846479886321));
#38431=CARTESIAN_POINT('Ctrl Pts',(-86.7128111916705,-34.0649500616042,
119.79383037859));
#38432=CARTESIAN_POINT('Ctrl Pts',(-85.9598601244536,-34.4120820241742,
119.741180870859));
#38433=CARTESIAN_POINT('Ctrl Pts',(-85.394843294405,-35.1668552757097,119.688531363128));
#38434=CARTESIAN_POINT('Ctrl Pts',(-85.2739025313641,-35.9871047981258,
119.635881855397));
#38435=CARTESIAN_POINT('Ctrl Pts',(-85.1529617683233,-36.8073543205419,
119.583232347667));
#38436=CARTESIAN_POINT('Ctrl Pts',(-85.4760970722901,-37.6930801138387,
119.530582839936));
#38437=CARTESIAN_POINT('Ctrl Pts',(-86.0968199466272,-38.2427518792084,
119.477933332205));
#38438=CARTESIAN_POINT('Ctrl Pts',(-86.7175428209643,-38.7924236445782,
119.425283824474));
#38439=CARTESIAN_POINT('Ctrl Pts',(-87.6358532656717,-39.0060413820208,
119.372634316743));
#38440=CARTESIAN_POINT('Ctrl Pts',(-88.4354492151556,-38.7867647287355,
119.319984809013));
#38441=CARTESIAN_POINT('Ctrl Pts',(-89.2350451646396,-38.5674880754502,
119.267335301282));
#38442=CARTESIAN_POINT('Ctrl Pts',(-89.9159266189002,-37.9153170314371,
119.214685793551));
#38443=CARTESIAN_POINT('Ctrl Pts',(-90.169426319852,-37.1259034269073,119.16203628582));
#38444=CARTESIAN_POINT('Ctrl Pts',(-90.248795953904,-36.87874152229,119.145551958044));
#38445=CARTESIAN_POINT('Ctrl Pts',(-90.2862698514454,-36.6181258889888,
119.129067630268));
#38446=CARTESIAN_POINT('Ctrl Pts',(-90.2842673953521,-36.3569499564742,
119.112583302492));
#38447=CARTESIAN_POINT('Ctrl Pts',(-90.2822198465711,-36.3543846296117,
119.387416697508));
#38448=CARTESIAN_POINT('Ctrl Pts',(-90.2813417393464,-36.8063685305952,
119.415885674646));
#38449=CARTESIAN_POINT('Ctrl Pts',(-90.1649363125751,-37.2587742908399,
119.444354651783));
#38450=CARTESIAN_POINT('Ctrl Pts',(-89.9357340391242,-37.6440823046029,
119.472823628921));
#38451=CARTESIAN_POINT('Ctrl Pts',(-89.5118555551979,-38.3566571593789,
119.525473136651));
#38452=CARTESIAN_POINT('Ctrl Pts',(-88.7021951591595,-38.8397477892134,
119.578122644382));
#38453=CARTESIAN_POINT('Ctrl Pts',(-87.8738000571021,-38.8743525238657,
119.630772152113));
#38454=CARTESIAN_POINT('Ctrl Pts',(-87.0454049550448,-38.9089572585181,
119.683421659844));
#38455=CARTESIAN_POINT('Ctrl Pts',(-86.1982751469685,-38.4950760979882,
119.736071167575));
#38456=CARTESIAN_POINT('Ctrl Pts',(-85.7164440946653,-37.8203355247142,
119.788720675305));
#38457=CARTESIAN_POINT('Ctrl Pts',(-85.234613042362,-37.1455949514403,119.841370183036));
#38458=CARTESIAN_POINT('Ctrl Pts',(-85.1180807458316,-36.2099949654222,
119.894019690767));
#38459=CARTESIAN_POINT('Ctrl Pts',(-85.4196752561595,-35.4376761026093,
119.946669198498));
#38460=CARTESIAN_POINT('Ctrl Pts',(-85.7212697664874,-34.6653572397964,
119.999318706229));
#38461=CARTESIAN_POINT('Ctrl Pts',(-86.4409910836734,-34.0563195001886,
120.05196821396));
#38462=CARTESIAN_POINT('Ctrl Pts',(-87.2525646854532,-33.8866598330932,
120.10461772169));
#38463=CARTESIAN_POINT('Ctrl Pts',(-88.064138287233,-33.7170001659977,120.157267229421));
#38464=CARTESIAN_POINT('Ctrl Pts',(-88.9675641736066,-33.9867185714146,
120.209916737152));
#38465=CARTESIAN_POINT('Ctrl Pts',(-89.5532875619044,-34.5735444679974,
120.262566244883));
#38466=CARTESIAN_POINT('Ctrl Pts',(-90.0162727716681,-35.0374011557315,
120.304183062425));
#38467=CARTESIAN_POINT('Ctrl Pts',(-90.28075376653,-35.6993902911316,120.345799879966));
#38468=CARTESIAN_POINT('Ctrl Pts',(-90.2867226440827,-36.3571243050301,
120.387416697508));
#38469=CARTESIAN_POINT('Origin',(-87.7685555885722,-36.3549260746835,114.));
#38470=CARTESIAN_POINT('',(-90.2887582439581,-36.3533471924086,121.387416697508));
#38471=CARTESIAN_POINT('',(-90.2835504011883,-36.3531642868356,121.112583302492));
#38472=CARTESIAN_POINT('',(-90.2860555885722,-36.3549260746835,114.));
#38473=CARTESIAN_POINT('',(-85.855089591907,-34.7189388713088,122.));
#38474=CARTESIAN_POINT('Ctrl Pts',(-90.2887582439581,-36.3533471924086,
121.387416697508));
#38475=CARTESIAN_POINT('Ctrl Pts',(-90.2833001895768,-37.0825700799613,
121.43366260848));
#38476=CARTESIAN_POINT('Ctrl Pts',(-89.9487704521404,-37.8160441629617,
121.479908519451));
#38477=CARTESIAN_POINT('Ctrl Pts',(-89.3912934070429,-38.2848774639003,
121.526154430423));
#38478=CARTESIAN_POINT('Ctrl Pts',(-88.756623413977,-38.8186293564175,121.578803938153));
#38479=CARTESIAN_POINT('Ctrl Pts',(-87.8329891255066,-39.009377613116,121.631453445884));
#38480=CARTESIAN_POINT('Ctrl Pts',(-87.0393721481588,-38.769223717878,121.684102953615));
#38481=CARTESIAN_POINT('Ctrl Pts',(-86.2457551708111,-38.5290698226399,
121.736752461346));
#38482=CARTESIAN_POINT('Ctrl Pts',(-85.5821555045859,-37.8580137754653,
121.789401969077));
#38483=CARTESIAN_POINT('Ctrl Pts',(-85.3491902632795,-37.0637278391879,
121.842051476807));
#38484=CARTESIAN_POINT('Ctrl Pts',(-85.1162250219731,-36.2694419029105,
121.894700984538));
#38485=CARTESIAN_POINT('Ctrl Pts',(-85.3138942055855,-35.3519260775303,
121.947350492269));
#38486=CARTESIAN_POINT('Ctrl Pts',(-85.855089591907,-34.7189388713087,122.));
#38487=CARTESIAN_POINT('',(-89.685665865028,-34.7163981196112,122.));
#38488=CARTESIAN_POINT('Origin',(-87.7685555885722,-36.3549260746835,122.));
#38489=CARTESIAN_POINT('Ctrl Pts',(-89.6856747112032,-34.7163919521555,
122.));
#38490=CARTESIAN_POINT('Ctrl Pts',(-89.1628541599957,-34.1076769201533,
121.949053726697));
#38491=CARTESIAN_POINT('Ctrl Pts',(-88.3231296368472,-33.7675004995563,
121.898107453395));
#38492=CARTESIAN_POINT('Ctrl Pts',(-87.5244587636259,-33.8452632724063,
121.847161180092));
#38493=CARTESIAN_POINT('Ctrl Pts',(-86.6990867474188,-33.9256258081705,
121.794511672361));
#38494=CARTESIAN_POINT('Ctrl Pts',(-85.9175592756957,-34.4523397302599,
121.74186216463));
#38495=CARTESIAN_POINT('Ctrl Pts',(-85.5336746560242,-35.1871265144118,
121.689212656899));
#38496=CARTESIAN_POINT('Ctrl Pts',(-85.1497900363526,-35.9219132985637,
121.636563149169));
#38497=CARTESIAN_POINT('Ctrl Pts',(-85.1635482687327,-36.8647729447781,
121.583913641438));
#38498=CARTESIAN_POINT('Ctrl Pts',(-85.5689530570713,-37.5880327246192,
121.531264133707));
#38499=CARTESIAN_POINT('Ctrl Pts',(-85.9743578454099,-38.3112925044604,
121.478614625976));
#38500=CARTESIAN_POINT('Ctrl Pts',(-86.7714091897071,-38.8149524179282,
121.425965118245));
#38501=CARTESIAN_POINT('Ctrl Pts',(-87.5986589189311,-38.870803405099,121.373315610515));
#38502=CARTESIAN_POINT('Ctrl Pts',(-88.4259086481551,-38.9266543922699,
121.320666102784));
#38503=CARTESIAN_POINT('Ctrl Pts',(-89.2833567623059,-38.5346964531437,
121.268016595053));
#38504=CARTESIAN_POINT('Ctrl Pts',(-89.7823491181618,-37.872560629567,121.215367087322));
#38505=CARTESIAN_POINT('Ctrl Pts',(-90.1070645501236,-37.4416808426386,
121.181105825712));
#38506=CARTESIAN_POINT('Ctrl Pts',(-90.2799863217522,-36.8963900326682,
121.146844564102));
#38507=CARTESIAN_POINT('Ctrl Pts',(-90.2835504011883,-36.3531642868356,
121.112583302492));
#38508=CARTESIAN_POINT('Origin',(-87.7685555885722,-36.3549260746835,124.208423447177));
#38509=CARTESIAN_POINT('',(-90.8468255927006,-36.3541126078384,107.791576552823));
#38510=CARTESIAN_POINT('',(-90.8371847050479,-36.3546117509714,107.708423447177));
#38511=CARTESIAN_POINT('',(-90.8420555885722,-36.3549260746832,124.208423447177));
#38512=CARTESIAN_POINT('',(-86.9747563060399,-39.3241490284294,107.));
#38513=CARTESIAN_POINT('Ctrl Pts',(-90.8371847050479,-36.3546117509714,
107.708423447177));
#38514=CARTESIAN_POINT('Ctrl Pts',(-90.8375045645286,-35.8594362659055,
107.682880329042));
#38515=CARTESIAN_POINT('Ctrl Pts',(-90.4912522748027,-34.3441196931088,
107.604687703175));
#38516=CARTESIAN_POINT('Ctrl Pts',(-88.1200899635817,-32.7460643868788,
107.473845569577));
#38517=CARTESIAN_POINT('Ctrl Pts',(-84.9365304165877,-34.0865210383432,
107.315897046385));
#38518=CARTESIAN_POINT('Ctrl Pts',(-84.3257623763415,-37.4887078672662,
107.157948523192));
#38519=CARTESIAN_POINT('Ctrl Pts',(-85.9925177162683,-39.0615549760519,
107.052649507731));
#38520=CARTESIAN_POINT('Ctrl Pts',(-86.97475630604,-39.3241490284294,107.));
#38521=CARTESIAN_POINT('',(-88.5623548711056,-39.3241490284291,107.));
#38522=CARTESIAN_POINT('Origin',(-87.7685555885722,-36.3549260746835,107.));
#38523=CARTESIAN_POINT('Ctrl Pts',(-90.8468255927006,-36.3541126078384,
107.791576552823));
#38524=CARTESIAN_POINT('Ctrl Pts',(-90.8469816617586,-36.309603764564,107.789262006108));
#38525=CARTESIAN_POINT('Ctrl Pts',(-90.8260219475787,-35.2527942086462,
107.734297951662));
#38526=CARTESIAN_POINT('Ctrl Pts',(-89.6167529992886,-33.2347628855613,
107.626684389485));
#38527=CARTESIAN_POINT('Ctrl Pts',(-86.1660868316116,-33.1013875794135,
107.468735866293));
#38528=CARTESIAN_POINT('Ctrl Pts',(-84.1684777778814,-35.918700775767,107.3107873431));
#38529=CARTESIAN_POINT('Ctrl Pts',(-85.4209926009409,-39.0952448583635,
107.154542054336));
#38530=CARTESIAN_POINT('Ctrl Pts',(-87.6173027279392,-39.5801183929225,
107.050946273303));
#38531=CARTESIAN_POINT('Ctrl Pts',(-88.56426900845,-39.3292377960811,107.));
#38532=CARTESIAN_POINT('Origin',(-87.7685555885722,-36.3549260746835,124.208423447177));
#38533=CARTESIAN_POINT('',(-90.8384673493636,-36.3530606802369,108.791576552823));
#38534=CARTESIAN_POINT('',(-90.8436485370458,-36.357484352357,108.708423447177));
#38535=CARTESIAN_POINT('',(-90.8420555885722,-36.3549260746832,124.208423447177));
#38536=CARTESIAN_POINT('Ctrl Pts',(-90.8436485370458,-36.357484352357,108.708423447177));
#38537=CARTESIAN_POINT('Ctrl Pts',(-90.8362606803297,-35.5287363165806,
108.665444042093));
#38538=CARTESIAN_POINT('Ctrl Pts',(-90.0646116326147,-33.6726458843614,
108.569815129278));
#38539=CARTESIAN_POINT('Ctrl Pts',(-86.9355577566776,-32.8253529082965,
108.421536708732));
#38540=CARTESIAN_POINT('Ctrl Pts',(-84.3576615325144,-35.1229272723648,
108.26358818554));
#38541=CARTESIAN_POINT('Ctrl Pts',(-84.8723855412168,-38.5375840624727,
108.105639662347));
#38542=CARTESIAN_POINT('Ctrl Pts',(-88.0128424342027,-39.9731543052364,
107.947691139155));
#38543=CARTESIAN_POINT('Ctrl Pts',(-90.4599971769878,-38.4267875285153,
107.815285734098));
#38544=CARTESIAN_POINT('Ctrl Pts',(-90.8368452697583,-36.8800926082682,
107.735529836772));
#38545=CARTESIAN_POINT('Ctrl Pts',(-90.8371847050479,-36.3546117509714,
107.708423447177));
#38546=CARTESIAN_POINT('Ctrl Pts',(-90.8384673493637,-36.3530606802369,
108.791576552823));
#38547=CARTESIAN_POINT('Ctrl Pts',(-90.8406114808459,-35.9705776970889,
108.771825719159));
#38548=CARTESIAN_POINT('Ctrl Pts',(-90.5976170520827,-34.5711416081288,
108.699425377765));
#38549=CARTESIAN_POINT('Ctrl Pts',(-88.5106433977503,-32.8051167774314,
108.57437552864));
#38550=CARTESIAN_POINT('Ctrl Pts',(-85.2017899780534,-33.7929771900336,
108.416427005448));
#38551=CARTESIAN_POINT('Ctrl Pts',(-84.2201468213852,-37.1036893633033,
108.258478482255));
#38552=CARTESIAN_POINT('Ctrl Pts',(-86.4557339663443,-39.7354987833619,
108.100529959063));
#38553=CARTESIAN_POINT('Ctrl Pts',(-89.8314224577491,-39.3086388322812,
107.944895982585));
#38554=CARTESIAN_POINT('Ctrl Pts',(-90.8434315242634,-37.3220562992096,
107.841911513839));
#38555=CARTESIAN_POINT('Ctrl Pts',(-90.8468255927006,-36.3541126078384,
107.791576552823));
#38556=CARTESIAN_POINT('Origin',(-87.7685555885722,-36.3549260746835,124.208423447177));
#38557=CARTESIAN_POINT('',(-90.8403906014318,-36.3575187352786,109.791576552823));
#38558=CARTESIAN_POINT('',(-90.8446864850876,-36.3526580234404,109.708423447177));
#38559=CARTESIAN_POINT('',(-90.8420555885722,-36.3549260746832,124.208423447177));
#38560=CARTESIAN_POINT('Ctrl Pts',(-90.8446864850876,-36.3526580234404,
109.708423447177));
#38561=CARTESIAN_POINT('Ctrl Pts',(-90.8459256065026,-36.2030382733544,
109.700657262876));
#38562=CARTESIAN_POINT('Ctrl Pts',(-90.7682627105974,-35.0403882853119,
109.640241570843));
#38563=CARTESIAN_POINT('Ctrl Pts',(-89.2869056328921,-33.0615291810096,
109.52717637108));
#38564=CARTESIAN_POINT('Ctrl Pts',(-85.840854849815,-33.2831483419104,109.369227847887));
#38565=CARTESIAN_POINT('Ctrl Pts',(-84.1425912719677,-36.2898545213693,
109.211279324695));
#38566=CARTESIAN_POINT('Ctrl Pts',(-85.731880137862,-39.3555599790778,109.053330801502));
#38567=CARTESIAN_POINT('Ctrl Pts',(-89.1677588894168,-39.7006801261729,
108.89538227831));
#38568=CARTESIAN_POINT('Ctrl Pts',(-90.7452906984258,-37.7438433497054,
108.780413160201));
#38569=CARTESIAN_POINT('Ctrl Pts',(-90.8453107595136,-36.5439475795324,
108.718093549824));
#38570=CARTESIAN_POINT('Ctrl Pts',(-90.8436485370458,-36.357484352357,108.708423447177));
#38571=CARTESIAN_POINT('Ctrl Pts',(-90.8403906014318,-36.3575187352786,
109.791576552823));
#38572=CARTESIAN_POINT('Ctrl Pts',(-90.8345311555102,-35.6385125258615,
109.754389432211));
#38573=CARTESIAN_POINT('Ctrl Pts',(-90.225320179554,-33.8925906158493,109.664552803868));
#38574=CARTESIAN_POINT('Ctrl Pts',(-87.3251105792218,-32.7555919072101,
109.522066667795));
#38575=CARTESIAN_POINT('Ctrl Pts',(-84.5122325649308,-34.7586145140015,
109.364118144603));
#38576=CARTESIAN_POINT('Ctrl Pts',(-84.6517636253375,-38.2089644036472,
109.20616962141));
#38577=CARTESIAN_POINT('Ctrl Pts',(-87.6171951129081,-39.9783138396851,
109.048221098218));
#38578=CARTESIAN_POINT('Ctrl Pts',(-90.3318846828953,-38.6520013205392,
108.910023408688));
#38579=CARTESIAN_POINT('Ctrl Pts',(-90.8348959009886,-36.9901569777125,
108.82447522689));
#38580=CARTESIAN_POINT('Ctrl Pts',(-90.8384673493637,-36.3530606802369,
108.791576552823));
#38581=CARTESIAN_POINT('Origin',(-87.7685555885722,-36.3549260746835,124.208423447177));
#38582=CARTESIAN_POINT('',(-90.8468973805148,-36.3542412677562,110.791576552823));
#38583=CARTESIAN_POINT('',(-90.8372748127875,-36.3545776583154,110.708423447177));
#38584=CARTESIAN_POINT('',(-90.8420555885722,-36.3549260746832,124.208423447177));
#38585=CARTESIAN_POINT('Ctrl Pts',(-90.8372748127875,-36.3545776583154,
110.708423447177));
#38586=CARTESIAN_POINT('Ctrl Pts',(-90.8377741082269,-35.8660461342068,
110.683220975927));
#38587=CARTESIAN_POINT('Ctrl Pts',(-90.4981130409743,-34.3575981264578,
110.605368996946));
#38588=CARTESIAN_POINT('Ctrl Pts',(-88.142588178909,-32.7477180991385,110.474867510234));
#38589=CARTESIAN_POINT('Ctrl Pts',(-84.9525260101083,-34.0697943170025,
110.316918987042));
#38590=CARTESIAN_POINT('Ctrl Pts',(-84.3156722087998,-37.4637299947607,
110.158970463849));
#38591=CARTESIAN_POINT('Ctrl Pts',(-86.8094427648148,-39.8523468925606,
110.001021940657));
#38592=CARTESIAN_POINT('Ctrl Pts',(-90.0074379512479,-39.1084279923414,
109.850839601766));
#38593=CARTESIAN_POINT('Ctrl Pts',(-90.837525196471,-37.217359577444,109.753306770606));
#38594=CARTESIAN_POINT('Ctrl Pts',(-90.8446864850876,-36.3526580234404,
109.708423447177));
#38595=CARTESIAN_POINT('Ctrl Pts',(-90.8468973805148,-36.3542412677562,
110.791576552823));
#38596=CARTESIAN_POINT('Ctrl Pts',(-90.8470130244964,-36.3162849770529,
110.789602652993));
#38597=CARTESIAN_POINT('Ctrl Pts',(-90.8292490828189,-35.2660374732868,
110.734979245433));
#38598=CARTESIAN_POINT('Ctrl Pts',(-89.6367304343865,-33.2465868380812,
110.627706330142));
#38599=CARTESIAN_POINT('Ctrl Pts',(-86.18704996557,-33.091386581079,110.46975780695));
#38600=CARTESIAN_POINT('Ctrl Pts',(-84.1712725456449,-35.8951383259589,
110.311809283757));
#38601=CARTESIAN_POINT('Ctrl Pts',(-85.4170422546641,-39.1157656406506,
110.153860760565));
#38602=CARTESIAN_POINT('Ctrl Pts',(-88.794857584793,-39.8332236842038,109.995912237372));
#38603=CARTESIAN_POINT('Ctrl Pts',(-90.6659684787637,-37.9705917203656,
109.875150834792));
#38604=CARTESIAN_POINT('Ctrl Pts',(-90.8428269562679,-36.6564811762577,
109.807038939942));
#38605=CARTESIAN_POINT('Ctrl Pts',(-90.8403906014318,-36.3575187352786,
109.791576552823));
#38606=CARTESIAN_POINT('Origin',(-87.7685555885722,-36.3549260746835,124.208423447177));
#38607=CARTESIAN_POINT('',(-90.83859299684,-36.3529840191205,111.791576552823));
#38608=CARTESIAN_POINT('',(-90.8434556139163,-36.3575218683383,111.708423447177));
#38609=CARTESIAN_POINT('',(-90.8420555885722,-36.3549260746832,124.208423447177));
#38610=CARTESIAN_POINT('Ctrl Pts',(-90.8434556139163,-36.3575218683383,
111.708423447177));
#38611=CARTESIAN_POINT('Ctrl Pts',(-90.8360747346033,-35.535209872403,111.665784688979));
#38612=CARTESIAN_POINT('Ctrl Pts',(-90.0746147978365,-33.6854550212672,
111.570496423049));
#38613=CARTESIAN_POINT('Ctrl Pts',(-86.9582294999899,-32.8200680318722,
111.422558649389));
#38614=CARTESIAN_POINT('Ctrl Pts',(-84.3656606335548,-35.1010697521711,
111.264610126197));
#38615=CARTESIAN_POINT('Ctrl Pts',(-84.8583931283879,-38.5189048657011,
111.106661603004));
#38616=CARTESIAN_POINT('Ctrl Pts',(-87.9896814174328,-39.974726224009,110.948713079812));
#38617=CARTESIAN_POINT('Ctrl Pts',(-90.4528393566696,-38.4399663599021,
110.81596702787));
#38618=CARTESIAN_POINT('Ctrl Pts',(-90.8367310494397,-36.8866184423715,
110.735870483658));
#38619=CARTESIAN_POINT('Ctrl Pts',(-90.8372748127875,-36.3545776583154,
110.708423447177));
#38620=CARTESIAN_POINT('Ctrl Pts',(-90.8385929968401,-36.3529840191205,
111.791576552823));
#38621=CARTESIAN_POINT('Ctrl Pts',(-90.8407926739791,-35.9771364929294,
111.772166366045));
#38622=CARTESIAN_POINT('Ctrl Pts',(-90.603358358261,-34.5844968131842,111.700106671536));
#38623=CARTESIAN_POINT('Ctrl Pts',(-88.5334211681103,-32.8099534783274,
111.575397469297));
#38624=CARTESIAN_POINT('Ctrl Pts',(-85.218293678275,-33.7765517317041,111.417448946105));
#38625=CARTESIAN_POINT('Ctrl Pts',(-84.2154110997942,-37.0808835841375,
111.259500422912));
#38626=CARTESIAN_POINT('Ctrl Pts',(-86.4340565652882,-39.7270118417731,
111.10155189972));
#38627=CARTESIAN_POINT('Ctrl Pts',(-89.8198041827813,-39.3209117944618,
110.945577276356));
#38628=CARTESIAN_POINT('Ctrl Pts',(-90.8439284714653,-37.3286869192262,
110.842252160724));
#38629=CARTESIAN_POINT('Ctrl Pts',(-90.8468973805148,-36.3542412677562,
110.791576552823));
#38630=CARTESIAN_POINT('Origin',(-87.7685555885722,-36.3549260746835,124.208423447177));
#38631=CARTESIAN_POINT('',(-90.8402145091085,-36.3574820750184,112.791576552823));
#38632=CARTESIAN_POINT('',(-90.8448622668699,-36.352723779621,112.708423447177));
#38633=CARTESIAN_POINT('',(-90.8420555885722,-36.3549260746832,124.208423447177));
#38634=CARTESIAN_POINT('Ctrl Pts',(-90.8448622668699,-36.352723779621,112.708423447177));
#38635=CARTESIAN_POINT('Ctrl Pts',(-90.8460231303374,-36.2096880966529,
112.700997909761));
#38636=CARTESIAN_POINT('Ctrl Pts',(-90.7722168019337,-35.0536859832189,
112.640922864614));
#38637=CARTESIAN_POINT('Ctrl Pts',(-89.3080212851796,-33.0713464545818,
112.528198311736));
#38638=CARTESIAN_POINT('Ctrl Pts',(-85.8606183524605,-33.2708337842943,
112.370249788544));
#38639=CARTESIAN_POINT('Ctrl Pts',(-84.1430840844366,-36.2665737952763,
112.212301265351));
#38640=CARTESIAN_POINT('Ctrl Pts',(-85.7126545654799,-39.3424201308827,
112.054352742159));
#38641=CARTESIAN_POINT('Ctrl Pts',(-89.1462479767601,-39.7095964662598,
111.896404218967));
#38642=CARTESIAN_POINT('Ctrl Pts',(-90.7410211189894,-37.7571591976099,
111.781094453973));
#38643=CARTESIAN_POINT('Ctrl Pts',(-90.8451885005493,-36.5505847007566,
111.71843419671));
#38644=CARTESIAN_POINT('Ctrl Pts',(-90.8434556139163,-36.3575218683383,
111.708423447177));
#38645=CARTESIAN_POINT('Ctrl Pts',(-90.8402145091085,-36.3574820750184,
112.791576552823));
#38646=CARTESIAN_POINT('Ctrl Pts',(-90.8345154562364,-35.6449586686011,
112.754730079097));
#38647=CARTESIAN_POINT('Ctrl Pts',(-90.2341641452897,-33.9056535345118,
112.66523409764));
#38648=CARTESIAN_POINT('Ctrl Pts',(-87.3482310363601,-32.7528187283548,
112.523088608452));
#38649=CARTESIAN_POINT('Ctrl Pts',(-84.5225496142588,-34.7377386154233,
112.365140085259));
#38650=CARTESIAN_POINT('Ctrl Pts',(-84.6399230862583,-38.1889131872696,
112.207191562067));
#38651=CARTESIAN_POINT('Ctrl Pts',(-87.5939324950497,-39.9772674223311,
112.049243038875));
#38652=CARTESIAN_POINT('Ctrl Pts',(-90.3237946343547,-38.6651865970509,
111.91070470246));
#38653=CARTESIAN_POINT('Ctrl Pts',(-90.8348261204439,-36.9966108268173,
111.824815873776));
#38654=CARTESIAN_POINT('Ctrl Pts',(-90.8385929968401,-36.3529840191205,
111.791576552823));
#38655=CARTESIAN_POINT('Origin',(-87.7685555885722,-36.3549260746835,124.208423447177));
#38656=CARTESIAN_POINT('',(-90.8469566168618,-36.3543571629327,113.791576552823));
#38657=CARTESIAN_POINT('',(-90.837300689892,-36.3544727396314,113.708423447177));
#38658=CARTESIAN_POINT('',(-90.8420555885722,-36.3549260746832,124.208423447177));
#38659=CARTESIAN_POINT('Ctrl Pts',(-90.837300689892,-36.3544727396314,113.708423447178));
#38660=CARTESIAN_POINT('Ctrl Pts',(-90.8379418665799,-35.872554563717,113.683561622813));
#38661=CARTESIAN_POINT('Ctrl Pts',(-90.5047601145692,-34.370924135607,113.606050290717));
#38662=CARTESIAN_POINT('Ctrl Pts',(-88.1657423456717,-32.7501941245154,
113.475889450891));
#38663=CARTESIAN_POINT('Ctrl Pts',(-84.9672568878733,-34.0517597016134,
113.317940927699));
#38664=CARTESIAN_POINT('Ctrl Pts',(-84.3086237643501,-37.4415361815354,
113.159992404506));
#38665=CARTESIAN_POINT('Ctrl Pts',(-86.7870055967793,-39.8461163253272,
113.002043881314));
#38666=CARTESIAN_POINT('Ctrl Pts',(-89.9969760262728,-39.1211063400793,
112.851520895538));
#38667=CARTESIAN_POINT('Ctrl Pts',(-90.8377922257333,-37.2238582333192,
112.753647417492));
#38668=CARTESIAN_POINT('Ctrl Pts',(-90.8448622668699,-36.352723779621,112.708423447177));
#38669=CARTESIAN_POINT('Ctrl Pts',(-90.8469566168618,-36.3543571629327,
113.791576552823));
#38670=CARTESIAN_POINT('Ctrl Pts',(-90.8470373001381,-36.3229528215875,
113.789943299879));
#38671=CARTESIAN_POINT('Ctrl Pts',(-90.8324321314168,-35.2792756470073,
113.735660539204));
#38672=CARTESIAN_POINT('Ctrl Pts',(-89.6566505635712,-33.2586464637551,
113.628728270799));
#38673=CARTESIAN_POINT('Ctrl Pts',(-86.2080377498421,-33.081299013048,113.470779747607));
#38674=CARTESIAN_POINT('Ctrl Pts',(-84.1742989994849,-35.8720496562593,
113.312831224414));
#38675=CARTESIAN_POINT('Ctrl Pts',(-85.3993633840806,-39.1006096620336,
113.154882701222));
#38676=CARTESIAN_POINT('Ctrl Pts',(-88.7725022847651,-39.8397418653489,
112.996934178029));
#38677=CARTESIAN_POINT('Ctrl Pts',(-90.6608462681957,-37.983942532784,112.875832128563));
#38678=CARTESIAN_POINT('Ctrl Pts',(-90.842658768144,-36.6630752697567,112.807379586827));
#38679=CARTESIAN_POINT('Ctrl Pts',(-90.8402145091085,-36.3574820750184,
112.791576552823));
#38680=CARTESIAN_POINT('Origin',(-87.7685555885722,-36.3549260746835,124.208423447177));
#38681=CARTESIAN_POINT('',(-90.8387238989822,-36.3529100687362,114.791576552823));
#38682=CARTESIAN_POINT('',(-90.8432614306157,-36.357555014658,114.708423447177));
#38683=CARTESIAN_POINT('',(-90.8420555885722,-36.3549260746832,124.208423447177));
#38684=CARTESIAN_POINT('Ctrl Pts',(-90.8432614306156,-36.357555014658,114.708423447177));
#38685=CARTESIAN_POINT('Ctrl Pts',(-90.835899599694,-35.5416796238816,114.666125335864));
#38686=CARTESIAN_POINT('Ctrl Pts',(-90.0845449691903,-33.6982785475639,
114.571177716821));
#38687=CARTESIAN_POINT('Ctrl Pts',(-86.9809435225561,-32.814937799838,114.423580590046));
#38688=CARTESIAN_POINT('Ctrl Pts',(-84.3737817930479,-35.0792456171238,
114.265632066854));
#38689=CARTESIAN_POINT('Ctrl Pts',(-84.8445582165638,-38.5001741072118,
114.107683543661));
#38690=CARTESIAN_POINT('Ctrl Pts',(-87.9664341279196,-39.9760714509759,
113.949735020469));
#38691=CARTESIAN_POINT('Ctrl Pts',(-90.445741982759,-38.4532613953824,113.816648321641));
#38692=CARTESIAN_POINT('Ctrl Pts',(-90.8365840564492,-36.8931053630604,
113.736211130544));
#38693=CARTESIAN_POINT('Ctrl Pts',(-90.837300689892,-36.3544727396314,113.708423447178));
#38694=CARTESIAN_POINT('Ctrl Pts',(-90.8387238989822,-36.3529100687362,
114.791576552823));
#38695=CARTESIAN_POINT('Ctrl Pts',(-90.8409734017537,-35.9836982214461,
114.772507012931));
#38696=CARTESIAN_POINT('Ctrl Pts',(-90.6090449884476,-34.5978521515366,
114.700787965308));
#38697=CARTESIAN_POINT('Ctrl Pts',(-88.556167663902,-32.8149377579708,114.576419409954));
#38698=CARTESIAN_POINT('Ctrl Pts',(-85.2349019889955,-33.760229656792,114.418470886761));
#38699=CARTESIAN_POINT('Ctrl Pts',(-84.2108229752343,-37.058053883591,114.260522363569));
#38700=CARTESIAN_POINT('Ctrl Pts',(-86.4124319184404,-39.7183735107193,
114.102573840377));
#38701=CARTESIAN_POINT('Ctrl Pts',(-89.8081172856445,-39.3331822950034,
113.946258570128));
#38702=CARTESIAN_POINT('Ctrl Pts',(-90.8444363957291,-37.335302512349,113.84259280761));
#38703=CARTESIAN_POINT('Ctrl Pts',(-90.8469566168618,-36.3543571629327,
113.791576552823));
#38704=CARTESIAN_POINT('Origin',(-87.7685555885722,-36.3549260746835,124.208423447177));
#38705=CARTESIAN_POINT('',(-90.8400417237333,-36.357441449847,115.791576552823));
#38706=CARTESIAN_POINT('',(-90.8450341690572,-36.3527935650275,115.708423447177));
#38707=CARTESIAN_POINT('',(-90.8420555885722,-36.3549260746832,124.208423447177));
#38708=CARTESIAN_POINT('Ctrl Pts',(-90.8450341690572,-36.3527935650275,
115.708423447177));
#38709=CARTESIAN_POINT('Ctrl Pts',(-90.846116704552,-36.216339568469,115.701338556647));
#38710=CARTESIAN_POINT('Ctrl Pts',(-90.7761239871613,-35.0669805123168,
115.641604158385));
#38711=CARTESIAN_POINT('Ctrl Pts',(-89.3290734088453,-33.081299051764,115.529220252393));
#38712=CARTESIAN_POINT('Ctrl Pts',(-85.8804606359022,-33.2586465003749,
115.371271729201));
#38713=CARTESIAN_POINT('Ctrl Pts',(-84.1437261327331,-36.243296469925,115.213323206008));
#38714=CARTESIAN_POINT('Ctrl Pts',(-85.6935142529687,-39.3291576070487,
115.055374682816));
#38715=CARTESIAN_POINT('Ctrl Pts',(-89.1246792426668,-39.7183734709399,
114.897426159623));
#38716=CARTESIAN_POINT('Ctrl Pts',(-90.7367043057794,-37.7704789876537,
114.781775747744));
#38717=CARTESIAN_POINT('Ctrl Pts',(-90.8450630531436,-36.5572199485125,
114.718774843595));
#38718=CARTESIAN_POINT('Ctrl Pts',(-90.8432614306156,-36.357555014658,114.708423447177));
#38719=CARTESIAN_POINT('Ctrl Pts',(-90.8400417237333,-36.357441449847,115.791576552823));
#38720=CARTESIAN_POINT('Ctrl Pts',(-90.8345081309196,-35.6514047555258,
115.755070725982));
#38721=CARTESIAN_POINT('Ctrl Pts',(-90.2429419326533,-33.9187286136303,
115.665915391411));
#38722=CARTESIAN_POINT('Ctrl Pts',(-87.3713688267741,-32.750194081883,115.524110549109));
#38723=CARTESIAN_POINT('Ctrl Pts',(-84.5330004881805,-34.7169293542972,
115.366162025916));
#38724=CARTESIAN_POINT('Ctrl Pts',(-84.628211554152,-38.1687864356674,115.208213502724));
#38725=CARTESIAN_POINT('Ctrl Pts',(-87.5706770468859,-39.9760714938026,
115.050264979531));
#38726=CARTESIAN_POINT('Ctrl Pts',(-90.3156407155774,-38.6783630959069,
114.911385996231));
#38727=CARTESIAN_POINT('Ctrl Pts',(-90.834762700592,-37.0030632464158,114.825156520661));
#38728=CARTESIAN_POINT('Ctrl Pts',(-90.8387238989822,-36.3529100687362,
114.791576552823));
#38729=CARTESIAN_POINT('Origin',(-87.7685555885722,-36.3549260746835,124.208423447177));
#38730=CARTESIAN_POINT('',(-90.8470055221225,-36.3544743326472,116.791576552823));
#38731=CARTESIAN_POINT('',(-90.8373333345046,-36.3543684810828,116.708423447177));
#38732=CARTESIAN_POINT('',(-90.8420555885722,-36.3549260746832,124.208423447177));
#38733=CARTESIAN_POINT('Ctrl Pts',(-90.8373333345046,-36.3543684810828,
116.708423447177));
#38734=CARTESIAN_POINT('Ctrl Pts',(-90.838111639097,-35.8790659960872,116.683902269699));
#38735=CARTESIAN_POINT('Ctrl Pts',(-90.5113488468397,-34.3842533323872,
116.606731584489));
#38736=CARTESIAN_POINT('Ctrl Pts',(-88.1888801358119,-32.7528187709561,
116.476911391548));
#38737=CARTESIAN_POINT('Ctrl Pts',(-84.9821032637396,-34.0338200465123,
116.318962868356));
#38738=CARTESIAN_POINT('Ctrl Pts',(-84.3017179684765,-37.4192975645625,
116.161014345163));
#38739=CARTESIAN_POINT('Ctrl Pts',(-86.7646089042542,-39.839741824135,116.003065821971));
#38740=CARTESIAN_POINT('Ctrl Pts',(-89.9864432824828,-39.1337639166678,
115.852202189309));
#38741=CARTESIAN_POINT('Ctrl Pts',(-90.8380721256472,-37.2303616928352,
115.753988064378));
#38742=CARTESIAN_POINT('Ctrl Pts',(-90.8450341690572,-36.3527935650275,
115.708423447177));
#38743=CARTESIAN_POINT('Ctrl Pts',(-90.8470055221225,-36.3544743326472,
116.791576552823));
#38744=CARTESIAN_POINT('Ctrl Pts',(-90.8470570093793,-36.3296210426277,
116.790283946765));
#38745=CARTESIAN_POINT('Ctrl Pts',(-90.8355715211677,-35.2925100683326,
116.736341832976));
#38746=CARTESIAN_POINT('Ctrl Pts',(-89.6764928472477,-33.2708337478186,
116.629750211456));
#38747=CARTESIAN_POINT('Ctrl Pts',(-86.2290898737567,-33.071346415748,116.471801688264));
#38748=CARTESIAN_POINT('Ctrl Pts',(-84.1774736431561,-35.848980894873,116.313853165071));
#38749=CARTESIAN_POINT('Ctrl Pts',(-85.3817821946438,-39.0853404809052,
116.155904641879));
#38750=CARTESIAN_POINT('Ctrl Pts',(-88.7501055919751,-39.8461163666165,
115.997956118686));
#38751=CARTESIAN_POINT('Ctrl Pts',(-90.655671847336,-37.9972943972299,115.876513422334));
#38752=CARTESIAN_POINT('Ctrl Pts',(-90.8424888003863,-36.6696664308027,
115.807720233713));
#38753=CARTESIAN_POINT('Ctrl Pts',(-90.8400417237333,-36.357441449847,115.791576552823));
#38754=CARTESIAN_POINT('Origin',(-87.7685555885722,-36.3549260746835,124.208423447177));
#38755=CARTESIAN_POINT('',(-90.838859936608,-36.3528391395051,117.791576552823));
#38756=CARTESIAN_POINT('',(-90.8430662275438,-36.3575836912129,117.708423447178));
#38757=CARTESIAN_POINT('',(-90.8420555885722,-36.3549260746832,124.208423447177));
#38758=CARTESIAN_POINT('Ctrl Pts',(-90.8430662275438,-36.3575836912129,
117.708423447178));
#38759=CARTESIAN_POINT('Ctrl Pts',(-90.8357358095233,-35.5481464964534,
117.66646598275));
#38760=CARTESIAN_POINT('Ctrl Pts',(-90.0944058341935,-33.7111196198065,
117.571859010592));
#38761=CARTESIAN_POINT('Ctrl Pts',(-87.0036900180789,-32.8099535202534,
117.424602530703));
#38762=CARTESIAN_POINT('Ctrl Pts',(-84.382042917881,-35.0574740779507,117.26665400751));
#38763=CARTESIAN_POINT('Ctrl Pts',(-84.8308438600728,-38.4813549008641,
117.108705484318));
#38764=CARTESIAN_POINT('Ctrl Pts',(-87.9431786800308,-39.9772673794902,
116.950756961126));
#38765=CARTESIAN_POINT('Ctrl Pts',(-90.4385842843359,-38.4665514124466,
116.817329615412));
#38766=CARTESIAN_POINT('Ctrl Pts',(-90.8364405385272,-36.8995896589381,
116.736551777429));
#38767=CARTESIAN_POINT('Ctrl Pts',(-90.8373333345046,-36.3543684810828,
116.708423447177));
#38768=CARTESIAN_POINT('Ctrl Pts',(-90.838859936608,-36.3528391395051,117.791576552823));
#38769=CARTESIAN_POINT('Ctrl Pts',(-90.8411535687101,-35.9902631012329,
117.772847659816));
#38770=CARTESIAN_POINT('Ctrl Pts',(-90.6146772191493,-34.6112077247612,
117.701469259079));
#38771=CARTESIAN_POINT('Ctrl Pts',(-88.5788816867368,-32.8200679900657,
117.577441350611));
#38772=CARTESIAN_POINT('Ctrl Pts',(-85.2516147613512,-33.7440145603012,
117.419492827418));
#38773=CARTESIAN_POINT('Ctrl Pts',(-84.2063815347296,-37.0351951933252,
117.261544304226));
#38774=CARTESIAN_POINT('Ctrl Pts',(-86.390863184092,-39.7095965059354,117.103595781033));
#38775=CARTESIAN_POINT('Ctrl Pts',(-89.7963570779285,-39.3454250335693,
116.946939863899));
#38776=CARTESIAN_POINT('Ctrl Pts',(-90.8449598671701,-37.3419275198467,
116.842933454495));
#38777=CARTESIAN_POINT('Ctrl Pts',(-90.8470055221225,-36.3544743326472,
116.791576552823));
#38778=CARTESIAN_POINT('Origin',(-87.7685555885722,-36.3549260746835,124.208423447177));
#38779=CARTESIAN_POINT('',(-90.8398724656877,-36.357396938907,118.791576552823));
#38780=CARTESIAN_POINT('',(-90.8452018287892,-36.3528672805891,118.708423447178));
#38781=CARTESIAN_POINT('',(-90.8420555885722,-36.3549260746832,124.208423447177));
#38782=CARTESIAN_POINT('Ctrl Pts',(-90.8452018287892,-36.3528672805891,
118.708423447178));
#38783=CARTESIAN_POINT('Ctrl Pts',(-90.8462062638201,-36.2229926114565,
118.701679203533));
#38784=CARTESIAN_POINT('Ctrl Pts',(-90.7799844648685,-35.0802718156704,
118.642285452157));
#38785=CARTESIAN_POINT('Ctrl Pts',(-89.350061192869,-33.0913866196758,118.53024219305));
#38786=CARTESIAN_POINT('Ctrl Pts',(-85.9003807648513,-33.2465868748436,
118.372293669858));
#38787=CARTESIAN_POINT('Ctrl Pts',(-84.1445176314521,-36.2200237470817,
118.214345146665));
#38788=CARTESIAN_POINT('Ctrl Pts',(-85.6744594936806,-39.3157724566742,
118.056396623473));
#38789=CARTESIAN_POINT('Ctrl Pts',(-89.1030545960746,-39.7270118018916,
117.89844810028));
#38790=CARTESIAN_POINT('Ctrl Pts',(-90.7323387978003,-37.783801391323,117.782457041515));
#38791=CARTESIAN_POINT('Ctrl Pts',(-90.8449342419241,-36.5638530083872,
117.719115490481));
#38792=CARTESIAN_POINT('Ctrl Pts',(-90.8430662275438,-36.3575836912129,
117.708423447178));
#38793=CARTESIAN_POINT('Ctrl Pts',(-90.8398724656877,-36.357396938907,118.791576552823));
#38794=CARTESIAN_POINT('Ctrl Pts',(-90.8345089923071,-35.6578509331832,
118.755411372868));
#38795=CARTESIAN_POINT('Ctrl Pts',(-90.2516537491596,-33.931815551476,118.666596685182));
#38796=CARTESIAN_POINT('Ctrl Pts',(-87.3945229938104,-32.7477180564772,
118.525132489766));
#38797=CARTESIAN_POINT('Ctrl Pts',(-84.5435847625254,-34.6961876275626,
118.367183966573));
#38798=CARTESIAN_POINT('Ctrl Pts',(-84.6166294974947,-38.1485848990669,
118.209235443381));
#38799=CARTESIAN_POINT('Ctrl Pts',(-87.5474297570977,-39.9747262668198,
118.051286920188));
#38800=CARTESIAN_POINT('Ctrl Pts',(-90.3074226582739,-38.6915302645955,
117.912067290002));
#38801=CARTESIAN_POINT('Ctrl Pts',(-90.8347058517495,-37.0095144752193,
117.825497167547));
#38802=CARTESIAN_POINT('Ctrl Pts',(-90.838859936608,-36.3528391395051,117.791576552823));
#38803=CARTESIAN_POINT('Origin',(-87.7685555885722,-36.3549260746835,124.208423447177));
#38804=CARTESIAN_POINT('',(-90.8470437519384,-36.3545924749754,119.791576552823));
#38805=CARTESIAN_POINT('',(-90.8373727075233,-36.3542650492899,119.708423447177));
#38806=CARTESIAN_POINT('',(-90.8420555885722,-36.3549260746832,124.208423447177));
#38807=CARTESIAN_POINT('Ctrl Pts',(-90.8373727075233,-36.3542650492899,
119.708423447177));
#38808=CARTESIAN_POINT('Ctrl Pts',(-90.8382832605688,-35.8855804672779,
119.684242916584));
#38809=CARTESIAN_POINT('Ctrl Pts',(-90.5178794747935,-34.3975854901708,
119.60741287826));
#38810=CARTESIAN_POINT('Ctrl Pts',(-88.2120005926768,-32.7555919497842,
119.477933332205));
#38811=CARTESIAN_POINT('Ctrl Pts',(-84.9970645257212,-34.0159760806577,
119.319984809012));
#38812=CARTESIAN_POINT('Ctrl Pts',(-84.2949551082748,-37.3970150683708,
119.16203628582));
#38813=CARTESIAN_POINT('Ctrl Pts',(-86.7422536044908,-39.8332236430662,
119.004087762628));
#38814=CARTESIAN_POINT('Ctrl Pts',(-89.9758395670128,-39.1464003470619,
118.85288348308));
#38815=CARTESIAN_POINT('Ctrl Pts',(-90.8383650569023,-37.2368701871385,
118.754328711263));
#38816=CARTESIAN_POINT('Ctrl Pts',(-90.8452018287892,-36.3528672805891,
118.708423447178));
#38817=CARTESIAN_POINT('Ctrl Pts',(-90.8470437519384,-36.3545924749754,
119.791576552823));
#38818=CARTESIAN_POINT('Ctrl Pts',(-90.84707219677,-36.3362895054686,119.79062459365));
#38819=CARTESIAN_POINT('Ctrl Pts',(-90.838667553572,-35.3057405991472,119.737023126747));
#38820=CARTESIAN_POINT('Ctrl Pts',(-89.6962563501485,-33.2831483055448,
119.630772152113));
#38821=CARTESIAN_POINT('Ctrl Pts',(-86.2502055262826,-33.0615291420779,
119.47282362892));
#38822=CARTESIAN_POINT('Ctrl Pts',(-84.1807963181542,-35.8259330212369,
119.314875105728));
#38823=CARTESIAN_POINT('Ctrl Pts',(-85.3642994245004,-39.0699587122372,
119.156926582536));
#38824=CARTESIAN_POINT('Ctrl Pts',(-88.7276684236758,-39.8523469339212,
118.998978059343));
#38825=CARTESIAN_POINT('Ctrl Pts',(-90.6504449905735,-38.010647188406,118.877194716105));
#38826=CARTESIAN_POINT('Ctrl Pts',(-90.8423171722627,-36.6762546265272,
118.808060880599));
#38827=CARTESIAN_POINT('Ctrl Pts',(-90.8398724656877,-36.357396938907,118.791576552823));
#38828=CARTESIAN_POINT('Origin',(-87.7685555885722,-36.3549260746835,124.208423447177));
#38829=CARTESIAN_POINT('',(-90.8389971204791,-36.3527751889037,120.791576552823));
#38830=CARTESIAN_POINT('',(-90.8428699659751,-36.357609793043,120.708423447177));
#38831=CARTESIAN_POINT('',(-90.8420555885722,-36.3549260746832,124.208423447177));
#38832=CARTESIAN_POINT('Ctrl Pts',(-90.8428699659751,-36.357609793043,120.708423447177));
#38833=CARTESIAN_POINT('Ctrl Pts',(-90.8355828378088,-35.5546125768694,
120.666806629636));
#38834=CARTESIAN_POINT('Ctrl Pts',(-90.1041980565863,-33.72397525936,120.572540304363));
#38835=CARTESIAN_POINT('Ctrl Pts',(-87.0264677882008,-32.8051168197105,
120.42562447136));
#38836=CARTESIAN_POINT('Ctrl Pts',(-84.3904437941137,-35.0357553412809,
120.267675948167));
#38837=CARTESIAN_POINT('Ctrl Pts',(-84.8172505627962,-38.4624483585915,
120.109727424975));
#38838=CARTESIAN_POINT('Ctrl Pts',(-87.9199160624454,-39.9783137967903,
119.951778901782));
#38839=CARTESIAN_POINT('Ctrl Pts',(-90.4313660245834,-38.4798362252759,
119.818010909183));
#38840=CARTESIAN_POINT('Ctrl Pts',(-90.8363006667865,-36.9060714126157,
119.736892424315));
#38841=CARTESIAN_POINT('Ctrl Pts',(-90.8373727075233,-36.3542650492899,
119.708423447177));
#38842=CARTESIAN_POINT('Ctrl Pts',(-90.8389971204791,-36.3527751889037,
120.791576552823));
#38843=CARTESIAN_POINT('Ctrl Pts',(-90.8413324494673,-35.9968317106162,
120.773188306702));
#38844=CARTESIAN_POINT('Ctrl Pts',(-90.6202676404303,-34.6245509810165,
120.70215055285));
#38845=CARTESIAN_POINT('Ctrl Pts',(-88.6015534311407,-32.8253528646868,
120.578463291268));
#38846=CARTESIAN_POINT('Ctrl Pts',(-85.2684356186448,-33.7279027825514,
120.420514768075));
#38847=CARTESIAN_POINT('Ctrl Pts',(-84.2020848645994,-37.0123105603124,
120.262566244883));
#38848=CARTESIAN_POINT('Ctrl Pts',(-86.3693522710391,-39.7006801660047,
120.10461772169));
#38849=CARTESIAN_POINT('Ctrl Pts',(-89.7845229475026,-39.3576400610631,
119.94762115767));
#38850=CARTESIAN_POINT('Ctrl Pts',(-90.8454990133535,-37.3485622609709,
119.843274101381));
#38851=CARTESIAN_POINT('Ctrl Pts',(-90.8470437519384,-36.3545924749754,
119.791576552823));
#38852=CARTESIAN_POINT('Origin',(-87.7685555885722,-36.3549260746835,124.208423447177));
#38853=CARTESIAN_POINT('',(-90.8388341582581,-36.3579404435482,121.791576552823));
#38854=CARTESIAN_POINT('',(-90.8453551362697,-36.3529984899081,121.708423447177));
#38855=CARTESIAN_POINT('',(-90.8420555885722,-36.3549260746832,124.208423447177));
#38856=CARTESIAN_POINT('',(-88.5623548711056,-39.3241490284291,122.));
#38857=CARTESIAN_POINT('Ctrl Pts',(-88.5623548711056,-39.3241490284291,
122.));
#38858=CARTESIAN_POINT('Ctrl Pts',(-89.5445934608772,-39.0615549760513,
121.947350492269));
#38859=CARTESIAN_POINT('Ctrl Pts',(-90.644289976571,-38.0238171899135,121.877876009877));
#38860=CARTESIAN_POINT('Ctrl Pts',(-90.8411753108947,-36.6834161555448,
121.808401527484));
#38861=CARTESIAN_POINT('Ctrl Pts',(-90.8388341582581,-36.3579404435482,
121.791576552823));
#38862=CARTESIAN_POINT('',(-86.9728468160199,-39.3292254485229,122.));
#38863=CARTESIAN_POINT('Origin',(-87.7685555885722,-36.3549260746835,122.));
#38864=CARTESIAN_POINT('Ctrl Pts',(-86.9728421809427,-39.3292377709744,
122.));
#38865=CARTESIAN_POINT('Ctrl Pts',(-87.9198084892423,-39.5801183955144,
121.949053726697));
#38866=CARTESIAN_POINT('Ctrl Pts',(-89.9803573410806,-39.1252163986582,
121.851861542423));
#38867=CARTESIAN_POINT('Ctrl Pts',(-90.8386916486268,-37.2432731849997,
121.754669358149));
#38868=CARTESIAN_POINT('Ctrl Pts',(-90.8453551362697,-36.3529984899081,
121.708423447177));
#38869=CARTESIAN_POINT('Origin',(36.3549260746835,-87.7685555885722,114.));
#38870=CARTESIAN_POINT('',(33.8414157234842,-87.7682981463998,107.387416697508));
#38871=CARTESIAN_POINT('',(33.839334999722,-87.7721278037521,107.112583302492));
#38872=CARTESIAN_POINT('',(33.8374260746835,-87.7685555885722,114.));
#38873=CARTESIAN_POINT('',(34.4414600780189,-86.1325683851968,107.));
#38874=CARTESIAN_POINT('Ctrl Pts',(33.839334999722,-87.7721278037521,107.112583302492));
#38875=CARTESIAN_POINT('Ctrl Pts',(33.8444805530708,-87.1794933281653,107.075055534995));
#38876=CARTESIAN_POINT('Ctrl Pts',(34.0557042465997,-86.5837520282674,107.037527767497));
#38877=CARTESIAN_POINT('Ctrl Pts',(34.441460078019,-86.1325683851967,107.));
#38878=CARTESIAN_POINT('',(33.8374260746835,-87.7685555885722,107.));
#38879=CARTESIAN_POINT('Origin',(36.3549260746835,-87.7685555885722,107.));
#38880=CARTESIAN_POINT('',(33.8374260746835,-87.7685555885722,106.));
#38881=CARTESIAN_POINT('',(33.8374260746835,-87.7685555885722,114.));
#38882=CARTESIAN_POINT('Origin',(36.3549260746835,-87.7685555885722,106.));
#38883=CARTESIAN_POINT('',(38.2720363880079,-86.1300276126115,107.));
#38884=CARTESIAN_POINT('Origin',(36.3549260746835,-87.7685555885722,107.));
#38885=CARTESIAN_POINT('Ctrl Pts',(38.2720452344323,-86.1300214449936,107.));
#38886=CARTESIAN_POINT('Ctrl Pts',(37.7492246942328,-85.5213064718756,107.050946273303));
#38887=CARTESIAN_POINT('Ctrl Pts',(36.9095001441611,-85.1811299415284,107.101892546605));
#38888=CARTESIAN_POINT('Ctrl Pts',(36.1108292477348,-85.2588926940752,107.152838819908));
#38889=CARTESIAN_POINT('Ctrl Pts',(35.2854572075469,-85.3392552088574,107.205488327639));
#38890=CARTESIAN_POINT('Ctrl Pts',(34.503929715814,-85.8659692054928,107.25813783537));
#38891=CARTESIAN_POINT('Ctrl Pts',(34.1200450888798,-86.6007560202748,107.3107873431));
#38892=CARTESIAN_POINT('Ctrl Pts',(33.9338019348801,-86.9572407667346,107.336330461236));
#38893=CARTESIAN_POINT('Ctrl Pts',(33.8411537247362,-87.3627005243321,107.361873579372));
#38894=CARTESIAN_POINT('Ctrl Pts',(33.8414157234842,-87.7682981463998,107.387416697508));
#38895=CARTESIAN_POINT('Origin',(36.3549260746835,-87.7685555885722,114.));
#38896=CARTESIAN_POINT('',(33.8361212073215,-87.7706510705991,108.387416697508));
#38897=CARTESIAN_POINT('',(33.833519260677,-87.7678892624363,108.112583302492));
#38898=CARTESIAN_POINT('',(33.8374260746835,-87.7685555885722,114.));
#38899=CARTESIAN_POINT('Ctrl Pts',(33.833519260677,-87.7678892624363,108.112583302492));
#38900=CARTESIAN_POINT('Ctrl Pts',(33.8333914248761,-87.7314321292875,108.110268755777));
#38901=CARTESIAN_POINT('Ctrl Pts',(33.8341143758752,-87.6949802329165,108.107954209062));
#38902=CARTESIAN_POINT('Ctrl Pts',(33.8357039923662,-87.6585662348268,108.105639662347));
#38903=CARTESIAN_POINT('Ctrl Pts',(33.8718633514296,-86.8302489398792,108.052990154616));
#38904=CARTESIAN_POINT('Ctrl Pts',(34.3564667264384,-86.0215415840135,108.000340646886));
#38905=CARTESIAN_POINT('Ctrl Pts',(35.0698410633522,-85.5989799369826,107.947691139155));
#38906=CARTESIAN_POINT('Ctrl Pts',(35.7832154002661,-85.1764182899517,107.895041631424));
#38907=CARTESIAN_POINT('Ctrl Pts',(36.725360699085,-85.1400023517557,107.842392123693));
#38908=CARTESIAN_POINT('Ctrl Pts',(37.4691398688133,-85.5064040383691,107.789742615962));
#38909=CARTESIAN_POINT('Ctrl Pts',(38.2129190385417,-85.8728057249826,107.737093108232));
#38910=CARTESIAN_POINT('Ctrl Pts',(38.7583320791794,-86.6420250364055,107.684443600501));
#38911=CARTESIAN_POINT('Ctrl Pts',(38.8581856892655,-87.4650122829143,107.63179409277));
#38912=CARTESIAN_POINT('Ctrl Pts',(38.9580392993515,-88.2879995294231,107.579144585039));
#38913=CARTESIAN_POINT('Ctrl Pts',(38.612333478886,-89.1647547110178,107.526495077308));
#38914=CARTESIAN_POINT('Ctrl Pts',(37.9776636366484,-89.6985066213742,107.473845569577));
#38915=CARTESIAN_POINT('Ctrl Pts',(37.3429937944108,-90.2322585317306,107.421196061847));
#38916=CARTESIAN_POINT('Ctrl Pts',(36.4193599304013,-90.4230071708486,107.368546554116));
#38917=CARTESIAN_POINT('Ctrl Pts',(35.6257427015425,-90.1828530278179,107.315897046385));
#38918=CARTESIAN_POINT('Ctrl Pts',(34.8321254726837,-89.9426988847871,107.263247538654));
#38919=CARTESIAN_POINT('Ctrl Pts',(34.1685248789757,-89.2716419596076,107.210598030923));
#38920=CARTESIAN_POINT('Ctrl Pts',(33.9355596837291,-88.4773561362653,107.157948523192));
#38921=CARTESIAN_POINT('Ctrl Pts',(33.868648532651,-88.2492251544312,107.142826782959));
#38922=CARTESIAN_POINT('Ctrl Pts',(33.8372616091025,-88.0109287021499,107.127705042725));
#38923=CARTESIAN_POINT('Ctrl Pts',(33.839334999722,-87.7721278037521,107.112583302492));
#38924=CARTESIAN_POINT('Ctrl Pts',(33.8414157234842,-87.7682981463998,107.387416697508));
#38925=CARTESIAN_POINT('Ctrl Pts',(33.8416937568902,-88.1987188610546,107.414523087103));
#38926=CARTESIAN_POINT('Ctrl Pts',(33.9466024502664,-88.6292948315277,107.441629476698));
#38927=CARTESIAN_POINT('Ctrl Pts',(34.1553234974974,-89.0016622559541,107.468735866293));
#38928=CARTESIAN_POINT('Ctrl Pts',(34.5607282951845,-89.7249220439228,107.521385374024));
#38929=CARTESIAN_POINT('Ctrl Pts',(35.3577796526943,-90.2285819869318,107.574034881754));
#38930=CARTESIAN_POINT('Ctrl Pts',(36.1850293994859,-90.284432979621,107.626684389485));
#38931=CARTESIAN_POINT('Ctrl Pts',(37.0122791462776,-90.3402839723102,107.679333897216));
#38932=CARTESIAN_POINT('Ctrl Pts',(37.869727282351,-89.9483260146797,107.731983404947));
#38933=CARTESIAN_POINT('Ctrl Pts',(38.3687196497657,-89.28619017419,107.784632912678));
#38934=CARTESIAN_POINT('Ctrl Pts',(38.8677120171805,-88.6240543337003,107.837282420409));
#38935=CARTESIAN_POINT('Ctrl Pts',(39.0082486159366,-87.6917406103514,107.889931928139));
#38936=CARTESIAN_POINT('Ctrl Pts',(38.7265916429298,-86.9119270220054,107.94258143587));
#38937=CARTESIAN_POINT('Ctrl Pts',(38.4449346699229,-86.1321134336593,107.995230943601));
#38938=CARTESIAN_POINT('Ctrl Pts',(37.741084125153,-85.5047999803161,108.047880451332));
#38939=CARTESIAN_POINT('Ctrl Pts',(36.9341334049065,-85.3143561749413,108.100529959063));
#38940=CARTESIAN_POINT('Ctrl Pts',(36.1271826846599,-85.1239123695665,108.153179466794));
#38941=CARTESIAN_POINT('Ctrl Pts',(35.2171317889366,-85.3703382121602,108.205828974524));
#38942=CARTESIAN_POINT('Ctrl Pts',(34.6165319102364,-85.9419268590616,108.258478482255));
#38943=CARTESIAN_POINT('Ctrl Pts',(34.126243841216,-86.4085321713532,108.301457887339));
#38944=CARTESIAN_POINT('Ctrl Pts',(33.8421725915064,-87.0918245700457,108.344437292424));
#38945=CARTESIAN_POINT('Ctrl Pts',(33.8361212073215,-87.7706510705991,108.387416697508));
#38946=CARTESIAN_POINT('Origin',(36.3549260746835,-87.7685555885722,114.));
#38947=CARTESIAN_POINT('',(33.8352710252958,-87.7666978305704,109.387416697508));
#38948=CARTESIAN_POINT('',(33.8403654904393,-87.7670276461582,109.112583302492));
#38949=CARTESIAN_POINT('',(33.8374260746835,-87.7685555885722,114.));
#38950=CARTESIAN_POINT('Ctrl Pts',(33.8403654904393,-87.7670276461582,109.112583302492));
#38951=CARTESIAN_POINT('Ctrl Pts',(33.8386092352284,-87.4537363502728,109.092832468829));
#38952=CARTESIAN_POINT('Ctrl Pts',(33.8929064240409,-87.1410318741097,109.073081635165));
#38953=CARTESIAN_POINT('Ctrl Pts',(34.0060459886766,-86.851305712434,109.053330801502));
#38954=CARTESIAN_POINT('Ctrl Pts',(34.3076404673954,-86.0789869309084,109.000681293771));
#38955=CARTESIAN_POINT('Ctrl Pts',(35.0273617091834,-85.4699492562897,108.94803178604));
#38956=CARTESIAN_POINT('Ctrl Pts',(35.8389352257471,-85.3002896064973,108.89538227831));
#38957=CARTESIAN_POINT('Ctrl Pts',(36.6505087423109,-85.1306299567049,108.842732770579));
#38958=CARTESIAN_POINT('Ctrl Pts',(37.5539345336504,-85.4003483317387,108.790083262848));
#38959=CARTESIAN_POINT('Ctrl Pts',(38.1396578606632,-85.9871741676922,108.737433755117));
#38960=CARTESIAN_POINT('Ctrl Pts',(38.7253811876761,-86.5740000036457,108.684784247386));
#38961=CARTESIAN_POINT('Ctrl Pts',(38.9934020503622,-87.4779333005189,108.632134739655));
#38962=CARTESIAN_POINT('Ctrl Pts',(38.8222180782562,-88.2891852027425,108.579485231925));
#38963=CARTESIAN_POINT('Ctrl Pts',(38.6510341061502,-89.1004371049661,108.526835724194));
#38964=CARTESIAN_POINT('Ctrl Pts',(38.0406452992521,-89.81900761254,108.474186216463));
#38965=CARTESIAN_POINT('Ctrl Pts',(37.2677604715886,-90.1191528459469,108.421536708732));
#38966=CARTESIAN_POINT('Ctrl Pts',(36.4948756439251,-90.4192980793539,108.368887201001));
#38967=CARTESIAN_POINT('Ctrl Pts',(35.5594947954961,-90.3010180385939,108.316237693271));
#38968=CARTESIAN_POINT('Ctrl Pts',(34.8856620428406,-89.817914401199,108.26358818554));
#38969=CARTESIAN_POINT('Ctrl Pts',(34.2414519296223,-89.3560486819745,108.213253224524));
#38970=CARTESIAN_POINT('Ctrl Pts',(33.8362993342051,-88.5607306269994,108.162918263508));
#38971=CARTESIAN_POINT('Ctrl Pts',(33.833519260677,-87.7678892624363,108.112583302492));
#38972=CARTESIAN_POINT('Ctrl Pts',(33.8361212073215,-87.7706510705991,108.387416697508));
#38973=CARTESIAN_POINT('Ctrl Pts',(33.8347596829796,-87.9233828714858,108.397086800155));
#38974=CARTESIAN_POINT('Ctrl Pts',(33.8474721473246,-88.0758885985998,108.406756902801));
#38975=CARTESIAN_POINT('Ctrl Pts',(33.8750764150749,-88.2256493871394,108.416427005448));
#38976=CARTESIAN_POINT('Ctrl Pts',(34.0253696602909,-89.0410318171065,108.469076513179));
#38977=CARTESIAN_POINT('Ctrl Pts',(34.6171050124002,-89.7750452258316,108.521726020909));
#38978=CARTESIAN_POINT('Ctrl Pts',(35.3820267013402,-90.0949373484143,108.57437552864));
#38979=CARTESIAN_POINT('Ctrl Pts',(36.1469483902803,-90.4148294709971,108.627025036371));
#38980=CARTESIAN_POINT('Ctrl Pts',(37.0850564160513,-90.3206003074374,108.679674544102));
#38981=CARTESIAN_POINT('Ctrl Pts',(37.7710745227806,-89.8549664615314,108.732324051833));
#38982=CARTESIAN_POINT('Ctrl Pts',(38.4570926295099,-89.3893326156255,108.784973559563));
#38983=CARTESIAN_POINT('Ctrl Pts',(38.8910208171977,-88.5522940873732,108.837623067294));
#38984=CARTESIAN_POINT('Ctrl Pts',(38.8761439749966,-87.7233099317579,108.890272575025));
#38985=CARTESIAN_POINT('Ctrl Pts',(38.8612671327955,-86.8943257761426,108.942922082756));
#38986=CARTESIAN_POINT('Ctrl Pts',(38.3975852607055,-86.0733959931642,108.995571590487));
#38987=CARTESIAN_POINT('Ctrl Pts',(37.6953016620874,-85.6326764378238,109.048221098218));
#38988=CARTESIAN_POINT('Ctrl Pts',(36.9930180634693,-85.1919568824835,109.100870605948));
#38989=CARTESIAN_POINT('Ctrl Pts',(36.052132738323,-85.131447554781,109.153520113679));
#38990=CARTESIAN_POINT('Ctrl Pts',(35.2991816545013,-85.4785795250109,109.20616962141));
#38991=CARTESIAN_POINT('Ctrl Pts',(34.5462305706795,-85.8257114952409,109.258819129141));
#38992=CARTESIAN_POINT('Ctrl Pts',(33.9812137281822,-86.5804847634032,109.311468636872));
#38993=CARTESIAN_POINT('Ctrl Pts',(33.8602729624767,-87.4007343039005,109.364118144603));
#38994=CARTESIAN_POINT('Ctrl Pts',(33.8424333222492,-87.5217270610896,109.371884328904));
#38995=CARTESIAN_POINT('Ctrl Pts',(33.8342560624626,-87.6441444765438,109.379650513206));
#38996=CARTESIAN_POINT('Ctrl Pts',(33.8352710252958,-87.7666978305704,109.387416697508));
#38997=CARTESIAN_POINT('Origin',(36.3549260746835,-87.7685555885722,114.));
#38998=CARTESIAN_POINT('',(33.8413419169939,-87.7682702011519,110.387416697508));
#38999=CARTESIAN_POINT('',(33.838790157295,-87.7706792333693,110.112583302492));
#39000=CARTESIAN_POINT('',(33.8374260746835,-87.7685555885722,114.));
#39001=CARTESIAN_POINT('Ctrl Pts',(33.838790157295,-87.7706792333693,110.112583302492));
#39002=CARTESIAN_POINT('Ctrl Pts',(33.8435896215492,-87.1817422166418,110.07539618188));
#39003=CARTESIAN_POINT('Ctrl Pts',(34.0501481060936,-86.5897716217229,110.038209061269));
#39004=CARTESIAN_POINT('Ctrl Pts',(34.4278436124566,-86.1422290384201,110.001021940657));
#39005=CARTESIAN_POINT('Ctrl Pts',(34.9625847312916,-85.5085984611698,109.948372432926));
#39006=CARTESIAN_POINT('Ctrl Pts',(35.8403680076269,-85.1644721430316,109.895722925195));
#39007=CARTESIAN_POINT('Ctrl Pts',(36.6632637439612,-85.2658545033766,109.843073417464));
#39008=CARTESIAN_POINT('Ctrl Pts',(37.4861594802956,-85.3672368637215,109.790423909734));
#39009=CARTESIAN_POINT('Ctrl Pts',(38.254167676629,-85.9141279025497,109.737774402003));
#39010=CARTESIAN_POINT('Ctrl Pts',(38.6191234908882,-86.6586029124452,109.685124894272));
#39011=CARTESIAN_POINT('Ctrl Pts',(38.9840793051474,-87.4030779223408,109.632475386541));
#39012=CARTESIAN_POINT('Ctrl Pts',(38.9459827373325,-88.3451369033038,109.57982587881));
#39013=CARTESIAN_POINT('Ctrl Pts',(38.5221042978734,-89.0577116832849,109.527176371079));
#39014=CARTESIAN_POINT('Ctrl Pts',(38.0982258584144,-89.770286463266,109.474526863349));
#39015=CARTESIAN_POINT('Ctrl Pts',(37.2885655473112,-90.2533770422654,109.421877355618));
#39016=CARTESIAN_POINT('Ctrl Pts',(36.460170532168,-90.2879817733584,109.369227847887));
#39017=CARTESIAN_POINT('Ctrl Pts',(35.6317755170249,-90.3225865044515,109.316578340156));
#39018=CARTESIAN_POINT('Ctrl Pts',(34.7846457978417,-89.9087053876382,109.263928832425));
#39019=CARTESIAN_POINT('Ctrl Pts',(34.3028147960749,-89.2339648850153,109.211279324695));
#39020=CARTESIAN_POINT('Ctrl Pts',(34.0017369367378,-88.8123452187986,109.178380650627));
#39021=CARTESIAN_POINT('Ctrl Pts',(33.8432908589959,-88.2888723645746,109.14548197656));
#39022=CARTESIAN_POINT('Ctrl Pts',(33.8403654904393,-87.7670276461582,109.112583302492));
#39023=CARTESIAN_POINT('Ctrl Pts',(33.8352710252958,-87.7666978305704,109.387416697508));
#39024=CARTESIAN_POINT('Ctrl Pts',(33.8411368280303,-88.4749738142835,109.432300020937));
#39025=CARTESIAN_POINT('Ctrl Pts',(34.1540286364703,-89.1877902316456,109.477183344366));
#39026=CARTESIAN_POINT('Ctrl Pts',(34.6831903958788,-89.6563814347206,109.522066667795));
#39027=CARTESIAN_POINT('Ctrl Pts',(35.3039132839001,-90.2060532122112,109.574716175526));
#39028=CARTESIAN_POINT('Ctrl Pts',(36.2222237488564,-90.4196709543603,109.627365683257));
#39029=CARTESIAN_POINT('Ctrl Pts',(37.0218197159702,-90.2003942962398,109.680015190987));
#39030=CARTESIAN_POINT('Ctrl Pts',(37.821415683084,-89.9811176381194,109.732664698718));
#39031=CARTESIAN_POINT('Ctrl Pts',(38.5022971523554,-89.3289465797295,109.785314206449));
#39032=CARTESIAN_POINT('Ctrl Pts',(38.7557968588963,-88.5395329577955,109.83796371418));
#39033=CARTESIAN_POINT('Ctrl Pts',(39.0092965654372,-87.7501193358615,109.890613221911));
#39034=CARTESIAN_POINT('Ctrl Pts',(38.8354145092477,-86.8234631503834,109.943262729642));
#39035=CARTESIAN_POINT('Ctrl Pts',(38.3129774786581,-86.1796498892039,109.995912237372));
#39036=CARTESIAN_POINT('Ctrl Pts',(37.7905404480686,-85.5358366280243,110.048561745103));
#39037=CARTESIAN_POINT('Ctrl Pts',(36.9195484430791,-85.1748662911433,110.101211252834));
#39038=CARTESIAN_POINT('Ctrl Pts',(36.0948524429973,-85.2603792927236,110.153860760565));
#39039=CARTESIAN_POINT('Ctrl Pts',(35.2701564429156,-85.3458922943038,110.206510268296));
#39040=CARTESIAN_POINT('Ctrl Pts',(34.4917564477417,-85.8778886343454,110.259159776027));
#39041=CARTESIAN_POINT('Ctrl Pts',(34.1125282588601,-86.6151958615018,110.311809283757));
#39042=CARTESIAN_POINT('Ctrl Pts',(33.9309978336103,-86.9681329542853,110.337011755008));
#39043=CARTESIAN_POINT('Ctrl Pts',(33.8409329447111,-87.3681146281553,110.362214226258));
#39044=CARTESIAN_POINT('Ctrl Pts',(33.8413419169939,-87.7682702011519,110.387416697508));
#39045=CARTESIAN_POINT('Origin',(36.3549260746835,-87.7685555885722,114.));
#39046=CARTESIAN_POINT('',(33.8362792303601,-87.7706817999754,111.387416697508));
#39047=CARTESIAN_POINT('',(33.833460463321,-87.7679946641417,111.112583302492));
#39048=CARTESIAN_POINT('',(33.8374260746835,-87.7685555885722,114.));
#39049=CARTESIAN_POINT('Ctrl Pts',(33.833460463321,-87.7679946641417,111.112583302492));
#39050=CARTESIAN_POINT('Ctrl Pts',(33.8333657394917,-87.7369047176017,111.110609402663));
#39051=CARTESIAN_POINT('Ctrl Pts',(33.8338915410514,-87.7058180485741,111.108635502833));
#39052=CARTESIAN_POINT('Ctrl Pts',(33.8350478473288,-87.6747548496521,111.106661603004));
#39053=CARTESIAN_POINT('Ctrl Pts',(33.8658898157962,-86.846211218651,111.054012095273));
#39054=CARTESIAN_POINT('Ctrl Pts',(34.3452981965331,-86.034365164692,111.001362587543));
#39055=CARTESIAN_POINT('Ctrl Pts',(35.0559404903895,-85.6072547508361,110.948713079812));
#39056=CARTESIAN_POINT('Ctrl Pts',(35.7665827842458,-85.1801443369802,110.896063572081));
#39057=CARTESIAN_POINT('Ctrl Pts',(36.7084589912216,-85.1377695632274,110.84341406435));
#39058=CARTESIAN_POINT('Ctrl Pts',(37.4545838558529,-85.4993403886895,110.790764556619));
#39059=CARTESIAN_POINT('Ctrl Pts',(38.2007087204842,-85.8609112141515,110.738115048888));
#39060=CARTESIAN_POINT('Ctrl Pts',(38.7510822427711,-86.6264276388286,110.685465541158));
#39061=CARTESIAN_POINT('Ctrl Pts',(38.8562009557426,-87.4488544330359,110.632816033427));
#39062=CARTESIAN_POINT('Ctrl Pts',(38.9613196687142,-88.2712812272431,110.580166525696));
#39063=CARTESIAN_POINT('Ctrl Pts',(38.6211835723705,-89.1506183909805,110.527517017965));
#39064=CARTESIAN_POINT('Ctrl Pts',(37.9899881937451,-89.6882317922063,110.474867510234));
#39065=CARTESIAN_POINT('Ctrl Pts',(37.3587928151197,-90.2258451934322,110.422218002503));
#39066=CARTESIAN_POINT('Ctrl Pts',(36.4365381542126,-90.4217348321464,110.369568494773));
#39067=CARTESIAN_POINT('Ctrl Pts',(35.6413143367002,-90.1870971210926,110.316918987042));
#39068=CARTESIAN_POINT('Ctrl Pts',(34.8460905191878,-89.9524594100387,110.264269479311));
#39069=CARTESIAN_POINT('Ctrl Pts',(34.17789754507,-89.2872943492169,110.21161997158));
#39070=CARTESIAN_POINT('Ctrl Pts',(33.9396505386785,-88.4931444006248,110.158970463849));
#39071=CARTESIAN_POINT('Ctrl Pts',(33.8696808922075,-88.2599142249784,110.14350807673));
#39072=CARTESIAN_POINT('Ctrl Pts',(33.8367945423336,-88.0155589656965,110.128045689611));
#39073=CARTESIAN_POINT('Ctrl Pts',(33.838790157295,-87.7706792333693,110.112583302492));
#39074=CARTESIAN_POINT('Ctrl Pts',(33.8413419169939,-87.7682702011519,110.387416697508));
#39075=CARTESIAN_POINT('Ctrl Pts',(33.8417873128861,-88.2040641556771,110.414863733989));
#39076=CARTESIAN_POINT('Ctrl Pts',(33.9495396432895,-88.6400643640522,110.442310770469));
#39077=CARTESIAN_POINT('Ctrl Pts',(34.1633179751479,-89.0157286166987,110.46975780695));
#39078=CARTESIAN_POINT('Ctrl Pts',(34.5733922629067,-89.7363360304679,110.522407314681));
#39079=CARTESIAN_POINT('Ctrl Pts',(35.3735972210135,-90.2349327437351,110.575056822411));
#39080=CARTESIAN_POINT('Ctrl Pts',(36.2011721004088,-90.2854875184755,110.627706330142));
#39081=CARTESIAN_POINT('Ctrl Pts',(37.028746979804,-90.336042293216,110.680355837873));
#39082=CARTESIAN_POINT('Ctrl Pts',(37.8836917804877,-89.9385551294297,110.733005345604));
#39083=CARTESIAN_POINT('Ctrl Pts',(38.3784302779913,-89.2732207883705,110.785654853335));
#39084=CARTESIAN_POINT('Ctrl Pts',(38.873168775495,-88.6078864473114,110.838304361066));
#39085=CARTESIAN_POINT('Ctrl Pts',(39.0077009698187,-87.6747049289793,110.890953868796));
#39086=CARTESIAN_POINT('Ctrl Pts',(38.7210387365027,-86.8967198839624,110.943603376527));
#39087=CARTESIAN_POINT('Ctrl Pts',(38.4343765031867,-86.1187348389456,110.996252884258));
#39088=CARTESIAN_POINT('Ctrl Pts',(37.7265198422309,-85.495946267244,111.048902391989));
#39089=CARTESIAN_POINT('Ctrl Pts',(36.9183648066211,-85.3106858972247,111.10155189972));
#39090=CARTESIAN_POINT('Ctrl Pts',(36.1102097710112,-85.1254255272055,111.154201407451));
#39091=CARTESIAN_POINT('Ctrl Pts',(35.2017563607472,-85.3776933588685,111.206850915181));
#39092=CARTESIAN_POINT('Ctrl Pts',(34.6048381146989,-85.9531276069116,111.259500422912));
#39093=CARTESIAN_POINT('Ctrl Pts',(34.1214175880013,-86.419149091613,111.302139181111));
#39094=CARTESIAN_POINT('Ctrl Pts',(33.8423248995646,-87.0971270513523,111.344777939309));
#39095=CARTESIAN_POINT('Ctrl Pts',(33.8362792303601,-87.7706817999754,111.387416697508));
#39096=CARTESIAN_POINT('Origin',(36.3549260746835,-87.7685555885722,114.));
#39097=CARTESIAN_POINT('',(33.8351270426488,-87.7667516913842,112.387416697508));
#39098=CARTESIAN_POINT('',(33.8402625727925,-87.7669648534793,112.112583302492));
#39099=CARTESIAN_POINT('',(33.8374260746835,-87.7685555885722,114.));
#39100=CARTESIAN_POINT('Ctrl Pts',(33.8402625727925,-87.7669648534793,112.112583302492));
#39101=CARTESIAN_POINT('Ctrl Pts',(33.8384608202137,-87.4591086515179,112.093173115714));
#39102=CARTESIAN_POINT('Ctrl Pts',(33.8908470321291,-87.1518442311906,112.073762928937));
#39103=CARTESIAN_POINT('Ctrl Pts',(34.000204726143,-86.8664069145517,112.054352742159));
#39104=CARTESIAN_POINT('Ctrl Pts',(34.2968339560602,-86.0921673680098,112.001703234428));
#39105=CARTESIAN_POINT('Ctrl Pts',(35.0126298328924,-85.478520341233,111.949053726697));
#39106=CARTESIAN_POINT('Ctrl Pts',(35.8230971808513,-85.3036533821964,111.896404218967));
#39107=CARTESIAN_POINT('Ctrl Pts',(36.6335645288102,-85.1287864231598,111.843754711236));
#39108=CARTESIAN_POINT('Ctrl Pts',(37.5387033478958,-85.3926995318635,111.791105203505));
#39109=CARTESIAN_POINT('Ctrl Pts',(38.1281827187525,-85.9757517137513,111.738455695774));
#39110=CARTESIAN_POINT('Ctrl Pts',(38.7176620896091,-86.5588038956392,111.685806188043));
#39111=CARTESIAN_POINT('Ctrl Pts',(38.9914820122369,-87.4609951507114,111.633156680312));
#39112=CARTESIAN_POINT('Ctrl Pts',(38.8255103886397,-88.2733307929391,111.580507172582));
#39113=CARTESIAN_POINT('Ctrl Pts',(38.6595387650426,-89.0856664351667,111.527857664851));
#39114=CARTESIAN_POINT('Ctrl Pts',(38.0537755952206,-89.8081464645499,111.47520815712));
#39115=CARTESIAN_POINT('Ctrl Pts',(37.2828344004873,-90.113245546376,111.422558649389));
#39116=CARTESIAN_POINT('Ctrl Pts',(36.5118932057541,-90.4183446282021,111.369909141658));
#39117=CARTESIAN_POINT('Ctrl Pts',(35.5757739861097,-90.306062762471,111.317259633927));
#39118=CARTESIAN_POINT('Ctrl Pts',(34.8988521543865,-89.8273012255838,111.264610126197));
#39119=CARTESIAN_POINT('Ctrl Pts',(34.2473090193628,-89.3664890932904,111.213934518295));
#39120=CARTESIAN_POINT('Ctrl Pts',(33.8358922927207,-88.5661617834507,111.163258910394));
#39121=CARTESIAN_POINT('Ctrl Pts',(33.833460463321,-87.7679946641417,111.112583302492));
#39122=CARTESIAN_POINT('Ctrl Pts',(33.8362792303601,-87.7706817999754,111.387416697508));
#39123=CARTESIAN_POINT('Ctrl Pts',(33.8348598250416,-87.9288193295271,111.39742744704));
#39124=CARTESIAN_POINT('Ctrl Pts',(33.8484912873127,-88.086713043325,111.407438196572));
#39125=CARTESIAN_POINT('Ctrl Pts',(33.878062949579,-88.2415626538203,111.417448946105));
#39126=CARTESIAN_POINT('Ctrl Pts',(34.0335891123402,-89.0559627882629,111.470098453835));
#39127=CARTESIAN_POINT('Ctrl Pts',(34.6300245196953,-89.7861623927248,111.522747961566));
#39128=CARTESIAN_POINT('Ctrl Pts',(35.396984249603,-90.10113658053,111.575397469297));
#39129=CARTESIAN_POINT('Ctrl Pts',(36.1639439795107,-90.4161107683353,111.628046977028));
#39130=CARTESIAN_POINT('Ctrl Pts',(37.1014280319711,-90.3158595394838,111.680696484759));
#39131=CARTESIAN_POINT('Ctrl Pts',(37.7844422679447,-89.8458302640747,111.733345992489));
#39132=CARTESIAN_POINT('Ctrl Pts',(38.4674565039183,-89.3758009886656,111.78599550022));
#39133=CARTESIAN_POINT('Ctrl Pts',(38.8960009234051,-88.5359936666988,111.838645007951));
#39134=CARTESIAN_POINT('Ctrl Pts',(38.8758014306258,-87.7071221767951,111.891294515682));
#39135=CARTESIAN_POINT('Ctrl Pts',(38.8556019378465,-86.8782506868913,111.943944023413));
#39136=CARTESIAN_POINT('Ctrl Pts',(38.3866585328012,-86.0603150290506,111.996593531144));
#39137=CARTESIAN_POINT('Ctrl Pts',(37.6815595770325,-85.6241138955609,112.049243038874));
#39138=CARTESIAN_POINT('Ctrl Pts',(36.9764606212637,-85.1879127620711,112.101892546605));
#39139=CARTESIAN_POINT('Ctrl Pts',(36.0352061147715,-85.1334461529325,112.154542054336));
#39140=CARTESIAN_POINT('Ctrl Pts',(35.2844994745933,-85.4854056771343,112.207191562067));
#39141=CARTESIAN_POINT('Ctrl Pts',(34.5337928344152,-85.8373652013361,112.259841069798));
#39142=CARTESIAN_POINT('Ctrl Pts',(33.973634060551,-86.5957508588782,112.312490577529));
#39143=CARTESIAN_POINT('Ctrl Pts',(33.8579626149027,-87.4167600445428,112.365140085259));
#39144=CARTESIAN_POINT('Ctrl Pts',(33.8416486419014,-87.5325528541995,112.372565622676));
#39145=CARTESIAN_POINT('Ctrl Pts',(33.8341761808045,-87.6495913386691,112.379991160092));
#39146=CARTESIAN_POINT('Ctrl Pts',(33.8351270426488,-87.7667516913842,112.387416697508));
#39147=CARTESIAN_POINT('Origin',(36.3549260746835,-87.7685555885722,114.));
#39148=CARTESIAN_POINT('',(33.8413207210893,-87.7681842623864,113.387416697508));
#39149=CARTESIAN_POINT('',(33.8389343942797,-87.7706492050004,113.112583302492));
#39150=CARTESIAN_POINT('',(33.8374260746835,-87.7685555885722,114.));
#39151=CARTESIAN_POINT('Ctrl Pts',(33.8389343942797,-87.7706492050004,113.112583302492));
#39152=CARTESIAN_POINT('Ctrl Pts',(33.8436024808034,-87.1870222434737,113.075736828766));
#39153=CARTESIAN_POINT('Ctrl Pts',(34.0460600744816,-86.6004731251508,113.03889035504));
#39154=CARTESIAN_POINT('Ctrl Pts',(34.4174406984265,-86.1546363600791,113.002043881314));
#39155=CARTESIAN_POINT('Ctrl Pts',(34.9481022530933,-85.5175852711787,112.949394373583));
#39156=CARTESIAN_POINT('Ctrl Pts',(35.8236578008925,-85.1678297944825,112.896744865852));
#39157=CARTESIAN_POINT('Ctrl Pts',(36.6471875486386,-85.2639262566846,112.844095358121));
#39158=CARTESIAN_POINT('Ctrl Pts',(37.4707172963847,-85.3600227188868,112.791445850391));
#39159=CARTESIAN_POINT('Ctrl Pts',(38.2422212440775,-85.9019711199873,112.73879634266));
#39160=CARTESIAN_POINT('Ctrl Pts',(38.6119498091466,-86.644087393655,112.686146834929));
#39161=CARTESIAN_POINT('Ctrl Pts',(38.9816783742156,-87.3862036673227,112.633497327198));
#39162=CARTESIAN_POINT('Ctrl Pts',(38.9496315566609,-88.3284878135576,112.580847819467));
#39163=CARTESIAN_POINT('Ctrl Pts',(38.5303372938909,-89.0437696438026,112.528198311736));
#39164=CARTESIAN_POINT('Ctrl Pts',(38.1110430311208,-89.7590514740476,112.475548804006));
#39165=CARTESIAN_POINT('Ctrl Pts',(37.3045013231354,-90.2473309883026,112.422899296275));
#39166=CARTESIAN_POINT('Ctrl Pts',(36.4763455883213,-90.2872540939552,112.370249788544));
#39167=CARTESIAN_POINT('Ctrl Pts',(35.6481898535072,-90.3271771996077,112.317600280813));
#39168=CARTESIAN_POINT('Ctrl Pts',(34.7984200918643,-89.9187438966577,112.264950773082));
#39169=CARTESIAN_POINT('Ctrl Pts',(34.312266502544,-89.2471112120292,112.212301265351));
#39170=CARTESIAN_POINT('Ctrl Pts',(34.0053421667922,-88.8230879812494,112.179061944398));
#39171=CARTESIAN_POINT('Ctrl Pts',(33.8433480161699,-88.2941587038847,112.145822623445));
#39172=CARTESIAN_POINT('Ctrl Pts',(33.8402625727925,-87.7669648534793,112.112583302492));
#39173=CARTESIAN_POINT('Ctrl Pts',(33.8351270426488,-87.7667516913842,112.387416697508));
#39174=CARTESIAN_POINT('Ctrl Pts',(33.8409181046838,-88.4802968553584,112.432640667823));
#39175=CARTESIAN_POINT('Ctrl Pts',(34.1591480267783,-89.1983623702661,112.477864638137));
#39176=CARTESIAN_POINT('Ctrl Pts',(34.6953465824845,-89.667076732345,112.523088608452));
#39177=CARTESIAN_POINT('Ctrl Pts',(35.3195861131473,-90.2127515206959,112.575738116183));
#39178=CARTESIAN_POINT('Ctrl Pts',(36.2392492919054,-90.4204683836109,112.628387623914));
#39179=CARTESIAN_POINT('Ctrl Pts',(37.0374208018146,-90.1960620399989,112.681037131644));
#39180=CARTESIAN_POINT('Ctrl Pts',(37.8355923117237,-89.9716556963869,112.733686639375));
#39181=CARTESIAN_POINT('Ctrl Pts',(38.5122721527838,-89.315126146248,112.786336147106));
#39182=CARTESIAN_POINT('Ctrl Pts',(38.7606978091938,-88.5241010774157,112.838985654837));
#39183=CARTESIAN_POINT('Ctrl Pts',(39.0091234656037,-87.7330760085833,112.891635162568));
#39184=CARTESIAN_POINT('Ctrl Pts',(38.8292949373637,-86.8075554210577,112.944284670298));
#39185=CARTESIAN_POINT('Ctrl Pts',(38.3027347531324,-86.1671099989753,112.996934178029));
#39186=CARTESIAN_POINT('Ctrl Pts',(37.7761745689011,-85.526664576893,113.04958368576));
#39187=CARTESIAN_POINT('Ctrl Pts',(36.9028827286787,-85.171294320254,113.102233193491));
#39188=CARTESIAN_POINT('Ctrl Pts',(36.0787528082445,-85.2621009308566,113.154882701222));
#39189=CARTESIAN_POINT('Ctrl Pts',(35.2546228878104,-85.3529075414593,113.207532208953));
#39190=CARTESIAN_POINT('Ctrl Pts',(34.4796548871646,-85.8898910193036,113.260181716683));
#39191=CARTESIAN_POINT('Ctrl Pts',(34.1051687646067,-86.6296180705161,113.312831224414));
#39192=CARTESIAN_POINT('Ctrl Pts',(33.9283312478418,-86.9789273958571,113.337693048779));
#39193=CARTESIAN_POINT('Ctrl Pts',(33.8407955340496,-87.373445674795,113.362554873143));
#39194=CARTESIAN_POINT('Ctrl Pts',(33.8413207210893,-87.7681842623864,113.387416697508));
#39195=CARTESIAN_POINT('Origin',(36.3549260746835,-87.7685555885722,114.));
#39196=CARTESIAN_POINT('',(33.8364382856638,-87.7707089500853,114.387416697508));
#39197=CARTESIAN_POINT('',(33.8334119429091,-87.7680895937245,114.112583302492));
#39198=CARTESIAN_POINT('',(33.8374260746835,-87.7685555885722,114.));
#39199=CARTESIAN_POINT('Ctrl Pts',(33.8334119429091,-87.7680895937245,114.112583302492));
#39200=CARTESIAN_POINT('Ctrl Pts',(33.8333458553462,-87.7423663400699,114.110950049548));
#39201=CARTESIAN_POINT('Ctrl Pts',(33.8337057988272,-87.7166449805644,114.109316796605));
#39202=CARTESIAN_POINT('Ctrl Pts',(33.8344974997795,-87.6909369173853,114.107683543661));
#39203=CARTESIAN_POINT('Ctrl Pts',(33.8600187551162,-86.8622123304467,114.05503403593));
#39204=CARTESIAN_POINT('Ctrl Pts',(34.3342043907143,-86.0473047321551,114.002384528199));
#39205=CARTESIAN_POINT('Ctrl Pts',(35.0420895595274,-85.6156400900488,113.949735020469));
#39206=CARTESIAN_POINT('Ctrl Pts',(35.7499747283406,-85.1839754479424,113.897085512738));
#39207=CARTESIAN_POINT('Ctrl Pts',(36.6915594303689,-85.1355537620213,113.844436005007));
#39208=CARTESIAN_POINT('Ctrl Pts',(37.4399905594498,-85.4923262672584,113.791786497276));
#39209=CARTESIAN_POINT('Ctrl Pts',(38.1884216885307,-85.8490987724954,113.739136989545));
#39210=CARTESIAN_POINT('Ctrl Pts',(38.7436992446643,-86.6110654688906,113.686487481814));
#39211=CARTESIAN_POINT('Ctrl Pts',(38.8540965917791,-87.4328003417179,113.633837974084));
#39212=CARTESIAN_POINT('Ctrl Pts',(38.964493938894,-88.2545352145452,113.581188466353));
#39213=CARTESIAN_POINT('Ctrl Pts',(38.63001107699,-89.1360382638046,113.528538958622));
#39214=CARTESIAN_POINT('Ctrl Pts',(38.0022807250933,-89.677693486966,113.475889450891));
#39215=CARTESIAN_POINT('Ctrl Pts',(37.3745503731965,-90.2193487101274,113.42323994316));
#39216=CARTESIAN_POINT('Ctrl Pts',(36.453572531307,-90.4211561071909,113.37059043543));
#39217=CARTESIAN_POINT('Ctrl Pts',(35.6568584989078,-90.191629363545,113.317940927699));
#39218=CARTESIAN_POINT('Ctrl Pts',(34.8601444665087,-89.962102619899,113.265291419968));
#39219=CARTESIAN_POINT('Ctrl Pts',(34.1876942435999,-89.3012417355436,113.212641912237));
#39220=CARTESIAN_POINT('Ctrl Pts',(33.9443529129126,-88.5086379428137,113.159992404506));
#39221=CARTESIAN_POINT('Ctrl Pts',(33.8713126986855,-88.2707336350879,113.144189370502));
#39222=CARTESIAN_POINT('Ctrl Pts',(33.8369323049992,-88.0209601787902,113.128386336497));
#39223=CARTESIAN_POINT('Ctrl Pts',(33.8389343942797,-87.7706492050004,113.112583302492));
#39224=CARTESIAN_POINT('Ctrl Pts',(33.8413207210893,-87.7681842623864,113.387416697508));
#39225=CARTESIAN_POINT('Ctrl Pts',(33.8419077146645,-88.2093775844676,113.415204380874));
#39226=CARTESIAN_POINT('Ctrl Pts',(33.9525020875792,-88.6508461203768,113.442992064241));
#39227=CARTESIAN_POINT('Ctrl Pts',(34.17137125074,-89.0297752185784,113.470779747607));
#39228=CARTESIAN_POINT('Ctrl Pts',(34.5860641039011,-89.7477346908476,113.523429255338));
#39229=CARTESIAN_POINT('Ctrl Pts',(35.3894540546931,-90.2411830108054,113.576078763068));
#39230=CARTESIAN_POINT('Ctrl Pts',(36.2173364859249,-90.2864228863751,113.628728270799));
#39231=CARTESIAN_POINT('Ctrl Pts',(37.0452189171568,-90.3316627619448,113.68137777853));
#39232=CARTESIAN_POINT('Ctrl Pts',(37.8975938288284,-89.9286941931264,113.734027286261));
#39233=CARTESIAN_POINT('Ctrl Pts',(38.3880500166391,-89.2601968527262,113.786676793992));
#39234=CARTESIAN_POINT('Ctrl Pts',(38.8785062044498,-88.591699512326,113.839326301722));
#39235=CARTESIAN_POINT('Ctrl Pts',(39.0070436683995,-87.6576734003441,113.891975809453));
#39236=CARTESIAN_POINT('Ctrl Pts',(38.7153919038517,-86.8815450510873,113.944625317184));
#39237=CARTESIAN_POINT('Ctrl Pts',(38.423740139304,-86.1054167018305,113.997274824915));
#39238=CARTESIAN_POINT('Ctrl Pts',(37.7118991462587,-85.4871861152989,114.049924332646));
#39239=CARTESIAN_POINT('Ctrl Pts',(36.9025712140805,-85.3071187265799,114.102573840377));
#39240=CARTESIAN_POINT('Ctrl Pts',(36.0932432819023,-85.1270513378609,114.155223348107));
#39241=CARTESIAN_POINT('Ctrl Pts',(35.1864284105912,-85.3851471469545,114.207872855838));
#39242=CARTESIAN_POINT('Ctrl Pts',(34.5932173322921,-85.9644023436228,114.260522363569));
#39243=CARTESIAN_POINT('Ctrl Pts',(34.1166372216047,-86.4297704323915,114.302820474882));
#39244=CARTESIAN_POINT('Ctrl Pts',(33.8424683523542,-87.1024264168637,114.345118586195));
#39245=CARTESIAN_POINT('Ctrl Pts',(33.8364382856638,-87.7707089500853,114.387416697508));
#39246=CARTESIAN_POINT('Origin',(36.3549260746835,-87.7685555885722,114.));
#39247=CARTESIAN_POINT('',(33.8349862377778,-87.7668088525252,115.387416697508));
#39248=CARTESIAN_POINT('',(33.8401553510245,-87.7669042808192,115.112583302492));
#39249=CARTESIAN_POINT('',(33.8374260746835,-87.7685555885722,114.));
#39250=CARTESIAN_POINT('Ctrl Pts',(33.8401553510245,-87.7669042808192,115.112583302492));
#39251=CARTESIAN_POINT('Ctrl Pts',(33.8383127863372,-87.4644833544989,115.0935137626));
#39252=CARTESIAN_POINT('Ctrl Pts',(33.8888249380179,-87.1626571750687,115.074444222708));
#39253=CARTESIAN_POINT('Ctrl Pts',(33.9944605731161,-86.8815451741916,115.055374682816));
#39254=CARTESIAN_POINT('Ctrl Pts',(34.2861122971867,-86.1054169326509,115.002725175085));
#39255=CARTESIAN_POINT('Ctrl Pts',(34.9979531914383,-85.4871864319215,114.950075667354));
#39256=CARTESIAN_POINT('Ctrl Pts',(35.8072810112928,-85.3071190681936,114.897426159623));
#39257=CARTESIAN_POINT('Ctrl Pts',(36.6166088311474,-85.1270517044657,114.844776651893));
#39258=CARTESIAN_POINT('Ctrl Pts',(37.523423576605,-85.3851474777394,114.792127144162));
#39259=CARTESIAN_POINT('Ctrl Pts',(38.1166345725743,-85.9644025940151,114.739477636431));
#39260=CARTESIAN_POINT('Ctrl Pts',(38.7098455685436,-86.5436577102908,114.6868281287));
#39261=CARTESIAN_POINT('Ctrl Pts',(38.9894528150246,-87.4440721695685,114.634178620969));
#39262=CARTESIAN_POINT('Ctrl Pts',(38.8287006187602,-88.2574567691686,114.581529113239));
#39263=CARTESIAN_POINT('Ctrl Pts',(38.6679484224957,-89.0708413687687,114.528879605508));
#39264=CARTESIAN_POINT('Ctrl Pts',(38.0668367834858,-89.7971961086912,114.476230097777));
#39265=CARTESIAN_POINT('Ctrl Pts',(37.2978705222835,-90.1072391131326,114.423580590046));
#39266=CARTESIAN_POINT('Ctrl Pts',(36.5289042610813,-90.4172821175741,114.370931082315));
#39267=CARTESIAN_POINT('Ctrl Pts',(35.5920833776866,-90.3110133865345,114.318281574584));
#39268=CARTESIAN_POINT('Ctrl Pts',(34.912101373527,-89.8366082332219,114.265632066854));
#39269=CARTESIAN_POINT('Ctrl Pts',(34.25321325339,-89.3769197153828,114.214615812066));
#39270=CARTESIAN_POINT('Ctrl Pts',(33.835476252641,-88.5715806068579,114.163599557279));
#39271=CARTESIAN_POINT('Ctrl Pts',(33.8334119429091,-87.7680895937245,114.112583302492));
#39272=CARTESIAN_POINT('Ctrl Pts',(33.8364382856638,-87.7707089500853,114.387416697508));
#39273=CARTESIAN_POINT('Ctrl Pts',(33.834962578858,-87.9342542528365,114.397768093926));
#39274=CARTESIAN_POINT('Ctrl Pts',(33.8495457647187,-88.0975376286172,114.408119490344));
#39275=CARTESIAN_POINT('Ctrl Pts',(33.8811511872807,-88.2574568370208,114.418470886762));
#39276=CARTESIAN_POINT('Ctrl Pts',(34.0419034058551,-89.0708415495077,114.471120394492));
#39277=CARTESIAN_POINT('Ctrl Pts',(34.6430151282909,-89.7971963902384,114.523769902223));
#39278=CARTESIAN_POINT('Ctrl Pts',(35.4119814962151,-90.1072394377098,114.576419409954));
#39279=CARTESIAN_POINT('Ctrl Pts',(36.1809478641394,-90.4172824851811,114.629068917685));
#39280=CARTESIAN_POINT('Ctrl Pts',(37.117768877552,-90.3110137393931,114.681718425416));
#39281=CARTESIAN_POINT('Ctrl Pts',(37.797750976084,-89.8366085202398,114.734367933147));
#39282=CARTESIAN_POINT('Ctrl Pts',(38.477733074616,-89.3622033010865,114.787017440877));
#39283=CARTESIAN_POINT('Ctrl Pts',(38.9008762582673,-88.5196616085678,114.839666948608));
#39284=CARTESIAN_POINT('Ctrl Pts',(38.8753549993888,-87.6909369066135,114.892316456339));
#39285=CARTESIAN_POINT('Ctrl Pts',(38.8498337405103,-86.8622122046593,114.94496596407));
#39286=CARTESIAN_POINT('Ctrl Pts',(38.3756480391019,-86.0473044932694,114.997615471801));
#39287=CARTESIAN_POINT('Ctrl Pts',(37.667762772044,-85.6156397912537,115.050264979531));
#39288=CARTESIAN_POINT('Ctrl Pts',(36.9598775049861,-85.183975089238,115.102914487262));
#39289=CARTESIAN_POINT('Ctrl Pts',(36.0182926722788,-85.1355533965965,115.155563994993));
#39290=CARTESIAN_POINT('Ctrl Pts',(35.2698614393257,-85.4923259513485,115.208213502724));
#39291=CARTESIAN_POINT('Ctrl Pts',(34.5214302063727,-85.8490985061005,115.260863010455));
#39292=CARTESIAN_POINT('Ctrl Pts',(33.9661525731739,-86.6110653082461,115.313512518185));
#39293=CARTESIAN_POINT('Ctrl Pts',(33.8557552107373,-87.432800295119,115.366162025916));
#39294=CARTESIAN_POINT('Ctrl Pts',(33.8408993600097,-87.5433787730203,115.373246916447));
#39295=CARTESIAN_POINT('Ctrl Pts',(33.8340995342799,-87.6550395510862,115.380331806977));
#39296=CARTESIAN_POINT('Ctrl Pts',(33.8349862377778,-87.7668088525252,115.387416697508));
#39297=CARTESIAN_POINT('Origin',(36.3549260746835,-87.7685555885722,114.));
#39298=CARTESIAN_POINT('',(33.8412939819271,-87.7680988643367,116.387416697508));
#39299=CARTESIAN_POINT('',(33.8390759225476,-87.7706159289776,116.112583302492));
#39300=CARTESIAN_POINT('',(33.8374260746835,-87.7685555885722,114.));
#39301=CARTESIAN_POINT('Ctrl Pts',(33.8390759225476,-87.7706159289776,116.112583302492));
#39302=CARTESIAN_POINT('Ctrl Pts',(33.8436084809604,-87.1923022245829,116.076077475652));
#39303=CARTESIAN_POINT('Ctrl Pts',(34.0420143053501,-86.6111786929465,116.039571648811));
#39304=CARTESIAN_POINT('Ctrl Pts',(34.4071176665644,-86.1671102212336,116.003065821971));
#39305=CARTESIAN_POINT('Ctrl Pts',(34.9336777777165,-85.5266648880365,115.95041631424));
#39306=CARTESIAN_POINT('Ctrl Pts',(35.8069694967381,-85.1712946807182,115.897766806509));
#39307=CARTESIAN_POINT('Ctrl Pts',(36.6310993027942,-85.2621012787183,115.845117298778));
#39308=CARTESIAN_POINT('Ctrl Pts',(37.4552291088503,-85.3529078767185,115.792467791047));
#39309=CARTESIAN_POINT('Ctrl Pts',(38.2301970019409,-85.8898912800372,115.739818283317));
#39310=CARTESIAN_POINT('Ctrl Pts',(38.6046830725251,-86.6296182285857,115.687168775586));
#39311=CARTESIAN_POINT('Ctrl Pts',(38.9791691431092,-87.3693451771342,115.634519267855));
#39312=CARTESIAN_POINT('Ctrl Pts',(38.9531733911867,-88.3118156709127,115.581869760124));
#39313=CARTESIAN_POINT('Ctrl Pts',(38.5384805955792,-89.0297750435388,115.529220252393));
#39314=CARTESIAN_POINT('Ctrl Pts',(38.1237877999717,-89.7477344161649,115.476570744663));
#39315=CARTESIAN_POINT('Ctrl Pts',(37.3203979606791,-90.2411826676387,115.423921236932));
#39316=CARTESIAN_POINT('Ctrl Pts',(36.492515644346,-90.2864225369295,115.371271729201));
#39317=CARTESIAN_POINT('Ctrl Pts',(35.6646333280129,-90.3316624062204,115.31862222147));
#39318=CARTESIAN_POINT('Ctrl Pts',(34.8122585346393,-89.9286938933283,115.265972713739));
#39319=CARTESIAN_POINT('Ctrl Pts',(34.3218024148975,-89.2601966457063,115.213323206008));
#39320=CARTESIAN_POINT('Ctrl Pts',(34.0089884601789,-88.8338276815323,115.17974323817));
#39321=CARTESIAN_POINT('Ctrl Pts',(33.8433999632852,-88.2994438720784,115.146163270331));
#39322=CARTESIAN_POINT('Ctrl Pts',(33.8401553510245,-87.7669042808192,115.112583302492));
#39323=CARTESIAN_POINT('Ctrl Pts',(33.8349862377778,-87.7668088525252,115.387416697508));
#39324=CARTESIAN_POINT('Ctrl Pts',(33.8406888390072,-88.4856238310819,115.432981314708));
#39325=CARTESIAN_POINT('Ctrl Pts',(34.1643126089722,-89.2089274255769,115.478545931909));
#39326=CARTESIAN_POINT('Ctrl Pts',(34.707571195643,-89.6776937519279,115.524110549109));
#39327=CARTESIAN_POINT('Ctrl Pts',(35.33530163466,-90.2193490502639,115.57676005684));
#39328=CARTESIAN_POINT('Ctrl Pts',(36.2562796043687,-90.4211564753357,115.62940956457));
#39329=CARTESIAN_POINT('Ctrl Pts',(37.0529937473409,-90.1916296998348,115.682059072301));
#39330=CARTESIAN_POINT('Ctrl Pts',(37.8497078903132,-89.9621029243338,115.734708580032));
#39331=CARTESIAN_POINT('Ctrl Pts',(38.5221582065491,-89.3012419482601,115.787358087763));
#39332=CARTESIAN_POINT('Ctrl Pts',(38.765499571009,-88.5086380455277,115.840007595494));
#39333=CARTESIAN_POINT('Ctrl Pts',(39.0088409354689,-87.7160341427952,115.892657103225));
#39334=CARTESIAN_POINT('Ctrl Pts',(38.8230733481528,-86.791687313404,115.945306610955));
#39335=CARTESIAN_POINT('Ctrl Pts',(38.2924117198376,-86.1546361360895,115.997956118686));
#39336=CARTESIAN_POINT('Ctrl Pts',(37.7617500915224,-85.5175849587751,116.050605626417));
#39337=CARTESIAN_POINT('Ctrl Pts',(36.886194422208,-85.1678294335373,116.103255134148));
#39338=CARTESIAN_POINT('Ctrl Pts',(36.0626645601672,-85.2639259090762,116.155904641879));
#39339=CARTESIAN_POINT('Ctrl Pts',(35.2391346981264,-85.360022384615,116.208554149609));
#39340=CARTESIAN_POINT('Ctrl Pts',(34.4676306433592,-85.9019708609303,116.26120365734));
#39341=CARTESIAN_POINT('Ctrl Pts',(34.0979020269767,-86.6440872375935,116.313853165071));
#39342=CARTESIAN_POINT('Ctrl Pts',(33.9257032465489,-86.9897232780147,116.33837434255));
#39343=CARTESIAN_POINT('Ctrl Pts',(33.8406564735888,-87.3787791810735,116.362895520029));
#39344=CARTESIAN_POINT('Ctrl Pts',(33.8412939819271,-87.7680988643367,116.387416697508));
#39345=CARTESIAN_POINT('Origin',(36.3549260746835,-87.7685555885722,114.));
#39346=CARTESIAN_POINT('',(33.8365981762608,-87.7707324390162,117.387416697508));
#39347=CARTESIAN_POINT('',(33.8333718846759,-87.7681855672794,117.112583302492));
#39348=CARTESIAN_POINT('',(33.8374260746835,-87.7685555885722,114.));
#39349=CARTESIAN_POINT('Ctrl Pts',(33.8333718846759,-87.7681855672794,117.112583302492));
#39350=CARTESIAN_POINT('Ctrl Pts',(33.8333297115333,-87.7478282709333,117.111290696434));
#39351=CARTESIAN_POINT('Ctrl Pts',(33.8335551478591,-87.7274719322915,117.109998090376));
#39352=CARTESIAN_POINT('Ctrl Pts',(33.8340510686044,-87.7071221853206,117.108705484318));
#39353=CARTESIAN_POINT('Ctrl Pts',(33.8542505585804,-86.8782508104529,117.056055976587));
#39354=CARTESIAN_POINT('Ctrl Pts',(34.323193898543,-86.0603152661305,117.003406468856));
#39355=CARTESIAN_POINT('Ctrl Pts',(35.0282927564538,-85.6241141931798,116.950756961126));
#39356=CARTESIAN_POINT('Ctrl Pts',(35.7333916143645,-85.187913120229,116.898107453395));
#39357=CARTESIAN_POINT('Ctrl Pts',(36.6746459902234,-85.1334465186498,116.845457945664));
#39358=CARTESIAN_POINT('Ctrl Pts',(37.4253525262137,-85.4854059940045,116.792808437933));
#39359=CARTESIAN_POINT('Ctrl Pts',(38.1760590622039,-85.8373654693593,116.740158930202));
#39360=CARTESIAN_POINT('Ctrl Pts',(38.7362177583255,-86.5957510216481,116.687509422471));
#39361=CARTESIAN_POINT('Ctrl Pts',(38.8518891879201,-87.4167600933678,116.634859914741));
#39362=CARTESIAN_POINT('Ctrl Pts',(38.9675606175146,-88.2377691650875,116.58221040701));
#39363=CARTESIAN_POINT('Ctrl Pts',(38.6387447805821,-89.121401756238,116.529560899279));
#39364=CARTESIAN_POINT('Ctrl Pts',(38.0145053365551,-89.6670764688566,116.476911391548));
#39365=CARTESIAN_POINT('Ctrl Pts',(37.3902658925281,-90.2127511814751,116.424261883817));
#39366=CARTESIAN_POINT('Ctrl Pts',(36.4706028414066,-90.4204680155617,116.371612376086));
#39367=CARTESIAN_POINT('Ctrl Pts',(35.6724314422729,-90.196061703094,116.318962868356));
#39368=CARTESIAN_POINT('Ctrl Pts',(34.8742600431391,-89.9716553906263,116.266313360625));
#39369=CARTESIAN_POINT('Ctrl Pts',(34.1975802959931,-89.3151259316045,116.213663852894));
#39370=CARTESIAN_POINT('Ctrl Pts',(33.9491546740614,-88.5241009725556,116.161014345163));
#39371=CARTESIAN_POINT('Ctrl Pts',(33.8729810470265,-88.2815525601278,116.144870664273));
#39372=CARTESIAN_POINT('Ctrl Pts',(33.8370715253604,-88.0263589899167,116.128726983382));
#39373=CARTESIAN_POINT('Ctrl Pts',(33.8390759225476,-87.7706159289776,116.112583302492));
#39374=CARTESIAN_POINT('Ctrl Pts',(33.8412939819271,-87.7680988643367,116.387416697508));
#39375=CARTESIAN_POINT('Ctrl Pts',(33.8420252700186,-88.2146888632784,116.41554502776));
#39376=CARTESIAN_POINT('Ctrl Pts',(33.9555039285579,-88.6616259565057,116.443673358012));
#39377=CARTESIAN_POINT('Ctrl Pts',(34.1795145535585,-89.0437698207844,116.471801688264));
#39378=CARTESIAN_POINT('Ctrl Pts',(34.5988088745207,-89.7590517503008,116.524451195994));
#39379=CARTESIAN_POINT('Ctrl Pts',(35.405350694443,-90.2473313323226,116.577100703725));
#39380=CARTESIAN_POINT('Ctrl Pts',(36.2335065441938,-90.2872544435161,116.629750211456));
#39381=CARTESIAN_POINT('Ctrl Pts',(37.0616623939446,-90.3271775547097,116.682399719187));
#39382=CARTESIAN_POINT('Ctrl Pts',(37.9114322735241,-89.918744195075,116.735049226918));
#39383=CARTESIAN_POINT('Ctrl Pts',(38.3975859303161,-89.2471114172331,116.787698734649));
#39384=CARTESIAN_POINT('Ctrl Pts',(38.8837395871081,-88.5754786393912,116.840348242379));
#39385=CARTESIAN_POINT('Ctrl Pts',(39.0062770211127,-87.6406464433422,116.89299775011));
#39386=CARTESIAN_POINT('Ctrl Pts',(38.7096477500276,-86.8664067893463,116.945647257841));
#39387=CARTESIAN_POINT('Ctrl Pts',(38.4130184789425,-86.0921671353504,116.998296765572));
#39388=CARTESIAN_POINT('Ctrl Pts',(37.6972225027677,-85.4785200234076,117.050946273303));
#39389=CARTESIAN_POINT('Ctrl Pts',(36.886755042327,-85.3036530401017,117.103595781034));
#39390=CARTESIAN_POINT('Ctrl Pts',(36.0762875818863,-85.1287860567958,117.156245288764));
#39391=CARTESIAN_POINT('Ctrl Pts',(35.1711486371797,-85.3926992021267,117.208894796495));
#39392=CARTESIAN_POINT('Ctrl Pts',(34.5816691845112,-85.9757514649342,117.261544304226));
#39393=CARTESIAN_POINT('Ctrl Pts',(34.111901009423,-86.4403976815922,117.303501768653));
#39394=CARTESIAN_POINT('Ctrl Pts',(33.8426025126824,-87.107723424266,117.345459233081));
#39395=CARTESIAN_POINT('Ctrl Pts',(33.8365981762608,-87.7707324390162,117.387416697508));
#39396=CARTESIAN_POINT('Origin',(36.3549260746835,-87.7685555885722,114.));
#39397=CARTESIAN_POINT('',(33.8348489078967,-87.7668692328515,118.387416697508));
#39398=CARTESIAN_POINT('',(33.8400439227885,-87.7668461827817,118.112583302492));
#39399=CARTESIAN_POINT('',(33.8374260746835,-87.7685555885722,114.));
#39400=CARTESIAN_POINT('Ctrl Pts',(33.8400439227885,-87.7668461827817,118.112583302492));
#39401=CARTESIAN_POINT('Ctrl Pts',(33.8381652118261,-87.4698606386811,118.093854409486));
#39402=CARTESIAN_POINT('Ctrl Pts',(33.8868400327939,-87.1734708669246,118.075125516479));
#39403=CARTESIAN_POINT('Ctrl Pts',(33.9888137412488,-86.8967200049607,118.056396623473));
#39404=CARTESIAN_POINT('Ctrl Pts',(34.2754759347802,-86.1187350679177,118.003747115742));
#39405=CARTESIAN_POINT('Ctrl Pts',(34.9833324974952,-85.4959465826508,117.951097608011));
#39406=CARTESIAN_POINT('Ctrl Pts',(35.7914874209442,-85.3106862383434,117.89844810028));
#39407=CARTESIAN_POINT('Ctrl Pts',(36.5996423443932,-85.1254258940359,117.845798592549));
#39408=CARTESIAN_POINT('Ctrl Pts',(37.5080956285762,-85.3776936906878,117.793149084819));
#39409=CARTESIAN_POINT('Ctrl Pts',(38.1050137917803,-85.9531278588686,117.740499577088));
#39410=CARTESIAN_POINT('Ctrl Pts',(38.7019319549844,-86.5285620270495,117.687850069357));
#39411=CARTESIAN_POINT('Ctrl Pts',(38.9873149972096,-87.4271625667592,117.635200561626));
#39412=CARTESIAN_POINT('Ctrl Pts',(38.8317888560331,-88.241562588174,117.582551053895));
#39413=CARTESIAN_POINT('Ctrl Pts',(38.6762627148567,-89.0559626095889,117.529901546165));
#39414=CARTESIAN_POINT('Ctrl Pts',(38.0798273902785,-89.7861621127089,117.477252038434));
#39415=CARTESIAN_POINT('Ctrl Pts',(37.3128677668143,-90.1011362567998,117.424602530703));
#39416=CARTESIAN_POINT('Ctrl Pts',(36.54590814335,-90.4161104008908,117.371953022972));
#39417=CARTESIAN_POINT('Ctrl Pts',(35.6084242209996,-90.3158591859526,117.319303515241));
#39418=CARTESIAN_POINT('Ctrl Pts',(34.9254100798192,-89.845829975777,117.26665400751));
#39419=CARTESIAN_POINT('Ctrl Pts',(34.2591647225201,-89.3873405241043,117.215297105838));
#39420=CARTESIAN_POINT('Ctrl Pts',(33.8350474778894,-88.5770071415669,117.163940204165));
#39421=CARTESIAN_POINT('Ctrl Pts',(33.8333718846759,-87.7681855672794,117.112583302492));
#39422=CARTESIAN_POINT('Ctrl Pts',(33.8365981762608,-87.7707324390162,117.387416697508));
#39423=CARTESIAN_POINT('Ctrl Pts',(33.8350680879701,-87.9396873840551,117.398108740812));
#39424=CARTESIAN_POINT('Ctrl Pts',(33.8506359548791,-88.108362006809,117.408800784115));
#39425=CARTESIAN_POINT('Ctrl Pts',(33.8843414178438,-88.2733308629943,117.419492827418));
#39426=CARTESIAN_POINT('Ctrl Pts',(34.0503130644754,-89.0856666179632,117.472142335149));
#39427=CARTESIAN_POINT('Ctrl Pts',(34.6560763183689,-89.8081467476169,117.52479184288));
#39428=CARTESIAN_POINT('Ctrl Pts',(35.4270176200981,-90.1132458717868,117.577441350611));
#39429=CARTESIAN_POINT('Ctrl Pts',(36.1979589218274,-90.4183449959567,117.630090858342));
#39430=CARTESIAN_POINT('Ctrl Pts',(37.1340782713924,-90.3060631146427,117.682740366073));
#39431=CARTESIAN_POINT('Ctrl Pts',(37.8110001970633,-89.8273015113101,117.735389873803));
#39432=CARTESIAN_POINT('Ctrl Pts',(38.4879221227341,-89.3485399079774,117.788039381534));
#39433=CARTESIAN_POINT('Ctrl Pts',(38.9056466245108,-88.5032985826261,117.840688889265));
#39434=CARTESIAN_POINT('Ctrl Pts',(38.8748046517631,-87.6747548366344,117.893338396996));
#39435=CARTESIAN_POINT('Ctrl Pts',(38.8439626790154,-86.8462110906427,117.945987904727));
#39436=CARTESIAN_POINT('Ctrl Pts',(38.3645542317434,-86.0343649240108,117.998637412458));
#39437=CARTESIAN_POINT('Ctrl Pts',(37.6539118392597,-85.6072544508775,118.051286920188));
#39438=CARTESIAN_POINT('Ctrl Pts',(36.943269446776,-85.1801439777442,118.103936427919));
#39439=CARTESIAN_POINT('Ctrl Pts',(36.0013931090806,-85.1377691981096,118.15658593565));
#39440=CARTESIAN_POINT('Ctrl Pts',(35.2552681408972,-85.4993400737528,118.209235443381));
#39441=CARTESIAN_POINT('Ctrl Pts',(34.5091431727139,-85.8609109493961,118.261884951112));
#39442=CARTESIAN_POINT('Ctrl Pts',(33.9587695740425,-86.6264274803171,118.314534458842));
#39443=CARTESIAN_POINT('Ctrl Pts',(33.8536508464817,-87.4488543886655,118.367183966573));
#39444=CARTESIAN_POINT('Ctrl Pts',(33.8401854535299,-87.554204802926,118.373928210218));
#39445=CARTESIAN_POINT('Ctrl Pts',(33.8340261763932,-87.6604890504481,118.380672453863));
#39446=CARTESIAN_POINT('Ctrl Pts',(33.8348489078967,-87.7668692328515,118.387416697508));
#39447=CARTESIAN_POINT('Origin',(36.3549260746835,-87.7685555885722,114.));
#39448=CARTESIAN_POINT('',(33.8412617315361,-87.7680141434736,119.387416697508));
#39449=CARTESIAN_POINT('',(33.8392145615825,-87.7705794701237,119.112583302492));
#39450=CARTESIAN_POINT('',(33.8374260746835,-87.7685555885722,114.));
#39451=CARTESIAN_POINT('Ctrl Pts',(33.8392145615825,-87.7705794701237,119.112583302492));
#39452=CARTESIAN_POINT('Ctrl Pts',(33.8436077753976,-87.1975822800088,119.076418122537));
#39453=CARTESIAN_POINT('Ctrl Pts',(34.0380106829751,-86.6218882277961,119.040252942582));
#39454=CARTESIAN_POINT('Ctrl Pts',(34.3968749424612,-86.1796501097232,119.004087762628));
#39455=CARTESIAN_POINT('Ctrl Pts',(34.9193119005448,-85.5358369378978,118.951438254897));
#39456=CARTESIAN_POINT('Ctrl Pts',(35.7903037846505,-85.1748666511118,118.898788747166));
#39457=CARTESIAN_POINT('Ctrl Pts',(36.6149996702752,-85.2603796408235,118.846139239435));
#39458=CARTESIAN_POINT('Ctrl Pts',(37.4396955558998,-85.3458926305352,118.793489731704));
#39459=CARTESIAN_POINT('Ctrl Pts',(38.2180954430434,-85.8778888967446,118.740840223974));
#39460=CARTESIAN_POINT('Ctrl Pts',(38.5973235792934,-86.6151960215733,118.688190716243));
#39461=CARTESIAN_POINT('Ctrl Pts',(38.9765517155434,-87.352503146402,118.635541208512));
#39462=CARTESIAN_POINT('Ctrl Pts',(38.9566081008998,-88.2951211298501,118.582891700781));
#39463=CARTESIAN_POINT('Ctrl Pts',(38.5465338700534,-89.0157284436085,118.53024219305));
#39464=CARTESIAN_POINT('Ctrl Pts',(38.136459639207,-89.736335757367,118.477592685319));
#39465=CARTESIAN_POINT('Ctrl Pts',(37.3362547921579,-90.2349324014359,118.424943177589));
#39466=CARTESIAN_POINT('Ctrl Pts',(36.5086800276188,-90.2854871691599,118.372293669858));
#39467=CARTESIAN_POINT('Ctrl Pts',(35.6811052630797,-90.3360419368839,118.319644162127));
#39468=CARTESIAN_POINT('Ctrl Pts',(34.8261605810507,-89.938554828263,118.266994654396));
#39469=CARTESIAN_POINT('Ctrl Pts',(34.3314221522101,-89.273220579543,118.214345146665));
#39470=CARTESIAN_POINT('Ctrl Pts',(34.0126759310704,-88.8445642124375,118.180424531941));
#39471=CARTESIAN_POINT('Ctrl Pts',(33.8434465280954,-88.3047280648933,118.146503917216));
#39472=CARTESIAN_POINT('Ctrl Pts',(33.8400439227885,-87.7668461827817,118.112583302492));
#39473=CARTESIAN_POINT('Ctrl Pts',(33.8348489078967,-87.7668692328515,118.387416697508));
#39474=CARTESIAN_POINT('Ctrl Pts',(33.8404488993749,-88.4909549307934,118.433321961594));
#39475=CARTESIAN_POINT('Ctrl Pts',(34.1695225039494,-89.2194852526625,118.47922722568));
#39476=CARTESIAN_POINT('Ctrl Pts',(34.7198637286972,-89.6882320586299,118.525132489766));
#39477=CARTESIAN_POINT('Ctrl Pts',(35.3510591949238,-90.2258455344702,118.577781997497));
#39478=CARTESIAN_POINT('Ctrl Pts',(36.2733139838272,-90.4217352003751,118.630431505227));
#39479=CARTESIAN_POINT('Ctrl Pts',(37.0685379117059,-90.1870974567552,118.683081012958));
#39480=CARTESIAN_POINT('Ctrl Pts',(37.8637618395846,-89.9524597131353,118.735730520689));
#39481=CARTESIAN_POINT('Ctrl Pts',(38.5319549064386,-89.2872945599906,118.78838002842));
#39482=CARTESIAN_POINT('Ctrl Pts',(38.7702019458957,-88.4931445011848,118.841029536151));
#39483=CARTESIAN_POINT('Ctrl Pts',(39.0084489853528,-87.698994442379,118.893679043881));
#39484=CARTESIAN_POINT('Ctrl Pts',(38.8167499974131,-86.7758594779121,118.946328551612));
#39485=CARTESIAN_POINT('Ctrl Pts',(38.2820088043637,-86.1422288127157,118.998978059343));
#39486=CARTESIAN_POINT('Ctrl Pts',(37.7472676113142,-85.5085981475193,119.051627567074));
#39487=CARTESIAN_POINT('Ctrl Pts',(36.8694842131551,-85.1644717815935,119.104277074805));
#39488=CARTESIAN_POINT('Ctrl Pts',(36.0465883626135,-85.2658541560218,119.156926582536));
#39489=CARTESIAN_POINT('Ctrl Pts',(35.223692512072,-85.3672365304501,119.209576090266));
#39490=CARTESIAN_POINT('Ctrl Pts',(34.455684209148,-85.9141276452325,119.262225597997));
#39491=CARTESIAN_POINT('Ctrl Pts',(34.090728344239,-86.6586027584256,119.314875105728));
#39492=CARTESIAN_POINT('Ctrl Pts',(33.9231137389559,-87.000520546956,119.339055636321));
#39493=CARTESIAN_POINT('Ctrl Pts',(33.8405158986517,-87.3841151764434,119.363236166915));
#39494=CARTESIAN_POINT('Ctrl Pts',(33.8412617315361,-87.7680141434736,119.387416697508));
#39495=CARTESIAN_POINT('Origin',(36.3549260746835,-87.7685555885722,114.));
#39496=CARTESIAN_POINT('',(33.8367589339947,-87.7707538181913,120.387416697508));
#39497=CARTESIAN_POINT('',(33.8333405706013,-87.7682823373648,120.112583302492));
#39498=CARTESIAN_POINT('',(33.8374260746835,-87.7685555885722,114.));
#39499=CARTESIAN_POINT('Ctrl Pts',(33.8333405706013,-87.7682823373648,120.112583302492));
#39500=CARTESIAN_POINT('Ctrl Pts',(33.8333172714765,-87.7532903997163,120.11163134332));
#39501=CARTESIAN_POINT('Ctrl Pts',(33.833439535064,-87.7382988522033,120.110679384147));
#39502=CARTESIAN_POINT('Ctrl Pts',(33.8337085241762,-87.7233099378653,120.109727424975));
#39503=CARTESIAN_POINT('Ctrl Pts',(33.8485853642248,-86.8943258971421,120.057077917244));
#39504=CARTESIAN_POINT('Ctrl Pts',(34.3122671721632,-86.0733962284342,120.004428409513));
#39505=CARTESIAN_POINT('Ctrl Pts',(35.0145506733614,-85.632676734342,119.951778901782));
#39506=CARTESIAN_POINT('Ctrl Pts',(35.7168341745595,-85.1919572402497,119.899129394052));
#39507=CARTESIAN_POINT('Ctrl Pts',(36.6577193690174,-85.1314479207731,119.846479886321));
#39508=CARTESIAN_POINT('Ctrl Pts',(37.4106703483145,-85.4785798427839,119.79383037859));
#39509=CARTESIAN_POINT('Ctrl Pts',(38.1636213276117,-85.8257117647948,119.741180870859));
#39510=CARTESIAN_POINT('Ctrl Pts',(38.728638091748,-86.580484928293,119.688531363128));
#39511=CARTESIAN_POINT('Ctrl Pts',(38.8495788406817,-87.4007343549724,119.635881855397));
#39512=CARTESIAN_POINT('Ctrl Pts',(38.9705195896155,-88.2209837816518,119.583232347667));
#39513=CARTESIAN_POINT('Ctrl Pts',(38.6473843233466,-89.1067094715124,119.530582839936));
#39514=CARTESIAN_POINT('Ctrl Pts',(38.026661521466,-89.656381172705,119.477933332205));
#39515=CARTESIAN_POINT('Ctrl Pts',(37.4059387195854,-90.2060528738975,119.425283824474));
#39516=CARTESIAN_POINT('Ctrl Pts',(36.4876283820932,-90.4196705864219,119.372634316743));
#39517=CARTESIAN_POINT('Ctrl Pts',(35.6880325259561,-90.2003939587395,119.319984809013));
#39518=CARTESIAN_POINT('Ctrl Pts',(34.888436669819,-89.9811173310572,119.267335301282));
#39519=CARTESIAN_POINT('Ctrl Pts',(34.2075552950369,-89.3289463631679,119.214685793551));
#39520=CARTESIAN_POINT('Ctrl Pts',(33.9540556236766,-88.5395328507908,119.16203628582));
#39521=CARTESIAN_POINT('Ctrl Pts',(33.8746859988896,-88.2923709750261,119.145551958044));
#39522=CARTESIAN_POINT('Ctrl Pts',(33.8372121057229,-88.0317553721487,119.129067630268));
#39523=CARTESIAN_POINT('Ctrl Pts',(33.8392145615825,-87.7705794701237,119.112583302492));
#39524=CARTESIAN_POINT('Ctrl Pts',(33.8412617315361,-87.7680141434736,119.387416697508));
#39525=CARTESIAN_POINT('Ctrl Pts',(33.8421398387907,-88.2199980597614,119.415885674646));
#39526=CARTESIAN_POINT('Ctrl Pts',(33.9585452695053,-88.6724038353267,119.444354651783));
#39527=CARTESIAN_POINT('Ctrl Pts',(34.18774755072,-89.0577118621484,119.472823628921));
#39528=CARTESIAN_POINT('Ctrl Pts',(34.6116260490043,-89.7702867410744,119.525473136651));
#39529=CARTESIAN_POINT('Ctrl Pts',(35.4212864724672,-90.2533773873225,119.578122644382));
#39530=CARTESIAN_POINT('Ctrl Pts',(36.2496816025878,-90.2879821231239,119.630772152113));
#39531=CARTESIAN_POINT('Ctrl Pts',(37.0780767327084,-90.3225868589254,119.683421659844));
#39532=CARTESIAN_POINT('Ctrl Pts',(37.9252065694868,-89.9087056842802,119.736071167575));
#39533=CARTESIAN_POINT('Ctrl Pts',(38.4070376381075,-89.2339650881938,119.788720675305));
#39534=CARTESIAN_POINT('Ctrl Pts',(38.8888687067281,-88.5592244921074,119.841370183036));
#39535=CARTESIAN_POINT('Ctrl Pts',(39.0054010071911,-87.62362447458,119.894019690767));
#39536=CARTESIAN_POINT('Ctrl Pts',(38.703806486657,-86.8513055855209,119.946669198498));
#39537=CARTESIAN_POINT('Ctrl Pts',(38.4022119661228,-86.0789866964619,119.999318706229));
#39538=CARTESIAN_POINT('Ctrl Pts',(37.6824906245914,-85.4699489358712,120.05196821396));
#39539=CARTESIAN_POINT('Ctrl Pts',(36.8709169952967,-85.3002892631886,120.10461772169));
#39540=CARTESIAN_POINT('Ctrl Pts',(36.0593433660019,-85.130629590506,120.157267229421));
#39541=CARTESIAN_POINT('Ctrl Pts',(35.1559174489438,-85.4003480057315,120.209916737152));
#39542=CARTESIAN_POINT('Ctrl Pts',(34.5701940408579,-85.9871739218915,120.262566244883));
#39543=CARTESIAN_POINT('Ctrl Pts',(34.1072088154528,-86.4510306251003,120.304183062425));
#39544=CARTESIAN_POINT('Ctrl Pts',(33.8427278117577,-87.1130197820786,120.345799879966));
#39545=CARTESIAN_POINT('Ctrl Pts',(33.8367589339947,-87.7707538181913,120.387416697508));
#39546=CARTESIAN_POINT('Origin',(36.3549260746835,-87.7685555885722,114.));
#39547=CARTESIAN_POINT('',(33.8347233377312,-87.7669766891919,121.387416697508));
#39548=CARTESIAN_POINT('',(33.8399315564717,-87.7667938053724,121.112583302492));
#39549=CARTESIAN_POINT('',(33.8374260746835,-87.7685555885722,114.));
#39550=CARTESIAN_POINT('',(38.2683920713486,-86.1325683851973,122.));
#39551=CARTESIAN_POINT('Ctrl Pts',(33.8347233377312,-87.7669766891919,121.387416697508));
#39552=CARTESIAN_POINT('Ctrl Pts',(33.8401813734862,-88.496199628224,121.43366260848));
#39553=CARTESIAN_POINT('Ctrl Pts',(34.1747110856035,-89.2296737968849,121.479908519451));
#39554=CARTESIAN_POINT('Ctrl Pts',(34.7321881734164,-89.698507092816,121.526154430423));
#39555=CARTESIAN_POINT('Ctrl Pts',(35.3668582151122,-90.2322589796322,121.578803938153));
#39556=CARTESIAN_POINT('Ctrl Pts',(36.2904926403925,-90.4230071131142,121.631453445884));
#39557=CARTESIAN_POINT('Ctrl Pts',(37.0841095365915,-90.1828532978381,121.684102953615));
#39558=CARTESIAN_POINT('Ctrl Pts',(37.8777264327904,-89.942699482562,121.736752461346));
#39559=CARTESIAN_POINT('Ctrl Pts',(38.5413257999079,-89.2716437185279,121.789401969077));
#39560=CARTESIAN_POINT('Ctrl Pts',(38.7742910561279,-88.477357745742,121.842051476808));
#39561=CARTESIAN_POINT('Ctrl Pts',(39.0072563123478,-87.6830717729562,121.894700984538));
#39562=CARTESIAN_POINT('Ctrl Pts',(38.8095874576702,-86.7655555914187,121.947350492269));
#39563=CARTESIAN_POINT('Ctrl Pts',(38.2683920713486,-86.1325683851972,122.));
#39564=CARTESIAN_POINT('',(34.4378159936203,-86.1300277429912,122.));
#39565=CARTESIAN_POINT('Origin',(36.3549260746835,-87.7685555885722,122.));
#39566=CARTESIAN_POINT('Ctrl Pts',(34.4378071488063,-86.1300215764196,122.));
#39567=CARTESIAN_POINT('Ctrl Pts',(34.9606277583611,-85.5213062324827,121.949053726697));
#39568=CARTESIAN_POINT('Ctrl Pts',(35.8003521387853,-85.1811303941408,121.898107453395));
#39569=CARTESIAN_POINT('Ctrl Pts',(36.599022889058,-85.2588932747863,121.847161180092));
#39570=CARTESIAN_POINT('Ctrl Pts',(37.4243947782061,-85.3392559219499,121.794511672361));
#39571=CARTESIAN_POINT('Ctrl Pts',(38.2059221439901,-85.8659694487247,121.74186216463));
#39572=CARTESIAN_POINT('Ctrl Pts',(38.5898067252272,-86.6007560705761,121.6892126569));
#39573=CARTESIAN_POINT('Ctrl Pts',(38.9736913064644,-87.3355426924275,121.636563149169));
#39574=CARTESIAN_POINT('Ctrl Pts',(38.9599331031547,-88.2784024093554,121.583913641438));
#39575=CARTESIAN_POINT('Ctrl Pts',(38.5545283643142,-89.0016621462416,121.531264133707));
#39576=CARTESIAN_POINT('Ctrl Pts',(38.1491236254738,-89.7249218831277,121.478614625976));
#39577=CARTESIAN_POINT('Ctrl Pts',(37.3520723511026,-90.2285816399721,121.425965118245));
#39578=CARTESIAN_POINT('Ctrl Pts',(36.5248227148927,-90.2844325978802,121.373315610515));
#39579=CARTESIAN_POINT('Ctrl Pts',(35.6975730786827,-90.3402835557883,121.320666102784));
#39580=CARTESIAN_POINT('Ctrl Pts',(34.840125080634,-89.9483257147602,121.268016595053));
#39581=CARTESIAN_POINT('Ctrl Pts',(34.3411327859834,-89.2861899807625,121.215367087322));
#39582=CARTESIAN_POINT('Ctrl Pts',(34.0164173938504,-88.8553102521269,121.181105825712));
#39583=CARTESIAN_POINT('Ctrl Pts',(33.8434956388037,-88.3100194968416,121.146844564102));
#39584=CARTESIAN_POINT('Ctrl Pts',(33.8399315564717,-87.7667938053724,121.112583302492));
#39585=CARTESIAN_POINT('Origin',(36.3549260746835,-87.7685555885722,124.208423447177));
#39586=CARTESIAN_POINT('',(33.276656425091,-87.7677421016288,107.791576552823));
#39587=CARTESIAN_POINT('',(33.2862968534675,-87.7682412892605,107.708423447177));
#39588=CARTESIAN_POINT('',(33.2814260746835,-87.768555588572,124.208423447177));
#39589=CARTESIAN_POINT('',(37.1487253572159,-90.7377785423181,107.));
#39590=CARTESIAN_POINT('Ctrl Pts',(33.2862968534675,-87.7682412892604,107.708423447177));
#39591=CARTESIAN_POINT('Ctrl Pts',(33.2859769912424,-87.2730658011076,107.682880329042));
#39592=CARTESIAN_POINT('Ctrl Pts',(33.6322292839702,-85.7577492023412,107.604687703175));
#39593=CARTESIAN_POINT('Ctrl Pts',(36.0033916884657,-84.1596935485673,107.473845569577));
#39594=CARTESIAN_POINT('Ctrl Pts',(39.1869513927685,-85.500150855768,107.315897046385));
#39595=CARTESIAN_POINT('Ctrl Pts',(39.797719117622,-88.9023362095446,107.157948523192));
#39596=CARTESIAN_POINT('Ctrl Pts',(38.1309639469875,-90.4751844899406,107.052649507731));
#39597=CARTESIAN_POINT('Ctrl Pts',(37.1487253572158,-90.7377785423181,107.));
#39598=CARTESIAN_POINT('',(35.5611267921502,-90.7377785423178,107.));
#39599=CARTESIAN_POINT('Origin',(36.3549260746835,-87.7685555885722,107.));
#39600=CARTESIAN_POINT('Ctrl Pts',(33.276656425091,-87.7677421016288,107.791576552823));
#39601=CARTESIAN_POINT('Ctrl Pts',(33.2765003562394,-87.7232332639992,107.789262006108));
#39602=CARTESIAN_POINT('Ctrl Pts',(33.2974600730684,-86.6664238442207,107.734297951662));
#39603=CARTESIAN_POINT('Ctrl Pts',(34.5067289212608,-84.6483928869776,107.626684389485));
#39604=CARTESIAN_POINT('Ctrl Pts',(37.9573945529429,-84.5150172531596,107.468735866293));
#39605=CARTESIAN_POINT('Ctrl Pts',(39.9550036656341,-87.3323307232591,107.3107873431));
#39606=CARTESIAN_POINT('Ctrl Pts',(38.7024883475988,-90.5088734081208,107.154542054336));
#39607=CARTESIAN_POINT('Ctrl Pts',(36.5061793313629,-90.9937479331884,107.050946273303));
#39608=CARTESIAN_POINT('Ctrl Pts',(35.5592127764325,-90.7428670628568,107.));
#39609=CARTESIAN_POINT('Origin',(36.3549260746835,-87.7685555885722,124.208423447177));
#39610=CARTESIAN_POINT('',(33.2850146722309,-87.7666901939308,108.791576552823));
#39611=CARTESIAN_POINT('',(33.2798330221166,-87.7711138662328,108.708423447177));
#39612=CARTESIAN_POINT('',(33.2814260746835,-87.768555588572,124.208423447177));
#39613=CARTESIAN_POINT('Ctrl Pts',(33.2798330221166,-87.7711138662328,108.708423447178));
#39614=CARTESIAN_POINT('Ctrl Pts',(33.2872208788364,-86.9423658028956,108.665444042093));
#39615=CARTESIAN_POINT('Ctrl Pts',(34.0588699517531,-85.0862753096796,108.569815129278));
#39616=CARTESIAN_POINT('Ctrl Pts',(37.1879239371534,-84.238982297281,108.421536708732));
#39617=CARTESIAN_POINT('Ctrl Pts',(39.7658202422379,-86.5365567546996,108.26358818554));
#39618=CARTESIAN_POINT('Ctrl Pts',(39.2510962268136,-89.9512136310206,108.105639662347));
#39619=CARTESIAN_POINT('Ctrl Pts',(36.1106392104622,-91.3867839779253,107.947691139155));
#39620=CARTESIAN_POINT('Ctrl Pts',(33.6634844053523,-89.8404170618379,107.815285734098));
#39621=CARTESIAN_POINT('Ctrl Pts',(33.2866362916695,-88.2937221498332,107.735529836772));
#39622=CARTESIAN_POINT('Ctrl Pts',(33.2862968534675,-87.7682412892604,107.708423447177));
#39623=CARTESIAN_POINT('Ctrl Pts',(33.2850146722309,-87.7666901939308,108.791576552823));
#39624=CARTESIAN_POINT('Ctrl Pts',(33.2828705409932,-87.3842072553396,108.771825719159));
#39625=CARTESIAN_POINT('Ctrl Pts',(33.5258649413941,-85.9847713296537,108.699425377765));
#39626=CARTESIAN_POINT('Ctrl Pts',(35.6128383524474,-84.2187467086474,108.57437552864));
#39627=CARTESIAN_POINT('Ctrl Pts',(38.9216913848391,-85.2066069974257,108.416427005448));
#39628=CARTESIAN_POINT('Ctrl Pts',(39.9033344292869,-88.5173188003331,108.258478482255));
#39629=CARTESIAN_POINT('Ctrl Pts',(37.6677475399111,-91.14912788279,108.100529959063));
#39630=CARTESIAN_POINT('Ctrl Pts',(34.2920594545513,-90.7222680374125,107.944895982585));
#39631=CARTESIAN_POINT('Ctrl Pts',(33.2800504890387,-88.7356856702426,107.841911513839));
#39632=CARTESIAN_POINT('Ctrl Pts',(33.276656425091,-87.7677421016288,107.791576552823));
#39633=CARTESIAN_POINT('Origin',(36.3549260746835,-87.7685555885722,124.208423447177));
#39634=CARTESIAN_POINT('',(33.2830914204259,-87.7711482488633,109.791576552823));
#39635=CARTESIAN_POINT('',(33.2787950739713,-87.766287537244,109.708423447178));
#39636=CARTESIAN_POINT('',(33.2814260746835,-87.768555588572,124.208423447177));
#39637=CARTESIAN_POINT('Ctrl Pts',(33.2787950739713,-87.766287537244,109.708423447178));
#39638=CARTESIAN_POINT('Ctrl Pts',(33.2775559525143,-87.6166677820898,109.700657262876));
#39639=CARTESIAN_POINT('Ctrl Pts',(33.3552188510478,-86.4540177546672,109.640241570843));
#39640=CARTESIAN_POINT('Ctrl Pts',(34.8365759788977,-84.4751585833882,109.527176371079));
#39641=CARTESIAN_POINT('Ctrl Pts',(38.2826268788027,-84.6967777516425,109.369227847887));
#39642=CARTESIAN_POINT('Ctrl Pts',(39.9808905139985,-87.7034840332521,109.211279324694));
#39643=CARTESIAN_POINT('Ctrl Pts',(38.3916015946044,-90.7691895942252,109.053330801502));
#39644=CARTESIAN_POINT('Ctrl Pts',(34.9557227260359,-91.1143097541466,108.89538227831));
#39645=CARTESIAN_POINT('Ctrl Pts',(33.3781908644244,-89.1574729097927,108.780413160201));
#39646=CARTESIAN_POINT('Ctrl Pts',(33.278170799648,-87.9575770996091,108.718093549824));
#39647=CARTESIAN_POINT('Ctrl Pts',(33.2798330221166,-87.7711138662328,108.708423447178));
#39648=CARTESIAN_POINT('Ctrl Pts',(33.2830914204259,-87.7711482488633,109.791576552823));
#39649=CARTESIAN_POINT('Ctrl Pts',(33.2889508656634,-87.052142123377,109.754389432211));
#39650=CARTESIAN_POINT('Ctrl Pts',(33.8981617705012,-85.3062204171677,109.664552803868));
#39651=CARTESIAN_POINT('Ctrl Pts',(36.7983710322676,-84.1692218413362,109.522066667795));
#39652=CARTESIAN_POINT('Ctrl Pts',(39.611248718183,-86.1722442141325,109.364118144603));
#39653=CARTESIAN_POINT('Ctrl Pts',(39.4717176740767,-89.6225937013098,109.20616962141));
#39654=CARTESIAN_POINT('Ctrl Pts',(36.506286532656,-91.3919429301732,109.048221098218));
#39655=CARTESIAN_POINT('Ctrl Pts',(33.7915972796456,-90.0656305669141,108.910023408688));
#39656=CARTESIAN_POINT('Ctrl Pts',(33.2885861201985,-88.4037864171892,108.82447522689));
#39657=CARTESIAN_POINT('Ctrl Pts',(33.2850146722309,-87.7666901939308,108.791576552823));
#39658=CARTESIAN_POINT('Origin',(36.3549260746835,-87.7685555885722,124.208423447177));
#39659=CARTESIAN_POINT('',(33.2765846421026,-87.7678707817249,110.791576552823));
#39660=CARTESIAN_POINT('',(33.2862067465171,-87.7682071721922,110.708423447177));
#39661=CARTESIAN_POINT('',(33.2814260746835,-87.768555588572,124.208423447177));
#39662=CARTESIAN_POINT('Ctrl Pts',(33.2862067465171,-87.7682071721922,110.708423447177));
#39663=CARTESIAN_POINT('Ctrl Pts',(33.2857074510608,-87.2796756315349,110.683220975927));
#39664=CARTESIAN_POINT('Ctrl Pts',(33.6253685298192,-85.7712275726879,110.605368996946));
#39665=CARTESIAN_POINT('Ctrl Pts',(35.9808934716759,-84.1613474908357,110.474867510234));
#39666=CARTESIAN_POINT('Ctrl Pts',(39.1709557485403,-85.4834237534817,110.316918987042));
#39667=CARTESIAN_POINT('Ctrl Pts',(39.8078095714184,-88.8773595462129,110.158970463849));
#39668=CARTESIAN_POINT('Ctrl Pts',(37.3140389309351,-91.2659765249159,110.001021940657));
#39669=CARTESIAN_POINT('Ctrl Pts',(34.1160436361588,-90.5220575995161,109.850839601766));
#39670=CARTESIAN_POINT('Ctrl Pts',(33.285956362831,-88.6309891205378,109.753306770607));
#39671=CARTESIAN_POINT('Ctrl Pts',(33.2787950739713,-87.766287537244,109.708423447178));
#39672=CARTESIAN_POINT('Ctrl Pts',(33.2765846421026,-87.7678707817249,110.791576552823));
#39673=CARTESIAN_POINT('Ctrl Pts',(33.2764689981345,-87.7299144954526,110.789602652993));
#39674=CARTESIAN_POINT('Ctrl Pts',(33.2942329377382,-86.679667114291,110.734979245433));
#39675=CARTESIAN_POINT('Ctrl Pts',(34.4867514469574,-84.660216714833,110.627706330142));
#39676=CARTESIAN_POINT('Ctrl Pts',(37.9364315130628,-84.5050164759499,110.46975780695));
#39677=CARTESIAN_POINT('Ctrl Pts',(39.9522086976689,-87.3087678935207,110.311809283757));
#39678=CARTESIAN_POINT('Ctrl Pts',(38.7064391340791,-90.5293948322461,110.153860760565));
#39679=CARTESIAN_POINT('Ctrl Pts',(35.3286241982722,-91.2468527920333,109.995912237372));
#39680=CARTESIAN_POINT('Ctrl Pts',(33.4575135227322,-89.3842210456531,109.875150834792));
#39681=CARTESIAN_POINT('Ctrl Pts',(33.2806550658742,-88.070110654944,109.807038939942));
#39682=CARTESIAN_POINT('Ctrl Pts',(33.2830914204259,-87.7711482488633,109.791576552823));
#39683=CARTESIAN_POINT('Origin',(36.3549260746835,-87.7685555885722,124.208423447177));
#39684=CARTESIAN_POINT('',(33.2848890248079,-87.7666135332359,111.791576552823));
#39685=CARTESIAN_POINT('',(33.2800259451788,-87.7711513823149,111.708423447177));
#39686=CARTESIAN_POINT('',(33.2814260746835,-87.768555588572,124.208423447177));
#39687=CARTESIAN_POINT('Ctrl Pts',(33.2800259451788,-87.7711513823149,111.708423447177));
#39688=CARTESIAN_POINT('Ctrl Pts',(33.2874068247419,-86.9488393585243,111.665784688979));
#39689=CARTESIAN_POINT('Ctrl Pts',(34.0488667873028,-85.0990844447291,111.570496423049));
#39690=CARTESIAN_POINT('Ctrl Pts',(37.1652521907151,-84.2336974260193,111.422558649389));
#39691=CARTESIAN_POINT('Ctrl Pts',(39.7578211449723,-86.5146992235859,111.264610126197));
#39692=CARTESIAN_POINT('Ctrl Pts',(39.2650886334483,-89.9325344528934,111.106661603004));
#39693=CARTESIAN_POINT('Ctrl Pts',(36.1338002383326,-91.3883558605165,110.948713079812));
#39694=CARTESIAN_POINT('Ctrl Pts',(33.6706422156574,-89.8535959444207,110.815967027869));
#39695=CARTESIAN_POINT('Ctrl Pts',(33.2867505098833,-88.300247974271,110.735870483658));
#39696=CARTESIAN_POINT('Ctrl Pts',(33.2862067465171,-87.7682071721922,110.708423447177));
#39697=CARTESIAN_POINT('Ctrl Pts',(33.2848890248079,-87.7666135332359,111.791576552823));
#39698=CARTESIAN_POINT('Ctrl Pts',(33.2826893479257,-87.3907660509209,111.772166366045));
#39699=CARTESIAN_POINT('Ctrl Pts',(33.5201236359259,-85.9981265337506,111.700106671536));
#39700=CARTESIAN_POINT('Ctrl Pts',(35.5900605844347,-84.2235834060515,111.575397469297));
#39701=CARTESIAN_POINT('Ctrl Pts',(38.9051876872665,-85.1901815465887,111.417448946105));
#39702=CARTESIAN_POINT('Ctrl Pts',(39.9080701486722,-88.4945130132787,111.259500422912));
#39703=CARTESIAN_POINT('Ctrl Pts',(37.6894249421801,-91.1406409620089,111.10155189972));
#39704=CARTESIAN_POINT('Ctrl Pts',(34.3036777199347,-90.7345409621052,110.945577276356));
#39705=CARTESIAN_POINT('Ctrl Pts',(33.2795535508054,-88.7423163194395,110.842252160724));
#39706=CARTESIAN_POINT('Ctrl Pts',(33.2765846421026,-87.7678707817249,110.791576552823));
#39707=CARTESIAN_POINT('Origin',(36.3549260746835,-87.7685555885722,124.208423447177));
#39708=CARTESIAN_POINT('',(33.2832675127287,-87.7711115886087,112.791576552823));
#39709=CARTESIAN_POINT('',(33.2786192921776,-87.7663532934355,112.708423447177));
#39710=CARTESIAN_POINT('',(33.2814260746835,-87.768555588572,124.208423447177));
#39711=CARTESIAN_POINT('Ctrl Pts',(33.2786192921776,-87.7663532934355,112.708423447177));
#39712=CARTESIAN_POINT('Ctrl Pts',(33.2774584286707,-87.6233176056221,112.700997909761));
#39713=CARTESIAN_POINT('Ctrl Pts',(33.3512647595745,-86.467315453029,112.640922864614));
#39714=CARTESIAN_POINT('Ctrl Pts',(34.8154603259275,-84.484975857241,112.528198311736));
#39715=CARTESIAN_POINT('Ctrl Pts',(38.2628633754255,-84.6844631937108,112.370249788544));
#39716=CARTESIAN_POINT('Ctrl Pts',(39.9803977016302,-87.6802033061719,112.212301265351));
#39717=CARTESIAN_POINT('Ctrl Pts',(38.4108271674185,-90.7560497459711,112.054352742159));
#39718=CARTESIAN_POINT('Ctrl Pts',(34.9772336398273,-91.1232260937864,111.896404218966));
#39719=CARTESIAN_POINT('Ctrl Pts',(33.3824604435757,-89.1707887589986,111.781094453973));
#39720=CARTESIAN_POINT('Ctrl Pts',(33.2782930584871,-87.9642142212732,111.71843419671));
#39721=CARTESIAN_POINT('Ctrl Pts',(33.2800259451788,-87.7711513823149,111.708423447177));
#39722=CARTESIAN_POINT('Ctrl Pts',(33.2832675127287,-87.7711115886087,112.791576552823));
#39723=CARTESIAN_POINT('Ctrl Pts',(33.2889665649355,-87.0585882653705,112.754730079097));
#39724=CARTESIAN_POINT('Ctrl Pts',(33.889317805798,-85.3192833343254,112.66523409764));
#39725=CARTESIAN_POINT('Ctrl Pts',(36.7752505778273,-84.1664486627489,112.523088608452));
#39726=CARTESIAN_POINT('Ctrl Pts',(39.6009316700625,-86.1513683181001,112.365140085259));
#39727=CARTESIAN_POINT('Ctrl Pts',(39.4835582117651,-89.6025424870611,112.207191562067));
#39728=CARTESIAN_POINT('Ctrl Pts',(36.5295491478211,-91.3908965133523,112.049243038874));
#39729=CARTESIAN_POINT('Ctrl Pts',(33.7996873271964,-90.0788158412429,111.91070470246));
#39730=CARTESIAN_POINT('Ctrl Pts',(33.2886559007642,-88.4102402657966,111.824815873776));
#39731=CARTESIAN_POINT('Ctrl Pts',(33.2848890248079,-87.7666135332359,111.791576552823));
#39732=CARTESIAN_POINT('Origin',(36.3549260746835,-87.7685555885722,124.208423447177));
#39733=CARTESIAN_POINT('',(33.2765254057624,-87.7679866768878,113.791576552823));
#39734=CARTESIAN_POINT('',(33.2861808694117,-87.7681022535048,113.708423447177));
#39735=CARTESIAN_POINT('',(33.2814260746835,-87.768555588572,124.208423447177));
#39736=CARTESIAN_POINT('Ctrl Pts',(33.2861808694117,-87.7681022535048,113.708423447177));
#39737=CARTESIAN_POINT('Ctrl Pts',(33.285539692702,-87.2861840612657,113.683561622813));
#39738=CARTESIAN_POINT('Ctrl Pts',(33.618721455999,-85.7845535822887,113.606050290717));
#39739=CARTESIAN_POINT('Ctrl Pts',(35.9577393041295,-84.1638235162957,113.475889450891));
#39740=CARTESIAN_POINT('Ctrl Pts',(39.1562248702749,-85.4653891374834,113.317940927699));
#39741=CARTESIAN_POINT('Ctrl Pts',(39.8148580161093,-88.8551657322322,113.159992404506));
#39742=CARTESIAN_POINT('Ctrl Pts',(37.3364760997262,-91.2597459574781,113.002043881314));
#39743=CARTESIAN_POINT('Ctrl Pts',(34.1265055614965,-90.5347359476712,112.851520895538));
#39744=CARTESIAN_POINT('Ctrl Pts',(33.2856893335538,-88.6374877766429,112.753647417492));
#39745=CARTESIAN_POINT('Ctrl Pts',(33.2786192921776,-87.7663532934355,112.708423447177));
#39746=CARTESIAN_POINT('Ctrl Pts',(33.2765254057624,-87.7679866768878,113.791576552823));
#39747=CARTESIAN_POINT('Ctrl Pts',(33.2764447224955,-87.7365823392088,113.789943299879));
#39748=CARTESIAN_POINT('Ctrl Pts',(33.2910498895119,-86.6929052864662,113.735660539204));
#39749=CARTESIAN_POINT('Ctrl Pts',(34.4668313200981,-84.6722763390996,113.628728270799));
#39750=CARTESIAN_POINT('Ctrl Pts',(37.9154437312407,-84.4949289090955,113.470779747607));
#39751=CARTESIAN_POINT('Ctrl Pts',(39.949182244182,-87.2856792265183,113.312831224414));
#39752=CARTESIAN_POINT('Ctrl Pts',(38.724118002599,-90.5142388553946,113.154882701222));
#39753=CARTESIAN_POINT('Ctrl Pts',(35.3509794956904,-91.2533709724249,112.996934178029));
#39754=CARTESIAN_POINT('Ctrl Pts',(33.4626357327023,-89.3975718565036,112.875832128563));
#39755=CARTESIAN_POINT('Ctrl Pts',(33.2808232539786,-88.0767047476726,112.807379586827));
#39756=CARTESIAN_POINT('Ctrl Pts',(33.2832675127287,-87.7711115886087,112.791576552823));
#39757=CARTESIAN_POINT('Origin',(36.3549260746835,-87.7685555885722,124.208423447177));
#39758=CARTESIAN_POINT('',(33.2847581226811,-87.7665395828602,114.791576552823));
#39759=CARTESIAN_POINT('',(33.2802201284861,-87.7711845286359,114.708423447177));
#39760=CARTESIAN_POINT('',(33.2814260746835,-87.768555588572,124.208423447177));
#39761=CARTESIAN_POINT('Ctrl Pts',(33.2802201284861,-87.7711845286358,114.708423447177));
#39762=CARTESIAN_POINT('Ctrl Pts',(33.2875819596571,-86.9553091102221,114.666125335864));
#39763=CARTESIAN_POINT('Ctrl Pts',(34.0389366156125,-85.1119079714602,114.571177716821));
#39764=CARTESIAN_POINT('Ctrl Pts',(37.1425381673794,-84.2285671938113,114.423580590046));
#39765=CARTESIAN_POINT('Ctrl Pts',(39.749699985204,-86.4928750877993,114.265632066854));
#39766=CARTESIAN_POINT('Ctrl Pts',(39.278923545741,-89.9138036937695,114.107683543661));
#39767=CARTESIAN_POINT('Ctrl Pts',(36.1570475286333,-91.3897010875291,113.949735020469));
#39768=CARTESIAN_POINT('Ctrl Pts',(33.6777395898086,-89.8668909803513,113.816648321641));
#39769=CARTESIAN_POINT('Ctrl Pts',(33.2868975028787,-88.3067348951798,113.736211130544));
#39770=CARTESIAN_POINT('Ctrl Pts',(33.2861808694117,-87.7681022535048,113.708423447177));
#39771=CARTESIAN_POINT('Ctrl Pts',(33.2847581226811,-87.7665395828602,114.791576552823));
#39772=CARTESIAN_POINT('Ctrl Pts',(33.2825086201721,-87.3973277786715,114.772507012931));
#39773=CARTESIAN_POINT('Ctrl Pts',(33.5144370064031,-86.011481870544,114.700787965308));
#39774=CARTESIAN_POINT('Ctrl Pts',(35.5673140912984,-84.2285676851132,114.576419409954));
#39775=CARTESIAN_POINT('Ctrl Pts',(38.8885793784847,-85.1738594735819,114.418470886761));
#39776=CARTESIAN_POINT('Ctrl Pts',(39.9126582726965,-88.4716833153973,114.260522363569));
#39777=CARTESIAN_POINT('Ctrl Pts',(37.7110495865035,-91.1320026319635,114.102573840377));
#39778=CARTESIAN_POINT('Ctrl Pts',(34.3153646157072,-90.7468114612145,113.946258570128));
#39779=CARTESIAN_POINT('Ctrl Pts',(33.2790456266009,-88.7489319117899,113.84259280761));
#39780=CARTESIAN_POINT('Ctrl Pts',(33.2765254057624,-87.7679866768878,113.791576552823));
#39781=CARTESIAN_POINT('Origin',(36.3549260746835,-87.7685555885722,124.208423447177));
#39782=CARTESIAN_POINT('',(33.2834402980838,-87.7710709634421,115.791576552823));
#39783=CARTESIAN_POINT('',(33.2784473899845,-87.766423078844,115.708423447177));
#39784=CARTESIAN_POINT('',(33.2814260746835,-87.768555588572,124.208423447177));
#39785=CARTESIAN_POINT('Ctrl Pts',(33.2784473899845,-87.766423078844,115.708423447177));
#39786=CARTESIAN_POINT('Ctrl Pts',(33.277364854453,-87.6299690776632,115.701338556647));
#39787=CARTESIAN_POINT('Ctrl Pts',(33.3473575742145,-86.4806099825772,115.641604158385));
#39788=CARTESIAN_POINT('Ctrl Pts',(34.7944082015486,-84.4949284547604,115.529220252393));
#39789=CARTESIAN_POINT('Ctrl Pts',(38.2430210913116,-84.6722759093786,115.371271729201));
#39790=CARTESIAN_POINT('Ctrl Pts',(39.979755653312,-87.6569259800321,115.213323206008));
#39791=CARTESIAN_POINT('Ctrl Pts',(38.4299674805782,-90.7427872216878,115.055374682816));
#39792=CARTESIAN_POINT('Ctrl Pts',(34.9988023746513,-91.1320030987637,114.897426159623));
#39793=CARTESIAN_POINT('Ctrl Pts',(33.3867772569319,-89.1841085494937,114.781775747744));
#39794=CARTESIAN_POINT('Ctrl Pts',(33.2784185058971,-87.9708494692539,114.718774843595));
#39795=CARTESIAN_POINT('Ctrl Pts',(33.2802201284861,-87.7711845286358,114.708423447177));
#39796=CARTESIAN_POINT('Ctrl Pts',(33.2834402980838,-87.7710709634421,115.791576552823));
#39797=CARTESIAN_POINT('Ctrl Pts',(33.2889738902515,-87.0650343515427,115.755070725982));
#39798=CARTESIAN_POINT('Ctrl Pts',(33.880540019459,-85.3323584119177,115.665915391411));
#39799=CARTESIAN_POINT('Ctrl Pts',(36.7521127901144,-84.1638240165833,115.524110549109));
#39800=CARTESIAN_POINT('Ctrl Pts',(39.5904807973608,-86.1305590594033,115.366162025916));
#39801=CARTESIAN_POINT('Ctrl Pts',(39.4952697425043,-89.5824157378083,115.208213502724));
#39802=CARTESIAN_POINT('Ctrl Pts',(36.55280459327,-91.3897005849636,115.050264979531));
#39803=CARTESIAN_POINT('Ctrl Pts',(33.8078412450219,-90.0919923385608,114.911385996231));
#39804=CARTESIAN_POINT('Ctrl Pts',(33.2887193206088,-88.4166926846419,114.825156520661));
#39805=CARTESIAN_POINT('Ctrl Pts',(33.2847581226811,-87.7665395828602,114.791576552823));
#39806=CARTESIAN_POINT('Origin',(36.3549260746835,-87.7685555885722,124.208423447177));
#39807=CARTESIAN_POINT('',(33.2764765005074,-87.7681038465887,116.791576552823));
#39808=CARTESIAN_POINT('',(33.286148224798,-87.7679979949527,116.708423447177));
#39809=CARTESIAN_POINT('',(33.2814260746835,-87.768555588572,124.208423447177));
#39810=CARTESIAN_POINT('Ctrl Pts',(33.286148224798,-87.7679979949527,116.708423447177));
#39811=CARTESIAN_POINT('Ctrl Pts',(33.2853699201791,-87.2926954938565,116.683902269698));
#39812=CARTESIAN_POINT('Ctrl Pts',(33.6121327235052,-85.7978827795205,116.606731584489));
#39813=CARTESIAN_POINT('Ctrl Pts',(35.9346015132054,-84.1664481628253,116.476911391548));
#39814=CARTESIAN_POINT('Ctrl Pts',(39.1413784939057,-85.4474494817745,116.318962868356));
#39815=CARTESIAN_POINT('Ctrl Pts',(39.8217638122167,-88.8329271145059,116.161014345163));
#39816=CARTESIAN_POINT('Ctrl Pts',(37.35887279301,-91.2533714560701,116.003065821971));
#39817=CARTESIAN_POINT('Ctrl Pts',(34.1370383056434,-90.5473935246883,115.852202189309));
#39818=CARTESIAN_POINT('Ctrl Pts',(33.2854094336303,-88.6439912363789,115.753988064378));
#39819=CARTESIAN_POINT('Ctrl Pts',(33.2784473899845,-87.766423078844,115.708423447177));
#39820=CARTESIAN_POINT('Ctrl Pts',(33.2764765005074,-87.7681038465887,116.791576552823));
#39821=CARTESIAN_POINT('Ctrl Pts',(33.2764250132567,-87.7432505594706,116.790283946765));
#39822=CARTESIAN_POINT('Ctrl Pts',(33.2879105001274,-86.7061397062465,116.736341832976));
#39823=CARTESIAN_POINT('Ctrl Pts',(34.446989038738,-84.6844636217403,116.629750211456));
#39824=CARTESIAN_POINT('Ctrl Pts',(37.8943916097836,-84.4849763129574,116.471801688264));
#39825=CARTESIAN_POINT('Ctrl Pts',(39.9460076008814,-87.2626104678248,116.313853165071));
#39826=CARTESIAN_POINT('Ctrl Pts',(38.7416991899834,-90.4989696760488,116.155904641879));
#39827=CARTESIAN_POINT('Ctrl Pts',(35.3733761858658,-91.2597454729484,115.997956118686));
#39828=CARTESIAN_POINT('Ctrl Pts',(33.467810152958,-89.4109237193908,115.876513422334));
#39829=CARTESIAN_POINT('Ctrl Pts',(33.2809932217164,-88.0832959079491,115.807720233713));
#39830=CARTESIAN_POINT('Ctrl Pts',(33.2834402980838,-87.7710709634421,115.791576552823));
#39831=CARTESIAN_POINT('Origin',(36.3549260746835,-87.7685555885722,124.208423447177));
#39832=CARTESIAN_POINT('',(33.2846220850711,-87.7664686536375,117.791576552823));
#39833=CARTESIAN_POINT('',(33.2804153315645,-87.7712132051916,117.708423447177));
#39834=CARTESIAN_POINT('',(33.2814260746835,-87.768555588572,124.208423447177));
#39835=CARTESIAN_POINT('Ctrl Pts',(33.2804153315645,-87.7712132051916,117.708423447177));
#39836=CARTESIAN_POINT('Ctrl Pts',(33.2877457498334,-86.961775983013,117.66646598275));
#39837=CARTESIAN_POINT('Ctrl Pts',(34.029075750275,-85.1247490441378,117.571859010592));
#39838=CARTESIAN_POINT('Ctrl Pts',(37.1197916710861,-84.2235829140579,117.424602530703));
#39839=CARTESIAN_POINT('Ctrl Pts',(39.7414388600909,-86.4711035478885,117.26665400751));
#39840=CARTESIAN_POINT('Ctrl Pts',(39.2926379026969,-89.8949844867843,117.108705484318));
#39841=CARTESIAN_POINT('Ctrl Pts',(36.1803029773098,-91.3908970160839,116.950756961125));
#39842=CARTESIAN_POINT('Ctrl Pts',(33.6848972884743,-89.8801809978657,116.817329615412));
#39843=CARTESIAN_POINT('Ctrl Pts',(33.2870410208056,-88.3132191912772,116.736551777429));
#39844=CARTESIAN_POINT('Ctrl Pts',(33.286148224798,-87.7679979949527,116.708423447177));
#39845=CARTESIAN_POINT('Ctrl Pts',(33.2846220850711,-87.7664686536375,117.791576552823));
#39846=CARTESIAN_POINT('Ctrl Pts',(33.2823284532367,-87.403892657692,117.772847659816));
#39847=CARTESIAN_POINT('Ctrl Pts',(33.508804776359,-86.0248374422096,117.701469259079));
#39848=CARTESIAN_POINT('Ctrl Pts',(35.544600071115,-84.2336979166091,117.577441350611));
#39849=CARTESIAN_POINT('Ctrl Pts',(38.87186660808,-85.1576443789841,117.419492827418));
#39850=CARTESIAN_POINT('Ctrl Pts',(39.9170997126827,-88.4488246277999,117.261544304226));
#39851=CARTESIAN_POINT('Ctrl Pts',(37.7326183183341,-91.1232256282042,117.103595781033));
#39852=CARTESIAN_POINT('Ctrl Pts',(34.3271248220504,-90.7590541983513,116.946939863899));
#39853=CARTESIAN_POINT('Ctrl Pts',(33.2785221552211,-88.7555569185142,116.842933454495));
#39854=CARTESIAN_POINT('Ctrl Pts',(33.2764765005074,-87.7681038465887,116.791576552823));
#39855=CARTESIAN_POINT('Origin',(36.3549260746835,-87.7685555885722,124.208423447177));
#39856=CARTESIAN_POINT('',(33.2836095561072,-87.7710264525037,118.791576552823));
#39857=CARTESIAN_POINT('',(33.2782797302468,-87.7664967944082,118.708423447177));
#39858=CARTESIAN_POINT('',(33.2814260746835,-87.768555588572,124.208423447177));
#39859=CARTESIAN_POINT('Ctrl Pts',(33.2782797302468,-87.7664967944082,118.708423447177));
#39860=CARTESIAN_POINT('Ctrl Pts',(33.2772752951819,-87.6366221208762,118.701679203533));
#39861=CARTESIAN_POINT('Ctrl Pts',(33.3434970963766,-86.4939012863813,118.642285452157));
#39862=CARTESIAN_POINT('Ctrl Pts',(34.7734204168137,-84.5050160230137,118.53024219305));
#39863=CARTESIAN_POINT('Ctrl Pts',(38.2231009616876,-84.6602162834389,118.372293669858));
#39864=CARTESIAN_POINT('Ctrl Pts',(39.9789641545662,-87.6336532564003,118.214345146665));
#39865=CARTESIAN_POINT('Ctrl Pts',(38.4490222405119,-90.7294020708598,118.056396623473));
#39866=CARTESIAN_POINT('Ctrl Pts',(35.0204270219759,-91.1406414300081,117.89844810028));
#39867=CARTESIAN_POINT('Ctrl Pts',(33.3911427650589,-89.1974309536143,117.782457041515));
#39868=CARTESIAN_POINT('Ctrl Pts',(33.278547317121,-87.9774825293533,117.719115490481));
#39869=CARTESIAN_POINT('Ctrl Pts',(33.2804153315645,-87.7712132051916,117.708423447177));
#39870=CARTESIAN_POINT('Ctrl Pts',(33.2836095561072,-87.7710264525037,118.791576552823));
#39871=CARTESIAN_POINT('Ctrl Pts',(33.2889730288622,-87.0714805284451,118.755411372868));
#39872=CARTESIAN_POINT('Ctrl Pts',(33.8718282039732,-85.3454453482408,118.666596685182));
#39873=CARTESIAN_POINT('Ctrl Pts',(36.7289586257789,-84.1613479914634,118.525132489766));
#39874=CARTESIAN_POINT('Ctrl Pts',(39.5798965242524,-86.1098173350916,118.367183966573));
#39875=CARTESIAN_POINT('Ctrl Pts',(39.506851797809,-89.5622142035652,118.209235443381));
#39876=CARTESIAN_POINT('Ctrl Pts',(36.5760518803447,-91.3883553581382,118.051286920188));
#39877=CARTESIAN_POINT('Ctrl Pts',(33.816059301366,-90.1051595057121,117.912067290002));
#39878=CARTESIAN_POINT('Ctrl Pts',(33.2887761694447,-88.4231439126922,117.825497167547));
#39879=CARTESIAN_POINT('Ctrl Pts',(33.2846220850711,-87.7664686536375,117.791576552823));
#39880=CARTESIAN_POINT('Origin',(36.3549260746835,-87.7685555885722,124.208423447177));
#39881=CARTESIAN_POINT('',(33.2764382705934,-87.7682219887363,119.791576552823));
#39882=CARTESIAN_POINT('',(33.2861088517784,-87.7678945631458,119.708423447177));
#39883=CARTESIAN_POINT('',(33.2814260746835,-87.768555588572,124.208423447177));
#39884=CARTESIAN_POINT('Ctrl Pts',(33.2861088517784,-87.7678945631458,119.708423447177));
#39885=CARTESIAN_POINT('Ctrl Pts',(33.2851982987019,-87.2992099652641,119.684242916584));
#39886=CARTESIAN_POINT('Ctrl Pts',(33.6056020953296,-85.8112149377787,119.60741287826));
#39887=CARTESIAN_POINT('Ctrl Pts',(35.9114810555574,-84.1692213417312,119.477933332205));
#39888=CARTESIAN_POINT('Ctrl Pts',(39.1264172314171,-85.4296055153237,119.319984809012));
#39889=CARTESIAN_POINT('Ctrl Pts',(39.8285266726477,-88.8106446175552,119.16203628582));
#39890=CARTESIAN_POINT('Ctrl Pts',(37.3812280935308,-91.2468532747826,119.004087762628));
#39891=CARTESIAN_POINT('Ctrl Pts',(34.1476420214725,-90.5600299555096,118.85288348308));
#39892=CARTESIAN_POINT('Ctrl Pts',(33.2851165023653,-88.6504997309026,118.754328711263));
#39893=CARTESIAN_POINT('Ctrl Pts',(33.2782797302468,-87.7664967944082,118.708423447177));
#39894=CARTESIAN_POINT('Ctrl Pts',(33.2764382705934,-87.7682219887363,119.791576552823));
#39895=CARTESIAN_POINT('Ctrl Pts',(33.2764098257633,-87.749919021363,119.79062459365));
#39896=CARTESIAN_POINT('Ctrl Pts',(33.2848144678827,-86.7193702351704,119.737023126747));
#39897=CARTESIAN_POINT('Ctrl Pts',(34.4272255383588,-84.6967781783805,119.630772152113));
#39898=CARTESIAN_POINT('Ctrl Pts',(37.8732759596097,-84.4751590402537,119.47282362892));
#39899=CARTESIAN_POINT('Ctrl Pts',(39.9426849263303,-87.2395625969708,119.314875105728));
#39900=CARTESIAN_POINT('Ctrl Pts',(38.7591819580553,-90.4835879091297,119.156926582536));
#39901=CARTESIAN_POINT('Ctrl Pts',(35.3958133515618,-91.2659760395494,118.998978059343));
#39902=CARTESIAN_POINT('Ctrl Pts',(33.4730370091077,-89.4242765090044,118.877194716105));
#39903=CARTESIAN_POINT('Ctrl Pts',(33.2811648498173,-88.0898841029006,118.808060880599));
#39904=CARTESIAN_POINT('Ctrl Pts',(33.2836095561072,-87.7710264525037,118.791576552823));
#39905=CARTESIAN_POINT('Origin',(36.3549260746835,-87.7685555885722,124.208423447177));
#39906=CARTESIAN_POINT('',(33.2844849022013,-87.7664047084671,120.791576552823));
#39907=CARTESIAN_POINT('',(33.2806115932904,-87.7712393060438,120.708423447177));
#39908=CARTESIAN_POINT('',(33.2814260746835,-87.768555588572,124.208423447177));
#39909=CARTESIAN_POINT('Ctrl Pts',(33.2806115932904,-87.7712393060438,120.708423447177));
#39910=CARTESIAN_POINT('Ctrl Pts',(33.2878987217132,-86.9682420627499,120.666806629636));
#39911=CARTESIAN_POINT('Ctrl Pts',(34.0192835273626,-85.1376046855688,120.572540304363));
#39912=CARTESIAN_POINT('Ctrl Pts',(37.0970139002824,-84.2187462125039,120.42562447136));
#39913=CARTESIAN_POINT('Ctrl Pts',(39.7330379835356,-86.4493848109254,120.267675948167));
#39914=CARTESIAN_POINT('Ctrl Pts',(39.3062312004495,-89.8760779436413,120.109727424975));
#39915=CARTESIAN_POINT('Ctrl Pts',(36.2035655956772,-91.3919434335384,119.951778901782));
#39916=CARTESIAN_POINT('Ctrl Pts',(33.6921155484724,-89.8934658111114,119.818010909183));
#39917=CARTESIAN_POINT('Ctrl Pts',(33.2871808925518,-88.319700945156,119.736892424315));
#39918=CARTESIAN_POINT('Ctrl Pts',(33.2861088517784,-87.7678945631458,119.708423447177));
#39919=CARTESIAN_POINT('Ctrl Pts',(33.2844849022013,-87.7664047084671,120.791576552823));
#39920=CARTESIAN_POINT('Ctrl Pts',(33.2821495713156,-87.410461265801,120.773188306702));
#39921=CARTESIAN_POINT('Ctrl Pts',(33.5032143465596,-86.0381806733766,120.70215055285));
#39922=CARTESIAN_POINT('Ctrl Pts',(35.5219283374979,-84.238982809065,120.578463291268));
#39923=CARTESIAN_POINT('Ctrl Pts',(38.8550457481358,-85.1415325934838,120.420514768075));
#39924=CARTESIAN_POINT('Ctrl Pts',(39.921396384874,-88.4259400024622,120.262566244883));
#39925=CARTESIAN_POINT('Ctrl Pts',(37.7541292274747,-91.1143092867255,120.10461772169));
#39926=CARTESIAN_POINT('Ctrl Pts',(34.3389589518385,-90.7712692257301,119.94762115767));
#39927=CARTESIAN_POINT('Ctrl Pts',(33.277983009097,-88.7621916588756,119.843274101381));
#39928=CARTESIAN_POINT('Ctrl Pts',(33.2764382705934,-87.7682219887363,119.791576552823));
#39929=CARTESIAN_POINT('Origin',(36.3549260746835,-87.7685555885722,124.208423447177));
#39930=CARTESIAN_POINT('',(33.2846473629325,-87.7715718261143,121.791576552823));
#39931=CARTESIAN_POINT('',(33.2781264274053,-87.766627982914,121.708423447177));
#39932=CARTESIAN_POINT('',(33.2814260746835,-87.768555588572,124.208423447177));
#39933=CARTESIAN_POINT('',(35.5611267921505,-90.7377785423179,122.));
#39934=CARTESIAN_POINT('Ctrl Pts',(35.5611267921506,-90.7377785423179,122.));
#39935=CARTESIAN_POINT('Ctrl Pts',(34.5788882023789,-90.4751844899402,121.947350492269));
#39936=CARTESIAN_POINT('Ctrl Pts',(33.479191301356,-89.437449369678,121.877876009877));
#39937=CARTESIAN_POINT('Ctrl Pts',(33.2823061516979,-88.0970477652926,121.808401527484));
#39938=CARTESIAN_POINT('Ctrl Pts',(33.2846473629325,-87.7715718261144,121.791576552823));
#39939=CARTESIAN_POINT('',(37.1506348820562,-90.7428550338497,122.));
#39940=CARTESIAN_POINT('Origin',(36.3549260746835,-87.7685555885722,122.));
#39941=CARTESIAN_POINT('Ctrl Pts',(37.1506395173468,-90.7428673568179,122.));
#39942=CARTESIAN_POINT('Ctrl Pts',(36.203673288632,-90.9937479020275,121.949053726697));
#39943=CARTESIAN_POINT('Ctrl Pts',(34.1431241348909,-90.5388461742994,121.851861542423));
#39944=CARTESIAN_POINT('Ctrl Pts',(33.2847898923083,-88.6569027408543,121.754669358149));
#39945=CARTESIAN_POINT('Ctrl Pts',(33.2781264274053,-87.766627982914,121.708423447177));
#39946=CARTESIAN_POINT('Origin',(-36.3549260746835,87.7685555885722,114.));
#39947=CARTESIAN_POINT('',(-38.8684362443696,87.7688130730525,107.387416697508));
#39948=CARTESIAN_POINT('',(-38.8705165012504,87.7649826536256,107.112583302492));
#39949=CARTESIAN_POINT('',(-38.8724260746835,87.7685555885722,114.));
#39950=CARTESIAN_POINT('',(-38.2683920713485,89.4045427919473,107.));
#39951=CARTESIAN_POINT('Ctrl Pts',(-38.8705165012504,87.7649826536256,107.112583302492));
#39952=CARTESIAN_POINT('Ctrl Pts',(-38.8653711927169,88.3576174120498,107.075055534995));
#39953=CARTESIAN_POINT('Ctrl Pts',(-38.6541479027676,88.9533591488767,107.037527767497));
#39954=CARTESIAN_POINT('Ctrl Pts',(-38.2683920713485,89.4045427919473,107.));
#39955=CARTESIAN_POINT('',(-38.8724260746835,87.7685555885722,107.));
#39956=CARTESIAN_POINT('Origin',(-36.3549260746835,87.7685555885722,107.));
#39957=CARTESIAN_POINT('',(-38.8724260746835,87.7685555885722,106.));
#39958=CARTESIAN_POINT('',(-38.8724260746835,87.7685555885722,114.));
#39959=CARTESIAN_POINT('Origin',(-36.3549260746835,87.7685555885722,106.));
#39960=CARTESIAN_POINT('',(-34.4378158812449,89.4070834968744,107.));
#39961=CARTESIAN_POINT('Origin',(-36.3549260746835,87.7685555885722,107.));
#39962=CARTESIAN_POINT('Ctrl Pts',(-34.4378070356398,89.4070896639597,107.));
#39963=CARTESIAN_POINT('Ctrl Pts',(-34.960627611636,90.0158048285236,107.050946273303));
#39964=CARTESIAN_POINT('Ctrl Pts',(-35.8003520741518,90.3559810018596,107.101892546605));
#39965=CARTESIAN_POINT('Ctrl Pts',(-36.5990228951286,90.2782181832502,107.152838819908));
#39966=CARTESIAN_POINT('Ctrl Pts',(-37.4243948573446,90.1978556001967,107.205488327639));
#39967=CARTESIAN_POINT('Ctrl Pts',(-38.2059222840348,89.6711418460179,107.25813783537));
#39968=CARTESIAN_POINT('Ctrl Pts',(-38.5898068873655,88.9363551308301,107.3107873431));
#39969=CARTESIAN_POINT('Ctrl Pts',(-38.7760500299138,88.579870432689,107.336330461236));
#39970=CARTESIAN_POINT('Ctrl Pts',(-38.86869823836,88.174410689784,107.361873579372));
#39971=CARTESIAN_POINT('Ctrl Pts',(-38.8684362443696,87.7688130730525,107.387416697508));
#39972=CARTESIAN_POINT('Origin',(-36.3549260746835,87.7685555885722,114.));
#39973=CARTESIAN_POINT('',(-38.8737307616524,87.7664601065225,108.387416697508));
#39974=CARTESIAN_POINT('',(-38.8763330919825,87.769221903177,108.112583302492));
#39975=CARTESIAN_POINT('',(-38.8724260746835,87.7685555885722,114.));
#39976=CARTESIAN_POINT('Ctrl Pts',(-38.8763330919825,87.769221903177,108.112583302492));
#39977=CARTESIAN_POINT('Ctrl Pts',(-38.8764609279018,87.8056790395625,108.110268755777));
#39978=CARTESIAN_POINT('Ctrl Pts',(-38.8757379769668,87.8421309392208,108.107954209062));
#39979=CARTESIAN_POINT('Ctrl Pts',(-38.8741483604852,87.8785449406493,108.105639662347));
#39980=CARTESIAN_POINT('Ctrl Pts',(-38.8379890016353,88.7068623115507,108.052990154616));
#39981=CARTESIAN_POINT('Ctrl Pts',(-38.3533855985534,89.5155697700692,108.000340646886));
#39982=CARTESIAN_POINT('Ctrl Pts',(-37.6400111963707,89.9381314370947,107.947691139155));
#39983=CARTESIAN_POINT('Ctrl Pts',(-36.9266367941881,90.3606931041203,107.895041631424));
#39984=CARTESIAN_POINT('Ctrl Pts',(-35.9844913929046,90.3971089796529,107.842392123693));
#39985=CARTESIAN_POINT('Ctrl Pts',(-35.240712177595,90.0307072878974,107.789742615962));
#39986=CARTESIAN_POINT('Ctrl Pts',(-34.4969329622854,89.6643055961419,107.737093108232));
#39987=CARTESIAN_POINT('Ctrl Pts',(-33.9515199329497,88.8950863370982,107.684443600501));
#39988=CARTESIAN_POINT('Ctrl Pts',(-33.8516662806639,88.0720989817,107.63179409277));
#39989=CARTESIAN_POINT('Ctrl Pts',(-33.7518126283782,87.2491116263017,107.579144585039));
#39990=CARTESIAN_POINT('Ctrl Pts',(-34.0975183531424,86.3723561745487,107.526495077308));
#39991=CARTESIAN_POINT('Ctrl Pts',(-34.7321883128989,85.8386042781123,107.473845569577));
#39992=CARTESIAN_POINT('Ctrl Pts',(-35.3668582726554,85.304852381676,107.421196061847));
#39993=CARTESIAN_POINT('Ctrl Pts',(-36.2904924674042,85.1141040405562,107.368546554116));
#39994=CARTESIAN_POINT('Ctrl Pts',(-37.0841095003195,85.3542579905456,107.315897046385));
#39995=CARTESIAN_POINT('Ctrl Pts',(-37.8777265332349,85.5944119405351,107.263247538654));
#39996=CARTESIAN_POINT('Ctrl Pts',(-38.5413264043166,86.2654681816338,107.210598030923));
#39997=CARTESIAN_POINT('Ctrl Pts',(-38.7742916354254,87.0597540929315,107.157948523192));
#39998=CARTESIAN_POINT('Ctrl Pts',(-38.8412027968037,87.2878851000279,107.142826782959));
#39999=CARTESIAN_POINT('Ctrl Pts',(-38.872589793222,87.5261816412588,107.127705042725));
#40000=CARTESIAN_POINT('Ctrl Pts',(-38.8705165012504,87.7649826536256,107.112583302492));
#40001=CARTESIAN_POINT('Ctrl Pts',(-38.8684362443696,87.7688130730525,107.387416697508));
#40002=CARTESIAN_POINT('Ctrl Pts',(-38.8681582160124,87.33839236406,107.414523087103));
#40003=CARTESIAN_POINT('Ctrl Pts',(-38.7632495349544,86.9078163887126,107.441629476698));
#40004=CARTESIAN_POINT('Ctrl Pts',(-38.5545285033691,86.5354489778792,107.468735866293));
#40005=CARTESIAN_POINT('Ctrl Pts',(-38.149123736071,85.812189216313,107.521385374024));
#40006=CARTESIAN_POINT('Ctrl Pts',(-37.3520724215038,85.3085293693773,107.574034881755));
#40007=CARTESIAN_POINT('Ctrl Pts',(-36.5248227318176,85.2526783946356,107.626684389485));
#40008=CARTESIAN_POINT('Ctrl Pts',(-35.6975730421315,85.1968274198939,107.679333897216));
#40009=CARTESIAN_POINT('Ctrl Pts',(-34.8401249773264,85.5887853173462,107.731983404947));
#40010=CARTESIAN_POINT('Ctrl Pts',(-34.341132647486,86.2509211028512,107.784632912678));
#40011=CARTESIAN_POINT('Ctrl Pts',(-33.8421403176455,86.9130568883562,107.837282420409));
#40012=CARTESIAN_POINT('Ctrl Pts',(-33.7016037227697,87.8453705619139,107.88993192814));
#40013=CARTESIAN_POINT('Ctrl Pts',(-33.983260674345,88.6251840983987,107.94258143587));
#40014=CARTESIAN_POINT('Ctrl Pts',(-34.2649176259204,89.4049976348835,107.995230943601));
#40015=CARTESIAN_POINT('Ctrl Pts',(-34.9687681239468,90.0323110342953,108.047880451332));
#40016=CARTESIAN_POINT('Ctrl Pts',(-35.7757187871427,90.2227548238847,108.100529959063));
#40017=CARTESIAN_POINT('Ctrl Pts',(-36.5826694503386,90.413198613474,108.153179466794));
#40018=CARTESIAN_POINT('Ctrl Pts',(-37.4927202787039,90.1667727932408,108.205828974524));
#40019=CARTESIAN_POINT('Ctrl Pts',(-38.0933201138925,89.59518418843,108.258478482255));
#40020=CARTESIAN_POINT('Ctrl Pts',(-38.5836081473929,89.1285789104982,108.30145788734));
#40021=CARTESIAN_POINT('Ctrl Pts',(-38.8676793774738,88.4452865593138,108.344437292424));
#40022=CARTESIAN_POINT('Ctrl Pts',(-38.8737307616524,87.7664601065225,108.387416697508));
#40023=CARTESIAN_POINT('Origin',(-36.3549260746835,87.7685555885722,114.));
#40024=CARTESIAN_POINT('',(-38.8745809434987,87.7704133464264,109.387416697508));
#40025=CARTESIAN_POINT('',(-38.869486864403,87.7700835308745,109.112583302492));
#40026=CARTESIAN_POINT('',(-38.8724260746835,87.7685555885722,114.));
#40027=CARTESIAN_POINT('Ctrl Pts',(-38.869486864403,87.7700835308745,109.112583302492));
#40028=CARTESIAN_POINT('Ctrl Pts',(-38.8712431197542,88.0833748523089,109.092832468829));
#40029=CARTESIAN_POINT('Ctrl Pts',(-38.8169459265052,88.3960793540123,109.073081635165));
#40030=CARTESIAN_POINT('Ctrl Pts',(-38.7038063526327,88.6858055394416,109.053330801502));
#40031=CARTESIAN_POINT('Ctrl Pts',(-38.4022118492914,89.4581243842876,109.000681293771));
#40032=CARTESIAN_POINT('Ctrl Pts',(-37.6824905487707,90.067162109531,108.94803178604));
#40033=CARTESIAN_POINT('Ctrl Pts',(-36.8709169658262,90.2368217728017,108.89538227831));
#40034=CARTESIAN_POINT('Ctrl Pts',(-36.0593433828818,90.4064814360724,108.842732770579));
#40035=CARTESIAN_POINT('Ctrl Pts',(-35.1559175175137,90.1367630373703,108.790083262848));
#40036=CARTESIAN_POINT('Ctrl Pts',(-34.570194142762,89.5499371541887,108.737433755117));
#40037=CARTESIAN_POINT('Ctrl Pts',(-33.9844707680103,88.9631112710072,108.684784247386));
#40038=CARTESIAN_POINT('Ctrl Pts',(-33.716449883875,88.0591779033461,108.632134739656));
#40039=CARTESIAN_POINT('Ctrl Pts',(-33.8876338696815,87.2479259334627,108.579485231925));
#40040=CARTESIAN_POINT('Ctrl Pts',(-34.058817855488,86.4366739635793,108.526835724194));
#40041=CARTESIAN_POINT('Ctrl Pts',(-34.6692067112364,85.7181033914734,108.474186216463));
#40042=CARTESIAN_POINT('Ctrl Pts',(-35.4420916027083,85.4179581360558,108.421536708732));
#40043=CARTESIAN_POINT('Ctrl Pts',(-36.2149764941802,85.1178128806382,108.368887201001));
#40044=CARTESIAN_POINT('Ctrl Pts',(-37.1503574213755,85.2360929419088,108.316237693271));
#40045=CARTESIAN_POINT('Ctrl Pts',(-37.8241902276642,85.7191966141862,108.26358818554));
#40046=CARTESIAN_POINT('Ctrl Pts',(-38.468400392158,86.1810623667598,108.213253224524));
#40047=CARTESIAN_POINT('Ctrl Pts',(-38.8735530158786,86.9763804682205,108.162918263508));
#40048=CARTESIAN_POINT('Ctrl Pts',(-38.8763330919825,87.769221903177,108.112583302492));
#40049=CARTESIAN_POINT('Ctrl Pts',(-38.8737307616524,87.7664601065225,108.387416697508));
#40050=CARTESIAN_POINT('Ctrl Pts',(-38.8750922859929,87.6137283163819,108.397086800155));
#40051=CARTESIAN_POINT('Ctrl Pts',(-38.8623798226398,87.4612226000268,108.406756902801));
#40052=CARTESIAN_POINT('Ctrl Pts',(-38.8347755569173,87.3114618221123,108.416427005448));
#40053=CARTESIAN_POINT('Ctrl Pts',(-38.6844823227415,86.4960794499939,108.469076513179));
#40054=CARTESIAN_POINT('Ctrl Pts',(-38.0927470123779,85.7620660951455,108.521726020909));
#40055=CARTESIAN_POINT('Ctrl Pts',(-37.3278253781081,85.4421739957963,108.57437552864));
#40056=CARTESIAN_POINT('Ctrl Pts',(-36.5629037438382,85.1222818964472,108.627025036371));
#40057=CARTESIAN_POINT('Ctrl Pts',(-35.6247957856621,85.2165110525973,108.679674544102));
#40058=CARTESIAN_POINT('Ctrl Pts',(-34.9387777281827,85.6821448649725,108.732324051833));
#40059=CARTESIAN_POINT('Ctrl Pts',(-34.2527596707034,86.1477786773477,108.784973559563));
#40060=CARTESIAN_POINT('Ctrl Pts',(-33.8188315139207,86.984817145948,108.837623067294));
#40061=CARTESIAN_POINT('Ctrl Pts',(-33.8337083550104,87.8138012422328,108.890272575025));
#40062=CARTESIAN_POINT('Ctrl Pts',(-33.8485851961001,88.6427853385176,108.942922082756));
#40063=CARTESIAN_POINT('Ctrl Pts',(-34.3122670350621,89.4637150624868,108.995571590487));
#40064=CARTESIAN_POINT('Ctrl Pts',(-35.0145505833724,89.9044345861986,109.048221098218));
#40065=CARTESIAN_POINT('Ctrl Pts',(-35.7168341316828,90.3451541099105,109.100870605948));
#40066=CARTESIAN_POINT('Ctrl Pts',(-36.6577193893416,90.4056634333649,109.153520113679));
#40067=CARTESIAN_POINT('Ctrl Pts',(-37.4106704191868,90.0585314880353,109.20616962141));
#40068=CARTESIAN_POINT('Ctrl Pts',(-38.1636214490319,89.7113995427057,109.258819129141));
#40069=CARTESIAN_POINT('Ctrl Pts',(-38.7286382510635,88.956626328592,109.311468636872));
#40070=CARTESIAN_POINT('Ctrl Pts',(-38.849579008108,88.1363768468704,109.364118144603));
#40071=CARTESIAN_POINT('Ctrl Pts',(-38.867418647058,88.0153840983512,109.371884328904));
#40072=CARTESIAN_POINT('Ctrl Pts',(-38.875595906259,87.8929666916698,109.379650513206));
#40073=CARTESIAN_POINT('Ctrl Pts',(-38.8745809434987,87.7704133464264,109.387416697508));
#40074=CARTESIAN_POINT('Origin',(-36.3549260746835,87.7685555885722,114.));
#40075=CARTESIAN_POINT('',(-38.8685100522263,87.768840975972,110.387416697508));
#40076=CARTESIAN_POINT('',(-38.8710621976983,87.7664319436008,110.112583302492));
#40077=CARTESIAN_POINT('',(-38.8724260746835,87.7685555885722,114.));
#40078=CARTESIAN_POINT('Ctrl Pts',(-38.8710621976983,87.7664319436008,110.112583302492));
#40079=CARTESIAN_POINT('Ctrl Pts',(-38.8662627330518,88.3553690084551,110.07539618188));
#40080=CARTESIAN_POINT('Ctrl Pts',(-38.6597042316269,88.9473396517482,110.038209061269));
#40081=CARTESIAN_POINT('Ctrl Pts',(-38.2820086943977,89.3948822716282,110.001021940657));
#40082=CARTESIAN_POINT('Ctrl Pts',(-37.7472675318623,90.0285129006648,109.948372432926));
#40083=CARTESIAN_POINT('Ctrl Pts',(-36.8694841837922,90.3726392469423,109.895722925195));
#40084=CARTESIAN_POINT('Ctrl Pts',(-36.046588380208,90.2712568783045,109.843073417465));
#40085=CARTESIAN_POINT('Ctrl Pts',(-35.2236925766238,90.1698745096667,109.790423909734));
#40086=CARTESIAN_POINT('Ctrl Pts',(-34.4556843175256,89.6229834261135,109.737774402003));
#40087=CARTESIAN_POINT('Ctrl Pts',(-34.0907284734417,88.8785083553923,109.685124894272));
#40088=CARTESIAN_POINT('Ctrl Pts',(-33.7257726293578,88.134033284671,109.632475386541));
#40089=CARTESIAN_POINT('Ctrl Pts',(-33.7638692002882,87.1919742267815,109.57982587881));
#40090=CARTESIAN_POINT('Ctrl Pts',(-34.1877476743859,86.4793993885376,109.52717637108));
#40091=CARTESIAN_POINT('Ctrl Pts',(-34.6116261484836,85.7668245502937,109.474526863349));
#40092=CARTESIAN_POINT('Ctrl Pts',(-35.4212865257487,85.2837339316954,109.421877355618));
#40093=CARTESIAN_POINT('Ctrl Pts',(-36.2496816085953,85.2491291978299,109.369227847887));
#40094=CARTESIAN_POINT('Ctrl Pts',(-37.0780766914418,85.2145244639644,109.316578340156));
#40095=CARTESIAN_POINT('Ctrl Pts',(-37.9252064798698,85.6284056148317,109.263928832425));
#40096=CARTESIAN_POINT('Ctrl Pts',(-38.4070375210029,86.3031461724895,109.211279324695));
#40097=CARTESIAN_POINT('Ctrl Pts',(-38.7081154049386,86.7247658730955,109.178380650627));
#40098=CARTESIAN_POINT('Ctrl Pts',(-38.8665614956128,87.248238769901,109.14548197656));
#40099=CARTESIAN_POINT('Ctrl Pts',(-38.869486864403,87.7700835308745,109.112583302492));
#40100=CARTESIAN_POINT('Ctrl Pts',(-38.8745809434987,87.7704133464264,109.387416697508));
#40101=CARTESIAN_POINT('Ctrl Pts',(-38.8687151411856,87.062137413473,109.432300020937));
#40102=CARTESIAN_POINT('Ctrl Pts',(-38.5558233551588,86.3493210472154,109.477183344366));
#40103=CARTESIAN_POINT('Ctrl Pts',(-38.0266616336717,85.8807298777288,109.522066667795));
#40104=CARTESIAN_POINT('Ctrl Pts',(-37.4059387901335,85.3310581396386,109.574716175526));
#40105=CARTESIAN_POINT('Ctrl Pts',(-36.4876283909998,85.1174404127878,109.627365683257));
#40106=CARTESIAN_POINT('Ctrl Pts',(-35.6880324811944,85.33671705519,109.680015190988));
#40107=CARTESIAN_POINT('Ctrl Pts',(-34.888436571389,85.5559936975923,109.732664698718));
#40108=CARTESIAN_POINT('Ctrl Pts',(-34.2075551509121,86.2081647092476,109.785314206449));
#40109=CARTESIAN_POINT('Ctrl Pts',(-33.9540554625385,86.9975782746064,109.83796371418));
#40110=CARTESIAN_POINT('Ctrl Pts',(-33.7005557741649,87.7869918399651,109.890613221911));
#40111=CARTESIAN_POINT('Ctrl Pts',(-33.8744378178946,88.7136479590273,109.943262729642));
#40112=CARTESIAN_POINT('Ctrl Pts',(-34.396874811042,89.3574611740643,109.995912237372));
#40113=CARTESIAN_POINT('Ctrl Pts',(-34.9193118041894,90.0012743891014,110.048561745103));
#40114=CARTESIAN_POINT('Ctrl Pts',(-35.7903037467545,90.3622447001133,110.101211252834));
#40115=CARTESIAN_POINT('Ctrl Pts',(-36.6149996877306,90.2767317046619,110.153860760565));
#40116=CARTESIAN_POINT('Ctrl Pts',(-37.4396956287066,90.1912187092105,110.206510268296));
#40117=CARTESIAN_POINT('Ctrl Pts',(-38.2180955680935,89.6592224072959,110.259159776027));
#40118=CARTESIAN_POINT('Ctrl Pts',(-38.5973237297961,88.9219152329815,110.311809283757));
#40119=CARTESIAN_POINT('Ctrl Pts',(-38.7788541420356,88.5689781654928,110.337011755008));
#40120=CARTESIAN_POINT('Ctrl Pts',(-38.8689190244798,88.1689965202894,110.362214226258));
#40121=CARTESIAN_POINT('Ctrl Pts',(-38.8685100522263,87.768840975972,110.387416697508));
#40122=CARTESIAN_POINT('Origin',(-36.3549260746835,87.7685555885722,114.));
#40123=CARTESIAN_POINT('',(-38.8735727384972,87.7664293773215,111.387416697508));
#40124=CARTESIAN_POINT('',(-38.8763918921078,87.7691165130487,111.112583302492));
#40125=CARTESIAN_POINT('',(-38.8724260746835,87.7685555885722,114.));
#40126=CARTESIAN_POINT('Ctrl Pts',(-38.8763918921078,87.7691165130487,111.112583302492));
#40127=CARTESIAN_POINT('Ctrl Pts',(-38.876486615945,87.8002064621293,111.110609402663));
#40128=CARTESIAN_POINT('Ctrl Pts',(-38.8759608143423,87.8312931336973,111.108635502833));
#40129=CARTESIAN_POINT('Ctrl Pts',(-38.8748045079704,87.8623563351577,111.106661603004));
#40130=CARTESIAN_POINT('Ctrl Pts',(-38.8439625369826,88.69090003387,111.054012095273));
#40131=CARTESIAN_POINT('Ctrl Pts',(-38.3645541170671,89.5027461541754,111.001362587543));
#40132=CARTESIAN_POINT('Ctrl Pts',(-37.6539117651349,89.9298566029362,110.948713079812));
#40133=CARTESIAN_POINT('Ctrl Pts',(-36.9432694132028,90.356967051697,110.896063572081));
#40134=CARTESIAN_POINT('Ctrl Pts',(-36.0013931292541,90.3993418289132,110.84341406435));
#40135=CARTESIAN_POINT('Ctrl Pts',(-35.2552682036472,90.0377709739024,110.790764556619));
#40136=CARTESIAN_POINT('Ctrl Pts',(-34.5091432780402,89.6762001188916,110.738115048888));
#40137=CARTESIAN_POINT('Ctrl Pts',(-33.9587697107751,88.9106836316539,110.685465541158));
#40138=CARTESIAN_POINT('Ctrl Pts',(-33.8536509892128,88.0882567702357,110.632816033427));
#40139=CARTESIAN_POINT('Ctrl Pts',(-33.7485322676505,87.2658299088175,110.580166525696));
#40140=CARTESIAN_POINT('Ctrl Pts',(-34.088668391791,86.3864926732189,110.527517017965));
#40141=CARTESIAN_POINT('Ctrl Pts',(-34.7198638219995,85.8488792280571,110.474867510234));
#40142=CARTESIAN_POINT('Ctrl Pts',(-35.351059252208,85.3112657828952,110.422218002503));
#40143=CARTESIAN_POINT('Ctrl Pts',(-36.2733139884845,85.1153761281701,110.369568494773));
#40144=CARTESIAN_POINT('Ctrl Pts',(-37.0685378709851,85.3500138584002,110.316918987042));
#40145=CARTESIAN_POINT('Ctrl Pts',(-37.8637617534856,85.5846515886302,110.264269479311));
#40146=CARTESIAN_POINT('Ctrl Pts',(-38.5319547822102,86.2498167038154,110.21161997158));
#40147=CARTESIAN_POINT('Ctrl Pts',(-38.7702018080721,87.0439667173058,110.158970463849));
#40148=CARTESIAN_POINT('Ctrl Pts',(-38.8401714602612,87.277196912012,110.14350807673));
#40149=CARTESIAN_POINT('Ctrl Pts',(-38.8730578128227,87.5215521912624,110.128045689611));
#40150=CARTESIAN_POINT('Ctrl Pts',(-38.8710621976983,87.7664319436008,110.112583302492));
#40151=CARTESIAN_POINT('Ctrl Pts',(-38.8685100522263,87.768840975972,110.387416697508));
#40152=CARTESIAN_POINT('Ctrl Pts',(-38.868064656366,87.3330470526798,110.414863733989));
#40153=CARTESIAN_POINT('Ctrl Pts',(-38.760312333685,86.8970468755525,110.442310770469));
#40154=CARTESIAN_POINT('Ctrl Pts',(-38.5465340171477,86.5213826498296,110.46975780695));
#40155=CARTESIAN_POINT('Ctrl Pts',(-38.1364597587785,85.800775287706,110.522407314681));
#40156=CARTESIAN_POINT('Ctrl Pts',(-37.336254858022,85.3021786101729,110.575056822411));
#40157=CARTESIAN_POINT('Ctrl Pts',(-36.5086800379385,85.2516238390558,110.627706330142));
#40158=CARTESIAN_POINT('Ctrl Pts',(-35.6811052178551,85.2010690679386,110.680355837873));
#40159=CARTESIAN_POINT('Ctrl Pts',(-34.8261604784448,85.5985562032374,110.733005345604));
#40160=CARTESIAN_POINT('Ctrl Pts',(-34.3314220163987,86.2638904966127,110.785654853335));
#40161=CARTESIAN_POINT('Ctrl Pts',(-33.8366835543527,86.9292247899879,110.838304361066));
#40162=CARTESIAN_POINT('Ctrl Pts',(-33.702151369671,87.8624062414395,110.890953868796));
#40163=CARTESIAN_POINT('Ctrl Pts',(-33.9888135824423,88.6403912306986,110.943603376527));
#40164=CARTESIAN_POINT('Ctrl Pts',(-34.2754757952136,89.4183762199577,110.996252884258));
#40165=CARTESIAN_POINT('Ctrl Pts',(-34.9833324054377,90.0411647470242,111.048902391989));
#40166=CARTESIAN_POINT('Ctrl Pts',(-35.7914873831277,90.2264251037659,111.10155189972));
#40167=CARTESIAN_POINT('Ctrl Pts',(-36.5996423608176,90.4116854605075,111.154201407451));
#40168=CARTESIAN_POINT('Ctrl Pts',(-37.5080957059732,90.1594176469243,111.206850915181));
#40169=CARTESIAN_POINT('Ctrl Pts',(-38.1050139092408,89.5839834401221,111.259500422912));
#40170=CARTESIAN_POINT('Ctrl Pts',(-38.5884344012918,89.1179619888201,111.302139181111));
#40171=CARTESIAN_POINT('Ctrl Pts',(-38.867527069726,88.4399840776712,111.344777939309));
#40172=CARTESIAN_POINT('Ctrl Pts',(-38.8735727384972,87.7664293773215,111.387416697508));
#40173=CARTESIAN_POINT('Origin',(-36.3549260746835,87.7685555885722,114.));
#40174=CARTESIAN_POINT('',(-38.8747249261259,87.7703594856308,112.387416697508));
#40175=CARTESIAN_POINT('',(-38.8695897820805,87.7701463237952,112.112583302492));
#40176=CARTESIAN_POINT('',(-38.8724260746835,87.7685555885722,114.));
#40177=CARTESIAN_POINT('Ctrl Pts',(-38.8695897820805,87.7701463237952,112.112583302492));
#40178=CARTESIAN_POINT('Ctrl Pts',(-38.8713915348065,88.0780025509154,112.093173115714));
#40179=CARTESIAN_POINT('Ctrl Pts',(-38.8190053186101,88.3852669963532,112.073762928937));
#40180=CARTESIAN_POINT('Ctrl Pts',(-38.7096476156592,88.6707043363187,112.054352742159));
#40181=CARTESIAN_POINT('Ctrl Pts',(-38.4130183615007,89.4449439461339,112.001703234428));
#40182=CARTESIAN_POINT('Ctrl Pts',(-37.6972224261715,90.05859102306,111.949053726697));
#40183=CARTESIAN_POINT('Ctrl Pts',(-36.8867550119788,90.2334579963873,111.896404218967));
#40184=CARTESIAN_POINT('Ctrl Pts',(-36.076287597786,90.4083249697147,111.843754711236));
#40185=CARTESIAN_POINT('Ctrl Pts',(-35.1711487047297,90.1444118394433,111.791105203505));
#40186=CARTESIAN_POINT('Ctrl Pts',(-34.5816692856989,89.5613596099067,111.738455695774));
#40187=CARTESIAN_POINT('Ctrl Pts',(-33.9921898666682,88.9783073803701,111.685806188043));
#40188=CARTESIAN_POINT('Ctrl Pts',(-33.7183699216629,88.0761160515683,111.633156680312));
#40189=CARTESIAN_POINT('Ctrl Pts',(-33.8843415588236,87.2637803429541,111.580507172582));
#40190=CARTESIAN_POINT('Ctrl Pts',(-34.0503131959844,86.4514446343399,111.527857664851));
#40191=CARTESIAN_POINT('Ctrl Pts',(-34.6560764153111,85.7289645459133,111.47520815712));
#40192=CARTESIAN_POINT('Ctrl Pts',(-35.4270176730479,85.4238654391534,111.422558649389));
#40193=CARTESIAN_POINT('Ctrl Pts',(-36.1979589307848,85.1187663323936,111.369909141658));
#40194=CARTESIAN_POINT('Ctrl Pts',(-37.1340782269316,85.2310482073005,111.317259633927));
#40195=CARTESIAN_POINT('Ctrl Pts',(-37.811000113975,85.7098097833135,111.264610126197));
#40196=CARTESIAN_POINT('Ctrl Pts',(-38.462543302245,86.1706219532658,111.213934518295));
#40197=CARTESIAN_POINT('Ctrl Pts',(-38.8739600625095,86.9709493285109,111.163258910394));
#40198=CARTESIAN_POINT('Ctrl Pts',(-38.8763918921078,87.7691165130487,111.112583302492));
#40199=CARTESIAN_POINT('Ctrl Pts',(-38.8735727384972,87.7664293773215,111.387416697508));
#40200=CARTESIAN_POINT('Ctrl Pts',(-38.8749921437139,87.6082918591033,111.39742744704));
#40201=CARTESIAN_POINT('Ctrl Pts',(-38.8613606824198,87.4503981566214,111.407438196572));
#40202=CARTESIAN_POINT('Ctrl Pts',(-38.8317890222728,87.2955485572239,111.417448946105));
#40203=CARTESIAN_POINT('Ctrl Pts',(-38.6762628706579,86.4811484811489,111.470098453835));
#40204=CARTESIAN_POINT('Ctrl Pts',(-38.0798275060489,85.75094892902,111.522747961566));
#40205=CARTESIAN_POINT('Ctrl Pts',(-37.3128678311087,85.4359747637889,111.575397469297));
#40206=CARTESIAN_POINT('Ctrl Pts',(-36.5459081561684,85.1210005985578,111.628046977028));
#40207=CARTESIAN_POINT('Ctrl Pts',(-35.6084241708969,85.2212518202244,111.680696484759));
#40208=CARTESIAN_POINT('Ctrl Pts',(-34.9254099838746,85.6912810619469,111.73334599249));
#40209=CARTESIAN_POINT('Ctrl Pts',(-34.2423957968523,86.1613103036694,111.78599550022));
#40210=CARTESIAN_POINT('Ctrl Pts',(-33.8138514080791,87.0011175654478,111.838645007951));
#40211=CARTESIAN_POINT('Ctrl Pts',(-33.8340508994108,87.8299889959469,111.891294515682));
#40212=CARTESIAN_POINT('Ctrl Pts',(-33.8542503907425,88.6588604264459,111.943944023413));
#40213=CARTESIAN_POINT('Ctrl Pts',(-34.3231937621791,89.4767960256657,111.996593531144));
#40214=CARTESIAN_POINT('Ctrl Pts',(-35.0282926674139,89.912997127893,112.049243038875));
#40215=CARTESIAN_POINT('Ctrl Pts',(-35.7333915726487,90.3491982301204,112.101892546605));
#40216=CARTESIAN_POINT('Ctrl Pts',(-36.6746460116818,90.4036648353553,112.154542054336));
#40217=CARTESIAN_POINT('Ctrl Pts',(-37.4253525980572,90.0517053363782,112.207191562067));
#40218=CARTESIAN_POINT('Ctrl Pts',(-38.1760591844327,89.699745837401,112.259841069798));
#40219=CARTESIAN_POINT('Ctrl Pts',(-38.7362179181505,88.9413602342117,112.312490577529));
#40220=CARTESIAN_POINT('Ctrl Pts',(-38.8518893555087,88.1203511073884,112.365140085259));
#40221=CARTESIAN_POINT('Ctrl Pts',(-38.8682033273407,88.0045583060305,112.372565622676));
#40222=CARTESIAN_POINT('Ctrl Pts',(-38.875675787902,87.8875198299491,112.379991160092));
#40223=CARTESIAN_POINT('Ctrl Pts',(-38.8747249261259,87.7703594856308,112.387416697508));
#40224=CARTESIAN_POINT('Origin',(-36.3549260746835,87.7685555885722,114.));
#40225=CARTESIAN_POINT('',(-38.8685312481293,87.7689269147315,113.387416697508));
#40226=CARTESIAN_POINT('',(-38.8709179607018,87.766461971973,113.112583302492));
#40227=CARTESIAN_POINT('',(-38.8724260746835,87.7685555885722,114.));
#40228=CARTESIAN_POINT('Ctrl Pts',(-38.8709179607018,87.766461971973,113.112583302492));
#40229=CARTESIAN_POINT('Ctrl Pts',(-38.8662498737967,88.3500889811953,113.075736828766));
#40230=CARTESIAN_POINT('Ctrl Pts',(-38.6637922635731,88.9366381474527,113.03889035504));
#40231=CARTESIAN_POINT('Ctrl Pts',(-38.2924116092779,89.3824749489596,113.002043881314));
#40232=CARTESIAN_POINT('Ctrl Pts',(-37.761750011244,90.0195260899217,112.949394373583));
#40233=CARTESIAN_POINT('Ctrl Pts',(-36.8861943918917,90.3692815952011,112.896744865852));
#40234=CARTESIAN_POINT('Ctrl Pts',(-36.0626645768443,90.2731851251457,112.844095358121));
#40235=CARTESIAN_POINT('Ctrl Pts',(-35.2391347617969,90.1770886550904,112.791445850391));
#40236=CARTESIAN_POINT('Ctrl Pts',(-34.4676307510543,89.6351402097004,112.73879634266));
#40237=CARTESIAN_POINT('Ctrl Pts',(-34.0979021557698,88.8930238753848,112.686146834929));
#40238=CARTESIAN_POINT('Ctrl Pts',(-33.7281735604853,88.1509075410691,112.633497327198));
#40239=CARTESIAN_POINT('Ctrl Pts',(-33.7602203806589,87.2086233178279,112.580847819467));
#40240=CARTESIAN_POINT('Ctrl Pts',(-34.1795146776949,86.4933414291279,112.528198311736));
#40241=CARTESIAN_POINT('Ctrl Pts',(-34.5988089747308,85.7780595404278,112.475548804006));
#40242=CARTESIAN_POINT('Ctrl Pts',(-35.4053507486292,85.289779986269,112.422899296275));
#40243=CARTESIAN_POINT('Ctrl Pts',(-36.2335065511227,85.2498568773537,112.370249788544));
#40244=CARTESIAN_POINT('Ctrl Pts',(-37.0616623536162,85.2099337684384,112.317600280813));
#40245=CARTESIAN_POINT('Ctrl Pts',(-37.9114321847049,85.6183671047667,112.264950773082));
#40246=CARTESIAN_POINT('Ctrl Pts',(-38.3975858137553,86.289999844283,112.212301265352));
#40247=CARTESIAN_POINT('Ctrl Pts',(-38.70451017459,86.7140231097153,112.179061944398));
#40248=CARTESIAN_POINT('Ctrl Pts',(-38.8665043384509,87.2429524303057,112.145822623445));
#40249=CARTESIAN_POINT('Ctrl Pts',(-38.8695897820805,87.7701463237952,112.112583302492));
#40250=CARTESIAN_POINT('Ctrl Pts',(-38.8747249261259,87.7703594856308,112.387416697508));
#40251=CARTESIAN_POINT('Ctrl Pts',(-38.8689338645059,87.0568143727958,112.432640667823));
#40252=CARTESIAN_POINT('Ctrl Pts',(-38.5507039652186,86.3387489093515,112.477864638137));
#40253=CARTESIAN_POINT('Ctrl Pts',(-38.0145054479413,85.8700345808651,112.523088608452));
#40254=CARTESIAN_POINT('Ctrl Pts',(-37.3902659620173,85.3243598316224,112.575738116183));
#40255=CARTESIAN_POINT('Ctrl Pts',(-36.4706028491709,85.1166429835945,112.628387623914));
#40256=CARTESIAN_POINT('Ctrl Pts',(-35.6724313964662,85.3410493111235,112.681037131644));
#40257=CARTESIAN_POINT('Ctrl Pts',(-34.8742599437615,85.5654556386525,112.733686639375));
#40258=CARTESIAN_POINT('Ctrl Pts',(-34.1975801511987,86.2219851417385,112.786336147106));
#40259=CARTESIAN_POINT('Ctrl Pts',(-33.9491545125933,87.0130101538787,112.838985654837));
#40260=CARTESIAN_POINT('Ctrl Pts',(-33.700728873988,87.8040351660187,112.891635162568));
#40261=CARTESIAN_POINT('Ctrl Pts',(-33.88055738934,88.7295556872129,112.944284670298));
#40262=CARTESIAN_POINT('Ctrl Pts',(-34.4071175358331,89.3700010633948,112.996934178029));
#40263=CARTESIAN_POINT('Ctrl Pts',(-34.9336776823263,90.0104464395768,113.04958368576));
#40264=CARTESIAN_POINT('Ctrl Pts',(-35.8069694599605,90.3658166707465,113.102233193491));
#40265=CARTESIAN_POINT('Ctrl Pts',(-36.6310993213297,90.2750100666518,113.154882701222));
#40266=CARTESIAN_POINT('Ctrl Pts',(-37.455229182699,90.1842034625571,113.207532208953));
#40267=CARTESIAN_POINT('Ctrl Pts',(-38.2301971278032,89.6472200231979,113.260181716683));
#40268=CARTESIAN_POINT('Ctrl Pts',(-38.6046832235218,88.9074930250012,113.312831224414));
#40269=CARTESIAN_POINT('Ctrl Pts',(-38.7815207276128,88.5581837246951,113.337693048779));
#40270=CARTESIAN_POINT('Ctrl Pts',(-38.8690564351314,88.1636654740321,113.362554873143));
#40271=CARTESIAN_POINT('Ctrl Pts',(-38.8685312481293,87.7689269147315,113.387416697508));
#40272=CARTESIAN_POINT('Origin',(-36.3549260746835,87.7685555885722,114.));
#40273=CARTESIAN_POINT('',(-38.8734136832049,87.7664022272136,114.387416697508));
#40274=CARTESIAN_POINT('',(-38.8764404125238,87.769021583458,114.112583302492));
#40275=CARTESIAN_POINT('',(-38.8724260746835,87.7685555885722,114.));
#40276=CARTESIAN_POINT('Ctrl Pts',(-38.8764404125238,87.769021583458,114.112583302492));
#40277=CARTESIAN_POINT('Ctrl Pts',(-38.8765065000921,87.7947448392147,114.110950049548));
#40278=CARTESIAN_POINT('Ctrl Pts',(-38.8761465565816,87.8204662008222,114.109316796605));
#40279=CARTESIAN_POINT('Ctrl Pts',(-38.8753548555647,87.8461742661021,114.107683543661));
#40280=CARTESIAN_POINT('Ctrl Pts',(-38.8498335981424,88.6748989207666,114.05503403593));
#40281=CARTESIAN_POINT('Ctrl Pts',(-38.3756479237925,89.489806585655,114.002384528199));
#40282=CARTESIAN_POINT('Ctrl Pts',(-37.6677626971288,89.9214712630384,113.949735020469));
#40283=CARTESIAN_POINT('Ctrl Pts',(-36.9598774704652,90.3531359404218,113.897085512738));
#40284=CARTESIAN_POINT('Ctrl Pts',(-36.0182926914878,90.4015576303001,113.844436005007));
#40285=CARTESIAN_POINT('Ctrl Pts',(-35.2698615012428,90.0447850959066,113.791786497276));
#40286=CARTESIAN_POINT('Ctrl Pts',(-34.5214303109978,89.6880125615131,113.739136989545));
#40287=CARTESIAN_POINT('Ctrl Pts',(-33.9661527094851,88.9260458028477,113.686487481814));
#40288=CARTESIAN_POINT('Ctrl Pts',(-33.8557553533482,88.1043108628658,113.633837974084));
#40289=CARTESIAN_POINT('Ctrl Pts',(-33.7453579972113,87.2825759228839,113.581188466353));
#40290=CARTESIAN_POINT('Ctrl Pts',(-34.0798408864501,86.4010728015853,113.528538958622));
#40291=CARTESIAN_POINT('Ctrl Pts',(-34.7075712896468,85.8594175341581,113.475889450891));
#40292=CARTESIAN_POINT('Ctrl Pts',(-35.3353016928435,85.3177622667309,113.42323994316));
#40293=CARTESIAN_POINT('Ctrl Pts',(-36.2562796099981,85.1159548531751,113.37059043543));
#40294=CARTESIAN_POINT('Ctrl Pts',(-37.0529937075072,85.3454816155785,113.317940927699));
#40295=CARTESIAN_POINT('Ctrl Pts',(-37.8497078050162,85.575008377982,113.265291419968));
#40296=CARTESIAN_POINT('Ctrl Pts',(-38.5221580828798,86.2358693163448,113.212641912237));
#40297=CARTESIAN_POINT('Ctrl Pts',(-38.7654994334537,87.0284731738487,113.159992404506));
#40298=CARTESIAN_POINT('Ctrl Pts',(-38.83853965365,87.2663775010168,113.144189370502));
#40299=CARTESIAN_POINT('Ctrl Pts',(-38.872920050146,87.5161509777269,113.128386336497));
#40300=CARTESIAN_POINT('Ctrl Pts',(-38.8709179607018,87.766461971973,113.112583302492));
#40301=CARTESIAN_POINT('Ctrl Pts',(-38.8685312481293,87.7689269147315,113.387416697508));
#40302=CARTESIAN_POINT('Ctrl Pts',(-38.8679442545962,87.3277336242702,113.415204380874));
#40303=CARTESIAN_POINT('Ctrl Pts',(-38.7573498896077,86.8862651200007,113.442992064241));
#40304=CARTESIAN_POINT('Ctrl Pts',(-38.538480742133,86.5073360489567,113.470779747607));
#40305=CARTESIAN_POINT('Ctrl Pts',(-38.1237879186926,85.7893766281432,113.523429255338));
#40306=CARTESIAN_POINT('Ctrl Pts',(-37.320398025479,85.2959283435506,113.576078763068));
#40307=CARTESIAN_POINT('Ctrl Pts',(-36.4925156535809,85.2506884712233,113.628728270799));
#40308=CARTESIAN_POINT('Ctrl Pts',(-35.6646332816829,85.205448598896,113.68137777853));
#40309=CARTESIAN_POINT('Ctrl Pts',(-34.8122584311004,85.608417138834,113.734027286261));
#40310=CARTESIAN_POINT('Ctrl Pts',(-34.3218022784405,86.2769144313234,113.786676793992));
#40311=CARTESIAN_POINT('Ctrl Pts',(-33.8313461257806,86.9454117238129,113.839326301722));
#40312=CARTESIAN_POINT('Ctrl Pts',(-33.7028086710432,87.8794377688538,113.891975809453));
#40313=CARTESIAN_POINT('Ctrl Pts',(-33.9944604146885,88.655566062486,113.944625317184));
#40314=CARTESIAN_POINT('Ctrl Pts',(-34.2861121583339,89.4316943561181,113.997274824915));
#40315=CARTESIAN_POINT('Ctrl Pts',(-34.997953100362,90.0499248983415,114.049924332646));
#40316=CARTESIAN_POINT('Ctrl Pts',(-35.8072809745362,90.229992274155,114.102573840377));
#40317=CARTESIAN_POINT('Ctrl Pts',(-36.6166088487104,90.4100596499686,114.155223348107));
#40318=CARTESIAN_POINT('Ctrl Pts',(-37.5234236550307,90.1519638593725,114.207872855838));
#40319=CARTESIAN_POINT('Ctrl Pts',(-38.1166346908146,89.572708704219,114.260522363569));
#40320=CARTESIAN_POINT('Ctrl Pts',(-38.5932147673457,89.1073406488029,114.302820474882));
#40321=CARTESIAN_POINT('Ctrl Pts',(-38.8673836169466,88.4346847125397,114.345118586195));
#40322=CARTESIAN_POINT('Ctrl Pts',(-38.8734136832049,87.7664022272136,114.387416697508));
#40323=CARTESIAN_POINT('Origin',(-36.3549260746835,87.7685555885722,114.));
#40324=CARTESIAN_POINT('',(-38.8748657309868,87.7703023244941,115.387416697508));
#40325=CARTESIAN_POINT('',(-38.8696970038573,87.7702068964603,115.112583302492));
#40326=CARTESIAN_POINT('',(-38.8724260746835,87.7685555885722,114.));
#40327=CARTESIAN_POINT('Ctrl Pts',(-38.8696970038573,87.7702068964603,115.112583302492));
#40328=CARTESIAN_POINT('Ctrl Pts',(-38.8715395686952,88.0726278474952,115.0935137626));
#40329=CARTESIAN_POINT('Ctrl Pts',(-38.8210274128864,88.3744540515915,115.074444222708));
#40330=CARTESIAN_POINT('Ctrl Pts',(-38.7153917691555,88.6555660754418,115.055374682816));
#40331=CARTESIAN_POINT('Ctrl Pts',(-38.4237400212503,89.4316943804101,115.002725175085));
#40332=CARTESIAN_POINT('Ctrl Pts',(-37.7118990688249,90.0499249316633,114.950075667354));
#40333=CARTESIAN_POINT('Ctrl Pts',(-36.9025711828297,90.2299923101069,114.897426159623));
#40334=CARTESIAN_POINT('Ctrl Pts',(-36.0932432968344,90.4100596885505,114.844776651893));
#40335=CARTESIAN_POINT('Ctrl Pts',(-35.1864284772691,90.1519638941845,114.792127144162));
#40336=CARTESIAN_POINT('Ctrl Pts',(-34.5932174328208,89.5727087305704,114.739477636431));
#40337=CARTESIAN_POINT('Ctrl Pts',(-34.0000063883724,88.9934535669563,114.6868281287));
#40338=CARTESIAN_POINT('Ctrl Pts',(-33.720399119041,88.093039034094,114.634178620969));
#40339=CARTESIAN_POINT('Ctrl Pts',(-33.8811513284425,87.2796543680216,114.581529113239));
#40340=CARTESIAN_POINT('Ctrl Pts',(-34.0419035378441,86.4662697019493,114.528879605508));
#40341=CARTESIAN_POINT('Ctrl Pts',(-34.6430152259786,85.7399149026668,114.476230097777));
#40342=CARTESIAN_POINT('Ctrl Pts',(-35.411981550023,85.4298718728877,114.423580590046));
#40343=CARTESIAN_POINT('Ctrl Pts',(-36.1809478740675,85.1198288431085,114.370931082315));
#40344=CARTESIAN_POINT('Ctrl Pts',(-37.117768834022,85.2260975828327,114.318281574584));
#40345=CARTESIAN_POINT('Ctrl Pts',(-37.7977508937519,85.700502774915,114.265632066854));
#40346=CARTESIAN_POINT('Ctrl Pts',(-38.4566390677353,86.1601913303212,114.214615812066));
#40347=CARTESIAN_POINT('Ctrl Pts',(-38.8743761026231,86.9655305046608,114.163599557279));
#40348=CARTESIAN_POINT('Ctrl Pts',(-38.8764404125238,87.769021583458,114.112583302492));
#40349=CARTESIAN_POINT('Ctrl Pts',(-38.8734136832049,87.7664022272136,114.387416697508));
#40350=CARTESIAN_POINT('Ctrl Pts',(-38.8748893899049,87.6028569361835,114.397768093926));
#40351=CARTESIAN_POINT('Ctrl Pts',(-38.8603062050893,87.4395735721051,114.408119490344));
#40352=CARTESIAN_POINT('Ctrl Pts',(-38.8287007847925,87.2796543751627,114.418470886762));
#40353=CARTESIAN_POINT('Ctrl Pts',(-38.667948577739,86.4662697209706,114.471120394492));
#40354=CARTESIAN_POINT('Ctrl Pts',(-38.0668368983844,85.7399149322973,114.523769902223));
#40355=CARTESIAN_POINT('Ctrl Pts',(-37.2978705855715,85.4298719070465,114.576419409954));
#40356=CARTESIAN_POINT('Ctrl Pts',(-36.5289042727585,85.1198288817958,114.629068917685));
#40357=CARTESIAN_POINT('Ctrl Pts',(-35.5920833264873,85.2260976199678,114.681718425416));
#40358=CARTESIAN_POINT('Ctrl Pts',(-34.9121012766892,85.7005028051209,114.734367933147));
#40359=CARTESIAN_POINT('Ctrl Pts',(-34.2321192268912,86.174907990274,114.787017440877));
#40360=CARTESIAN_POINT('Ctrl Pts',(-33.8089760735663,87.0174496224082,114.839666948608));
#40361=CARTESIAN_POINT('Ctrl Pts',(-33.8344973306158,87.8461742649683,114.892316456339));
#40362=CARTESIAN_POINT('Ctrl Pts',(-33.8600185876653,88.6748989075284,114.94496596407));
#40363=CARTESIAN_POINT('Ctrl Pts',(-34.3342042550892,89.4898065605143,114.997615471801));
#40364=CARTESIAN_POINT('Ctrl Pts',(-35.0420894714134,89.9214712315928,115.050264979531));
#40365=CARTESIAN_POINT('Ctrl Pts',(-35.7499746877377,90.3531359026713,115.102914487262));
#40366=CARTESIAN_POINT('Ctrl Pts',(-36.6915594529623,90.4015575918424,115.155563994993));
#40367=CARTESIAN_POINT('Ctrl Pts',(-37.4399906322757,90.04478506266,115.208213502724));
#40368=CARTESIAN_POINT('Ctrl Pts',(-38.1884218115891,89.6880125334775,115.260863010455));
#40369=CARTESIAN_POINT('Ctrl Pts',(-38.7436994049914,88.9260457859415,115.313512518185));
#40370=CARTESIAN_POINT('Ctrl Pts',(-38.8540967595159,88.1043108579619,115.366162025916));
#40371=CARTESIAN_POINT('Ctrl Pts',(-38.8689526091787,87.9937323879857,115.373246916447));
#40372=CARTESIAN_POINT('Ctrl Pts',(-38.8757524344211,87.8820716179226,115.380331806977));
#40373=CARTESIAN_POINT('Ctrl Pts',(-38.8748657309868,87.7703023244941,115.387416697508));
#40374=CARTESIAN_POINT('Origin',(-36.3549260746835,87.7685555885722,114.));
#40375=CARTESIAN_POINT('',(-38.8685579872896,87.7690123127748,116.387416697508));
#40376=CARTESIAN_POINT('',(-38.8707764324224,87.7664952479985,116.112583302492));
#40377=CARTESIAN_POINT('',(-38.8724260746835,87.7685555885722,114.));
#40378=CARTESIAN_POINT('Ctrl Pts',(-38.8707764324224,87.7664952479985,116.112583302492));
#40379=CARTESIAN_POINT('Ctrl Pts',(-38.8662438736391,88.3448089996547,116.076077475652));
#40380=CARTESIAN_POINT('Ctrl Pts',(-38.6678380330352,88.9259325787823,116.039571648811));
#40381=CARTESIAN_POINT('Ctrl Pts',(-38.3027346419836,89.3700010867857,116.003065821971));
#40382=CARTESIAN_POINT('Ctrl Pts',(-37.7761744877995,90.010446472322,115.95041631424));
#40383=CARTESIAN_POINT('Ctrl Pts',(-36.9028826974099,90.3658167086822,115.897766806509));
#40384=CARTESIAN_POINT('Ctrl Pts',(-36.0787528240034,90.2750101032611,115.845117298778));
#40385=CARTESIAN_POINT('Ctrl Pts',(-35.2546229505969,90.18420349784,115.792467791047));
#40386=CARTESIAN_POINT('Ctrl Pts',(-34.4796549941735,89.6472200506376,115.739818283317));
#40387=CARTESIAN_POINT('Ctrl Pts',(-34.1051688929851,88.9074930416363,115.687168775586));
#40388=CARTESIAN_POINT('Ctrl Pts',(-33.7306827917968,88.1677660326351,115.634519267855));
#40389=CARTESIAN_POINT('Ctrl Pts',(-33.7566785458437,87.2252954618351,115.581869760124));
#40390=CARTESIAN_POINT('Ctrl Pts',(-34.1713713753411,86.5073360305352,115.529220252393));
#40391=CARTESIAN_POINT('Ctrl Pts',(-34.5860642048385,85.7893765992352,115.476570744662));
#40392=CARTESIAN_POINT('Ctrl Pts',(-35.3894541097865,85.2959283074353,115.423921236932));
#40393=CARTESIAN_POINT('Ctrl Pts',(-36.2173364937766,85.2506884344473,115.371271729201));
#40394=CARTESIAN_POINT('Ctrl Pts',(-37.0452188777668,85.2054485614592,115.31862222147));
#40395=CARTESIAN_POINT('Ctrl Pts',(-37.897593740799,85.608417107283,115.265972713739));
#40396=CARTESIAN_POINT('Ctrl Pts',(-38.3880499006225,86.2769144095366,115.213323206008));
#40397=CARTESIAN_POINT('Ctrl Pts',(-38.7008638809052,86.7032834085547,115.17974323817));
#40398=CARTESIAN_POINT('Ctrl Pts',(-38.8664523913314,87.2376672616802,115.146163270331));
#40399=CARTESIAN_POINT('Ctrl Pts',(-38.8696970038573,87.7702068964603,115.112583302492));
#40400=CARTESIAN_POINT('Ctrl Pts',(-38.8748657309868,87.7703023244941,115.387416697508));
#40401=CARTESIAN_POINT('Ctrl Pts',(-38.8691631301662,87.0514873974544,115.432981314708));
#40402=CARTESIAN_POINT('Ctrl Pts',(-38.545539383395,86.3281838547981,115.478545931909));
#40403=CARTESIAN_POINT('Ctrl Pts',(-38.0022808356591,85.8594175620432,115.524110549109));
#40404=CARTESIAN_POINT('Ctrl Pts',(-37.3745504416311,85.3177623025274,115.57676005684));
#40405=CARTESIAN_POINT('Ctrl Pts',(-36.4535725379283,85.115954891919,115.62940956457));
#40406=CARTESIAN_POINT('Ctrl Pts',(-35.656858452056,85.34548165097,115.682059072301));
#40407=CARTESIAN_POINT('Ctrl Pts',(-34.8601443661838,85.5750084100209,115.734708580032));
#40408=CARTESIAN_POINT('Ctrl Pts',(-34.187694098142,86.2358693387312,115.787358087763));
#40409=CARTESIAN_POINT('Ctrl Pts',(-33.9443527511223,87.0284731846582,115.840007595494));
#40410=CARTESIAN_POINT('Ctrl Pts',(-33.7010114041026,87.8210770305853,115.892657103225));
#40411=CARTESIAN_POINT('Ctrl Pts',(-33.8867789781049,88.7454237937291,115.945306610955));
#40412=CARTESIAN_POINT('Ctrl Pts',(-34.417440568388,89.3824749253865,115.997956118686));
#40413=CARTESIAN_POINT('Ctrl Pts',(-34.9481021586711,90.0195260570439,116.050605626417));
#40414=CARTESIAN_POINT('Ctrl Pts',(-35.8236577652349,90.3692815572148,116.103255134148));
#40415=CARTESIAN_POINT('Ctrl Pts',(-36.6471875682538,90.2731850885631,116.155904641879));
#40416=CARTESIAN_POINT('Ctrl Pts',(-37.4707173712728,90.1770886199114,116.20855414961));
#40417=CARTESIAN_POINT('Ctrl Pts',(-38.2422213707468,89.6351401824371,116.26120365734));
#40418=CARTESIAN_POINT('Ctrl Pts',(-38.611949960631,88.8930238589608,116.313853165071));
#40419=CARTESIAN_POINT('Ctrl Pts',(-38.7841487287174,88.5473878433112,116.33837434255));
#40420=CARTESIAN_POINT('Ctrl Pts',(-38.8691954955822,88.1583319681357,116.362895520029));
#40421=CARTESIAN_POINT('Ctrl Pts',(-38.8685579872896,87.7690123127748,116.387416697508));
#40422=CARTESIAN_POINT('Origin',(-36.3549260746835,87.7685555885722,114.));
#40423=CARTESIAN_POINT('',(-38.8732537926193,87.7663787382843,117.387416697508));
#40424=CARTESIAN_POINT('',(-38.8764804707602,87.7689256098953,117.112583302492));
#40425=CARTESIAN_POINT('',(-38.8724260746835,87.7685555885722,114.));
#40426=CARTESIAN_POINT('Ctrl Pts',(-38.8764804707602,87.7689256098953,117.112583302492));
#40427=CARTESIAN_POINT('Ctrl Pts',(-38.8765226439062,87.789282907905,117.111290696434));
#40428=CARTESIAN_POINT('Ctrl Pts',(-38.876297207562,87.8096392482103,117.109998090376));
#40429=CARTESIAN_POINT('Ctrl Pts',(-38.8758012867762,87.8299889968442,117.108705484318));
#40430=CARTESIAN_POINT('Ctrl Pts',(-38.8556017951495,88.6588604394498,117.056055976587));
#40431=CARTESIAN_POINT('Ctrl Pts',(-38.3866584168635,89.4767960506164,117.003406468856));
#40432=CARTESIAN_POINT('Ctrl Pts',(-37.6815595013299,89.9129971592149,116.950756961126));
#40433=CARTESIAN_POINT('Ctrl Pts',(-36.9764605857964,90.3491982678134,116.898107453395));
#40434=CARTESIAN_POINT('Ctrl Pts',(-36.0352061330153,90.4036648738438,116.845457945664));
#40435=CARTESIAN_POINT('Ctrl Pts',(-35.2844995356751,90.0517053697259,116.792808437933));
#40436=CARTESIAN_POINT('Ctrl Pts',(-34.5337929383348,89.699745865608,116.740158930202));
#40437=CARTESIAN_POINT('Ctrl Pts',(-33.9736341964353,88.9413602513417,116.687509422471));
#40438=CARTESIAN_POINT('Ctrl Pts',(-33.8579627573876,88.1203511125267,116.634859914741));
#40439=CARTESIAN_POINT('Ctrl Pts',(-33.74229131834,87.2993419737117,116.58221040701));
#40440=CARTESIAN_POINT('Ctrl Pts',(-34.0711071821443,86.4157093103479,116.529560899279));
#40441=CARTESIAN_POINT('Ctrl Pts',(-34.6953466771859,85.8700345531351,116.476911391548));
#40442=CARTESIAN_POINT('Ctrl Pts',(-35.3195861722276,85.3243597959224,116.424261883817));
#40443=CARTESIAN_POINT('Ctrl Pts',(-36.2392492985068,85.1166429448606,116.371612376086));
#40444=CARTESIAN_POINT('Ctrl Pts',(-37.0374207628696,85.3410492756673,116.318962868356));
#40445=CARTESIAN_POINT('Ctrl Pts',(-37.8355922272323,85.5654556064741,116.266313360625));
#40446=CARTESIAN_POINT('Ctrl Pts',(-38.5122720296786,86.2219851191493,116.213663852894));
#40447=CARTESIAN_POINT('Ctrl Pts',(-38.7606976719125,87.0130101428432,116.161014345163));
#40448=CARTESIAN_POINT('Ctrl Pts',(-38.8368713051726,87.2555585750928,116.144870664273));
#40449=CARTESIAN_POINT('Ctrl Pts',(-38.8727808297734,87.5107521661593,116.128726983382));
#40450=CARTESIAN_POINT('Ctrl Pts',(-38.8707764324224,87.7664952479985,116.112583302492));
#40451=CARTESIAN_POINT('Ctrl Pts',(-38.8685579872896,87.7690123127748,116.387416697508));
#40452=CARTESIAN_POINT('Ctrl Pts',(-38.8678266992505,87.32242234584,116.41554502776));
#40453=CARTESIAN_POINT('Ctrl Pts',(-38.754348048844,86.8754852846444,116.443673358012));
#40454=CARTESIAN_POINT('Ctrl Pts',(-38.5303374398981,86.4933414477537,116.471801688264));
#40455=CARTESIAN_POINT('Ctrl Pts',(-38.1110431489864,85.7780595695012,116.524451195994));
#40456=CARTESIAN_POINT('Ctrl Pts',(-37.3045013868685,85.2897800224741,116.577100703725));
#40457=CARTESIAN_POINT('Ctrl Pts',(-36.476345596471,85.2498569141419,116.629750211456));
#40458=CARTESIAN_POINT('Ctrl Pts',(-35.6481898060736,85.2099338058097,116.682399719187));
#40459=CARTESIAN_POINT('Ctrl Pts',(-34.7984199873967,85.6183671361723,116.735049226918));
#40460=CARTESIAN_POINT('Ctrl Pts',(-34.3122663654471,86.2899998658787,116.787698734649));
#40461=CARTESIAN_POINT('Ctrl Pts',(-33.8261127434974,86.961632595585,116.840348242379));
#40462=CARTESIAN_POINT('Ctrl Pts',(-33.703575318275,87.8964647246352,116.89299775011));
#40463=CARTESIAN_POINT('Ctrl Pts',(-34.0002045681009,88.6707043231418,116.945647257841));
#40464=CARTESIAN_POINT('Ctrl Pts',(-34.2968338179268,89.4449439216484,116.998296765572));
#40465=CARTESIAN_POINT('Ctrl Pts',(-35.012629742801,90.0585909896116,117.050946273303));
#40466=CARTESIAN_POINT('Ctrl Pts',(-35.823097145156,90.2334579603849,117.103595781034));
#40467=CARTESIAN_POINT('Ctrl Pts',(-36.6335645475111,90.4083249311581,117.156245288764));
#40468=CARTESIAN_POINT('Ctrl Pts',(-37.5387034273469,90.1444118047415,117.208894796495));
#40469=CARTESIAN_POINT('Ctrl Pts',(-38.1281828377678,89.561359583721,117.261544304226));
#40470=CARTESIAN_POINT('Ctrl Pts',(-38.5979509791879,89.0967134003639,117.303501768653));
#40471=CARTESIAN_POINT('Ctrl Pts',(-38.867249456628,88.429387705517,117.345459233081));
#40472=CARTESIAN_POINT('Ctrl Pts',(-38.8732537926193,87.7663787382843,117.387416697508));
#40473=CARTESIAN_POINT('Origin',(-36.3549260746835,87.7685555885722,114.));
#40474=CARTESIAN_POINT('',(-38.8750030608581,87.7702419441723,118.387416697508));
#40475=CARTESIAN_POINT('',(-38.8698084321024,87.7702649945025,118.112583302492));
#40476=CARTESIAN_POINT('',(-38.8724260746835,87.7685555885722,114.));
#40477=CARTESIAN_POINT('Ctrl Pts',(-38.8698084321024,87.7702649945025,118.112583302492));
#40478=CARTESIAN_POINT('Ctrl Pts',(-38.8716871432184,88.0672505628736,118.093854409486));
#40479=CARTESIAN_POINT('Ctrl Pts',(-38.8230123182726,88.363640358852,118.075125516479));
#40480=CARTESIAN_POINT('Ctrl Pts',(-38.7210386014842,88.6403912434327,118.056396623473));
#40481=CARTESIAN_POINT('Ctrl Pts',(-38.434376384526,89.418376244055,118.003747115742));
#40482=CARTESIAN_POINT('Ctrl Pts',(-37.7265197639628,90.0411647802181,117.951097608011));
#40483=CARTESIAN_POINT('Ctrl Pts',(-36.9183647744689,90.2264251396656,117.89844810028));
#40484=CARTESIAN_POINT('Ctrl Pts',(-36.110209784975,90.4116854991132,117.84579859255));
#40485=CARTESIAN_POINT('Ctrl Pts',(-35.2017564265505,90.1594176818452,117.793149084819));
#40486=CARTESIAN_POINT('Ctrl Pts',(-34.6048382145644,89.5839834666382,117.740499577088));
#40487=CARTESIAN_POINT('Ctrl Pts',(-34.0079200025783,89.0085492514311,117.687850069357));
#40488=CARTESIAN_POINT('Ctrl Pts',(-33.7225369370307,88.1099486382851,117.635200561626));
#40489=CARTESIAN_POINT('Ctrl Pts',(-33.8780630909172,87.295548550315,117.582551053895));
#40490=CARTESIAN_POINT('Ctrl Pts',(-34.0335892448037,86.4811484623449,117.529901546165));
#40491=CARTESIAN_POINT('Ctrl Pts',(-34.6300246181243,85.7509488995507,117.477252038434));
#40492=CARTESIAN_POINT('Ctrl Pts',(-35.3969843042668,85.4359747297191,117.424602530703));
#40493=CARTESIAN_POINT('Ctrl Pts',(-36.1639439904093,85.1210005598875,117.371953022972));
#40494=CARTESIAN_POINT('Ctrl Pts',(-37.1014279893737,85.2212517830186,117.319303515241));
#40495=CARTESIAN_POINT('Ctrl Pts',(-37.7844421863721,85.6912810316064,117.266654007511));
#40496=CARTESIAN_POINT('Ctrl Pts',(-38.4506875981189,86.1497705207481,117.215297105838));
#40497=CARTESIAN_POINT('Ctrl Pts',(-38.8748048774098,86.9601039695085,117.163940204165));
#40498=CARTESIAN_POINT('Ctrl Pts',(-38.8764804707602,87.7689256098953,117.112583302492));
#40499=CARTESIAN_POINT('Ctrl Pts',(-38.8732537926193,87.7663787382843,117.387416697508));
#40500=CARTESIAN_POINT('Ctrl Pts',(-38.8747838808003,87.5974238053543,117.398108740811));
#40501=CARTESIAN_POINT('Ctrl Pts',(-38.8592160150071,87.4287491946892,117.408800784115));
#40502=CARTESIAN_POINT('Ctrl Pts',(-38.825510554458,87.263780350327,117.419492827418));
#40503=CARTESIAN_POINT('Ctrl Pts',(-38.6595389197215,86.4514446535778,117.472142335149));
#40504=CARTESIAN_POINT('Ctrl Pts',(-38.0537757092426,85.7289645757037,117.52479184288));
#40505=CARTESIAN_POINT('Ctrl Pts',(-37.2828344627662,85.4238654734001,117.577441350611));
#40506=CARTESIAN_POINT('Ctrl Pts',(-36.5118932162898,85.1187663710965,117.630090858342));
#40507=CARTESIAN_POINT('Ctrl Pts',(-35.5757739338159,85.2310482443633,117.682740366072));
#40508=CARTESIAN_POINT('Ctrl Pts',(-34.8988520566596,85.7098098133835,117.735389873803));
#40509=CARTESIAN_POINT('Ctrl Pts',(-34.2219301795033,86.1885713824036,117.788039381534));
#40510=CARTESIAN_POINT('Ctrl Pts',(-33.8042057076648,87.033812647177,117.840688889265));
#40511=CARTESIAN_POINT('Ctrl Pts',(-33.8350476782021,87.8623563337875,117.893338396996));
#40512=CARTESIAN_POINT('Ctrl Pts',(-33.8658896487394,88.690900020398,117.945987904727));
#40513=CARTESIAN_POINT('Ctrl Pts',(-34.3452980616525,89.5027461288456,117.998637412457));
#40514=CARTESIAN_POINT('Ctrl Pts',(-35.055940403205,89.929856571368,118.051286920188));
#40515=CARTESIAN_POINT('Ctrl Pts',(-35.7665827447574,90.3569670138905,118.103936427919));
#40516=CARTESIAN_POINT('Ctrl Pts',(-36.7084590149491,90.3993417904879,118.15658593565));
#40517=CARTESIAN_POINT('Ctrl Pts',(-37.4545839296581,90.0377709407583,118.209235443381));
#40518=CARTESIAN_POINT('Ctrl Pts',(-38.2007088443672,89.6762000910287,118.261884951112));
#40519=CARTESIAN_POINT('Ctrl Pts',(-38.7510824035936,88.9106836149721,118.314534458842));
#40520=CARTESIAN_POINT('Ctrl Pts',(-38.8562011236206,88.0882567655663,118.367183966573));
#40521=CARTESIAN_POINT('Ctrl Pts',(-38.8696665156073,87.9829063588563,118.373928210218));
#40522=CARTESIAN_POINT('Ctrl Pts',(-38.8758257923026,87.8766221189515,118.380672453863));
#40523=CARTESIAN_POINT('Ctrl Pts',(-38.8750030608581,87.7702419441723,118.387416697508));
#40524=CARTESIAN_POINT('Origin',(-36.3549260746835,87.7685555885722,114.));
#40525=CARTESIAN_POINT('',(-38.8685902376792,87.769097033614,119.387416697508));
#40526=CARTESIAN_POINT('',(-38.8706377933747,87.7665317068533,119.112583302492));
#40527=CARTESIAN_POINT('',(-38.8724260746835,87.7685555885722,114.));
#40528=CARTESIAN_POINT('Ctrl Pts',(-38.8706377933747,87.7665317068533,119.112583302492));
#40529=CARTESIAN_POINT('Ctrl Pts',(-38.866244579201,88.3395289437958,119.076418122537));
#40530=CARTESIAN_POINT('Ctrl Pts',(-38.6718416557376,88.9152230430577,119.040252942582));
#40531=CARTESIAN_POINT('Ctrl Pts',(-38.3129773669244,89.3574611972722,119.004087762628));
#40532=CARTESIAN_POINT('Ctrl Pts',(-37.7905403661463,90.0012744217129,118.951438254897));
#40533=CARTESIAN_POINT('Ctrl Pts',(-36.9195484108592,90.3622447379968,118.898788747166));
#40534=CARTESIAN_POINT('Ctrl Pts',(-36.0948524578377,90.2767317412963,118.846139239435));
#40535=CARTESIAN_POINT('Ctrl Pts',(-35.2701565048161,90.1912187445957,118.793489731704));
#40536=CARTESIAN_POINT('Ctrl Pts',(-34.4917565540599,89.6592224349109,118.740840223973));
#40537=CARTESIAN_POINT('Ctrl Pts',(-34.1125283868184,88.9219152498275,118.688190716243));
#40538=CARTESIAN_POINT('Ctrl Pts',(-33.7333002195769,88.1846080647441,118.635541208512));
#40539=CARTESIAN_POINT('Ctrl Pts',(-33.75324383585,87.2419900042621,118.582891700781));
#40540=CARTESIAN_POINT('Ctrl Pts',(-34.1633181002087,86.5213826316133,118.53024219305));
#40541=CARTESIAN_POINT('Ctrl Pts',(-34.5733923645675,85.8007752589644,118.477592685319));
#40542=CARTESIAN_POINT('Ctrl Pts',(-35.3735972770119,85.3021785741488,118.424943177589));
#40543=CARTESIAN_POINT('Ctrl Pts',(-36.2011721091829,85.2516238022933,118.372293669858));
#40544=CARTESIAN_POINT('Ctrl Pts',(-37.028746941354,85.2010690304378,118.319644162127));
#40545=CARTESIAN_POINT('Ctrl Pts',(-37.8836916932516,85.5985561715425,118.266994654396));
#40546=CARTESIAN_POINT('Ctrl Pts',(-38.3784301625238,86.2638904746356,118.214345146665));
#40547=CARTESIAN_POINT('Ctrl Pts',(-38.6971764097124,86.6925468767723,118.180424531941));
#40548=CARTESIAN_POINT('Ctrl Pts',(-38.8664058265174,87.2323830684335,118.146503917216));
#40549=CARTESIAN_POINT('Ctrl Pts',(-38.8698084321024,87.7702649945025,118.112583302492));
#40550=CARTESIAN_POINT('Ctrl Pts',(-38.8750030608581,87.7702419441723,118.387416697508));
#40551=CARTESIAN_POINT('Ctrl Pts',(-38.8694030697812,87.0461562981247,118.433321961594));
#40552=CARTESIAN_POINT('Ctrl Pts',(-38.5403294887911,86.3176260284683,118.47922722568));
#40553=CARTESIAN_POINT('Ctrl Pts',(-37.9899883034859,85.848879256096,118.525132489766));
#40554=CARTESIAN_POINT('Ctrl Pts',(-37.3587928824967,85.3112658187866,118.577781997497));
#40555=CARTESIAN_POINT('Ctrl Pts',(-36.4365381596906,85.115376166923,118.630431505227));
#40556=CARTESIAN_POINT('Ctrl Pts',(-35.6413142888051,85.3500138937257,118.683081012958));
#40557=CARTESIAN_POINT('Ctrl Pts',(-34.8460904179196,85.5846516205283,118.735730520689));
#40558=CARTESIAN_POINT('Ctrl Pts',(-34.1778973989547,86.2498167259973,118.78838002842));
#40559=CARTESIAN_POINT('Ctrl Pts',(-33.9396503765726,87.0439667278887,118.841029536151));
#40560=CARTESIAN_POINT('Ctrl Pts',(-33.7014033541905,87.83811672978,118.893679043881));
#40561=CARTESIAN_POINT('Ctrl Pts',(-33.8931023283913,88.7612516280936,118.946328551612));
#40562=CARTESIAN_POINT('Ctrl Pts',(-34.4278434831162,89.3948822478746,118.998978059343));
#40563=CARTESIAN_POINT('Ctrl Pts',(-34.9625846378412,90.0285128676557,119.051627567074));
#40564=CARTESIAN_POINT('Ctrl Pts',(-35.8403679730904,90.3726392089041,119.104277074805));
#40565=CARTESIAN_POINT('Ctrl Pts',(-36.6632637646553,90.2712568417485,119.156926582536));
#40566=CARTESIAN_POINT('Ctrl Pts',(-37.4861595562202,90.1698744745929,119.209576090266));
#40567=CARTESIAN_POINT('Ctrl Pts',(-38.2541678041008,89.6229833990333,119.262225597997));
#40568=CARTESIAN_POINT('Ctrl Pts',(-38.6191236428543,88.8785083391832,119.314875105728));
#40569=CARTESIAN_POINT('Ctrl Pts',(-38.7867382361248,88.5365905751519,119.339055636321));
#40570=CARTESIAN_POINT('Ctrl Pts',(-38.8693360705098,88.152995973142,119.363236166915));
#40571=CARTESIAN_POINT('Ctrl Pts',(-38.8685902376792,87.769097033614,119.387416697508));
#40572=CARTESIAN_POINT('Origin',(-36.3549260746835,87.7685555885722,114.));
#40573=CARTESIAN_POINT('',(-38.8730930351581,87.7663573574127,120.387416697508));
#40574=CARTESIAN_POINT('',(-38.8765117847785,87.7688288397063,120.112583302492));
#40575=CARTESIAN_POINT('',(-38.8724260746835,87.7685555885722,114.));
#40576=CARTESIAN_POINT('Ctrl Pts',(-38.8765117847785,87.7688288397063,120.112583302492));
#40577=CARTESIAN_POINT('Ctrl Pts',(-38.8765350839041,87.783820778578,120.11163134332));
#40578=CARTESIAN_POINT('Ctrl Pts',(-38.8764128203056,87.7988123273143,120.110679384147));
#40579=CARTESIAN_POINT('Ctrl Pts',(-38.8761438311705,87.8138012428756,120.109727424975));
#40580=CARTESIAN_POINT('Ctrl Pts',(-38.8612669898543,88.6427853512518,120.057077917244));
#40581=CARTESIAN_POINT('Ctrl Pts',(-38.3975851441409,89.463715087247,120.004428409513));
#40582=CARTESIAN_POINT('Ctrl Pts',(-37.6953015855779,89.9044346174046,119.951778901782));
#40583=CARTESIAN_POINT('Ctrl Pts',(-36.9930180270149,90.3451541475622,119.899129394052));
#40584=CARTESIAN_POINT('Ctrl Pts',(-36.0521327556023,90.4056634718823,119.846479886321));
#40585=CARTESIAN_POINT('Ctrl Pts',(-35.2991817147569,90.058531521478,119.79383037859));
#40586=CARTESIAN_POINT('Ctrl Pts',(-34.5462306739115,89.7113995710737,119.741180870859));
#40587=CARTESIAN_POINT('Ctrl Pts',(-33.9812138636332,88.956626345945,119.688531363128));
#40588=CARTESIAN_POINT('Ctrl Pts',(-33.8602731048237,88.136376852245,119.635881855397));
#40589=CARTESIAN_POINT('Ctrl Pts',(-33.7393323460141,87.316127358545,119.583232347667));
#40590=CARTESIAN_POINT('Ctrl Pts',(-34.0624676386734,86.4304015962738,119.530582839936));
#40591=CARTESIAN_POINT('Ctrl Pts',(-34.6831904912772,85.8807298501539,119.477933332205));
#40592=CARTESIAN_POINT('Ctrl Pts',(-35.3039133438809,85.3310581040341,119.425283824474));
#40593=CARTESIAN_POINT('Ctrl Pts',(-36.2222237564292,85.1174403740656,119.372634316743));
#40594=CARTESIAN_POINT('Ctrl Pts',(-37.0218196779139,85.3367170196712,119.319984809013));
#40595=CARTESIAN_POINT('Ctrl Pts',(-37.8214155993986,85.5559936652768,119.267335301282));
#40596=CARTESIAN_POINT('Ctrl Pts',(-38.5022970298196,86.2081646864565,119.214685793551));
#40597=CARTESIAN_POINT('Ctrl Pts',(-38.7557967218956,86.9975782633452,119.16203628582));
#40598=CARTESIAN_POINT('Ctrl Pts',(-38.8351663531686,87.2447401593083,119.145551958044));
#40599=CARTESIAN_POINT('Ctrl Pts',(-38.8726402493978,87.505355783484,119.129067630268));
#40600=CARTESIAN_POINT('Ctrl Pts',(-38.8706377933747,87.7665317068533,119.112583302492));
#40601=CARTESIAN_POINT('Ctrl Pts',(-38.8685902376792,87.769097033614,119.387416697508));
#40602=CARTESIAN_POINT('Ctrl Pts',(-38.867712130488,87.317113149706,119.415885674646));
#40603=CARTESIAN_POINT('Ctrl Pts',(-38.7513067081162,86.8647074065548,119.444354651783));
#40604=CARTESIAN_POINT('Ctrl Pts',(-38.5221044433275,86.4793994073616,119.472823628921));
#40605=CARTESIAN_POINT('Ctrl Pts',(-38.0982259754207,85.7668245795307,119.525473136651));
#40606=CARTESIAN_POINT('Ctrl Pts',(-37.2885656099805,85.2837339680096,119.578122644382));
#40607=CARTESIAN_POINT('Ctrl Pts',(-36.4601705392343,85.2491292346396,119.630772152113));
#40608=CARTESIAN_POINT('Ctrl Pts',(-35.6317754684881,85.2145245012696,119.683421659844));
#40609=CARTESIAN_POINT('Ctrl Pts',(-34.7846456924359,85.6284056460505,119.736071167575));
#40610=CARTESIAN_POINT('Ctrl Pts',(-34.3028146583386,86.3031461938721,119.788720675305));
#40611=CARTESIAN_POINT('Ctrl Pts',(-33.8209836242412,86.9778867416937,119.841370183036));
#40612=CARTESIAN_POINT('Ctrl Pts',(-33.7044513320988,87.913486692556,119.894019690767));
#40613=CARTESIAN_POINT('Ctrl Pts',(-34.0060458310393,88.685805526085,119.946669198498));
#40614=CARTESIAN_POINT('Ctrl Pts',(-34.3076403299799,89.458124359614,119.999318706229));
#40615=CARTESIAN_POINT('Ctrl Pts',(-35.0273616200035,90.0671620758098,120.05196821396));
#40616=CARTESIAN_POINT('Ctrl Pts',(-35.8389351910839,90.2368217366715,120.10461772169));
#40617=CARTESIAN_POINT('Ctrl Pts',(-36.6505087621644,90.4064813975333,120.157267229421));
#40618=CARTESIAN_POINT('Ctrl Pts',(-37.5539346143018,90.136763003061,120.209916737152));
#40619=CARTESIAN_POINT('Ctrl Pts',(-38.1396579805213,89.5499371283205,120.262566244883));
#40620=CARTESIAN_POINT('Ctrl Pts',(-38.6026431728332,89.0860804578518,120.304183062425));
#40621=CARTESIAN_POINT('Ctrl Pts',(-38.8671241578398,88.4240913465261,120.345799879966));
#40622=CARTESIAN_POINT('Ctrl Pts',(-38.8730930351581,87.7663573574127,120.387416697508));
#40623=CARTESIAN_POINT('Origin',(-36.3549260746835,87.7685555885722,114.));
#40624=CARTESIAN_POINT('',(-38.8751286390733,87.7701344517389,121.387416697508));
#40625=CARTESIAN_POINT('',(-38.8699207989934,87.7703173750275,121.112583302492));
#40626=CARTESIAN_POINT('',(-38.8724260746835,87.7685555885722,114.));
#40627=CARTESIAN_POINT('',(-34.4414600780185,89.4045427919472,122.));
#40628=CARTESIAN_POINT('Ctrl Pts',(-38.8751286390733,87.7701344517389,121.387416697508));
#40629=CARTESIAN_POINT('Ctrl Pts',(-38.8696705638905,87.0409116216481,121.43366260848));
#40630=CARTESIAN_POINT('Ctrl Pts',(-38.5351407981639,86.3074376342814,121.479908519451));
#40631=CARTESIAN_POINT('Ctrl Pts',(-37.9776638007606,85.8386043277258,121.526154430423));
#40632=CARTESIAN_POINT('Ctrl Pts',(-37.3429938619931,85.3048524288138,121.578803938153));
#40633=CARTESIAN_POINT('Ctrl Pts',(-36.4193597263055,85.1141040344884,121.631453445884));
#40634=CARTESIAN_POINT('Ctrl Pts',(-35.6257426583825,85.3542580189696,121.684102953615));
#40635=CARTESIAN_POINT('Ctrl Pts',(-34.8321255904596,85.5944120034508,121.736752461346));
#40636=CARTESIAN_POINT('Ctrl Pts',(-34.1685255903014,86.2654683667386,121.789401969077));
#40637=CARTESIAN_POINT('Ctrl Pts',(-33.9355603656107,87.0597542623074,121.842051476807));
#40638=CARTESIAN_POINT('Ctrl Pts',(-33.70259514092,87.8540401578761,121.894700984538));
#40639=CARTESIAN_POINT('Ctrl Pts',(-33.9002646916968,88.7715555857257,121.947350492269));
#40640=CARTESIAN_POINT('Ctrl Pts',(-34.4414600780185,89.4045427919472,122.));
#40641=CARTESIAN_POINT('',(-38.2720362925639,89.4070835106059,122.));
#40642=CARTESIAN_POINT('Origin',(-36.3549260746835,87.7685555885722,122.));
#40643=CARTESIAN_POINT('Ctrl Pts',(-38.2720451383381,89.4070896778011,122.));
#40644=CARTESIAN_POINT('Ctrl Pts',(-37.7492245696404,90.0158048033409,121.949053726697));
#40645=CARTESIAN_POINT('Ctrl Pts',(-36.9095000892721,90.3559810494937,121.898107453395));
#40646=CARTESIAN_POINT('Ctrl Pts',(-36.1108292529146,90.2782182443628,121.847161180092));
#40647=CARTESIAN_POINT('Ctrl Pts',(-35.2854572748038,90.1978556752386,121.794511672361));
#40648=CARTESIAN_POINT('Ctrl Pts',(-34.5039298348585,89.6711418716167,121.74186216463));
#40649=CARTESIAN_POINT('Ctrl Pts',(-34.1200452267186,88.9363551361257,121.6892126569));
#40650=CARTESIAN_POINT('Ctrl Pts',(-33.7361606185786,88.2015684006347,121.636563149169));
#40651=CARTESIAN_POINT('Ctrl Pts',(-33.749918842244,87.2587087332746,121.583913641438));
#40652=CARTESIAN_POINT('Ctrl Pts',(-34.1553236157352,86.5354489663317,121.531264133707));
#40653=CARTESIAN_POINT('Ctrl Pts',(-34.5607283892265,85.8121891993888,121.478614625976));
#40654=CARTESIAN_POINT('Ctrl Pts',(-35.3577797125436,85.308529332863,121.425965118246));
#40655=CARTESIAN_POINT('Ctrl Pts',(-36.1850294138675,85.2526783544614,121.373315610515));
#40656=CARTESIAN_POINT('Ctrl Pts',(-37.0122791151915,85.1968273760598,121.320666102784));
#40657=CARTESIAN_POINT('Ctrl Pts',(-37.8697271945221,85.5887852857824,121.268016595053));
#40658=CARTESIAN_POINT('Ctrl Pts',(-38.3687195320203,86.2509210824945,121.215367087322));
#40659=CARTESIAN_POINT('Ctrl Pts',(-38.693434952036,86.6818008519411,121.181105825712));
#40660=CARTESIAN_POINT('Ctrl Pts',(-38.8663567186898,87.2270916455049,121.146844564102));
#40661=CARTESIAN_POINT('Ctrl Pts',(-38.8699207989934,87.7703173750275,121.112583302492));
#40662=CARTESIAN_POINT('Origin',(-36.3549260746835,87.7685555885722,124.208423447177));
#40663=CARTESIAN_POINT('',(-39.4331959724664,87.7693690614377,107.791576552823));
#40664=CARTESIAN_POINT('',(-39.4235550742983,87.7688699395357,107.708423447177));
#40665=CARTESIAN_POINT('',(-39.4284260746835,87.7685555885726,124.208423447177));
#40666=CARTESIAN_POINT('',(-35.5611267921506,84.7993326348266,107.));
#40667=CARTESIAN_POINT('Ctrl Pts',(-39.4235550742983,87.7688699395357,107.708423447177));
#40668=CARTESIAN_POINT('Ctrl Pts',(-39.4238749307152,88.2640454211739,107.682880329042));
#40669=CARTESIAN_POINT('Ctrl Pts',(-39.0776226443318,89.7793619650307,107.604687703175));
#40670=CARTESIAN_POINT('Ctrl Pts',(-36.7064604371766,91.3774168831885,107.473845569577));
#40671=CARTESIAN_POINT('Ctrl Pts',(-33.5229010658053,90.036960964095,107.315897046385));
#40672=CARTESIAN_POINT('Ctrl Pts',(-32.9121326734567,86.6347724882534,107.157948523192));
#40673=CARTESIAN_POINT('Ctrl Pts',(-34.578888202379,85.0619266872042,107.052649507731));
#40674=CARTESIAN_POINT('Ctrl Pts',(-35.5611267921506,84.7993326348266,107.));
#40675=CARTESIAN_POINT('',(-37.1487253572163,84.7993326348265,107.));
#40676=CARTESIAN_POINT('Origin',(-36.3549260746835,87.7685555885722,107.));
#40677=CARTESIAN_POINT('Ctrl Pts',(-39.4331959724664,87.7693690614377,107.791576552823));
#40678=CARTESIAN_POINT('Ctrl Pts',(-39.4333520414626,87.8138779030189,107.789262006108));
#40679=CARTESIAN_POINT('Ctrl Pts',(-39.4123923264904,88.8706874181061,107.734297951662));
#40680=CARTESIAN_POINT('Ctrl Pts',(-38.2031234082454,90.8887186315066,107.626684389485));
#40681=CARTESIAN_POINT('Ctrl Pts',(-34.7524574012803,91.0220940358159,107.468735866293));
#40682=CARTESIAN_POINT('Ctrl Pts',(-32.7548483299835,88.204780757559,107.3107873431));
#40683=CARTESIAN_POINT('Ctrl Pts',(-34.0073633012862,85.0282370938957,107.154542054336));
#40684=CARTESIAN_POINT('Ctrl Pts',(-36.2036730954584,84.5433632626068,107.050946273303));
#40685=CARTESIAN_POINT('Ctrl Pts',(-37.1506394582515,84.7942439414616,107.));
#40686=CARTESIAN_POINT('Origin',(-36.3549260746835,87.7685555885722,124.208423447177));
#40687=CARTESIAN_POINT('',(-39.4248377279915,87.7704209830772,108.791576552823));
#40688=CARTESIAN_POINT('',(-39.4300189070168,87.765997310884,108.708423447177));
#40689=CARTESIAN_POINT('',(-39.4284260746835,87.7685555885726,124.208423447177));
#40690=CARTESIAN_POINT('Ctrl Pts',(-39.4300189070168,87.765997310884,108.708423447177));
#40691=CARTESIAN_POINT('Ctrl Pts',(-39.4226310503045,88.5947453159106,108.665444042093));
#40692=CARTESIAN_POINT('Ctrl Pts',(-38.6509820307071,90.4508356800763,108.569815129278));
#40693=CARTESIAN_POINT('Ctrl Pts',(-35.521928276906,91.298128615592,108.421536708732));
#40694=CARTESIAN_POINT('Ctrl Pts',(-32.944032143022,89.0005543557004,108.26358818554));
#40695=CARTESIAN_POINT('Ctrl Pts',(-33.4587561442345,85.5858976617427,108.105639662347));
#40696=CARTESIAN_POINT('Ctrl Pts',(-36.5992128995613,84.1503275352445,107.947691139155));
#40697=CARTESIAN_POINT('Ctrl Pts',(-39.0463675728263,85.696694156362,107.815285734098));
#40698=CARTESIAN_POINT('Ctrl Pts',(-39.4232156422602,87.2433890858758,107.735529836772));
#40699=CARTESIAN_POINT('Ctrl Pts',(-39.4235550742983,87.7688699395357,107.708423447177));
#40700=CARTESIAN_POINT('Ctrl Pts',(-39.4248377279915,87.7704209830772,108.791576552823));
#40701=CARTESIAN_POINT('Ctrl Pts',(-39.4269818594004,88.1529039528601,108.771825719159));
#40702=CARTESIAN_POINT('Ctrl Pts',(-39.1839874391446,89.552339992846,108.699425377765));
#40703=CARTESIAN_POINT('Ctrl Pts',(-37.0970138577844,91.3183647606488,108.57437552864));
#40704=CARTESIAN_POINT('Ctrl Pts',(-33.7881605542584,90.3305043851839,108.416427005448));
#40705=CARTESIAN_POINT('Ctrl Pts',(-32.8065174312516,87.0197923230117,108.258478482255));
#40706=CARTESIAN_POINT('Ctrl Pts',(-35.0421044995447,84.3879830042027,108.100529959063));
#40707=CARTESIAN_POINT('Ctrl Pts',(-38.4177928691641,84.8148429236005,107.944895982585));
#40708=CARTESIAN_POINT('Ctrl Pts',(-39.4298019053741,86.8014254068839,107.841911513839));
#40709=CARTESIAN_POINT('Ctrl Pts',(-39.4331959724664,87.7693690614377,107.791576552823));
#40710=CARTESIAN_POINT('Origin',(-36.3549260746835,87.7685555885722,124.208423447177));
#40711=CARTESIAN_POINT('',(-39.4267609799808,87.7659629280684,109.791576552823));
#40712=CARTESIAN_POINT('',(-39.4310568549431,87.7708236397202,109.708423447177));
#40713=CARTESIAN_POINT('',(-39.4284260746835,87.7685555885726,124.208423447177));
#40714=CARTESIAN_POINT('Ctrl Pts',(-39.431056854943,87.7708236397202,109.708423447178));
#40715=CARTESIAN_POINT('Ctrl Pts',(-39.4322959763111,87.9204433841515,109.700657262876));
#40716=CARTESIAN_POINT('Ctrl Pts',(-39.3546330833386,89.083093328256,109.640241570843));
#40717=CARTESIAN_POINT('Ctrl Pts',(-37.8732760615816,91.0619523578304,109.527176371079));
#40718=CARTESIAN_POINT('Ctrl Pts',(-34.4272254088536,90.8403332051346,109.369227847887));
#40719=CARTESIAN_POINT('Ctrl Pts',(-32.7289618949911,87.8336271396496,109.211279324695));
#40720=CARTESIAN_POINT('Ctrl Pts',(-34.3182507011933,84.7679217971554,109.053330801502));
#40721=CARTESIAN_POINT('Ctrl Pts',(-37.7541293221915,84.4228016643723,108.89538227831));
#40722=CARTESIAN_POINT('Ctrl Pts',(-39.3316610725117,86.3796383650939,108.780413160201));
#40723=CARTESIAN_POINT('Ctrl Pts',(-39.4316811294837,87.579534090627,108.718093549824));
#40724=CARTESIAN_POINT('Ctrl Pts',(-39.4300189070168,87.765997310884,108.708423447177));
#40725=CARTESIAN_POINT('Ctrl Pts',(-39.4267609799808,87.7659629280684,109.791576552823));
#40726=CARTESIAN_POINT('Ctrl Pts',(-39.4209015342644,88.4849691123104,109.754389432211));
#40727=CARTESIAN_POINT('Ctrl Pts',(-38.8116905796402,90.2308909611916,109.664552803868));
#40728=CARTESIAN_POINT('Ctrl Pts',(-35.9114810808611,91.3678896299961,109.522066667795));
#40729=CARTESIAN_POINT('Ctrl Pts',(-33.0986031650656,89.3648670933915,109.364118144603));
#40730=CARTESIAN_POINT('Ctrl Pts',(-33.2381342205824,85.9145173244662,109.20616962141));
#40731=CARTESIAN_POINT('Ctrl Pts',(-36.2035656043253,84.1451679505691,109.048221098218));
#40732=CARTESIAN_POINT('Ctrl Pts',(-38.918255079236,85.471480422957,108.910023408688));
#40733=CARTESIAN_POINT('Ctrl Pts',(-39.4212662797386,87.1333247078628,108.82447522689));
#40734=CARTESIAN_POINT('Ctrl Pts',(-39.4248377279915,87.7704209830772,108.791576552823));
#40735=CARTESIAN_POINT('Origin',(-36.3549260746835,87.7685555885722,124.208423447177));
#40736=CARTESIAN_POINT('',(-39.4332677588359,87.7692403954757,110.791576552823));
#40737=CARTESIAN_POINT('',(-39.4236451829169,87.7689040049272,110.708423447177));
#40738=CARTESIAN_POINT('',(-39.4284260746835,87.7685555885726,124.208423447177));
#40739=CARTESIAN_POINT('Ctrl Pts',(-39.4236451829169,87.7689040049272,110.708423447177));
#40740=CARTESIAN_POINT('Ctrl Pts',(-39.4241444783375,88.2574355105714,110.683220975927));
#40741=CARTESIAN_POINT('Ctrl Pts',(-39.0844834239227,89.7658834613085,110.605368996946));
#40742=CARTESIAN_POINT('Ctrl Pts',(-36.7289586508838,91.3757634277843,110.474867510234));
#40743=CARTESIAN_POINT('Ctrl Pts',(-33.5388966026528,90.0536872598855,110.316918987042));
#40744=CARTESIAN_POINT('Ctrl Pts',(-32.9020428254094,86.6597517104068,110.158970463849));
#40745=CARTESIAN_POINT('Ctrl Pts',(-35.3958132871802,84.2711349028723,110.001021940657));
#40746=CARTESIAN_POINT('Ctrl Pts',(-38.5938083527313,85.0150537749961,109.850839601766));
#40747=CARTESIAN_POINT('Ctrl Pts',(-39.4238955665977,86.9061221183966,109.753306770606));
#40748=CARTESIAN_POINT('Ctrl Pts',(-39.431056854943,87.7708236397202,109.708423447178));
#40749=CARTESIAN_POINT('Ctrl Pts',(-39.4332677588359,87.7692403954757,110.791576552823));
#40750=CARTESIAN_POINT('Ctrl Pts',(-39.4333834028134,87.8071966848497,110.789602652993));
#40751=CARTESIAN_POINT('Ctrl Pts',(-39.4156194617581,88.8574441518405,110.734979245433));
#40752=CARTESIAN_POINT('Ctrl Pts',(-38.223100855083,90.8768947163338,110.627706330142));
#40753=CARTESIAN_POINT('Ctrl Pts',(-34.7734205070594,91.0320949679017,110.46975780695));
#40754=CARTESIAN_POINT('Ctrl Pts',(-32.7576431577175,88.2283433211983,110.311809283757));
#40755=CARTESIAN_POINT('Ctrl Pts',(-34.0034128231148,85.0077161192772,110.153860760565));
#40756=CARTESIAN_POINT('Ctrl Pts',(-37.3812280349669,84.2902581008489,109.995912237372));
#40757=CARTESIAN_POINT('Ctrl Pts',(-39.2523388634201,86.1528899994607,109.875150834792));
#40758=CARTESIAN_POINT('Ctrl Pts',(-39.4291973347315,87.4670004975569,109.807038939942));
#40759=CARTESIAN_POINT('Ctrl Pts',(-39.4267609799808,87.7659629280684,109.791576552823));
#40760=CARTESIAN_POINT('Origin',(-36.3549260746835,87.7685555885722,124.208423447177));
#40761=CARTESIAN_POINT('',(-39.4249633754519,87.7704976440673,111.791576552823));
#40762=CARTESIAN_POINT('',(-39.4298259838121,87.7659597950156,111.708423447177));
#40763=CARTESIAN_POINT('',(-39.4284260746835,87.7685555885726,124.208423447177));
#40764=CARTESIAN_POINT('Ctrl Pts',(-39.4298259838121,87.7659597950156,111.708423447177));
#40765=CARTESIAN_POINT('Ctrl Pts',(-39.422445104778,88.5882717598716,111.665784688979));
#40766=CARTESIAN_POINT('Ctrl Pts',(-38.6609851967907,90.4380265410958,111.570496423049));
#40767=CARTESIAN_POINT('Ctrl Pts',(-35.544600016728,91.3034134977843,111.422558649389));
#40768=CARTESIAN_POINT('Ctrl Pts',(-32.9520312482784,89.0224118636959,111.264610126197));
#40769=CARTESIAN_POINT('Ctrl Pts',(-33.4447637244879,85.6045768793427,111.106661603004));
#40770=CARTESIAN_POINT('Ctrl Pts',(-36.5760518951862,84.1487555760565,110.948713079812));
#40771=CARTESIAN_POINT('Ctrl Pts',(-39.0392097413283,85.6835153821574,110.81596702787));
#40772=CARTESIAN_POINT('Ctrl Pts',(-39.4231014195896,87.2368632409793,110.735870483658));
#40773=CARTESIAN_POINT('Ctrl Pts',(-39.4236451829169,87.7689040049272,110.708423447177));
#40774=CARTESIAN_POINT('Ctrl Pts',(-39.4249633754519,87.7704976440673,111.791576552823));
#40775=CARTESIAN_POINT('Ctrl Pts',(-39.4271630525139,88.1463451570976,111.772166366045));
#40776=CARTESIAN_POINT('Ctrl Pts',(-39.1897287451099,89.5389847880784,111.700106671536));
#40777=CARTESIAN_POINT('Ctrl Pts',(-37.11979162744,91.3135280607988,111.575397469297));
#40778=CARTESIAN_POINT('Ctrl Pts',(-33.8046642536859,90.3469298412686,111.417448946105));
#40779=CARTESIAN_POINT('Ctrl Pts',(-32.8017817103211,87.0425981045389,111.259500422912));
#40780=CARTESIAN_POINT('Ctrl Pts',(-35.0204270981272,84.3964699395587,111.10155189972));
#40781=CARTESIAN_POINT('Ctrl Pts',(-38.4061745970663,84.8025699726496,110.945577276356));
#40782=CARTESIAN_POINT('Ctrl Pts',(-39.4302988498904,86.7947947781262,110.842252160724));
#40783=CARTESIAN_POINT('Ctrl Pts',(-39.4332677588359,87.7692403954757,110.791576552823));
#40784=CARTESIAN_POINT('Origin',(-36.3549260746835,87.7685555885722,124.208423447177));
#40785=CARTESIAN_POINT('',(-39.4265848876636,87.7659995883269,112.791576552823));
#40786=CARTESIAN_POINT('',(-39.4312326367126,87.7707578835516,112.708423447177));
#40787=CARTESIAN_POINT('',(-39.4284260746835,87.7685555885726,124.208423447177));
#40788=CARTESIAN_POINT('Ctrl Pts',(-39.4312326367126,87.7707578835516,112.708423447177));
#40789=CARTESIAN_POINT('Ctrl Pts',(-39.4323935001362,87.9137935611134,112.700997909761));
#40790=CARTESIAN_POINT('Ctrl Pts',(-39.358587174522,89.0697956308562,112.640922864614));
#40791=CARTESIAN_POINT('Ctrl Pts',(-37.8943917131075,91.0521350845713,112.528198311736));
#40792=CARTESIAN_POINT('Ctrl Pts',(-34.4469889106826,90.8526477623989,112.370249788544));
#40793=CARTESIAN_POINT('Ctrl Pts',(-32.7294547075721,87.8569078646409,112.212301265352));
#40794=CARTESIAN_POINT('Ctrl Pts',(-34.2990251292932,84.7810616452854,112.054352742159));
#40795=CARTESIAN_POINT('Ctrl Pts',(-37.732618410801,84.413885323785,111.896404218967));
#40796=CARTESIAN_POINT('Ctrl Pts',(-39.3273914927566,86.3663225186427,111.781094453973));
#40797=CARTESIAN_POINT('Ctrl Pts',(-39.4315588703796,87.5728969698939,111.71843419671));
#40798=CARTESIAN_POINT('Ctrl Pts',(-39.4298259838121,87.7659597950156,111.708423447177));
#40799=CARTESIAN_POINT('Ctrl Pts',(-39.4265848876636,87.7659995883269,112.791576552823));
#40800=CARTESIAN_POINT('Ctrl Pts',(-39.4208858349911,88.4785229697945,112.754730079097));
#40801=CARTESIAN_POINT('Ctrl Pts',(-38.8205345450662,90.2178280429807,112.66523409764));
#40802=CARTESIAN_POINT('Ctrl Pts',(-35.93460153719,91.3706628087708,112.523088608452));
#40803=CARTESIAN_POINT('Ctrl Pts',(-33.1089202140314,89.3857429912062,112.365140085259));
#40804=CARTESIAN_POINT('Ctrl Pts',(-33.2262936819204,85.934568540205,112.207191562067));
#40805=CARTESIAN_POINT('Ctrl Pts',(-36.1803029872748,84.1462143677634,112.049243038875));
#40806=CARTESIAN_POINT('Ctrl Pts',(-38.9101650309924,85.4582951470999,111.91070470246));
#40807=CARTESIAN_POINT('Ctrl Pts',(-39.4211964991877,87.1268708589074,111.824815873776));
#40808=CARTESIAN_POINT('Ctrl Pts',(-39.4249633754519,87.7704976440673,111.791576552823));
#40809=CARTESIAN_POINT('Origin',(-36.3549260746835,87.7685555885722,124.208423447177));
#40810=CARTESIAN_POINT('',(-39.4333269951809,87.7691245003032,113.791576552823));
#40811=CARTESIAN_POINT('',(-39.4236710600204,87.7690089236073,113.708423447177));
#40812=CARTESIAN_POINT('',(-39.4284260746835,87.7685555885726,124.208423447177));
#40813=CARTESIAN_POINT('Ctrl Pts',(-39.4236710600204,87.7690089236073,113.708423447178));
#40814=CARTESIAN_POINT('Ctrl Pts',(-39.4243122366841,88.2509270813075,113.683561622813));
#40815=CARTESIAN_POINT('Ctrl Pts',(-39.0911304972661,89.7525574526633,113.606050290717));
#40816=CARTESIAN_POINT('Ctrl Pts',(-36.7521128167719,91.3732874025,113.475889450891));
#40817=CARTESIAN_POINT('Ctrl Pts',(-33.5536274798598,90.071721874595,113.317940927699));
#40818=CARTESIAN_POINT('Ctrl Pts',(-32.8949943812288,86.6819455227893,113.159992404506));
#40819=CARTESIAN_POINT('Ctrl Pts',(-35.3733761199876,84.2773654698779,113.002043881314));
#40820=CARTESIAN_POINT('Ctrl Pts',(-38.583346428161,85.0023754277235,112.851520895538));
#40821=CARTESIAN_POINT('Ctrl Pts',(-39.4241625958431,86.8996234627776,112.753647417492));
#40822=CARTESIAN_POINT('Ctrl Pts',(-39.4312326367126,87.7707578835516,112.708423447177));
#40823=CARTESIAN_POINT('Ctrl Pts',(-39.4333269951809,87.7691245003032,113.791576552823));
#40824=CARTESIAN_POINT('Ctrl Pts',(-39.4334076784544,87.8005288405486,113.789943299879));
#40825=CARTESIAN_POINT('Ctrl Pts',(-39.4188025102445,88.8442059785835,113.735660539205));
#40826=CARTESIAN_POINT('Ctrl Pts',(-38.2430209835701,90.864835091082,113.628728270799));
#40827=CARTESIAN_POINT('Ctrl Pts',(-34.7944082905965,91.0421825355799,113.470779747607));
#40828=CARTESIAN_POINT('Ctrl Pts',(-32.7606696114516,88.2514319900887,113.312831224414));
#40829=CARTESIAN_POINT('Ctrl Pts',(-33.9857339531502,85.0228720973646,113.154882701222));
#40830=CARTESIAN_POINT('Ctrl Pts',(-37.3588727357218,84.2837399199298,112.996934178029));
#40831=CARTESIAN_POINT('Ctrl Pts',(-39.2472166530314,86.1395391875126,112.875832128563));
#40832=CARTESIAN_POINT('Ctrl Pts',(-39.4290291466135,87.460406404289,112.807379586827));
#40833=CARTESIAN_POINT('Ctrl Pts',(-39.4265848876636,87.7659995883269,112.791576552823));
#40834=CARTESIAN_POINT('Origin',(-36.3549260746835,87.7685555885722,124.208423447177));
#40835=CARTESIAN_POINT('',(-39.4250942775894,87.770571594449,114.791576552823));
#40836=CARTESIAN_POINT('',(-39.4296318005188,87.7659266486971,114.708423447177));
#40837=CARTESIAN_POINT('',(-39.4284260746835,87.7685555885726,124.208423447177));
#40838=CARTESIAN_POINT('Ctrl Pts',(-39.4296318005188,87.7659266486971,114.708423447177));
#40839=CARTESIAN_POINT('Ctrl Pts',(-39.4222699698754,88.5818020086375,114.666125335864));
#40840=CARTESIAN_POINT('Ctrl Pts',(-38.6709153677693,90.4252030152838,114.571177716821));
#40841=CARTESIAN_POINT('Ctrl Pts',(-35.5673140384357,91.3085437296246,114.423580590046));
#40842=CARTESIAN_POINT('Ctrl Pts',(-32.9601524074645,89.0442359979183,114.265632066854));
#40843=CARTESIAN_POINT('Ctrl Pts',(-33.4309288131869,85.623307637124,114.107683543661));
#40844=CARTESIAN_POINT('Ctrl Pts',(-36.5528046065515,84.1474103491404,113.949735020469));
#40845=CARTESIAN_POINT('Ctrl Pts',(-39.0321123676862,85.6702203471794,113.816648321641));
#40846=CARTESIAN_POINT('Ctrl Pts',(-39.4229544266047,87.2303763205356,113.736211130544));
#40847=CARTESIAN_POINT('Ctrl Pts',(-39.4236710600204,87.7690089236073,113.708423447178));
#40848=CARTESIAN_POINT('Ctrl Pts',(-39.4250942775894,87.770571594449,114.791576552823));
#40849=CARTESIAN_POINT('Ctrl Pts',(-39.4273437802822,88.1397834288107,114.772507012931));
#40850=CARTESIAN_POINT('Ctrl Pts',(-39.1954153750974,89.5256294501937,114.700787965308));
#40851=CARTESIAN_POINT('Ctrl Pts',(-37.1425381224351,91.3085437813298,114.576419409954));
#40852=CARTESIAN_POINT('Ctrl Pts',(-33.8212725638248,90.3632519156092,114.418470886762));
#40853=CARTESIAN_POINT('Ctrl Pts',(-32.7971935859219,87.0654278042858,114.260522363569));
#40854=CARTESIAN_POINT('Ctrl Pts',(-34.9988024520367,84.4051082703102,114.102573840377));
#40855=CARTESIAN_POINT('Ctrl Pts',(-38.3944877003389,84.7902994725376,113.946258570128));
#40856=CARTESIAN_POINT('Ctrl Pts',(-39.4308067741364,86.7881791852352,113.84259280761));
#40857=CARTESIAN_POINT('Ctrl Pts',(-39.4333269951809,87.7691245003032,113.791576552823));
#40858=CARTESIAN_POINT('Origin',(-36.3549260746835,87.7685555885722,124.208423447177));
#40859=CARTESIAN_POINT('',(-39.4264121022944,87.7660402134969,115.791576552823));
#40860=CARTESIAN_POINT('',(-39.4314045388933,87.7706880981477,115.708423447177));
#40861=CARTESIAN_POINT('',(-39.4284260746835,87.7685555885726,124.208423447177));
#40862=CARTESIAN_POINT('Ctrl Pts',(-39.4314045388933,87.7706880981477,115.708423447177));
#40863=CARTESIAN_POINT('Ctrl Pts',(-39.4324870743472,87.9071420895487,115.701338556647));
#40864=CARTESIAN_POINT('Ctrl Pts',(-39.362494359602,89.0565011022609,115.641604158386));
#40865=CARTESIAN_POINT('Ctrl Pts',(-37.9154438359774,91.0421824877652,115.529220252393));
#40866=CARTESIAN_POINT('Ctrl Pts',(-34.4668311933744,90.8648350458576,115.371271729201));
#40867=CARTESIAN_POINT('Ctrl Pts',(-32.7300967558443,87.8801851891123,115.213323206008));
#40868=CARTESIAN_POINT('Ctrl Pts',(-34.2798848175055,84.7943241686182,115.055374682816));
#40869=CARTESIAN_POINT('Ctrl Pts',(-37.7110496775229,84.4051083194366,114.897426159624));
#40870=CARTESIAN_POINT('Ctrl Pts',(-39.3230746797097,86.3530027291024,114.781775747744));
#40871=CARTESIAN_POINT('Ctrl Pts',(-39.4314334229786,87.5662617223888,114.718774843595));
#40872=CARTESIAN_POINT('Ctrl Pts',(-39.4296318005188,87.7659266486971,114.708423447177));
#40873=CARTESIAN_POINT('Ctrl Pts',(-39.4264121022944,87.7660402134969,115.791576552823));
#40874=CARTESIAN_POINT('Ctrl Pts',(-39.4208785096745,88.4720768830956,115.755070725982));
#40875=CARTESIAN_POINT('Ctrl Pts',(-38.8293123321225,90.2047529643201,115.665915391411));
#40876=CARTESIAN_POINT('Ctrl Pts',(-35.9577393267937,91.3732874551507,115.524110549109));
#40877=CARTESIAN_POINT('Ctrl Pts',(-33.1193710875871,89.4065522516036,115.366162025916));
#40878=CARTESIAN_POINT('Ctrl Pts',(-33.2145821502242,85.9546952911023,115.208213502724));
#40879=CARTESIAN_POINT('Ctrl Pts',(-36.1570475399255,84.14741029625,115.050264979531));
#40880=CARTESIAN_POINT('Ctrl Pts',(-38.9020111125005,85.4451186487052,114.911385996231));
#40881=CARTESIAN_POINT('Ctrl Pts',(-39.4211330793379,87.1204184395347,114.825156520661));
#40882=CARTESIAN_POINT('Ctrl Pts',(-39.4250942775894,87.770571594449,114.791576552823));
#40883=CARTESIAN_POINT('Origin',(-36.3549260746835,87.7685555885722,124.208423447177));
#40884=CARTESIAN_POINT('',(-39.4333759004399,87.7690073305927,116.791576552823));
#40885=CARTESIAN_POINT('',(-39.4237037046317,87.7691131821519,116.708423447178));
#40886=CARTESIAN_POINT('',(-39.4284260746835,87.7685555885726,124.208423447177));
#40887=CARTESIAN_POINT('Ctrl Pts',(-39.4237037046317,87.7691131821519,116.708423447178));
#40888=CARTESIAN_POINT('Ctrl Pts',(-39.4244820091948,88.2444156491833,116.683902269699));
#40889=CARTESIAN_POINT('Ctrl Pts',(-39.0977192292877,89.739228256387,116.606731584489));
#40890=CARTESIAN_POINT('Ctrl Pts',(-36.7752506060375,91.3706627561583,116.476911391548));
#40891=CARTESIAN_POINT('Ctrl Pts',(-33.5684738551649,90.0896615290181,116.318962868356));
#40892=CARTESIAN_POINT('Ctrl Pts',(-32.8880885856163,86.7041841389216,116.161014345163));
#40893=CARTESIAN_POINT('Ctrl Pts',(-35.3509794283091,84.2837399708291,116.003065821971));
#40894=CARTESIAN_POINT('Ctrl Pts',(-38.572813684769,84.9897178516136,115.852202189309));
#40895=CARTESIAN_POINT('Ctrl Pts',(-39.4244424957464,86.8931200035074,115.753988064378));
#40896=CARTESIAN_POINT('Ctrl Pts',(-39.4314045388933,87.7706880981477,115.708423447177));
#40897=CARTESIAN_POINT('Ctrl Pts',(-39.4333759004399,87.7690073305927,116.791576552823));
#40898=CARTESIAN_POINT('Ctrl Pts',(-39.4334273876949,87.7938606197418,116.790283946765));
#40899=CARTESIAN_POINT('Ctrl Pts',(-39.4219418998855,88.8309715577217,116.736341832976));
#40900=CARTESIAN_POINT('Ctrl Pts',(-38.2628632665517,90.8526478074454,116.629750211456));
#40901=CARTESIAN_POINT('Ctrl Pts',(-34.8154604137739,91.0521351325312,116.471801688264));
#40902=CARTESIAN_POINT('Ctrl Pts',(-32.7638442550116,88.2745007506674,116.313853165071));
#40903=CARTESIAN_POINT('Ctrl Pts',(-33.9681527643291,85.0381412779581,116.155904641879));
#40904=CARTESIAN_POINT('Ctrl Pts',(-37.3364760437162,84.2773654188855,115.997956118686));
#40905=CARTESIAN_POINT('Ctrl Pts',(-39.2420422323528,86.1261873235342,115.876513422334));
#40906=CARTESIAN_POINT('Ctrl Pts',(-39.4288591788618,87.4538152434738,115.807720233713));
#40907=CARTESIAN_POINT('Ctrl Pts',(-39.4264121022944,87.7660402134969,115.791576552823));
#40908=CARTESIAN_POINT('Origin',(-36.3549260746835,87.7685555885722,124.208423447177));
#40909=CARTESIAN_POINT('',(-39.4252303152106,87.7706425236776,117.791576552823));
#40910=CARTESIAN_POINT('',(-39.4294365974543,87.7658979721433,117.708423447178));
#40911=CARTESIAN_POINT('',(-39.4284260746835,87.7685555885726,124.208423447177));
#40912=CARTESIAN_POINT('Ctrl Pts',(-39.4294365974543,87.7658979721433,117.708423447178));
#40913=CARTESIAN_POINT('Ctrl Pts',(-39.4221061797108,88.57533513631,117.66646598275));
#40914=CARTESIAN_POINT('Ctrl Pts',(-38.6807762323999,90.4123619435266,117.571859010592));
#40915=CARTESIAN_POINT('Ctrl Pts',(-35.5900605330986,91.3135280090206,117.424602530703));
#40916=CARTESIAN_POINT('Ctrl Pts',(-32.9684135319854,89.0660075362686,117.26665400751));
#40917=CARTESIAN_POINT('Ctrl Pts',(-33.417214457214,85.6421268427602,117.108705484318));
#40918=CARTESIAN_POINT('Ctrl Pts',(-36.5295491595418,84.1462144206715,116.950756961126));
#40919=CARTESIAN_POINT('Ctrl Pts',(-39.0249546695335,85.6569303306175,116.817329615412));
#40920=CARTESIAN_POINT('Ctrl Pts',(-39.4228109086881,87.223892024903,116.736551777429));
#40921=CARTESIAN_POINT('Ctrl Pts',(-39.4237037046317,87.7691131821519,116.708423447178));
#40922=CARTESIAN_POINT('Ctrl Pts',(-39.4252303152106,87.7706425236776,117.791576552823));
#40923=CARTESIAN_POINT('Ctrl Pts',(-39.4275239472324,88.1332185492538,117.772847659816));
#40924=CARTESIAN_POINT('Ctrl Pts',(-39.2010476056018,89.5122738774369,117.701469259079));
#40925=CARTESIAN_POINT('Ctrl Pts',(-37.1652521444745,91.3034135494146,117.577441350611));
#40926=CARTESIAN_POINT('Ctrl Pts',(-33.8379853355952,90.3794670115321,117.419492827418));
#40927=CARTESIAN_POINT('Ctrl Pts',(-32.7927521455727,87.0882864937512,117.261544304226));
#40928=CARTESIAN_POINT('Ctrl Pts',(-34.9772337184436,84.4138852747866,117.103595781033));
#40929=CARTESIAN_POINT('Ctrl Pts',(-38.3827274930347,84.7780567344006,116.946939863899));
#40930=CARTESIAN_POINT('Ctrl Pts',(-39.4313302455591,86.7815541779694,116.842933454495));
#40931=CARTESIAN_POINT('Ctrl Pts',(-39.4333759004399,87.7690073305927,116.791576552823));
#40932=CARTESIAN_POINT('Origin',(-36.3549260746835,87.7685555885722,124.208423447177));
#40933=CARTESIAN_POINT('',(-39.4262428442554,87.7660847244363,118.791576552823));
#40934=CARTESIAN_POINT('',(-39.431572198619,87.7706143825889,118.708423447177));
#40935=CARTESIAN_POINT('',(-39.4284260746835,87.7685555885726,124.208423447177));
#40936=CARTESIAN_POINT('Ctrl Pts',(-39.431572198619,87.7706143825889,118.708423447177));
#40937=CARTESIAN_POINT('Ctrl Pts',(-39.4325766336119,87.9004890468128,118.701679203533));
#40938=CARTESIAN_POINT('Ctrl Pts',(-39.3663548371633,89.0432097994101,118.642285452157));
#40939=CARTESIAN_POINT('Ctrl Pts',(-37.936431619208,91.0320949202345,118.53024219305));
#40940=CARTESIAN_POINT('Ctrl Pts',(-34.4867513215705,90.8768946709331,118.372293669858));
#40941=CARTESIAN_POINT('Ctrl Pts',(-32.7308882545334,87.903457911076,118.214345146665));
#40942=CARTESIAN_POINT('Ctrl Pts',(-34.2608300589376,84.8077093184867,118.056396623473));
#40943=CARTESIAN_POINT('Ctrl Pts',(-37.6894250317483,84.3964699888117,117.89844810028));
#40944=CARTESIAN_POINT('Ctrl Pts',(-39.3187091718957,86.3396803259367,117.782457041515));
#40945=CARTESIAN_POINT('Ctrl Pts',(-39.431304611764,87.5596286627648,117.719115490481));
#40946=CARTESIAN_POINT('Ctrl Pts',(-39.4294365974543,87.7658979721433,117.708423447178));
#40947=CARTESIAN_POINT('Ctrl Pts',(-39.4262428442554,87.7660847244363,118.791576552823));
#40948=CARTESIAN_POINT('Ctrl Pts',(-39.4208793710626,88.4656307056646,118.755411372868));
#40949=CARTESIAN_POINT('Ctrl Pts',(-38.8380241483227,90.1916660269312,118.666596685182));
#40950=CARTESIAN_POINT('Ctrl Pts',(-35.9808934930197,91.3757634804708,118.525132489766));
#40951=CARTESIAN_POINT('Ctrl Pts',(-33.1299553615612,89.4272939776113,118.367183966573));
#40952=CARTESIAN_POINT('Ctrl Pts',(-33.2030000939727,85.9748968269957,118.209235443381));
#40953=CARTESIAN_POINT('Ctrl Pts',(-36.1338002509514,84.1487555231856,118.051286920188));
#40954=CARTESIAN_POINT('Ctrl Pts',(-38.8937930554849,85.4319514804777,117.912067290002));
#40955=CARTESIAN_POINT('Ctrl Pts',(-39.4210762304975,87.1139672109572,117.825497167547));
#40956=CARTESIAN_POINT('Ctrl Pts',(-39.4252303152106,87.7706425236776,117.791576552823));
#40957=CARTESIAN_POINT('Origin',(-36.3549260746835,87.7685555885722,124.208423447177));
#40958=CARTESIAN_POINT('',(-39.4334141302851,87.7688891883186,119.791576552823));
#40959=CARTESIAN_POINT('',(-39.4237430776497,87.7692166139293,119.708423447177));
#40960=CARTESIAN_POINT('',(-39.4284260746835,87.7685555885726,124.208423447177));
#40961=CARTESIAN_POINT('Ctrl Pts',(-39.4237430776497,87.7692166139293,119.708423447177));
#40962=CARTESIAN_POINT('Ctrl Pts',(-39.4246536306605,88.2379011782348,119.684242916584));
#40963=CARTESIAN_POINT('Ctrl Pts',(-39.1042498569938,89.725896099133,119.60741287826));
#40964=CARTESIAN_POINT('Ctrl Pts',(-36.7983710620289,91.3678895774169,119.477933332205));
#40965=CARTESIAN_POINT('Ctrl Pts',(-33.583435116581,90.1075054942073,119.319984809013));
#40966=CARTESIAN_POINT('Ctrl Pts',(-32.8813257256701,86.7264666342663,119.16203628582));
#40967=CARTESIAN_POINT('Ctrl Pts',(-35.3286241293906,84.2902581516539,119.004087762628));
#40968=CARTESIAN_POINT('Ctrl Pts',(-38.5622099696999,84.977081421696,118.85288348308));
#40969=CARTESIAN_POINT('Ctrl Pts',(-39.4247354269905,86.8866115094499,118.754328711263));
#40970=CARTESIAN_POINT('Ctrl Pts',(-39.431572198619,87.7706143825889,118.708423447177));
#40971=CARTESIAN_POINT('Ctrl Pts',(-39.4334141302851,87.7688891883186,119.791576552823));
#40972=CARTESIAN_POINT('Ctrl Pts',(-39.4334425751163,87.7871921571854,119.79062459365));
#40973=CARTESIAN_POINT('Ctrl Pts',(-39.4250379322418,88.817741027474,119.737023126747));
#40974=CARTESIAN_POINT('Ctrl Pts',(-38.2826267686962,90.8403332500451,119.630772152113));
#40975=CARTESIAN_POINT('Ctrl Pts',(-34.8365760655942,91.0619524059114,119.47282362892));
#40976=CARTESIAN_POINT('Ctrl Pts',(-32.7671669298757,88.2975486234688,119.314875105728));
#40977=CARTESIAN_POINT('Ctrl Pts',(-33.9506699948071,85.0535230461015,119.156926582536));
#40978=CARTESIAN_POINT('Ctrl Pts',(-37.3140388761979,84.2711348517919,118.998978059343));
#40979=CARTESIAN_POINT('Ctrl Pts',(-39.2368153757742,86.1128345328268,118.877194716105));
#40980=CARTESIAN_POINT('Ctrl Pts',(-39.4286875507449,87.4472270479811,118.808060880599));
#40981=CARTESIAN_POINT('Ctrl Pts',(-39.4262428442554,87.7660847244363,118.791576552823));
#40982=CARTESIAN_POINT('Origin',(-36.3549260746835,87.7685555885722,124.208423447177));
#40983=CARTESIAN_POINT('',(-39.4253674987814,87.7707064726519,120.791576552823));
#40984=CARTESIAN_POINT('',(-39.4292403360613,87.7658718692203,120.708423447177));
#40985=CARTESIAN_POINT('',(-39.4284260746835,87.7685555885726,124.208423447177));
#40986=CARTESIAN_POINT('Ctrl Pts',(-39.4292403360613,87.7658718692203,120.708423447177));
#40987=CARTESIAN_POINT('Ctrl Pts',(-39.4219532081813,88.5688690551349,120.666806629636));
#40988=CARTESIAN_POINT('Ctrl Pts',(-38.6905684542124,90.39950630607,120.572540304363));
#40989=CARTESIAN_POINT('Ctrl Pts',(-35.6128383024604,91.3183647084341,120.42562447136));
#40990=CARTESIAN_POINT('Ctrl Pts',(-32.9768144078577,89.0877262726116,120.267675948167));
#40991=CARTESIAN_POINT('Ctrl Pts',(-33.4036211604692,85.6610333840612,120.109727424975));
#40992=CARTESIAN_POINT('Ctrl Pts',(-36.5062865428284,84.1451680035439,119.951778901782));
#40993=CARTESIAN_POINT('Ctrl Pts',(-39.0177364100551,85.6436455182526,119.818010909183));
#40994=CARTESIAN_POINT('Ctrl Pts',(-39.4226710369536,87.21741027145,119.736892424315));
#40995=CARTESIAN_POINT('Ctrl Pts',(-39.4237430776497,87.7692166139293,119.708423447177));
#40996=CARTESIAN_POINT('Ctrl Pts',(-39.4253674987814,87.7707064726519,120.791576552823));
#40997=CARTESIAN_POINT('Ctrl Pts',(-39.4277028283381,88.1266499402521,120.773188306702));
#40998=CARTESIAN_POINT('Ctrl Pts',(-39.2066380294348,89.4989306286966,120.70215055285));
#40999=CARTESIAN_POINT('Ctrl Pts',(-37.1879238856457,91.2981286694523,120.578463291268));
#41000=CARTESIAN_POINT('Ctrl Pts',(-33.854806193682,90.395578791602,120.420514768075));
#41001=CARTESIAN_POINT('Ctrl Pts',(-32.7884554748253,87.1111711244642,120.262566244883));
#41002=CARTESIAN_POINT('Ctrl Pts',(-34.9557228065637,84.4228016151801,120.10461772169));
#41003=CARTESIAN_POINT('Ctrl Pts',(-38.3708933628005,84.765841706942,119.94762115767));
#41004=CARTESIAN_POINT('Ctrl Pts',(-39.4318693917246,86.7749194370741,119.843274101381));
#41005=CARTESIAN_POINT('Ctrl Pts',(-39.4334141302851,87.7688891883186,119.791576552823));
#41006=CARTESIAN_POINT('Origin',(-36.3549260746835,87.7685555885722,124.208423447177));
#41007=CARTESIAN_POINT('',(-39.4252046869538,87.7655406593158,121.791576552823));
#41008=CARTESIAN_POINT('',(-39.4317255112881,87.7704831500192,121.708423447178));
#41009=CARTESIAN_POINT('',(-39.4284260746835,87.7685555885726,124.208423447177));
#41010=CARTESIAN_POINT('',(-37.1487253572166,84.7993326348266,122.));
#41011=CARTESIAN_POINT('Ctrl Pts',(-37.1487253572165,84.7993326348266,122.));
#41012=CARTESIAN_POINT('Ctrl Pts',(-38.1309639469882,85.0619266872043,121.947350492269));
#41013=CARTESIAN_POINT('Ctrl Pts',(-39.230660578184,86.0996636740867,121.877876009877));
#41014=CARTESIAN_POINT('Ctrl Pts',(-39.427545857155,87.4400648792359,121.808401527484));
#41015=CARTESIAN_POINT('Ctrl Pts',(-39.4252046869538,87.7655406593158,121.791576552823));
#41016=CARTESIAN_POINT('',(-35.5592173411396,84.7942562942729,122.));
#41017=CARTESIAN_POINT('Origin',(-36.3549260746835,87.7685555885722,122.));
#41018=CARTESIAN_POINT('Ctrl Pts',(-35.5592127063049,84.794243972407,122.));
#41019=CARTESIAN_POINT('Ctrl Pts',(-36.5061791034278,84.5433632593369,121.949053726697));
#41020=CARTESIAN_POINT('Ctrl Pts',(-38.5667276181166,84.9982655567983,121.851861542423));
#41021=CARTESIAN_POINT('Ctrl Pts',(-39.4250619982496,86.8802085250801,121.754669358149));
#41022=CARTESIAN_POINT('Ctrl Pts',(-39.4317255112881,87.7704831500192,121.708423447178));
#41023=CARTESIAN_POINT('Origin',(0.,-94.,92.));
#41024=CARTESIAN_POINT('',(0.,-100.,94.));
#41025=CARTESIAN_POINT('',(0.,-100.,90.));
#41026=CARTESIAN_POINT('Ctrl Pts',(8.32667268468867E-16,-100.,94.));
#41027=CARTESIAN_POINT('Ctrl Pts',(0.251131643913751,-100.,94.));
#41028=CARTESIAN_POINT('Ctrl Pts',(0.518997821386429,-99.998956730068,93.9498099158249));
#41029=CARTESIAN_POINT('Ctrl Pts',(1.01175449350969,-99.995185177515,93.7457005158259));
#41030=CARTESIAN_POINT('Ctrl Pts',(1.23664555394558,-99.9925109419644,93.5917815708006));
#41031=CARTESIAN_POINT('Ctrl Pts',(1.591781571759,-99.9874880579221,93.2366455529872));
#41032=CARTESIAN_POINT('Ctrl Pts',(1.74570051630388,-99.9848135889912,93.0117544930956));
#41033=CARTESIAN_POINT('Ctrl Pts',(1.94980991520061,-99.9810415029486,92.5189978221538));
#41034=CARTESIAN_POINT('Ctrl Pts',(2.,-99.9799979995999,92.2511316452692));
#41035=CARTESIAN_POINT('Ctrl Pts',(2.,-99.9799979995999,91.7488683547308));
#41036=CARTESIAN_POINT('Ctrl Pts',(1.94980991520062,-99.9810415029486,91.4810021778462));
#41037=CARTESIAN_POINT('Ctrl Pts',(1.7457005163039,-99.9848135889912,90.9882455069044));
#41038=CARTESIAN_POINT('Ctrl Pts',(1.591781571759,-99.9874880579221,90.7633544470128));
#41039=CARTESIAN_POINT('Ctrl Pts',(1.23664555394558,-99.9925109419644,90.4082184291994));
#41040=CARTESIAN_POINT('Ctrl Pts',(1.01175449350969,-99.995185177515,90.2542994841741));
#41041=CARTESIAN_POINT('Ctrl Pts',(0.518997821386429,-99.998956730068,90.050190084175));
#41042=CARTESIAN_POINT('Ctrl Pts',(0.251131643913753,-100.,90.));
#41043=CARTESIAN_POINT('Ctrl Pts',(2.4980018054066E-15,-100.,90.));
#41044=CARTESIAN_POINT('',(2.00527236333692E-16,-90.,94.));
#41045=CARTESIAN_POINT('',(2.44929359829471E-16,-94.,94.));
#41046=CARTESIAN_POINT('',(-2.,-89.9777750336159,92.));
#41047=CARTESIAN_POINT('Ctrl Pts',(-2.,-89.9777750336159,92.));
#41048=CARTESIAN_POINT('Ctrl Pts',(-2.,-89.9777750336159,91.7488666698803));
#41049=CARTESIAN_POINT('Ctrl Pts',(-1.94980925677131,-89.9789345539658,
91.480999766208));
#41050=CARTESIAN_POINT('Ctrl Pts',(-1.74569936855886,-89.9831259365723,
90.9882435581214));
#41051=CARTESIAN_POINT('Ctrl Pts',(-1.59178067978086,-89.9860976603374,
90.7633535550347));
#41052=CARTESIAN_POINT('Ctrl Pts',(-1.23664644642618,-89.9916787455059,
90.40821932168));
#41053=CARTESIAN_POINT('Ctrl Pts',(-1.01175644254643,-89.9946501491172,
90.2543006320885));
#41054=CARTESIAN_POINT('Ctrl Pts',(-0.519000232590767,-89.9988407998655,
90.0501907423603));
#41055=CARTESIAN_POINT('Ctrl Pts',(-0.251133328053566,-90.,90.));
#41056=CARTESIAN_POINT('Ctrl Pts',(0.251133328053566,-90.,90.));
#41057=CARTESIAN_POINT('Ctrl Pts',(0.519000232590767,-89.9988407998655,
90.0501907423603));
#41058=CARTESIAN_POINT('Ctrl Pts',(1.01175644254643,-89.9946501491172,90.2543006320885));
#41059=CARTESIAN_POINT('Ctrl Pts',(1.23664644642618,-89.9916787455059,90.40821932168));
#41060=CARTESIAN_POINT('Ctrl Pts',(1.59178067978086,-89.9860976603374,90.7633535550347));
#41061=CARTESIAN_POINT('Ctrl Pts',(1.74569936855888,-89.9831259365723,90.9882435581214));
#41062=CARTESIAN_POINT('Ctrl Pts',(1.94980925677131,-89.9789345539658,91.480999766208));
#41063=CARTESIAN_POINT('Ctrl Pts',(2.,-89.9777750336159,91.7488666698804));
#41064=CARTESIAN_POINT('Ctrl Pts',(2.,-89.9777750336159,92.2511333301196));
#41065=CARTESIAN_POINT('Ctrl Pts',(1.94980925677131,-89.9789345539658,92.519000233792));
#41066=CARTESIAN_POINT('Ctrl Pts',(1.74569936855886,-89.9831259365723,93.0117564418786));
#41067=CARTESIAN_POINT('Ctrl Pts',(1.59178067978086,-89.9860976603374,93.2366464449653));
#41068=CARTESIAN_POINT('Ctrl Pts',(1.23664644642618,-89.9916787455059,93.59178067832));
#41069=CARTESIAN_POINT('Ctrl Pts',(1.01175644254643,-89.9946501491172,93.7456993679115));
#41070=CARTESIAN_POINT('Ctrl Pts',(0.519000232590768,-89.9988407998655,
93.9498092576397));
#41071=CARTESIAN_POINT('Ctrl Pts',(0.251133328053567,-90.,94.));
#41072=CARTESIAN_POINT('Ctrl Pts',(3.46944695195361E-16,-90.,94.));
#41073=CARTESIAN_POINT('Ctrl Pts',(1.56125112837913E-16,-90.,94.));
#41074=CARTESIAN_POINT('Ctrl Pts',(-0.251133328053566,-90.,94.));
#41075=CARTESIAN_POINT('Ctrl Pts',(-0.519000232590761,-89.9988407998655,
93.9498092576397));
#41076=CARTESIAN_POINT('Ctrl Pts',(-1.01175644254643,-89.9946501491172,
93.7456993679115));
#41077=CARTESIAN_POINT('Ctrl Pts',(-1.23664644642618,-89.9916787455059,
93.59178067832));
#41078=CARTESIAN_POINT('Ctrl Pts',(-1.59178067978086,-89.9860976603374,
93.2366464449653));
#41079=CARTESIAN_POINT('Ctrl Pts',(-1.74569936855886,-89.9831259365723,
93.0117564418786));
#41080=CARTESIAN_POINT('Ctrl Pts',(-1.94980925677131,-89.9789345539658,
92.519000233792));
#41081=CARTESIAN_POINT('Ctrl Pts',(-2.,-89.9777750336159,92.2511333301196));
#41082=CARTESIAN_POINT('Ctrl Pts',(-2.,-89.9777750336159,92.));
#41083=CARTESIAN_POINT('Ctrl Pts',(-6.93889390390723E-16,-100.,90.));
#41084=CARTESIAN_POINT('Ctrl Pts',(-0.251131643913751,-100.,90.));
#41085=CARTESIAN_POINT('Ctrl Pts',(-0.518997821386429,-99.998956730068,
90.050190084175));
#41086=CARTESIAN_POINT('Ctrl Pts',(-1.01175449350969,-99.995185177515,90.2542994841741));
#41087=CARTESIAN_POINT('Ctrl Pts',(-1.23664555394558,-99.9925109419644,
90.4082184291994));
#41088=CARTESIAN_POINT('Ctrl Pts',(-1.591781571759,-99.9874880579221,90.7633544470128));
#41089=CARTESIAN_POINT('Ctrl Pts',(-1.74570051630388,-99.9848135889912,
90.9882455069044));
#41090=CARTESIAN_POINT('Ctrl Pts',(-1.94980991520061,-99.9810415029486,
91.4810021778462));
#41091=CARTESIAN_POINT('Ctrl Pts',(-2.,-99.9799979995999,91.7488683547308));
#41092=CARTESIAN_POINT('Ctrl Pts',(-2.,-99.9799979995999,92.));
#41093=CARTESIAN_POINT('Ctrl Pts',(-2.,-99.9799979995999,92.2511316452692));
#41094=CARTESIAN_POINT('Ctrl Pts',(-1.94980991520061,-99.9810415029486,
92.5189978221538));
#41095=CARTESIAN_POINT('Ctrl Pts',(-1.74570051630388,-99.9848135889912,
93.0117544930956));
#41096=CARTESIAN_POINT('Ctrl Pts',(-1.591781571759,-99.9874880579221,93.2366455529872));
#41097=CARTESIAN_POINT('Ctrl Pts',(-1.23664555394558,-99.9925109419644,
93.5917815708006));
#41098=CARTESIAN_POINT('Ctrl Pts',(-1.01175449350969,-99.995185177515,93.7457005158259));
#41099=CARTESIAN_POINT('Ctrl Pts',(-0.518997821386429,-99.998956730068,
93.9498099158249));
#41100=CARTESIAN_POINT('Ctrl Pts',(-0.251131643913751,-100.,94.));
#41101=CARTESIAN_POINT('Ctrl Pts',(-7.63278329429795E-16,-100.,94.));
#41102=CARTESIAN_POINT('Origin',(0.,94.,92.));
#41103=CARTESIAN_POINT('',(0.,100.,94.));
#41104=CARTESIAN_POINT('',(0.,100.,90.));
#41105=CARTESIAN_POINT('Ctrl Pts',(2.77555756156289E-16,100.,94.));
#41106=CARTESIAN_POINT('Ctrl Pts',(-0.25113164391375,100.,94.));
#41107=CARTESIAN_POINT('Ctrl Pts',(-0.518997821386429,99.998956730068,93.9498099158249));
#41108=CARTESIAN_POINT('Ctrl Pts',(-1.01175449350969,99.995185177515,93.7457005158259));
#41109=CARTESIAN_POINT('Ctrl Pts',(-1.23664555394558,99.9925109419644,93.5917815708006));
#41110=CARTESIAN_POINT('Ctrl Pts',(-1.591781571759,99.9874880579221,93.2366455529872));
#41111=CARTESIAN_POINT('Ctrl Pts',(-1.74570051630388,99.9848135889912,93.0117544930956));
#41112=CARTESIAN_POINT('Ctrl Pts',(-1.94980991520061,99.9810415029486,92.5189978221538));
#41113=CARTESIAN_POINT('Ctrl Pts',(-2.,99.9799979995999,92.2511316452692));
#41114=CARTESIAN_POINT('Ctrl Pts',(-2.,99.9799979995999,91.7488683547308));
#41115=CARTESIAN_POINT('Ctrl Pts',(-1.94980991520061,99.9810415029486,91.4810021778462));
#41116=CARTESIAN_POINT('Ctrl Pts',(-1.74570051630388,99.9848135889912,90.9882455069044));
#41117=CARTESIAN_POINT('Ctrl Pts',(-1.591781571759,99.9874880579221,90.7633544470128));
#41118=CARTESIAN_POINT('Ctrl Pts',(-1.23664555394558,99.9925109419644,90.4082184291994));
#41119=CARTESIAN_POINT('Ctrl Pts',(-1.01175449350969,99.995185177515,90.2542994841741));
#41120=CARTESIAN_POINT('Ctrl Pts',(-0.518997821386428,99.998956730068,90.050190084175));
#41121=CARTESIAN_POINT('Ctrl Pts',(-0.251131643913752,100.,90.));
#41122=CARTESIAN_POINT('Ctrl Pts',(-2.28983498828939E-15,100.,90.));
#41123=CARTESIAN_POINT('Ctrl Pts',(1.94289029309402E-15,100.,90.));
#41124=CARTESIAN_POINT('Ctrl Pts',(0.251131643913752,100.,90.));
#41125=CARTESIAN_POINT('Ctrl Pts',(0.518997821386421,99.998956730068,90.050190084175));
#41126=CARTESIAN_POINT('Ctrl Pts',(1.01175449350969,99.995185177515,90.2542994841741));
#41127=CARTESIAN_POINT('Ctrl Pts',(1.23664555394558,99.9925109419644,90.4082184291994));
#41128=CARTESIAN_POINT('Ctrl Pts',(1.591781571759,99.9874880579221,90.7633544470128));
#41129=CARTESIAN_POINT('Ctrl Pts',(1.74570051630388,99.9848135889912,90.9882455069044));
#41130=CARTESIAN_POINT('Ctrl Pts',(1.94980991520061,99.9810415029486,91.4810021778462));
#41131=CARTESIAN_POINT('Ctrl Pts',(2.,99.9799979995999,91.7488683547308));
#41132=CARTESIAN_POINT('Ctrl Pts',(2.,99.9799979995999,92.));
#41133=CARTESIAN_POINT('Ctrl Pts',(2.,99.9799979995999,92.2511316452692));
#41134=CARTESIAN_POINT('Ctrl Pts',(1.94980991520061,99.9810415029486,92.5189978221538));
#41135=CARTESIAN_POINT('Ctrl Pts',(1.74570051630388,99.9848135889912,93.0117544930956));
#41136=CARTESIAN_POINT('Ctrl Pts',(1.591781571759,99.9874880579221,93.2366455529872));
#41137=CARTESIAN_POINT('Ctrl Pts',(1.23664555394558,99.9925109419644,93.5917815708006));
#41138=CARTESIAN_POINT('Ctrl Pts',(1.01175449350969,99.995185177515,93.7457005158259));
#41139=CARTESIAN_POINT('Ctrl Pts',(0.518997821386429,99.998956730068,93.9498099158249));
#41140=CARTESIAN_POINT('Ctrl Pts',(0.25113164391375,100.,94.));
#41141=CARTESIAN_POINT('Ctrl Pts',(-3.46944695195361E-17,100.,94.));
#41142=CARTESIAN_POINT('',(7.46965131266386E-16,90.,90.));
#41143=CARTESIAN_POINT('',(2.44929359829471E-16,94.,90.));
#41144=CARTESIAN_POINT('',(2.,89.9777750336159,92.));
#41145=CARTESIAN_POINT('Ctrl Pts',(2.,89.9777750336159,92.));
#41146=CARTESIAN_POINT('Ctrl Pts',(2.,89.9777750336159,91.7488666698804));
#41147=CARTESIAN_POINT('Ctrl Pts',(1.94980925677131,89.9789345539658,91.480999766208));
#41148=CARTESIAN_POINT('Ctrl Pts',(1.74569936855886,89.9831259365723,90.9882435581214));
#41149=CARTESIAN_POINT('Ctrl Pts',(1.59178067978086,89.9860976603374,90.7633535550347));
#41150=CARTESIAN_POINT('Ctrl Pts',(1.23664644642618,89.9916787455059,90.40821932168));
#41151=CARTESIAN_POINT('Ctrl Pts',(1.01175644254643,89.9946501491172,90.2543006320885));
#41152=CARTESIAN_POINT('Ctrl Pts',(0.519000232590768,89.9988407998655,90.0501907423603));
#41153=CARTESIAN_POINT('Ctrl Pts',(0.251133328053566,90.,90.));
#41154=CARTESIAN_POINT('Ctrl Pts',(-2.08166817117217E-16,90.,90.));
#41155=CARTESIAN_POINT('Ctrl Pts',(1.2490009027033E-15,90.,90.));
#41156=CARTESIAN_POINT('Ctrl Pts',(-0.251133328053565,90.,90.));
#41157=CARTESIAN_POINT('Ctrl Pts',(-0.519000232590767,89.9988407998655,
90.0501907423603));
#41158=CARTESIAN_POINT('Ctrl Pts',(-1.01175644254643,89.9946501491172,90.2543006320885));
#41159=CARTESIAN_POINT('Ctrl Pts',(-1.23664644642618,89.9916787455059,90.40821932168));
#41160=CARTESIAN_POINT('Ctrl Pts',(-1.59178067978086,89.9860976603374,90.7633535550347));
#41161=CARTESIAN_POINT('Ctrl Pts',(-1.74569936855888,89.9831259365723,90.9882435581214));
#41162=CARTESIAN_POINT('Ctrl Pts',(-1.94980925677131,89.9789345539658,91.480999766208));
#41163=CARTESIAN_POINT('Ctrl Pts',(-2.,89.9777750336159,91.7488666698804));
#41164=CARTESIAN_POINT('Ctrl Pts',(-2.,89.9777750336159,92.2511333301196));
#41165=CARTESIAN_POINT('Ctrl Pts',(-1.94980925677131,89.9789345539658,92.519000233792));
#41166=CARTESIAN_POINT('Ctrl Pts',(-1.74569936855886,89.9831259365723,93.0117564418786));
#41167=CARTESIAN_POINT('Ctrl Pts',(-1.59178067978086,89.9860976603374,93.2366464449653));
#41168=CARTESIAN_POINT('Ctrl Pts',(-1.23664644642618,89.9916787455059,93.59178067832));
#41169=CARTESIAN_POINT('Ctrl Pts',(-1.01175644254643,89.9946501491172,93.7456993679115));
#41170=CARTESIAN_POINT('Ctrl Pts',(-0.519000232590768,89.9988407998655,
93.9498092576397));
#41171=CARTESIAN_POINT('Ctrl Pts',(-0.251133328053566,90.,94.));
#41172=CARTESIAN_POINT('Ctrl Pts',(0.251133328053566,90.,94.));
#41173=CARTESIAN_POINT('Ctrl Pts',(0.519000232590767,89.9988407998655,93.9498092576397));
#41174=CARTESIAN_POINT('Ctrl Pts',(1.01175644254643,89.9946501491172,93.7456993679115));
#41175=CARTESIAN_POINT('Ctrl Pts',(1.23664644642618,89.9916787455059,93.59178067832));
#41176=CARTESIAN_POINT('Ctrl Pts',(1.59178067978086,89.9860976603374,93.2366464449653));
#41177=CARTESIAN_POINT('Ctrl Pts',(1.74569936855886,89.9831259365723,93.0117564418786));
#41178=CARTESIAN_POINT('Ctrl Pts',(1.94980925677131,89.9789345539658,92.519000233792));
#41179=CARTESIAN_POINT('Ctrl Pts',(2.,89.9777750336159,92.2511333301196));
#41180=CARTESIAN_POINT('Ctrl Pts',(2.,89.9777750336159,92.));
#41181=CARTESIAN_POINT('Origin',(-94.,0.,92.));
#41182=CARTESIAN_POINT('',(-100.,0.,94.));
#41183=CARTESIAN_POINT('',(-100.,0.,90.));
#41184=CARTESIAN_POINT('Ctrl Pts',(-100.,-8.32667268468867E-16,94.));
#41185=CARTESIAN_POINT('Ctrl Pts',(-100.,-0.251131643913751,94.));
#41186=CARTESIAN_POINT('Ctrl Pts',(-99.998956730068,-0.518997821386429,
93.9498099158249));
#41187=CARTESIAN_POINT('Ctrl Pts',(-99.995185177515,-1.01175449350969,93.7457005158259));
#41188=CARTESIAN_POINT('Ctrl Pts',(-99.9925109419644,-1.23664555394558,
93.5917815708006));
#41189=CARTESIAN_POINT('Ctrl Pts',(-99.9874880579221,-1.591781571759,93.2366455529872));
#41190=CARTESIAN_POINT('Ctrl Pts',(-99.9848135889912,-1.74570051630388,
93.0117544930956));
#41191=CARTESIAN_POINT('Ctrl Pts',(-99.9810415029486,-1.94980991520061,
92.5189978221538));
#41192=CARTESIAN_POINT('Ctrl Pts',(-99.9799979995999,-2.,92.2511316452692));
#41193=CARTESIAN_POINT('Ctrl Pts',(-99.9799979995999,-2.,91.7488683547308));
#41194=CARTESIAN_POINT('Ctrl Pts',(-99.9810415029486,-1.94980991520061,
91.4810021778462));
#41195=CARTESIAN_POINT('Ctrl Pts',(-99.9848135889912,-1.74570051630388,
90.9882455069044));
#41196=CARTESIAN_POINT('Ctrl Pts',(-99.9874880579221,-1.591781571759,90.7633544470128));
#41197=CARTESIAN_POINT('Ctrl Pts',(-99.9925109419644,-1.23664555394558,
90.4082184291994));
#41198=CARTESIAN_POINT('Ctrl Pts',(-99.995185177515,-1.01175449350969,90.2542994841741));
#41199=CARTESIAN_POINT('Ctrl Pts',(-99.998956730068,-0.518997821386429,
90.050190084175));
#41200=CARTESIAN_POINT('Ctrl Pts',(-100.,-0.251131643913753,90.));
#41201=CARTESIAN_POINT('Ctrl Pts',(-100.,-2.4980018054066E-15,90.));
#41202=CARTESIAN_POINT('',(-99.9799979995999,2.,92.));
#41203=CARTESIAN_POINT('Ctrl Pts',(-99.9799979995999,2.,92.));
#41204=CARTESIAN_POINT('Ctrl Pts',(-99.9799979995999,2.,92.2511316452692));
#41205=CARTESIAN_POINT('Ctrl Pts',(-99.9810415029486,1.94980991520061,92.5189978221538));
#41206=CARTESIAN_POINT('Ctrl Pts',(-99.9848135889912,1.74570051630388,93.0117544930956));
#41207=CARTESIAN_POINT('Ctrl Pts',(-99.9874880579221,1.591781571759,93.2366455529872));
#41208=CARTESIAN_POINT('Ctrl Pts',(-99.9925109419644,1.23664555394558,93.5917815708006));
#41209=CARTESIAN_POINT('Ctrl Pts',(-99.995185177515,1.01175449350969,93.7457005158259));
#41210=CARTESIAN_POINT('Ctrl Pts',(-99.998956730068,0.518997821386429,93.9498099158249));
#41211=CARTESIAN_POINT('Ctrl Pts',(-100.,0.251131643913751,94.));
#41212=CARTESIAN_POINT('Ctrl Pts',(-100.,2.42861286636753E-16,94.));
#41213=CARTESIAN_POINT('',(-89.9777750336159,2.,92.));
#41214=CARTESIAN_POINT('',(-94.,2.,92.));
#41215=CARTESIAN_POINT('',(-90.,-5.47621612664355E-15,94.));
#41216=CARTESIAN_POINT('Ctrl Pts',(-90.,3.46944695195361E-16,94.));
#41217=CARTESIAN_POINT('Ctrl Pts',(-90.,0.251133328053567,94.));
#41218=CARTESIAN_POINT('Ctrl Pts',(-89.9988407998655,0.519000232590767,
93.9498092576397));
#41219=CARTESIAN_POINT('Ctrl Pts',(-89.9946501491172,1.01175644254643,93.7456993679115));
#41220=CARTESIAN_POINT('Ctrl Pts',(-89.9916787455059,1.23664644642618,93.59178067832));
#41221=CARTESIAN_POINT('Ctrl Pts',(-89.9860976603374,1.59178067978086,93.2366464449653));
#41222=CARTESIAN_POINT('Ctrl Pts',(-89.9831259365723,1.74569936855886,93.0117564418786));
#41223=CARTESIAN_POINT('Ctrl Pts',(-89.9789345539658,1.94980925677131,92.519000233792));
#41224=CARTESIAN_POINT('Ctrl Pts',(-89.9777750336159,2.,92.2511333301196));
#41225=CARTESIAN_POINT('Ctrl Pts',(-89.9777750336159,2.,92.));
#41226=CARTESIAN_POINT('',(-90.,-5.16396590096773E-15,90.));
#41227=CARTESIAN_POINT('Ctrl Pts',(-90.,6.93889390390723E-16,90.));
#41228=CARTESIAN_POINT('Ctrl Pts',(-90.,-0.251133328053566,90.));
#41229=CARTESIAN_POINT('Ctrl Pts',(-89.9988407998655,-0.519000232590767,
90.0501907423603));
#41230=CARTESIAN_POINT('Ctrl Pts',(-89.9946501491172,-1.01175644254643,
90.2543006320885));
#41231=CARTESIAN_POINT('Ctrl Pts',(-89.9916787455059,-1.23664644642618,
90.40821932168));
#41232=CARTESIAN_POINT('Ctrl Pts',(-89.9860976603374,-1.59178067978086,
90.7633535550347));
#41233=CARTESIAN_POINT('Ctrl Pts',(-89.9831259365723,-1.74569936855888,
90.9882435581214));
#41234=CARTESIAN_POINT('Ctrl Pts',(-89.9789345539658,-1.94980925677131,
91.480999766208));
#41235=CARTESIAN_POINT('Ctrl Pts',(-89.9777750336159,-2.,91.7488666698804));
#41236=CARTESIAN_POINT('Ctrl Pts',(-89.9777750336159,-2.,92.2511333301196));
#41237=CARTESIAN_POINT('Ctrl Pts',(-89.9789345539658,-1.94980925677131,
92.519000233792));
#41238=CARTESIAN_POINT('Ctrl Pts',(-89.9831259365723,-1.74569936855886,
93.0117564418786));
#41239=CARTESIAN_POINT('Ctrl Pts',(-89.9860976603374,-1.59178067978086,
93.2366464449653));
#41240=CARTESIAN_POINT('Ctrl Pts',(-89.9916787455059,-1.23664644642618,
93.59178067832));
#41241=CARTESIAN_POINT('Ctrl Pts',(-89.9946501491172,-1.01175644254643,
93.7456993679115));
#41242=CARTESIAN_POINT('Ctrl Pts',(-89.9988407998655,-0.519000232590767,
93.9498092576397));
#41243=CARTESIAN_POINT('Ctrl Pts',(-90.,-0.251133328053567,94.));
#41244=CARTESIAN_POINT('Ctrl Pts',(-90.,-4.16333634234434E-16,94.));
#41245=CARTESIAN_POINT('Ctrl Pts',(-89.9777750336159,2.,92.));
#41246=CARTESIAN_POINT('Ctrl Pts',(-89.9777750336159,2.,91.7488666698804));
#41247=CARTESIAN_POINT('Ctrl Pts',(-89.9789345539658,1.94980925677131,91.480999766208));
#41248=CARTESIAN_POINT('Ctrl Pts',(-89.9831259365723,1.74569936855886,90.9882435581214));
#41249=CARTESIAN_POINT('Ctrl Pts',(-89.9860976603374,1.59178067978086,90.7633535550347));
#41250=CARTESIAN_POINT('Ctrl Pts',(-89.9916787455059,1.23664644642618,90.40821932168));
#41251=CARTESIAN_POINT('Ctrl Pts',(-89.9946501491172,1.01175644254643,90.2543006320885));
#41252=CARTESIAN_POINT('Ctrl Pts',(-89.9988407998655,0.519000232590768,
90.0501907423603));
#41253=CARTESIAN_POINT('Ctrl Pts',(-90.,0.251133328053566,90.));
#41254=CARTESIAN_POINT('Ctrl Pts',(-90.,-4.85722573273506E-16,90.));
#41255=CARTESIAN_POINT('Ctrl Pts',(-100.,3.12250225675825E-16,90.));
#41256=CARTESIAN_POINT('Ctrl Pts',(-100.,0.25113164391375,90.));
#41257=CARTESIAN_POINT('Ctrl Pts',(-99.998956730068,0.518997821386421,90.050190084175));
#41258=CARTESIAN_POINT('Ctrl Pts',(-99.995185177515,1.01175449350969,90.2542994841741));
#41259=CARTESIAN_POINT('Ctrl Pts',(-99.9925109419644,1.23664555394558,90.4082184291994));
#41260=CARTESIAN_POINT('Ctrl Pts',(-99.9874880579221,1.591781571759,90.7633544470128));
#41261=CARTESIAN_POINT('Ctrl Pts',(-99.9848135889912,1.74570051630388,90.9882455069044));
#41262=CARTESIAN_POINT('Ctrl Pts',(-99.9810415029486,1.94980991520061,91.4810021778462));
#41263=CARTESIAN_POINT('Ctrl Pts',(-99.9799979995999,2.,91.7488683547308));
#41264=CARTESIAN_POINT('Ctrl Pts',(-99.9799979995999,2.,92.));
#41265=CARTESIAN_POINT('Origin',(94.,0.,92.));
#41266=CARTESIAN_POINT('',(100.,0.,94.));
#41267=CARTESIAN_POINT('',(100.,0.,90.));
#41268=CARTESIAN_POINT('Ctrl Pts',(100.,8.32667268468867E-16,94.));
#41269=CARTESIAN_POINT('Ctrl Pts',(100.,0.251131643913751,94.));
#41270=CARTESIAN_POINT('Ctrl Pts',(99.998956730068,0.518997821386429,93.9498099158249));
#41271=CARTESIAN_POINT('Ctrl Pts',(99.995185177515,1.01175449350969,93.7457005158259));
#41272=CARTESIAN_POINT('Ctrl Pts',(99.9925109419644,1.23664555394558,93.5917815708006));
#41273=CARTESIAN_POINT('Ctrl Pts',(99.9874880579221,1.591781571759,93.2366455529872));
#41274=CARTESIAN_POINT('Ctrl Pts',(99.9848135889912,1.74570051630388,93.0117544930956));
#41275=CARTESIAN_POINT('Ctrl Pts',(99.9810415029486,1.94980991520061,92.5189978221538));
#41276=CARTESIAN_POINT('Ctrl Pts',(99.9799979995999,2.,92.2511316452692));
#41277=CARTESIAN_POINT('Ctrl Pts',(99.9799979995999,2.,91.7488683547308));
#41278=CARTESIAN_POINT('Ctrl Pts',(99.9810415029486,1.94980991520061,91.4810021778462));
#41279=CARTESIAN_POINT('Ctrl Pts',(99.9848135889912,1.74570051630388,90.9882455069044));
#41280=CARTESIAN_POINT('Ctrl Pts',(99.9874880579221,1.591781571759,90.7633544470128));
#41281=CARTESIAN_POINT('Ctrl Pts',(99.9925109419644,1.23664555394558,90.4082184291994));
#41282=CARTESIAN_POINT('Ctrl Pts',(99.995185177515,1.01175449350969,90.2542994841741));
#41283=CARTESIAN_POINT('Ctrl Pts',(99.998956730068,0.518997821386429,90.050190084175));
#41284=CARTESIAN_POINT('Ctrl Pts',(100.,0.251131643913753,90.));
#41285=CARTESIAN_POINT('Ctrl Pts',(100.,2.4980018054066E-15,90.));
#41286=CARTESIAN_POINT('',(99.9799979995999,-2.,92.));
#41287=CARTESIAN_POINT('Ctrl Pts',(99.9799979995999,-2.,92.));
#41288=CARTESIAN_POINT('Ctrl Pts',(99.9799979995999,-2.,92.2511316452692));
#41289=CARTESIAN_POINT('Ctrl Pts',(99.9810415029486,-1.94980991520061,92.5189978221538));
#41290=CARTESIAN_POINT('Ctrl Pts',(99.9848135889912,-1.74570051630388,93.0117544930956));
#41291=CARTESIAN_POINT('Ctrl Pts',(99.9874880579221,-1.591781571759,93.2366455529872));
#41292=CARTESIAN_POINT('Ctrl Pts',(99.9925109419644,-1.23664555394558,93.5917815708006));
#41293=CARTESIAN_POINT('Ctrl Pts',(99.995185177515,-1.01175449350969,93.7457005158259));
#41294=CARTESIAN_POINT('Ctrl Pts',(99.998956730068,-0.518997821386429,93.9498099158249));
#41295=CARTESIAN_POINT('Ctrl Pts',(100.,-0.251131643913751,94.));
#41296=CARTESIAN_POINT('Ctrl Pts',(100.,-2.42861286636753E-16,94.));
#41297=CARTESIAN_POINT('',(89.9777750336159,-2.,92.));
#41298=CARTESIAN_POINT('',(94.,-2.,92.));
#41299=CARTESIAN_POINT('Ctrl Pts',(89.9777750336159,-2.,92.));
#41300=CARTESIAN_POINT('Ctrl Pts',(89.9777750336159,-2.,91.7488666698804));
#41301=CARTESIAN_POINT('Ctrl Pts',(89.9789345539658,-1.94980925677131,91.480999766208));
#41302=CARTESIAN_POINT('Ctrl Pts',(89.9831259365723,-1.74569936855886,90.9882435581214));
#41303=CARTESIAN_POINT('Ctrl Pts',(89.9860976603374,-1.59178067978086,90.7633535550347));
#41304=CARTESIAN_POINT('Ctrl Pts',(89.9916787455059,-1.23664644642618,90.40821932168));
#41305=CARTESIAN_POINT('Ctrl Pts',(89.9946501491172,-1.01175644254643,90.2543006320885));
#41306=CARTESIAN_POINT('Ctrl Pts',(89.9988407998655,-0.519000232590768,
90.0501907423603));
#41307=CARTESIAN_POINT('Ctrl Pts',(90.,-0.251133328053566,90.));
#41308=CARTESIAN_POINT('Ctrl Pts',(90.,0.251133328053566,90.));
#41309=CARTESIAN_POINT('Ctrl Pts',(89.9988407998655,0.519000232590767,90.0501907423603));
#41310=CARTESIAN_POINT('Ctrl Pts',(89.9946501491172,1.01175644254643,90.2543006320885));
#41311=CARTESIAN_POINT('Ctrl Pts',(89.9916787455059,1.23664644642618,90.40821932168));
#41312=CARTESIAN_POINT('Ctrl Pts',(89.9860976603374,1.59178067978086,90.7633535550347));
#41313=CARTESIAN_POINT('Ctrl Pts',(89.9831259365723,1.74569936855888,90.9882435581214));
#41314=CARTESIAN_POINT('Ctrl Pts',(89.9789345539658,1.94980925677131,91.480999766208));
#41315=CARTESIAN_POINT('Ctrl Pts',(89.9777750336159,2.,91.7488666698804));
#41316=CARTESIAN_POINT('Ctrl Pts',(89.9777750336159,2.,92.2511333301196));
#41317=CARTESIAN_POINT('Ctrl Pts',(89.9789345539658,1.94980925677131,92.519000233792));
#41318=CARTESIAN_POINT('Ctrl Pts',(89.9831259365723,1.74569936855886,93.0117564418786));
#41319=CARTESIAN_POINT('Ctrl Pts',(89.9860976603374,1.59178067978086,93.2366464449653));
#41320=CARTESIAN_POINT('Ctrl Pts',(89.9916787455059,1.23664644642618,93.59178067832));
#41321=CARTESIAN_POINT('Ctrl Pts',(89.9946501491172,1.01175644254643,93.7456993679115));
#41322=CARTESIAN_POINT('Ctrl Pts',(89.9988407998655,0.519000232590767,93.9498092576397));
#41323=CARTESIAN_POINT('Ctrl Pts',(90.,0.251133328053566,94.));
#41324=CARTESIAN_POINT('Ctrl Pts',(90.,-0.251133328053566,94.));
#41325=CARTESIAN_POINT('Ctrl Pts',(89.9988407998655,-0.519000232590767,
93.9498092576397));
#41326=CARTESIAN_POINT('Ctrl Pts',(89.9946501491172,-1.01175644254643,93.7456993679115));
#41327=CARTESIAN_POINT('Ctrl Pts',(89.9916787455059,-1.23664644642618,93.59178067832));
#41328=CARTESIAN_POINT('Ctrl Pts',(89.9860976603374,-1.59178067978086,93.2366464449653));
#41329=CARTESIAN_POINT('Ctrl Pts',(89.9831259365723,-1.74569936855886,93.0117564418786));
#41330=CARTESIAN_POINT('Ctrl Pts',(89.9789345539658,-1.94980925677131,92.519000233792));
#41331=CARTESIAN_POINT('Ctrl Pts',(89.9777750336159,-2.,92.2511333301196));
#41332=CARTESIAN_POINT('Ctrl Pts',(89.9777750336159,-2.,92.));
#41333=CARTESIAN_POINT('Ctrl Pts',(100.,-3.12250225675825E-16,90.));
#41334=CARTESIAN_POINT('Ctrl Pts',(100.,-0.25113164391375,90.));
#41335=CARTESIAN_POINT('Ctrl Pts',(99.998956730068,-0.518997821386421,90.050190084175));
#41336=CARTESIAN_POINT('Ctrl Pts',(99.995185177515,-1.01175449350969,90.2542994841741));
#41337=CARTESIAN_POINT('Ctrl Pts',(99.9925109419644,-1.23664555394558,90.4082184291994));
#41338=CARTESIAN_POINT('Ctrl Pts',(99.9874880579221,-1.591781571759,90.7633544470128));
#41339=CARTESIAN_POINT('Ctrl Pts',(99.9848135889912,-1.74570051630388,90.9882455069044));
#41340=CARTESIAN_POINT('Ctrl Pts',(99.9810415029486,-1.94980991520061,91.4810021778462));
#41341=CARTESIAN_POINT('Ctrl Pts',(99.9799979995999,-2.,91.7488683547308));
#41342=CARTESIAN_POINT('Ctrl Pts',(99.9799979995999,-2.,92.));
#41343=CARTESIAN_POINT('Origin',(0.,-94.,70.));
#41344=CARTESIAN_POINT('',(0.,-100.,72.));
#41345=CARTESIAN_POINT('',(0.,-100.,68.));
#41346=CARTESIAN_POINT('Ctrl Pts',(-1.73472347597681E-15,-100.,72.));
#41347=CARTESIAN_POINT('Ctrl Pts',(0.251131643913749,-100.,72.));
#41348=CARTESIAN_POINT('Ctrl Pts',(0.51899782138642,-99.998956730068,71.949809915825));
#41349=CARTESIAN_POINT('Ctrl Pts',(1.01175449350968,-99.995185177515,71.7457005158259));
#41350=CARTESIAN_POINT('Ctrl Pts',(1.23664555394557,-99.9925109419644,71.5917815708006));
#41351=CARTESIAN_POINT('Ctrl Pts',(1.591781571759,-99.9874880579221,71.2366455529872));
#41352=CARTESIAN_POINT('Ctrl Pts',(1.74570051630387,-99.9848135889912,71.0117544930956));
#41353=CARTESIAN_POINT('Ctrl Pts',(1.94980991520061,-99.9810415029486,70.5189978221538));
#41354=CARTESIAN_POINT('Ctrl Pts',(2.,-99.9799979995999,70.2511316452692));
#41355=CARTESIAN_POINT('Ctrl Pts',(2.,-99.9799979995999,69.7488683547308));
#41356=CARTESIAN_POINT('Ctrl Pts',(1.94980991520061,-99.9810415029486,69.4810021778462));
#41357=CARTESIAN_POINT('Ctrl Pts',(1.74570051630388,-99.9848135889912,68.9882455069044));
#41358=CARTESIAN_POINT('Ctrl Pts',(1.591781571759,-99.9874880579221,68.7633544470128));
#41359=CARTESIAN_POINT('Ctrl Pts',(1.23664555394557,-99.9925109419644,68.4082184291994));
#41360=CARTESIAN_POINT('Ctrl Pts',(1.01175449350969,-99.995185177515,68.2542994841741));
#41361=CARTESIAN_POINT('Ctrl Pts',(0.518997821386427,-99.998956730068,68.0501900841751));
#41362=CARTESIAN_POINT('Ctrl Pts',(0.251131643913751,-100.,68.));
#41363=CARTESIAN_POINT('Ctrl Pts',(2.77555756156289E-16,-100.,68.));
#41364=CARTESIAN_POINT('',(-4.32646832397843E-16,-90.,72.));
#41365=CARTESIAN_POINT('',(2.44929359829471E-16,-94.,72.));
#41366=CARTESIAN_POINT('',(-2.,-89.9777750336159,70.));
#41367=CARTESIAN_POINT('Ctrl Pts',(-2.,-89.9777750336159,70.));
#41368=CARTESIAN_POINT('Ctrl Pts',(-2.,-89.9777750336159,69.7488666698804));
#41369=CARTESIAN_POINT('Ctrl Pts',(-1.9498092567713,-89.9789345539658,69.480999766208));
#41370=CARTESIAN_POINT('Ctrl Pts',(-1.74569936855887,-89.9831259365723,
68.9882435581214));
#41371=CARTESIAN_POINT('Ctrl Pts',(-1.59178067978086,-89.9860976603374,
68.7633535550347));
#41372=CARTESIAN_POINT('Ctrl Pts',(-1.23664644642618,-89.9916787455059,
68.40821932168));
#41373=CARTESIAN_POINT('Ctrl Pts',(-1.01175644254643,-89.9946501491172,
68.2543006320885));
#41374=CARTESIAN_POINT('Ctrl Pts',(-0.519000232590759,-89.9988407998655,
68.0501907423603));
#41375=CARTESIAN_POINT('Ctrl Pts',(-0.251133328053567,-90.,68.));
#41376=CARTESIAN_POINT('Ctrl Pts',(0.251133328053567,-90.,68.));
#41377=CARTESIAN_POINT('Ctrl Pts',(0.519000232590759,-89.9988407998655,
68.0501907423603));
#41378=CARTESIAN_POINT('Ctrl Pts',(1.01175644254643,-89.9946501491172,68.2543006320885));
#41379=CARTESIAN_POINT('Ctrl Pts',(1.23664644642618,-89.9916787455059,68.40821932168));
#41380=CARTESIAN_POINT('Ctrl Pts',(1.59178067978086,-89.9860976603374,68.7633535550347));
#41381=CARTESIAN_POINT('Ctrl Pts',(1.74569936855887,-89.9831259365723,68.9882435581214));
#41382=CARTESIAN_POINT('Ctrl Pts',(1.94980925677131,-89.9789345539658,69.480999766208));
#41383=CARTESIAN_POINT('Ctrl Pts',(2.,-89.9777750336159,69.7488666698804));
#41384=CARTESIAN_POINT('Ctrl Pts',(2.,-89.9777750336159,70.2511333301196));
#41385=CARTESIAN_POINT('Ctrl Pts',(1.9498092567713,-89.9789345539658,70.519000233792));
#41386=CARTESIAN_POINT('Ctrl Pts',(1.74569936855887,-89.9831259365723,71.0117564418786));
#41387=CARTESIAN_POINT('Ctrl Pts',(1.59178067978086,-89.9860976603374,71.2366464449653));
#41388=CARTESIAN_POINT('Ctrl Pts',(1.23664644642618,-89.9916787455059,71.59178067832));
#41389=CARTESIAN_POINT('Ctrl Pts',(1.01175644254643,-89.9946501491172,71.7456993679115));
#41390=CARTESIAN_POINT('Ctrl Pts',(0.519000232590759,-89.9988407998655,
71.9498092576397));
#41391=CARTESIAN_POINT('Ctrl Pts',(0.251133328053568,-90.,72.));
#41392=CARTESIAN_POINT('Ctrl Pts',(1.31838984174237E-15,-90.,72.));
#41393=CARTESIAN_POINT('Ctrl Pts',(-9.71445146547012E-16,-90.,72.));
#41394=CARTESIAN_POINT('Ctrl Pts',(-0.251133328053568,-90.,72.));
#41395=CARTESIAN_POINT('Ctrl Pts',(-0.519000232590759,-89.9988407998655,
71.9498092576397));
#41396=CARTESIAN_POINT('Ctrl Pts',(-1.01175644254643,-89.9946501491172,
71.7456993679115));
#41397=CARTESIAN_POINT('Ctrl Pts',(-1.23664644642618,-89.9916787455059,
71.59178067832));
#41398=CARTESIAN_POINT('Ctrl Pts',(-1.59178067978086,-89.9860976603374,
71.2366464449653));
#41399=CARTESIAN_POINT('Ctrl Pts',(-1.74569936855887,-89.9831259365723,
71.0117564418786));
#41400=CARTESIAN_POINT('Ctrl Pts',(-1.9498092567713,-89.9789345539658,70.519000233792));
#41401=CARTESIAN_POINT('Ctrl Pts',(-2.,-89.9777750336159,70.2511333301196));
#41402=CARTESIAN_POINT('Ctrl Pts',(-2.,-89.9777750336159,70.));
#41403=CARTESIAN_POINT('Ctrl Pts',(6.93889390390723E-16,-100.,68.));
#41404=CARTESIAN_POINT('Ctrl Pts',(-0.25113164391375,-100.,68.));
#41405=CARTESIAN_POINT('Ctrl Pts',(-0.518997821386426,-99.998956730068,
68.0501900841751));
#41406=CARTESIAN_POINT('Ctrl Pts',(-1.01175449350968,-99.995185177515,68.2542994841741));
#41407=CARTESIAN_POINT('Ctrl Pts',(-1.23664555394557,-99.9925109419644,
68.4082184291994));
#41408=CARTESIAN_POINT('Ctrl Pts',(-1.591781571759,-99.9874880579221,68.7633544470128));
#41409=CARTESIAN_POINT('Ctrl Pts',(-1.74570051630388,-99.9848135889912,
68.9882455069044));
#41410=CARTESIAN_POINT('Ctrl Pts',(-1.94980991520061,-99.9810415029486,
69.4810021778462));
#41411=CARTESIAN_POINT('Ctrl Pts',(-2.,-99.9799979995999,69.7488683547308));
#41412=CARTESIAN_POINT('Ctrl Pts',(-2.,-99.9799979995999,70.));
#41413=CARTESIAN_POINT('Ctrl Pts',(-2.,-99.9799979995999,70.2511316452692));
#41414=CARTESIAN_POINT('Ctrl Pts',(-1.94980991520061,-99.9810415029486,
70.5189978221538));
#41415=CARTESIAN_POINT('Ctrl Pts',(-1.74570051630388,-99.9848135889912,
71.0117544930956));
#41416=CARTESIAN_POINT('Ctrl Pts',(-1.591781571759,-99.9874880579221,71.2366455529872));
#41417=CARTESIAN_POINT('Ctrl Pts',(-1.23664555394557,-99.9925109419644,
71.5917815708006));
#41418=CARTESIAN_POINT('Ctrl Pts',(-1.01175449350968,-99.995185177515,71.7457005158259));
#41419=CARTESIAN_POINT('Ctrl Pts',(-0.51899782138642,-99.998956730068,71.949809915825));
#41420=CARTESIAN_POINT('Ctrl Pts',(-0.251131643913751,-100.,72.));
#41421=CARTESIAN_POINT('Ctrl Pts',(-6.93889390390723E-17,-100.,72.));
#41422=CARTESIAN_POINT('Origin',(0.,94.,70.));
#41423=CARTESIAN_POINT('',(0.,100.,72.));
#41424=CARTESIAN_POINT('',(0.,100.,68.));
#41425=CARTESIAN_POINT('Ctrl Pts',(1.45716771982052E-15,100.,72.));
#41426=CARTESIAN_POINT('Ctrl Pts',(-0.25113164391375,100.,72.));
#41427=CARTESIAN_POINT('Ctrl Pts',(-0.51899782138642,99.998956730068,71.949809915825));
#41428=CARTESIAN_POINT('Ctrl Pts',(-1.01175449350968,99.995185177515,71.7457005158259));
#41429=CARTESIAN_POINT('Ctrl Pts',(-1.23664555394557,99.9925109419644,71.5917815708006));
#41430=CARTESIAN_POINT('Ctrl Pts',(-1.591781571759,99.9874880579221,71.2366455529872));
#41431=CARTESIAN_POINT('Ctrl Pts',(-1.74570051630387,99.9848135889912,71.0117544930956));
#41432=CARTESIAN_POINT('Ctrl Pts',(-1.94980991520061,99.9810415029486,70.5189978221538));
#41433=CARTESIAN_POINT('Ctrl Pts',(-2.,99.9799979995999,70.2511316452692));
#41434=CARTESIAN_POINT('Ctrl Pts',(-2.,99.9799979995999,69.7488683547308));
#41435=CARTESIAN_POINT('Ctrl Pts',(-1.94980991520061,99.9810415029486,69.4810021778462));
#41436=CARTESIAN_POINT('Ctrl Pts',(-1.74570051630388,99.9848135889912,68.9882455069044));
#41437=CARTESIAN_POINT('Ctrl Pts',(-1.591781571759,99.9874880579221,68.7633544470128));
#41438=CARTESIAN_POINT('Ctrl Pts',(-1.23664555394558,99.9925109419644,68.4082184291994));
#41439=CARTESIAN_POINT('Ctrl Pts',(-1.01175449350969,99.995185177515,68.2542994841741));
#41440=CARTESIAN_POINT('Ctrl Pts',(-0.518997821386427,99.998956730068,68.0501900841751));
#41441=CARTESIAN_POINT('Ctrl Pts',(-0.251131643913751,100.,68.));
#41442=CARTESIAN_POINT('Ctrl Pts',(1.38777878078145E-16,100.,68.));
#41443=CARTESIAN_POINT('Ctrl Pts',(-8.32667268468867E-16,100.,68.));
#41444=CARTESIAN_POINT('Ctrl Pts',(0.25113164391375,100.,68.));
#41445=CARTESIAN_POINT('Ctrl Pts',(0.518997821386427,99.998956730068,68.0501900841751));
#41446=CARTESIAN_POINT('Ctrl Pts',(1.01175449350969,99.995185177515,68.2542994841741));
#41447=CARTESIAN_POINT('Ctrl Pts',(1.23664555394558,99.9925109419644,68.4082184291994));
#41448=CARTESIAN_POINT('Ctrl Pts',(1.591781571759,99.9874880579221,68.7633544470128));
#41449=CARTESIAN_POINT('Ctrl Pts',(1.74570051630388,99.9848135889912,68.9882455069044));
#41450=CARTESIAN_POINT('Ctrl Pts',(1.94980991520061,99.9810415029486,69.4810021778462));
#41451=CARTESIAN_POINT('Ctrl Pts',(2.,99.9799979995999,69.7488683547308));
#41452=CARTESIAN_POINT('Ctrl Pts',(2.,99.9799979995999,70.));
#41453=CARTESIAN_POINT('Ctrl Pts',(2.,99.9799979995999,70.2511316452692));
#41454=CARTESIAN_POINT('Ctrl Pts',(1.94980991520061,99.9810415029486,70.5189978221538));
#41455=CARTESIAN_POINT('Ctrl Pts',(1.74570051630388,99.9848135889912,71.0117544930956));
#41456=CARTESIAN_POINT('Ctrl Pts',(1.591781571759,99.9874880579221,71.2366455529872));
#41457=CARTESIAN_POINT('Ctrl Pts',(1.23664555394557,99.9925109419644,71.5917815708006));
#41458=CARTESIAN_POINT('Ctrl Pts',(1.01175449350968,99.995185177515,71.7457005158259));
#41459=CARTESIAN_POINT('Ctrl Pts',(0.51899782138642,99.998956730068,71.949809915825));
#41460=CARTESIAN_POINT('Ctrl Pts',(0.251131643913751,100.,72.));
#41461=CARTESIAN_POINT('Ctrl Pts',(-3.46944695195361E-16,100.,72.));
#41462=CARTESIAN_POINT('',(2.09200853713576E-16,90.,68.));
#41463=CARTESIAN_POINT('',(2.44929359829471E-16,94.,68.));
#41464=CARTESIAN_POINT('',(2.,89.9777750336159,70.));
#41465=CARTESIAN_POINT('Ctrl Pts',(2.,89.9777750336159,70.));
#41466=CARTESIAN_POINT('Ctrl Pts',(2.,89.9777750336159,69.7488666698804));
#41467=CARTESIAN_POINT('Ctrl Pts',(1.9498092567713,89.9789345539658,69.480999766208));
#41468=CARTESIAN_POINT('Ctrl Pts',(1.74569936855887,89.9831259365723,68.9882435581214));
#41469=CARTESIAN_POINT('Ctrl Pts',(1.59178067978086,89.9860976603374,68.7633535550347));
#41470=CARTESIAN_POINT('Ctrl Pts',(1.23664644642618,89.9916787455059,68.40821932168));
#41471=CARTESIAN_POINT('Ctrl Pts',(1.01175644254643,89.9946501491172,68.2543006320885));
#41472=CARTESIAN_POINT('Ctrl Pts',(0.519000232590759,89.9988407998655,68.0501907423603));
#41473=CARTESIAN_POINT('Ctrl Pts',(0.251133328053567,90.,68.));
#41474=CARTESIAN_POINT('Ctrl Pts',(4.85722573273506E-16,90.,68.));
#41475=CARTESIAN_POINT('Ctrl Pts',(1.73472347597681E-16,90.,68.));
#41476=CARTESIAN_POINT('Ctrl Pts',(-0.251133328053567,90.,68.));
#41477=CARTESIAN_POINT('Ctrl Pts',(-0.519000232590759,89.9988407998655,
68.0501907423603));
#41478=CARTESIAN_POINT('Ctrl Pts',(-1.01175644254643,89.9946501491172,68.2543006320885));
#41479=CARTESIAN_POINT('Ctrl Pts',(-1.23664644642618,89.9916787455059,68.40821932168));
#41480=CARTESIAN_POINT('Ctrl Pts',(-1.59178067978086,89.9860976603374,68.7633535550347));
#41481=CARTESIAN_POINT('Ctrl Pts',(-1.74569936855887,89.9831259365723,68.9882435581214));
#41482=CARTESIAN_POINT('Ctrl Pts',(-1.9498092567713,89.9789345539658,69.480999766208));
#41483=CARTESIAN_POINT('Ctrl Pts',(-2.,89.9777750336159,69.7488666698804));
#41484=CARTESIAN_POINT('Ctrl Pts',(-2.,89.9777750336159,70.2511333301196));
#41485=CARTESIAN_POINT('Ctrl Pts',(-1.9498092567713,89.9789345539658,70.519000233792));
#41486=CARTESIAN_POINT('Ctrl Pts',(-1.74569936855887,89.9831259365723,71.0117564418786));
#41487=CARTESIAN_POINT('Ctrl Pts',(-1.59178067978086,89.9860976603374,71.2366464449653));
#41488=CARTESIAN_POINT('Ctrl Pts',(-1.23664644642618,89.9916787455059,71.59178067832));
#41489=CARTESIAN_POINT('Ctrl Pts',(-1.01175644254643,89.9946501491172,71.7456993679115));
#41490=CARTESIAN_POINT('Ctrl Pts',(-0.519000232590759,89.9988407998655,
71.9498092576397));
#41491=CARTESIAN_POINT('Ctrl Pts',(-0.251133328053567,90.,72.));
#41492=CARTESIAN_POINT('Ctrl Pts',(0.251133328053566,90.,72.));
#41493=CARTESIAN_POINT('Ctrl Pts',(0.519000232590759,89.9988407998655,71.9498092576397));
#41494=CARTESIAN_POINT('Ctrl Pts',(1.01175644254643,89.9946501491172,71.7456993679115));
#41495=CARTESIAN_POINT('Ctrl Pts',(1.23664644642618,89.9916787455059,71.59178067832));
#41496=CARTESIAN_POINT('Ctrl Pts',(1.59178067978086,89.9860976603374,71.2366464449653));
#41497=CARTESIAN_POINT('Ctrl Pts',(1.74569936855887,89.9831259365723,71.0117564418786));
#41498=CARTESIAN_POINT('Ctrl Pts',(1.9498092567713,89.9789345539658,70.519000233792));
#41499=CARTESIAN_POINT('Ctrl Pts',(2.,89.9777750336159,70.2511333301196));
#41500=CARTESIAN_POINT('Ctrl Pts',(2.,89.9777750336159,70.));
#41501=CARTESIAN_POINT('Origin',(-94.,0.,70.));
#41502=CARTESIAN_POINT('',(-100.,0.,72.));
#41503=CARTESIAN_POINT('',(-100.,0.,68.));
#41504=CARTESIAN_POINT('Ctrl Pts',(-100.,1.73472347597681E-15,72.));
#41505=CARTESIAN_POINT('Ctrl Pts',(-100.,-0.251131643913749,72.));
#41506=CARTESIAN_POINT('Ctrl Pts',(-99.998956730068,-0.51899782138642,71.949809915825));
#41507=CARTESIAN_POINT('Ctrl Pts',(-99.995185177515,-1.01175449350968,71.7457005158259));
#41508=CARTESIAN_POINT('Ctrl Pts',(-99.9925109419644,-1.23664555394557,
71.5917815708006));
#41509=CARTESIAN_POINT('Ctrl Pts',(-99.9874880579221,-1.591781571759,71.2366455529872));
#41510=CARTESIAN_POINT('Ctrl Pts',(-99.9848135889912,-1.74570051630387,
71.0117544930956));
#41511=CARTESIAN_POINT('Ctrl Pts',(-99.9810415029486,-1.94980991520061,
70.5189978221538));
#41512=CARTESIAN_POINT('Ctrl Pts',(-99.9799979995999,-2.,70.2511316452692));
#41513=CARTESIAN_POINT('Ctrl Pts',(-99.9799979995999,-2.,69.7488683547308));
#41514=CARTESIAN_POINT('Ctrl Pts',(-99.9810415029486,-1.94980991520061,
69.4810021778462));
#41515=CARTESIAN_POINT('Ctrl Pts',(-99.9848135889912,-1.74570051630388,
68.9882455069044));
#41516=CARTESIAN_POINT('Ctrl Pts',(-99.9874880579221,-1.591781571759,68.7633544470128));
#41517=CARTESIAN_POINT('Ctrl Pts',(-99.9925109419644,-1.23664555394558,
68.4082184291994));
#41518=CARTESIAN_POINT('Ctrl Pts',(-99.995185177515,-1.01175449350969,68.2542994841741));
#41519=CARTESIAN_POINT('Ctrl Pts',(-99.998956730068,-0.518997821386428,
68.0501900841751));
#41520=CARTESIAN_POINT('Ctrl Pts',(-100.,-0.251131643913751,68.));
#41521=CARTESIAN_POINT('Ctrl Pts',(-100.,-4.85722573273506E-16,68.));
#41522=CARTESIAN_POINT('',(-99.9799979995999,2.,70.));
#41523=CARTESIAN_POINT('Ctrl Pts',(-99.9799979995999,2.,70.));
#41524=CARTESIAN_POINT('Ctrl Pts',(-99.9799979995999,2.,70.2511316452692));
#41525=CARTESIAN_POINT('Ctrl Pts',(-99.9810415029486,1.94980991520061,70.5189978221538));
#41526=CARTESIAN_POINT('Ctrl Pts',(-99.9848135889912,1.74570051630388,71.0117544930956));
#41527=CARTESIAN_POINT('Ctrl Pts',(-99.9874880579221,1.591781571759,71.2366455529872));
#41528=CARTESIAN_POINT('Ctrl Pts',(-99.9925109419644,1.23664555394557,71.5917815708006));
#41529=CARTESIAN_POINT('Ctrl Pts',(-99.995185177515,1.01175449350968,71.7457005158259));
#41530=CARTESIAN_POINT('Ctrl Pts',(-99.998956730068,0.51899782138642,71.949809915825));
#41531=CARTESIAN_POINT('Ctrl Pts',(-100.,0.251131643913751,72.));
#41532=CARTESIAN_POINT('Ctrl Pts',(-100.,-6.93889390390723E-17,72.));
#41533=CARTESIAN_POINT('',(-89.9777750336159,2.,70.));
#41534=CARTESIAN_POINT('',(-94.,2.,70.));
#41535=CARTESIAN_POINT('',(-90.,-4.92110461433098E-15,72.));
#41536=CARTESIAN_POINT('Ctrl Pts',(-90.,1.11022302462516E-15,72.));
#41537=CARTESIAN_POINT('Ctrl Pts',(-90.,0.251133328053568,72.));
#41538=CARTESIAN_POINT('Ctrl Pts',(-89.9988407998655,0.519000232590759,
71.9498092576397));
#41539=CARTESIAN_POINT('Ctrl Pts',(-89.9946501491172,1.01175644254643,71.7456993679115));
#41540=CARTESIAN_POINT('Ctrl Pts',(-89.9916787455059,1.23664644642618,71.59178067832));
#41541=CARTESIAN_POINT('Ctrl Pts',(-89.9860976603374,1.59178067978086,71.2366464449653));
#41542=CARTESIAN_POINT('Ctrl Pts',(-89.9831259365723,1.74569936855887,71.0117564418786));
#41543=CARTESIAN_POINT('Ctrl Pts',(-89.9789345539658,1.9498092567713,70.519000233792));
#41544=CARTESIAN_POINT('Ctrl Pts',(-89.9777750336159,2.,70.2511333301196));
#41545=CARTESIAN_POINT('Ctrl Pts',(-89.9777750336159,2.,70.));
#41546=CARTESIAN_POINT('',(-90.,-5.40682718760448E-15,68.));
#41547=CARTESIAN_POINT('Ctrl Pts',(-90.,2.08166817117217E-16,68.));
#41548=CARTESIAN_POINT('Ctrl Pts',(-90.,-0.251133328053567,68.));
#41549=CARTESIAN_POINT('Ctrl Pts',(-89.9988407998655,-0.519000232590759,
68.0501907423603));
#41550=CARTESIAN_POINT('Ctrl Pts',(-89.9946501491172,-1.01175644254643,
68.2543006320885));
#41551=CARTESIAN_POINT('Ctrl Pts',(-89.9916787455059,-1.23664644642618,
68.40821932168));
#41552=CARTESIAN_POINT('Ctrl Pts',(-89.9860976603374,-1.59178067978086,
68.7633535550347));
#41553=CARTESIAN_POINT('Ctrl Pts',(-89.9831259365723,-1.74569936855887,
68.9882435581214));
#41554=CARTESIAN_POINT('Ctrl Pts',(-89.9789345539658,-1.94980925677131,
69.480999766208));
#41555=CARTESIAN_POINT('Ctrl Pts',(-89.9777750336159,-2.,69.7488666698804));
#41556=CARTESIAN_POINT('Ctrl Pts',(-89.9777750336159,-2.,70.2511333301196));
#41557=CARTESIAN_POINT('Ctrl Pts',(-89.9789345539658,-1.9498092567713,70.519000233792));
#41558=CARTESIAN_POINT('Ctrl Pts',(-89.9831259365723,-1.74569936855886,
71.0117564418786));
#41559=CARTESIAN_POINT('Ctrl Pts',(-89.9860976603374,-1.59178067978086,
71.2366464449653));
#41560=CARTESIAN_POINT('Ctrl Pts',(-89.9916787455059,-1.23664644642618,
71.59178067832));
#41561=CARTESIAN_POINT('Ctrl Pts',(-89.9946501491172,-1.01175644254642,
71.7456993679115));
#41562=CARTESIAN_POINT('Ctrl Pts',(-89.9988407998655,-0.519000232590759,
71.9498092576397));
#41563=CARTESIAN_POINT('Ctrl Pts',(-90.,-0.251133328053567,72.));
#41564=CARTESIAN_POINT('Ctrl Pts',(-90.,-6.93889390390723E-17,72.));
#41565=CARTESIAN_POINT('Ctrl Pts',(-89.9777750336159,2.,70.));
#41566=CARTESIAN_POINT('Ctrl Pts',(-89.9777750336159,2.,69.7488666698804));
#41567=CARTESIAN_POINT('Ctrl Pts',(-89.9789345539658,1.9498092567713,69.480999766208));
#41568=CARTESIAN_POINT('Ctrl Pts',(-89.9831259365723,1.74569936855887,68.9882435581214));
#41569=CARTESIAN_POINT('Ctrl Pts',(-89.9860976603374,1.59178067978086,68.7633535550347));
#41570=CARTESIAN_POINT('Ctrl Pts',(-89.9916787455059,1.23664644642618,68.40821932168));
#41571=CARTESIAN_POINT('Ctrl Pts',(-89.9946501491172,1.01175644254643,68.2543006320885));
#41572=CARTESIAN_POINT('Ctrl Pts',(-89.9988407998655,0.519000232590759,
68.0501907423603));
#41573=CARTESIAN_POINT('Ctrl Pts',(-90.,0.251133328053566,68.));
#41574=CARTESIAN_POINT('Ctrl Pts',(-90.,-5.55111512312578E-16,68.));
#41575=CARTESIAN_POINT('Ctrl Pts',(-100.,-4.16333634234434E-16,68.));
#41576=CARTESIAN_POINT('Ctrl Pts',(-100.,0.25113164391375,68.));
#41577=CARTESIAN_POINT('Ctrl Pts',(-99.998956730068,0.518997821386425,68.0501900841751));
#41578=CARTESIAN_POINT('Ctrl Pts',(-99.995185177515,1.01175449350968,68.2542994841741));
#41579=CARTESIAN_POINT('Ctrl Pts',(-99.9925109419644,1.23664555394557,68.4082184291994));
#41580=CARTESIAN_POINT('Ctrl Pts',(-99.9874880579221,1.591781571759,68.7633544470128));
#41581=CARTESIAN_POINT('Ctrl Pts',(-99.9848135889912,1.74570051630388,68.9882455069044));
#41582=CARTESIAN_POINT('Ctrl Pts',(-99.9810415029486,1.94980991520061,69.4810021778462));
#41583=CARTESIAN_POINT('Ctrl Pts',(-99.9799979995999,2.,69.7488683547308));
#41584=CARTESIAN_POINT('Ctrl Pts',(-99.9799979995999,2.,70.));
#41585=CARTESIAN_POINT('Origin',(94.,0.,70.));
#41586=CARTESIAN_POINT('',(100.,0.,72.));
#41587=CARTESIAN_POINT('',(100.,0.,68.));
#41588=CARTESIAN_POINT('Ctrl Pts',(100.,-1.73472347597681E-15,72.));
#41589=CARTESIAN_POINT('Ctrl Pts',(100.,0.251131643913749,72.));
#41590=CARTESIAN_POINT('Ctrl Pts',(99.998956730068,0.51899782138642,71.949809915825));
#41591=CARTESIAN_POINT('Ctrl Pts',(99.995185177515,1.01175449350968,71.7457005158259));
#41592=CARTESIAN_POINT('Ctrl Pts',(99.9925109419644,1.23664555394557,71.5917815708006));
#41593=CARTESIAN_POINT('Ctrl Pts',(99.9874880579221,1.591781571759,71.2366455529872));
#41594=CARTESIAN_POINT('Ctrl Pts',(99.9848135889912,1.74570051630387,71.0117544930956));
#41595=CARTESIAN_POINT('Ctrl Pts',(99.9810415029486,1.94980991520061,70.5189978221538));
#41596=CARTESIAN_POINT('Ctrl Pts',(99.9799979995999,2.,70.2511316452692));
#41597=CARTESIAN_POINT('Ctrl Pts',(99.9799979995999,2.,69.7488683547308));
#41598=CARTESIAN_POINT('Ctrl Pts',(99.9810415029486,1.94980991520061,69.4810021778462));
#41599=CARTESIAN_POINT('Ctrl Pts',(99.9848135889912,1.74570051630388,68.9882455069044));
#41600=CARTESIAN_POINT('Ctrl Pts',(99.9874880579221,1.591781571759,68.7633544470128));
#41601=CARTESIAN_POINT('Ctrl Pts',(99.9925109419644,1.23664555394558,68.4082184291994));
#41602=CARTESIAN_POINT('Ctrl Pts',(99.995185177515,1.01175449350969,68.2542994841741));
#41603=CARTESIAN_POINT('Ctrl Pts',(99.998956730068,0.518997821386428,68.0501900841751));
#41604=CARTESIAN_POINT('Ctrl Pts',(100.,0.251131643913751,68.));
#41605=CARTESIAN_POINT('Ctrl Pts',(100.,4.85722573273506E-16,68.));
#41606=CARTESIAN_POINT('',(99.9799979995999,-2.,70.));
#41607=CARTESIAN_POINT('Ctrl Pts',(99.9799979995999,-2.,70.));
#41608=CARTESIAN_POINT('Ctrl Pts',(99.9799979995999,-2.,70.2511316452692));
#41609=CARTESIAN_POINT('Ctrl Pts',(99.9810415029486,-1.94980991520061,70.5189978221538));
#41610=CARTESIAN_POINT('Ctrl Pts',(99.9848135889912,-1.74570051630388,71.0117544930956));
#41611=CARTESIAN_POINT('Ctrl Pts',(99.9874880579221,-1.591781571759,71.2366455529872));
#41612=CARTESIAN_POINT('Ctrl Pts',(99.9925109419644,-1.23664555394557,71.5917815708006));
#41613=CARTESIAN_POINT('Ctrl Pts',(99.995185177515,-1.01175449350968,71.7457005158259));
#41614=CARTESIAN_POINT('Ctrl Pts',(99.998956730068,-0.51899782138642,71.949809915825));
#41615=CARTESIAN_POINT('Ctrl Pts',(100.,-0.251131643913751,72.));
#41616=CARTESIAN_POINT('Ctrl Pts',(100.,6.93889390390723E-17,72.));
#41617=CARTESIAN_POINT('',(89.9777750336159,-2.,70.));
#41618=CARTESIAN_POINT('',(94.,-2.,70.));
#41619=CARTESIAN_POINT('Ctrl Pts',(89.9777750336159,-2.,70.));
#41620=CARTESIAN_POINT('Ctrl Pts',(89.9777750336159,-2.,69.7488666698804));
#41621=CARTESIAN_POINT('Ctrl Pts',(89.9789345539658,-1.9498092567713,69.480999766208));
#41622=CARTESIAN_POINT('Ctrl Pts',(89.9831259365723,-1.74569936855887,68.9882435581214));
#41623=CARTESIAN_POINT('Ctrl Pts',(89.9860976603374,-1.59178067978086,68.7633535550347));
#41624=CARTESIAN_POINT('Ctrl Pts',(89.9916787455059,-1.23664644642618,68.40821932168));
#41625=CARTESIAN_POINT('Ctrl Pts',(89.9946501491172,-1.01175644254643,68.2543006320885));
#41626=CARTESIAN_POINT('Ctrl Pts',(89.9988407998655,-0.519000232590759,
68.0501907423603));
#41627=CARTESIAN_POINT('Ctrl Pts',(90.,-0.251133328053567,68.));
#41628=CARTESIAN_POINT('Ctrl Pts',(90.,0.251133328053567,68.));
#41629=CARTESIAN_POINT('Ctrl Pts',(89.9988407998655,0.519000232590759,68.0501907423603));
#41630=CARTESIAN_POINT('Ctrl Pts',(89.9946501491172,1.01175644254643,68.2543006320885));
#41631=CARTESIAN_POINT('Ctrl Pts',(89.9916787455059,1.23664644642618,68.40821932168));
#41632=CARTESIAN_POINT('Ctrl Pts',(89.9860976603374,1.59178067978086,68.7633535550347));
#41633=CARTESIAN_POINT('Ctrl Pts',(89.9831259365723,1.74569936855887,68.9882435581214));
#41634=CARTESIAN_POINT('Ctrl Pts',(89.9789345539658,1.94980925677131,69.480999766208));
#41635=CARTESIAN_POINT('Ctrl Pts',(89.9777750336159,2.,69.7488666698804));
#41636=CARTESIAN_POINT('Ctrl Pts',(89.9777750336159,2.,70.2511333301196));
#41637=CARTESIAN_POINT('Ctrl Pts',(89.9789345539658,1.9498092567713,70.519000233792));
#41638=CARTESIAN_POINT('Ctrl Pts',(89.9831259365723,1.74569936855886,71.0117564418786));
#41639=CARTESIAN_POINT('Ctrl Pts',(89.9860976603374,1.59178067978086,71.2366464449653));
#41640=CARTESIAN_POINT('Ctrl Pts',(89.9916787455059,1.23664644642618,71.59178067832));
#41641=CARTESIAN_POINT('Ctrl Pts',(89.9946501491172,1.01175644254642,71.7456993679115));
#41642=CARTESIAN_POINT('Ctrl Pts',(89.9988407998655,0.519000232590759,71.9498092576397));
#41643=CARTESIAN_POINT('Ctrl Pts',(90.,0.251133328053567,72.));
#41644=CARTESIAN_POINT('Ctrl Pts',(90.,-0.251133328053567,72.));
#41645=CARTESIAN_POINT('Ctrl Pts',(89.9988407998655,-0.519000232590759,
71.9498092576397));
#41646=CARTESIAN_POINT('Ctrl Pts',(89.9946501491172,-1.01175644254643,71.7456993679115));
#41647=CARTESIAN_POINT('Ctrl Pts',(89.9916787455059,-1.23664644642618,71.59178067832));
#41648=CARTESIAN_POINT('Ctrl Pts',(89.9860976603374,-1.59178067978086,71.2366464449653));
#41649=CARTESIAN_POINT('Ctrl Pts',(89.9831259365723,-1.74569936855887,71.0117564418786));
#41650=CARTESIAN_POINT('Ctrl Pts',(89.9789345539658,-1.9498092567713,70.519000233792));
#41651=CARTESIAN_POINT('Ctrl Pts',(89.9777750336159,-2.,70.2511333301196));
#41652=CARTESIAN_POINT('Ctrl Pts',(89.9777750336159,-2.,70.));
#41653=CARTESIAN_POINT('Ctrl Pts',(100.,4.16333634234434E-16,68.));
#41654=CARTESIAN_POINT('Ctrl Pts',(100.,-0.25113164391375,68.));
#41655=CARTESIAN_POINT('Ctrl Pts',(99.998956730068,-0.518997821386425,68.0501900841751));
#41656=CARTESIAN_POINT('Ctrl Pts',(99.995185177515,-1.01175449350968,68.2542994841741));
#41657=CARTESIAN_POINT('Ctrl Pts',(99.9925109419644,-1.23664555394557,68.4082184291994));
#41658=CARTESIAN_POINT('Ctrl Pts',(99.9874880579221,-1.591781571759,68.7633544470128));
#41659=CARTESIAN_POINT('Ctrl Pts',(99.9848135889912,-1.74570051630388,68.9882455069044));
#41660=CARTESIAN_POINT('Ctrl Pts',(99.9810415029486,-1.94980991520061,69.4810021778462));
#41661=CARTESIAN_POINT('Ctrl Pts',(99.9799979995999,-2.,69.7488683547308));
#41662=CARTESIAN_POINT('Ctrl Pts',(99.9799979995999,-2.,70.));
#41663=CARTESIAN_POINT('Origin',(0.,-94.,36.));
#41664=CARTESIAN_POINT('',(0.,-100.,38.));
#41665=CARTESIAN_POINT('',(0.,-100.,34.));
#41666=CARTESIAN_POINT('Ctrl Pts',(-6.24500451351651E-16,-100.,38.));
#41667=CARTESIAN_POINT('Ctrl Pts',(0.251131643913749,-100.,38.));
#41668=CARTESIAN_POINT('Ctrl Pts',(0.518997821386425,-99.998956730068,37.9498099158249));
#41669=CARTESIAN_POINT('Ctrl Pts',(1.01175449350969,-99.995185177515,37.7457005158259));
#41670=CARTESIAN_POINT('Ctrl Pts',(1.23664555394557,-99.9925109419644,37.5917815708006));
#41671=CARTESIAN_POINT('Ctrl Pts',(1.591781571759,-99.9874880579221,37.2366455529872));
#41672=CARTESIAN_POINT('Ctrl Pts',(1.74570051630387,-99.9848135889912,37.0117544930956));
#41673=CARTESIAN_POINT('Ctrl Pts',(1.94980991520061,-99.9810415029486,36.5189978221538));
#41674=CARTESIAN_POINT('Ctrl Pts',(2.,-99.9799979995999,36.2511316452692));
#41675=CARTESIAN_POINT('Ctrl Pts',(2.,-99.9799979995999,35.7488683547308));
#41676=CARTESIAN_POINT('Ctrl Pts',(1.94980991520061,-99.9810415029486,35.4810021778462));
#41677=CARTESIAN_POINT('Ctrl Pts',(1.74570051630388,-99.9848135889912,34.9882455069044));
#41678=CARTESIAN_POINT('Ctrl Pts',(1.591781571759,-99.9874880579221,34.7633544470128));
#41679=CARTESIAN_POINT('Ctrl Pts',(1.23664555394558,-99.9925109419644,34.4082184291994));
#41680=CARTESIAN_POINT('Ctrl Pts',(1.01175449350969,-99.995185177515,34.2542994841741));
#41681=CARTESIAN_POINT('Ctrl Pts',(0.518997821386428,-99.998956730068,34.050190084175));
#41682=CARTESIAN_POINT('Ctrl Pts',(0.251131643913751,-100.,34.));
#41683=CARTESIAN_POINT('Ctrl Pts',(1.38777878078145E-16,-100.,34.));
#41684=CARTESIAN_POINT('',(2.95937027512416E-16,-90.,38.));
#41685=CARTESIAN_POINT('',(2.44929359829471E-16,-94.,38.));
#41686=CARTESIAN_POINT('',(-2.,-89.9777750336159,36.));
#41687=CARTESIAN_POINT('Ctrl Pts',(-2.,-89.9777750336159,36.));
#41688=CARTESIAN_POINT('Ctrl Pts',(-2.,-89.9777750336159,35.7488666698804));
#41689=CARTESIAN_POINT('Ctrl Pts',(-1.94980925677131,-89.9789345539658,
35.480999766208));
#41690=CARTESIAN_POINT('Ctrl Pts',(-1.74569936855887,-89.9831259365723,
34.9882435581214));
#41691=CARTESIAN_POINT('Ctrl Pts',(-1.59178067978086,-89.9860976603374,
34.7633535550347));
#41692=CARTESIAN_POINT('Ctrl Pts',(-1.23664644642618,-89.9916787455059,
34.40821932168));
#41693=CARTESIAN_POINT('Ctrl Pts',(-1.01175644254643,-89.9946501491172,
34.2543006320885));
#41694=CARTESIAN_POINT('Ctrl Pts',(-0.519000232590761,-89.9988407998655,
34.0501907423603));
#41695=CARTESIAN_POINT('Ctrl Pts',(-0.251133328053567,-90.,34.));
#41696=CARTESIAN_POINT('Ctrl Pts',(0.251133328053567,-90.,34.));
#41697=CARTESIAN_POINT('Ctrl Pts',(0.519000232590761,-89.9988407998655,
34.0501907423603));
#41698=CARTESIAN_POINT('Ctrl Pts',(1.01175644254643,-89.9946501491172,34.2543006320885));
#41699=CARTESIAN_POINT('Ctrl Pts',(1.23664644642618,-89.9916787455059,34.40821932168));
#41700=CARTESIAN_POINT('Ctrl Pts',(1.59178067978086,-89.9860976603374,34.7633535550347));
#41701=CARTESIAN_POINT('Ctrl Pts',(1.74569936855887,-89.9831259365723,34.9882435581214));
#41702=CARTESIAN_POINT('Ctrl Pts',(1.94980925677131,-89.9789345539658,35.480999766208));
#41703=CARTESIAN_POINT('Ctrl Pts',(2.,-89.9777750336159,35.7488666698804));
#41704=CARTESIAN_POINT('Ctrl Pts',(2.,-89.9777750336159,36.2511333301197));
#41705=CARTESIAN_POINT('Ctrl Pts',(1.9498092567713,-89.9789345539658,36.519000233792));
#41706=CARTESIAN_POINT('Ctrl Pts',(1.74569936855886,-89.9831259365723,37.0117564418786));
#41707=CARTESIAN_POINT('Ctrl Pts',(1.59178067978086,-89.9860976603374,37.2366464449653));
#41708=CARTESIAN_POINT('Ctrl Pts',(1.23664644642618,-89.9916787455059,37.59178067832));
#41709=CARTESIAN_POINT('Ctrl Pts',(1.01175644254643,-89.9946501491172,37.7456993679115));
#41710=CARTESIAN_POINT('Ctrl Pts',(0.51900023259076,-89.9988407998655,37.9498092576397));
#41711=CARTESIAN_POINT('Ctrl Pts',(0.251133328053566,-90.,38.));
#41712=CARTESIAN_POINT('Ctrl Pts',(6.93889390390723E-17,-90.,38.));
#41713=CARTESIAN_POINT('Ctrl Pts',(0.,-90.,38.));
#41714=CARTESIAN_POINT('Ctrl Pts',(-0.251133328053566,-90.,38.));
#41715=CARTESIAN_POINT('Ctrl Pts',(-0.51900023259076,-89.9988407998655,
37.9498092576397));
#41716=CARTESIAN_POINT('Ctrl Pts',(-1.01175644254643,-89.9946501491172,
37.7456993679115));
#41717=CARTESIAN_POINT('Ctrl Pts',(-1.23664644642618,-89.9916787455059,
37.59178067832));
#41718=CARTESIAN_POINT('Ctrl Pts',(-1.59178067978086,-89.9860976603374,
37.2366464449653));
#41719=CARTESIAN_POINT('Ctrl Pts',(-1.74569936855887,-89.9831259365723,
37.0117564418786));
#41720=CARTESIAN_POINT('Ctrl Pts',(-1.94980925677131,-89.9789345539658,
36.519000233792));
#41721=CARTESIAN_POINT('Ctrl Pts',(-2.,-89.9777750336159,36.2511333301197));
#41722=CARTESIAN_POINT('Ctrl Pts',(-2.,-89.9777750336159,36.));
#41723=CARTESIAN_POINT('Ctrl Pts',(-1.38777878078145E-16,-100.,34.));
#41724=CARTESIAN_POINT('Ctrl Pts',(-0.251131643913752,-100.,34.));
#41725=CARTESIAN_POINT('Ctrl Pts',(-0.518997821386424,-99.998956730068,
34.050190084175));
#41726=CARTESIAN_POINT('Ctrl Pts',(-1.01175449350969,-99.995185177515,34.2542994841741));
#41727=CARTESIAN_POINT('Ctrl Pts',(-1.23664555394558,-99.9925109419644,
34.4082184291994));
#41728=CARTESIAN_POINT('Ctrl Pts',(-1.591781571759,-99.9874880579221,34.7633544470128));
#41729=CARTESIAN_POINT('Ctrl Pts',(-1.74570051630388,-99.9848135889912,
34.9882455069044));
#41730=CARTESIAN_POINT('Ctrl Pts',(-1.94980991520062,-99.9810415029486,
35.4810021778462));
#41731=CARTESIAN_POINT('Ctrl Pts',(-2.,-99.9799979995999,35.7488683547308));
#41732=CARTESIAN_POINT('Ctrl Pts',(-2.,-99.9799979995999,36.));
#41733=CARTESIAN_POINT('Ctrl Pts',(-2.,-99.9799979995999,36.2511316452692));
#41734=CARTESIAN_POINT('Ctrl Pts',(-1.94980991520061,-99.9810415029486,
36.5189978221538));
#41735=CARTESIAN_POINT('Ctrl Pts',(-1.74570051630387,-99.9848135889912,
37.0117544930956));
#41736=CARTESIAN_POINT('Ctrl Pts',(-1.591781571759,-99.9874880579221,37.2366455529872));
#41737=CARTESIAN_POINT('Ctrl Pts',(-1.23664555394557,-99.9925109419644,
37.5917815708006));
#41738=CARTESIAN_POINT('Ctrl Pts',(-1.01175449350969,-99.995185177515,37.7457005158259));
#41739=CARTESIAN_POINT('Ctrl Pts',(-0.518997821386425,-99.998956730068,
37.9498099158249));
#41740=CARTESIAN_POINT('Ctrl Pts',(-0.25113164391375,-100.,38.));
#41741=CARTESIAN_POINT('Ctrl Pts',(-4.16333634234434E-16,-100.,38.));
#41742=CARTESIAN_POINT('Origin',(0.,94.,36.));
#41743=CARTESIAN_POINT('',(0.,100.,38.));
#41744=CARTESIAN_POINT('',(0.,100.,34.));
#41745=CARTESIAN_POINT('Ctrl Pts',(5.55111512312578E-16,100.,38.));
#41746=CARTESIAN_POINT('Ctrl Pts',(-0.251131643913749,100.,38.));
#41747=CARTESIAN_POINT('Ctrl Pts',(-0.518997821386421,99.998956730068,37.9498099158249));
#41748=CARTESIAN_POINT('Ctrl Pts',(-1.01175449350968,99.995185177515,37.7457005158259));
#41749=CARTESIAN_POINT('Ctrl Pts',(-1.23664555394557,99.9925109419644,37.5917815708006));
#41750=CARTESIAN_POINT('Ctrl Pts',(-1.591781571759,99.9874880579221,37.2366455529872));
#41751=CARTESIAN_POINT('Ctrl Pts',(-1.74570051630387,99.9848135889912,37.0117544930956));
#41752=CARTESIAN_POINT('Ctrl Pts',(-1.94980991520061,99.9810415029486,36.5189978221538));
#41753=CARTESIAN_POINT('Ctrl Pts',(-2.,99.9799979995999,36.2511316452692));
#41754=CARTESIAN_POINT('Ctrl Pts',(-2.,99.9799979995999,35.7488683547308));
#41755=CARTESIAN_POINT('Ctrl Pts',(-1.94980991520062,99.9810415029486,35.4810021778462));
#41756=CARTESIAN_POINT('Ctrl Pts',(-1.74570051630388,99.9848135889912,34.9882455069044));
#41757=CARTESIAN_POINT('Ctrl Pts',(-1.591781571759,99.9874880579221,34.7633544470128));
#41758=CARTESIAN_POINT('Ctrl Pts',(-1.23664555394558,99.9925109419644,34.4082184291994));
#41759=CARTESIAN_POINT('Ctrl Pts',(-1.01175449350969,99.995185177515,34.2542994841741));
#41760=CARTESIAN_POINT('Ctrl Pts',(-0.518997821386425,99.998956730068,34.050190084175));
#41761=CARTESIAN_POINT('Ctrl Pts',(-0.251131643913753,100.,34.));
#41762=CARTESIAN_POINT('Ctrl Pts',(-9.71445146547012E-16,100.,34.));
#41763=CARTESIAN_POINT('Ctrl Pts',(2.77555756156289E-16,100.,34.));
#41764=CARTESIAN_POINT('Ctrl Pts',(0.251131643913752,100.,34.));
#41765=CARTESIAN_POINT('Ctrl Pts',(0.518997821386428,99.998956730068,34.050190084175));
#41766=CARTESIAN_POINT('Ctrl Pts',(1.01175449350969,99.995185177515,34.2542994841741));
#41767=CARTESIAN_POINT('Ctrl Pts',(1.23664555394558,99.9925109419644,34.4082184291994));
#41768=CARTESIAN_POINT('Ctrl Pts',(1.591781571759,99.9874880579221,34.7633544470128));
#41769=CARTESIAN_POINT('Ctrl Pts',(1.74570051630388,99.9848135889912,34.9882455069044));
#41770=CARTESIAN_POINT('Ctrl Pts',(1.94980991520061,99.9810415029486,35.4810021778462));
#41771=CARTESIAN_POINT('Ctrl Pts',(2.,99.9799979995999,35.7488683547308));
#41772=CARTESIAN_POINT('Ctrl Pts',(2.,99.9799979995999,36.));
#41773=CARTESIAN_POINT('Ctrl Pts',(2.,99.9799979995999,36.2511316452692));
#41774=CARTESIAN_POINT('Ctrl Pts',(1.94980991520061,99.9810415029486,36.5189978221538));
#41775=CARTESIAN_POINT('Ctrl Pts',(1.74570051630387,99.9848135889912,37.0117544930956));
#41776=CARTESIAN_POINT('Ctrl Pts',(1.591781571759,99.9874880579221,37.2366455529872));
#41777=CARTESIAN_POINT('Ctrl Pts',(1.23664555394557,99.9925109419644,37.5917815708006));
#41778=CARTESIAN_POINT('Ctrl Pts',(1.01175449350968,99.995185177515,37.7457005158259));
#41779=CARTESIAN_POINT('Ctrl Pts',(0.518997821386424,99.998956730068,37.949809915825));
#41780=CARTESIAN_POINT('Ctrl Pts',(0.25113164391375,100.,38.));
#41781=CARTESIAN_POINT('Ctrl Pts',(1.38777878078145E-16,100.,38.));
#41782=CARTESIAN_POINT('',(4.00020436071024E-16,90.,34.));
#41783=CARTESIAN_POINT('',(2.44929359829471E-16,94.,34.));
#41784=CARTESIAN_POINT('',(2.,89.9777750336159,36.));
#41785=CARTESIAN_POINT('Ctrl Pts',(2.,89.9777750336159,36.));
#41786=CARTESIAN_POINT('Ctrl Pts',(2.,89.9777750336159,35.7488666698804));
#41787=CARTESIAN_POINT('Ctrl Pts',(1.94980925677131,89.9789345539658,35.480999766208));
#41788=CARTESIAN_POINT('Ctrl Pts',(1.74569936855887,89.9831259365723,34.9882435581214));
#41789=CARTESIAN_POINT('Ctrl Pts',(1.59178067978086,89.9860976603374,34.7633535550347));
#41790=CARTESIAN_POINT('Ctrl Pts',(1.23664644642618,89.9916787455059,34.40821932168));
#41791=CARTESIAN_POINT('Ctrl Pts',(1.01175644254643,89.9946501491172,34.2543006320885));
#41792=CARTESIAN_POINT('Ctrl Pts',(0.519000232590761,89.9988407998655,34.0501907423603));
#41793=CARTESIAN_POINT('Ctrl Pts',(0.251133328053567,90.,34.));
#41794=CARTESIAN_POINT('Ctrl Pts',(0.,90.,34.));
#41795=CARTESIAN_POINT('Ctrl Pts',(5.55111512312578E-16,90.,34.));
#41796=CARTESIAN_POINT('Ctrl Pts',(-0.251133328053567,90.,34.));
#41797=CARTESIAN_POINT('Ctrl Pts',(-0.519000232590761,89.9988407998655,
34.0501907423603));
#41798=CARTESIAN_POINT('Ctrl Pts',(-1.01175644254643,89.9946501491172,34.2543006320885));
#41799=CARTESIAN_POINT('Ctrl Pts',(-1.23664644642618,89.9916787455059,34.40821932168));
#41800=CARTESIAN_POINT('Ctrl Pts',(-1.59178067978086,89.9860976603374,34.7633535550347));
#41801=CARTESIAN_POINT('Ctrl Pts',(-1.74569936855887,89.9831259365723,34.9882435581214));
#41802=CARTESIAN_POINT('Ctrl Pts',(-1.94980925677131,89.9789345539658,35.480999766208));
#41803=CARTESIAN_POINT('Ctrl Pts',(-2.,89.9777750336159,35.7488666698804));
#41804=CARTESIAN_POINT('Ctrl Pts',(-2.,89.9777750336159,36.2511333301197));
#41805=CARTESIAN_POINT('Ctrl Pts',(-1.9498092567713,89.9789345539658,36.519000233792));
#41806=CARTESIAN_POINT('Ctrl Pts',(-1.74569936855886,89.9831259365723,37.0117564418786));
#41807=CARTESIAN_POINT('Ctrl Pts',(-1.59178067978086,89.9860976603374,37.2366464449653));
#41808=CARTESIAN_POINT('Ctrl Pts',(-1.23664644642618,89.9916787455059,37.59178067832));
#41809=CARTESIAN_POINT('Ctrl Pts',(-1.01175644254643,89.9946501491172,37.7456993679115));
#41810=CARTESIAN_POINT('Ctrl Pts',(-0.519000232590762,89.9988407998655,
37.9498092576397));
#41811=CARTESIAN_POINT('Ctrl Pts',(-0.251133328053566,90.,38.));
#41812=CARTESIAN_POINT('Ctrl Pts',(0.251133328053565,90.,38.));
#41813=CARTESIAN_POINT('Ctrl Pts',(0.519000232590761,89.9988407998655,37.9498092576397));
#41814=CARTESIAN_POINT('Ctrl Pts',(1.01175644254643,89.9946501491172,37.7456993679115));
#41815=CARTESIAN_POINT('Ctrl Pts',(1.23664644642618,89.9916787455059,37.59178067832));
#41816=CARTESIAN_POINT('Ctrl Pts',(1.59178067978086,89.9860976603374,37.2366464449653));
#41817=CARTESIAN_POINT('Ctrl Pts',(1.74569936855886,89.9831259365723,37.0117564418786));
#41818=CARTESIAN_POINT('Ctrl Pts',(1.9498092567713,89.9789345539658,36.519000233792));
#41819=CARTESIAN_POINT('Ctrl Pts',(2.,89.9777750336159,36.2511333301197));
#41820=CARTESIAN_POINT('Ctrl Pts',(2.,89.9777750336159,36.));
#41821=CARTESIAN_POINT('Origin',(-94.,0.,36.));
#41822=CARTESIAN_POINT('',(-100.,0.,38.));
#41823=CARTESIAN_POINT('',(-100.,0.,34.));
#41824=CARTESIAN_POINT('Ctrl Pts',(-100.,-5.55111512312578E-16,38.));
#41825=CARTESIAN_POINT('Ctrl Pts',(-100.,-0.251131643913751,38.));
#41826=CARTESIAN_POINT('Ctrl Pts',(-99.998956730068,-0.518997821386424,
37.949809915825));
#41827=CARTESIAN_POINT('Ctrl Pts',(-99.995185177515,-1.01175449350968,37.7457005158259));
#41828=CARTESIAN_POINT('Ctrl Pts',(-99.9925109419644,-1.23664555394557,
37.5917815708006));
#41829=CARTESIAN_POINT('Ctrl Pts',(-99.9874880579221,-1.591781571759,37.2366455529872));
#41830=CARTESIAN_POINT('Ctrl Pts',(-99.9848135889912,-1.74570051630387,
37.0117544930956));
#41831=CARTESIAN_POINT('Ctrl Pts',(-99.9810415029486,-1.94980991520061,
36.5189978221538));
#41832=CARTESIAN_POINT('Ctrl Pts',(-99.9799979995999,-2.,36.2511316452692));
#41833=CARTESIAN_POINT('Ctrl Pts',(-99.9799979995999,-2.,35.7488683547308));
#41834=CARTESIAN_POINT('Ctrl Pts',(-99.9810415029486,-1.94980991520061,
35.4810021778462));
#41835=CARTESIAN_POINT('Ctrl Pts',(-99.9848135889912,-1.74570051630388,
34.9882455069044));
#41836=CARTESIAN_POINT('Ctrl Pts',(-99.9874880579221,-1.591781571759,34.7633544470128));
#41837=CARTESIAN_POINT('Ctrl Pts',(-99.9925109419644,-1.23664555394558,
34.4082184291994));
#41838=CARTESIAN_POINT('Ctrl Pts',(-99.995185177515,-1.01175449350969,34.2542994841741));
#41839=CARTESIAN_POINT('Ctrl Pts',(-99.998956730068,-0.518997821386425,
34.050190084175));
#41840=CARTESIAN_POINT('Ctrl Pts',(-100.,-0.251131643913752,34.));
#41841=CARTESIAN_POINT('Ctrl Pts',(-100.,-7.63278329429795E-16,34.));
#41842=CARTESIAN_POINT('',(-99.9799979995999,2.,36.));
#41843=CARTESIAN_POINT('Ctrl Pts',(-99.9799979995999,2.,36.));
#41844=CARTESIAN_POINT('Ctrl Pts',(-99.9799979995999,2.,36.2511316452692));
#41845=CARTESIAN_POINT('Ctrl Pts',(-99.9810415029486,1.94980991520061,36.5189978221538));
#41846=CARTESIAN_POINT('Ctrl Pts',(-99.9848135889912,1.74570051630387,37.0117544930956));
#41847=CARTESIAN_POINT('Ctrl Pts',(-99.9874880579221,1.591781571759,37.2366455529872));
#41848=CARTESIAN_POINT('Ctrl Pts',(-99.9925109419644,1.23664555394557,37.5917815708006));
#41849=CARTESIAN_POINT('Ctrl Pts',(-99.995185177515,1.01175449350969,37.7457005158259));
#41850=CARTESIAN_POINT('Ctrl Pts',(-99.998956730068,0.518997821386425,37.9498099158249));
#41851=CARTESIAN_POINT('Ctrl Pts',(-100.,0.25113164391375,38.));
#41852=CARTESIAN_POINT('Ctrl Pts',(-100.,-6.93889390390723E-17,38.));
#41853=CARTESIAN_POINT('',(-89.9777750336159,2.,36.));
#41854=CARTESIAN_POINT('',(-94.,2.,36.));
#41855=CARTESIAN_POINT('',(-90.,-5.78846635231938E-15,38.));
#41856=CARTESIAN_POINT('Ctrl Pts',(-90.,-6.24500451351651E-16,38.));
#41857=CARTESIAN_POINT('Ctrl Pts',(-90.,0.251133328053565,38.));
#41858=CARTESIAN_POINT('Ctrl Pts',(-89.9988407998655,0.519000232590761,
37.9498092576397));
#41859=CARTESIAN_POINT('Ctrl Pts',(-89.9946501491172,1.01175644254643,37.7456993679115));
#41860=CARTESIAN_POINT('Ctrl Pts',(-89.9916787455059,1.23664644642618,37.59178067832));
#41861=CARTESIAN_POINT('Ctrl Pts',(-89.9860976603374,1.59178067978086,37.2366464449653));
#41862=CARTESIAN_POINT('Ctrl Pts',(-89.9831259365723,1.74569936855886,37.0117564418786));
#41863=CARTESIAN_POINT('Ctrl Pts',(-89.9789345539658,1.9498092567713,36.519000233792));
#41864=CARTESIAN_POINT('Ctrl Pts',(-89.9777750336159,2.,36.2511333301197));
#41865=CARTESIAN_POINT('Ctrl Pts',(-89.9777750336159,2.,36.));
#41866=CARTESIAN_POINT('',(-90.,-5.16396590096773E-15,34.));
#41867=CARTESIAN_POINT('Ctrl Pts',(-90.,6.24500451351651E-16,34.));
#41868=CARTESIAN_POINT('Ctrl Pts',(-90.,-0.251133328053567,34.));
#41869=CARTESIAN_POINT('Ctrl Pts',(-89.9988407998655,-0.519000232590761,
34.0501907423603));
#41870=CARTESIAN_POINT('Ctrl Pts',(-89.9946501491172,-1.01175644254643,
34.2543006320885));
#41871=CARTESIAN_POINT('Ctrl Pts',(-89.9916787455059,-1.23664644642618,
34.40821932168));
#41872=CARTESIAN_POINT('Ctrl Pts',(-89.9860976603374,-1.59178067978086,
34.7633535550347));
#41873=CARTESIAN_POINT('Ctrl Pts',(-89.9831259365723,-1.74569936855887,
34.9882435581214));
#41874=CARTESIAN_POINT('Ctrl Pts',(-89.9789345539658,-1.94980925677131,
35.480999766208));
#41875=CARTESIAN_POINT('Ctrl Pts',(-89.9777750336159,-2.,35.7488666698804));
#41876=CARTESIAN_POINT('Ctrl Pts',(-89.9777750336159,-2.,36.2511333301197));
#41877=CARTESIAN_POINT('Ctrl Pts',(-89.9789345539658,-1.9498092567713,36.519000233792));
#41878=CARTESIAN_POINT('Ctrl Pts',(-89.9831259365723,-1.74569936855886,
37.0117564418786));
#41879=CARTESIAN_POINT('Ctrl Pts',(-89.9860976603374,-1.59178067978086,
37.2366464449653));
#41880=CARTESIAN_POINT('Ctrl Pts',(-89.9916787455059,-1.23664644642618,
37.59178067832));
#41881=CARTESIAN_POINT('Ctrl Pts',(-89.9946501491172,-1.01175644254643,
37.7456993679115));
#41882=CARTESIAN_POINT('Ctrl Pts',(-89.9988407998655,-0.519000232590762,
37.9498092576397));
#41883=CARTESIAN_POINT('Ctrl Pts',(-90.,-0.251133328053566,38.));
#41884=CARTESIAN_POINT('Ctrl Pts',(-90.,-4.85722573273506E-16,38.));
#41885=CARTESIAN_POINT('Ctrl Pts',(-89.9777750336159,2.,36.));
#41886=CARTESIAN_POINT('Ctrl Pts',(-89.9777750336159,2.,35.7488666698804));
#41887=CARTESIAN_POINT('Ctrl Pts',(-89.9789345539658,1.94980925677131,35.480999766208));
#41888=CARTESIAN_POINT('Ctrl Pts',(-89.9831259365723,1.74569936855887,34.9882435581214));
#41889=CARTESIAN_POINT('Ctrl Pts',(-89.9860976603374,1.59178067978086,34.7633535550347));
#41890=CARTESIAN_POINT('Ctrl Pts',(-89.9916787455059,1.23664644642618,34.40821932168));
#41891=CARTESIAN_POINT('Ctrl Pts',(-89.9946501491172,1.01175644254643,34.2543006320885));
#41892=CARTESIAN_POINT('Ctrl Pts',(-89.9988407998655,0.519000232590761,
34.0501907423603));
#41893=CARTESIAN_POINT('Ctrl Pts',(-90.,0.251133328053567,34.));
#41894=CARTESIAN_POINT('Ctrl Pts',(-90.,6.93889390390723E-17,34.));
#41895=CARTESIAN_POINT('Ctrl Pts',(-100.,2.77555756156289E-16,34.));
#41896=CARTESIAN_POINT('Ctrl Pts',(-100.,0.251131643913752,34.));
#41897=CARTESIAN_POINT('Ctrl Pts',(-99.998956730068,0.518997821386424,34.050190084175));
#41898=CARTESIAN_POINT('Ctrl Pts',(-99.995185177515,1.01175449350969,34.2542994841741));
#41899=CARTESIAN_POINT('Ctrl Pts',(-99.9925109419644,1.23664555394558,34.4082184291994));
#41900=CARTESIAN_POINT('Ctrl Pts',(-99.9874880579221,1.591781571759,34.7633544470128));
#41901=CARTESIAN_POINT('Ctrl Pts',(-99.9848135889912,1.74570051630388,34.9882455069044));
#41902=CARTESIAN_POINT('Ctrl Pts',(-99.9810415029486,1.94980991520061,35.4810021778462));
#41903=CARTESIAN_POINT('Ctrl Pts',(-99.9799979995999,2.,35.7488683547308));
#41904=CARTESIAN_POINT('Ctrl Pts',(-99.9799979995999,2.,36.));
#41905=CARTESIAN_POINT('Origin',(94.,0.,36.));
#41906=CARTESIAN_POINT('',(100.,0.,38.));
#41907=CARTESIAN_POINT('',(100.,0.,34.));
#41908=CARTESIAN_POINT('Ctrl Pts',(100.,5.55111512312578E-16,38.));
#41909=CARTESIAN_POINT('Ctrl Pts',(100.,0.251131643913751,38.));
#41910=CARTESIAN_POINT('Ctrl Pts',(99.998956730068,0.518997821386424,37.949809915825));
#41911=CARTESIAN_POINT('Ctrl Pts',(99.995185177515,1.01175449350968,37.7457005158259));
#41912=CARTESIAN_POINT('Ctrl Pts',(99.9925109419644,1.23664555394557,37.5917815708006));
#41913=CARTESIAN_POINT('Ctrl Pts',(99.9874880579221,1.591781571759,37.2366455529872));
#41914=CARTESIAN_POINT('Ctrl Pts',(99.9848135889912,1.74570051630387,37.0117544930956));
#41915=CARTESIAN_POINT('Ctrl Pts',(99.9810415029486,1.94980991520061,36.5189978221538));
#41916=CARTESIAN_POINT('Ctrl Pts',(99.9799979995999,2.,36.2511316452692));
#41917=CARTESIAN_POINT('Ctrl Pts',(99.9799979995999,2.,35.7488683547308));
#41918=CARTESIAN_POINT('Ctrl Pts',(99.9810415029486,1.94980991520061,35.4810021778462));
#41919=CARTESIAN_POINT('Ctrl Pts',(99.9848135889912,1.74570051630388,34.9882455069044));
#41920=CARTESIAN_POINT('Ctrl Pts',(99.9874880579221,1.591781571759,34.7633544470128));
#41921=CARTESIAN_POINT('Ctrl Pts',(99.9925109419644,1.23664555394558,34.4082184291994));
#41922=CARTESIAN_POINT('Ctrl Pts',(99.995185177515,1.01175449350969,34.2542994841741));
#41923=CARTESIAN_POINT('Ctrl Pts',(99.998956730068,0.518997821386425,34.050190084175));
#41924=CARTESIAN_POINT('Ctrl Pts',(100.,0.251131643913752,34.));
#41925=CARTESIAN_POINT('Ctrl Pts',(100.,7.63278329429795E-16,34.));
#41926=CARTESIAN_POINT('',(99.9799979995999,-2.,36.));
#41927=CARTESIAN_POINT('Ctrl Pts',(99.9799979995999,-2.,36.));
#41928=CARTESIAN_POINT('Ctrl Pts',(99.9799979995999,-2.,36.2511316452692));
#41929=CARTESIAN_POINT('Ctrl Pts',(99.9810415029486,-1.94980991520061,36.5189978221538));
#41930=CARTESIAN_POINT('Ctrl Pts',(99.9848135889912,-1.74570051630387,37.0117544930956));
#41931=CARTESIAN_POINT('Ctrl Pts',(99.9874880579221,-1.591781571759,37.2366455529872));
#41932=CARTESIAN_POINT('Ctrl Pts',(99.9925109419644,-1.23664555394557,37.5917815708006));
#41933=CARTESIAN_POINT('Ctrl Pts',(99.995185177515,-1.01175449350969,37.7457005158259));
#41934=CARTESIAN_POINT('Ctrl Pts',(99.998956730068,-0.518997821386425,37.9498099158249));
#41935=CARTESIAN_POINT('Ctrl Pts',(100.,-0.25113164391375,38.));
#41936=CARTESIAN_POINT('Ctrl Pts',(100.,6.93889390390723E-17,38.));
#41937=CARTESIAN_POINT('',(89.9777750336159,-2.,36.));
#41938=CARTESIAN_POINT('',(94.,-2.,36.));
#41939=CARTESIAN_POINT('Ctrl Pts',(89.9777750336159,-2.,36.));
#41940=CARTESIAN_POINT('Ctrl Pts',(89.9777750336159,-2.,35.7488666698804));
#41941=CARTESIAN_POINT('Ctrl Pts',(89.9789345539658,-1.94980925677131,35.480999766208));
#41942=CARTESIAN_POINT('Ctrl Pts',(89.9831259365723,-1.74569936855887,34.9882435581214));
#41943=CARTESIAN_POINT('Ctrl Pts',(89.9860976603374,-1.59178067978086,34.7633535550347));
#41944=CARTESIAN_POINT('Ctrl Pts',(89.9916787455059,-1.23664644642618,34.40821932168));
#41945=CARTESIAN_POINT('Ctrl Pts',(89.9946501491172,-1.01175644254643,34.2543006320885));
#41946=CARTESIAN_POINT('Ctrl Pts',(89.9988407998655,-0.519000232590761,
34.0501907423603));
#41947=CARTESIAN_POINT('Ctrl Pts',(90.,-0.251133328053568,34.));
#41948=CARTESIAN_POINT('Ctrl Pts',(90.,0.251133328053567,34.));
#41949=CARTESIAN_POINT('Ctrl Pts',(89.9988407998655,0.519000232590761,34.0501907423603));
#41950=CARTESIAN_POINT('Ctrl Pts',(89.9946501491172,1.01175644254643,34.2543006320885));
#41951=CARTESIAN_POINT('Ctrl Pts',(89.9916787455059,1.23664644642618,34.40821932168));
#41952=CARTESIAN_POINT('Ctrl Pts',(89.9860976603374,1.59178067978086,34.7633535550347));
#41953=CARTESIAN_POINT('Ctrl Pts',(89.9831259365723,1.74569936855887,34.9882435581214));
#41954=CARTESIAN_POINT('Ctrl Pts',(89.9789345539658,1.94980925677131,35.480999766208));
#41955=CARTESIAN_POINT('Ctrl Pts',(89.9777750336159,2.,35.7488666698804));
#41956=CARTESIAN_POINT('Ctrl Pts',(89.9777750336159,2.,36.2511333301197));
#41957=CARTESIAN_POINT('Ctrl Pts',(89.9789345539658,1.9498092567713,36.519000233792));
#41958=CARTESIAN_POINT('Ctrl Pts',(89.9831259365723,1.74569936855886,37.0117564418786));
#41959=CARTESIAN_POINT('Ctrl Pts',(89.9860976603374,1.59178067978086,37.2366464449653));
#41960=CARTESIAN_POINT('Ctrl Pts',(89.9916787455059,1.23664644642618,37.59178067832));
#41961=CARTESIAN_POINT('Ctrl Pts',(89.9946501491172,1.01175644254643,37.7456993679115));
#41962=CARTESIAN_POINT('Ctrl Pts',(89.9988407998655,0.519000232590762,37.9498092576397));
#41963=CARTESIAN_POINT('Ctrl Pts',(90.,0.251133328053566,38.));
#41964=CARTESIAN_POINT('Ctrl Pts',(90.,-0.251133328053565,38.));
#41965=CARTESIAN_POINT('Ctrl Pts',(89.9988407998655,-0.519000232590761,
37.9498092576397));
#41966=CARTESIAN_POINT('Ctrl Pts',(89.9946501491172,-1.01175644254643,37.7456993679115));
#41967=CARTESIAN_POINT('Ctrl Pts',(89.9916787455059,-1.23664644642618,37.59178067832));
#41968=CARTESIAN_POINT('Ctrl Pts',(89.9860976603374,-1.59178067978086,37.2366464449653));
#41969=CARTESIAN_POINT('Ctrl Pts',(89.9831259365723,-1.74569936855886,37.0117564418786));
#41970=CARTESIAN_POINT('Ctrl Pts',(89.9789345539658,-1.9498092567713,36.519000233792));
#41971=CARTESIAN_POINT('Ctrl Pts',(89.9777750336159,-2.,36.2511333301197));
#41972=CARTESIAN_POINT('Ctrl Pts',(89.9777750336159,-2.,36.));
#41973=CARTESIAN_POINT('Ctrl Pts',(100.,-2.77555756156289E-16,34.));
#41974=CARTESIAN_POINT('Ctrl Pts',(100.,-0.251131643913752,34.));
#41975=CARTESIAN_POINT('Ctrl Pts',(99.998956730068,-0.518997821386424,34.050190084175));
#41976=CARTESIAN_POINT('Ctrl Pts',(99.995185177515,-1.01175449350969,34.2542994841741));
#41977=CARTESIAN_POINT('Ctrl Pts',(99.9925109419644,-1.23664555394558,34.4082184291994));
#41978=CARTESIAN_POINT('Ctrl Pts',(99.9874880579221,-1.591781571759,34.7633544470128));
#41979=CARTESIAN_POINT('Ctrl Pts',(99.9848135889912,-1.74570051630388,34.9882455069044));
#41980=CARTESIAN_POINT('Ctrl Pts',(99.9810415029486,-1.94980991520061,35.4810021778462));
#41981=CARTESIAN_POINT('Ctrl Pts',(99.9799979995999,-2.,35.7488683547308));
#41982=CARTESIAN_POINT('Ctrl Pts',(99.9799979995999,-2.,36.));
#41983=CARTESIAN_POINT('Origin',(-36.3549260746835,87.7685555885722,107.));
#41984=CARTESIAN_POINT('Ctrl Pts',(-38.2683920713485,89.4045427919473,107.));
#41985=CARTESIAN_POINT('Ctrl Pts',(-38.3305296090722,89.3461487645065,107.));
#41986=CARTESIAN_POINT('Ctrl Pts',(-38.3892917721933,89.2845008284283,107.));
#41987=CARTESIAN_POINT('Ctrl Pts',(-38.4446665812863,89.2199754596173,107.));
#41988=CARTESIAN_POINT('Ctrl Pts',(-38.501396469585,89.1538710878815,107.));
#41989=CARTESIAN_POINT('Ctrl Pts',(-38.5545716594879,89.0847462416478,107.));
#41990=CARTESIAN_POINT('Ctrl Pts',(-38.6041503825645,89.0129594416844,107.));
#41991=CARTESIAN_POINT('Ctrl Pts',(-38.617088116682,88.9942264353979,107.));
#41992=CARTESIAN_POINT('Ctrl Pts',(-38.6297807726147,88.9753119423136,107.));
#41993=CARTESIAN_POINT('Ctrl Pts',(-38.6422272327037,88.9562219002017,107.));
#41994=CARTESIAN_POINT('Ctrl Pts',(-38.6523972170385,88.9406234547127,107.));
#41995=CARTESIAN_POINT('Ctrl Pts',(-38.662403269216,88.9249068962603,107.));
#41996=CARTESIAN_POINT('Ctrl Pts',(-38.6722359315353,88.9090900594939,107.));
#41997=CARTESIAN_POINT('Ctrl Pts',(-38.7196800505418,88.8327713716876,107.));
#41998=CARTESIAN_POINT('Ctrl Pts',(-38.7631406056323,88.7540453242351,107.));
#41999=CARTESIAN_POINT('Ctrl Pts',(-38.8025829106836,88.67330446842,107.));
#42000=CARTESIAN_POINT('Ctrl Pts',(-38.8344113785719,88.6081496116427,107.));
#42001=CARTESIAN_POINT('Ctrl Pts',(-38.8636227066877,88.5416816457212,107.));
#42002=CARTESIAN_POINT('Ctrl Pts',(-38.8901815095572,88.474089043938,107.));
#42003=CARTESIAN_POINT('Ctrl Pts',(-38.9007829847814,88.4471081104725,107.));
#42004=CARTESIAN_POINT('Ctrl Pts',(-38.9109616320996,88.4199478294018,107.));
#42005=CARTESIAN_POINT('Ctrl Pts',(-38.9207144403471,88.3926196422929,107.));
#42006=CARTESIAN_POINT('Ctrl Pts',(-38.9259553817286,88.3779340847521,107.));
#42007=CARTESIAN_POINT('Ctrl Pts',(-38.9310729716149,88.3632008585835,107.));
#42008=CARTESIAN_POINT('Ctrl Pts',(-38.9360627431239,88.3484342176154,107.));
#42009=CARTESIAN_POINT('Ctrl Pts',(-38.9656015479925,88.2610176043829,107.));
#42010=CARTESIAN_POINT('Ctrl Pts',(-38.9907048899124,88.1723198874215,107.));
#42011=CARTESIAN_POINT('Ctrl Pts',(-39.0113402006962,88.082738876299,107.));
#42012=CARTESIAN_POINT('Ctrl Pts',(-39.0322969781321,87.9917623297253,107.));
#42013=CARTESIAN_POINT('Ctrl Pts',(-39.0486459305825,87.8998739484332,107.));
#42014=CARTESIAN_POINT('Ctrl Pts',(-39.0603111188663,87.8074572392324,107.));
#42015=CARTESIAN_POINT('Ctrl Pts',(-39.0718855922787,87.7157592128064,107.));
#42016=CARTESIAN_POINT('Ctrl Pts',(-39.0788492094664,87.6235401137,107.));
#42017=CARTESIAN_POINT('Ctrl Pts',(-39.0810808446038,87.5311553610101,107.));
#42018=CARTESIAN_POINT('Ctrl Pts',(-39.0821914618531,87.4851782663684,107.));
#42019=CARTESIAN_POINT('Ctrl Pts',(-39.0821293210671,87.4391599303236,107.));
#42020=CARTESIAN_POINT('Ctrl Pts',(-39.0808746940999,87.3931434632704,107.));
#42021=CARTESIAN_POINT('Ctrl Pts',(-39.0805049187082,87.3795810598021,107.));
#42022=CARTESIAN_POINT('Ctrl Pts',(-39.0800315353698,87.3660188180032,107.));
#42023=CARTESIAN_POINT('Ctrl Pts',(-39.0794539826403,87.3524578415654,107.));
#42024=CARTESIAN_POINT('Ctrl Pts',(-39.0788334726149,87.3378882249662,107.));
#42025=CARTESIAN_POINT('Ctrl Pts',(-39.0780931235918,87.3233298551507,107.));
#42026=CARTESIAN_POINT('Ctrl Pts',(-39.0772328870959,87.3087866606173,107.));
#42027=CARTESIAN_POINT('Ctrl Pts',(-39.071581078401,87.2132369441038,107.));
#42028=CARTESIAN_POINT('Ctrl Pts',(-39.0607566330613,87.1183089467729,107.));
#42029=CARTESIAN_POINT('Ctrl Pts',(-39.0446890962994,87.0243983125872,107.));
#42030=CARTESIAN_POINT('Ctrl Pts',(-39.0423087640973,87.0104858809568,107.));
#42031=CARTESIAN_POINT('Ctrl Pts',(-39.039813274356,86.9965957440252,107.));
#42032=CARTESIAN_POINT('Ctrl Pts',(-39.0372023054818,86.9827291574775,107.));
#42033=CARTESIAN_POINT('Ctrl Pts',(-39.020256651193,86.8927325343363,107.));
#42034=CARTESIAN_POINT('Ctrl Pts',(-38.998451114988,86.8037280854647,107.));
#42035=CARTESIAN_POINT('Ctrl Pts',(-38.9720882464109,86.7159480589121,107.));
#42036=CARTESIAN_POINT('Ctrl Pts',(-38.9451294332351,86.626183725055,107.));
#42037=CARTESIAN_POINT('Ctrl Pts',(-38.9134047085586,86.5376990962214,107.));
#42038=CARTESIAN_POINT('Ctrl Pts',(-38.8771833655368,86.4507462170881,107.));
#42039=CARTESIAN_POINT('Ctrl Pts',(-38.8646932387025,86.4207624451355,107.));
#42040=CARTESIAN_POINT('Ctrl Pts',(-38.8516679859885,86.3909608889171,107.));
#42041=CARTESIAN_POINT('Ctrl Pts',(-38.838117277065,86.3613522223643,107.));
#42042=CARTESIAN_POINT('Ctrl Pts',(-38.8314262146987,86.3467320696029,107.));
#42043=CARTESIAN_POINT('Ctrl Pts',(-38.8246070262069,86.3321589503315,107.));
#42044=CARTESIAN_POINT('Ctrl Pts',(-38.8176608165039,86.3176341721329,107.));
#42045=CARTESIAN_POINT('Ctrl Pts',(-38.8121670423093,86.3061464896326,107.));
#42046=CARTESIAN_POINT('Ctrl Pts',(-38.8065942532154,86.2946900708772,107.));
#42047=CARTESIAN_POINT('Ctrl Pts',(-38.8009475899525,86.283274492168,107.));
#42048=CARTESIAN_POINT('Ctrl Pts',(-38.758223644909,86.1969016141157,107.));
#42049=CARTESIAN_POINT('Ctrl Pts',(-38.7112088421257,86.1127270557926,107.));
#42050=CARTESIAN_POINT('Ctrl Pts',(-38.660245836794,86.0310004544778,107.));
#42051=CARTESIAN_POINT('Ctrl Pts',(-38.6082721210866,85.9476530318752,107.));
#42052=CARTESIAN_POINT('Ctrl Pts',(-38.5521917328472,85.8668508545203,107.));
#42053=CARTESIAN_POINT('Ctrl Pts',(-38.4923131112639,85.7888657379894,107.));
#42054=CARTESIAN_POINT('Ctrl Pts',(-38.4319476605325,85.7102465816819,107.));
#42055=CARTESIAN_POINT('Ctrl Pts',(-38.3677215052906,85.6344896425683,107.));
#42056=CARTESIAN_POINT('Ctrl Pts',(-38.299901338034,85.5618926996275,107.));
#42057=CARTESIAN_POINT('Ctrl Pts',(-38.262900667006,85.5222859615134,107.));
#42058=CARTESIAN_POINT('Ctrl Pts',(-38.2248294325612,85.4836201949921,107.));
#42059=CARTESIAN_POINT('Ctrl Pts',(-38.1857255936742,85.4459475341521,107.));
#42060=CARTESIAN_POINT('Ctrl Pts',(-38.1737580085947,85.4344179558138,107.));
#42061=CARTESIAN_POINT('Ctrl Pts',(-38.1616936808026,85.4229814184087,107.));
#42062=CARTESIAN_POINT('Ctrl Pts',(-38.1495336354026,85.4116394784339,107.));
#42063=CARTESIAN_POINT('Ctrl Pts',(-38.1389878579288,85.4018032014168,107.));
#42064=CARTESIAN_POINT('Ctrl Pts',(-38.1283712028283,85.3920391899121,107.));
#42065=CARTESIAN_POINT('Ctrl Pts',(-38.1176934507031,85.3823564375337,107.));
#42066=CARTESIAN_POINT('Ctrl Pts',(-38.0421189670067,85.3138243154934,107.));
#42067=CARTESIAN_POINT('Ctrl Pts',(-37.9633677633205,85.2492485396459,107.));
#42068=CARTESIAN_POINT('Ctrl Pts',(-37.8817671861085,85.1889108818132,107.));
#42069=CARTESIAN_POINT('Ctrl Pts',(-37.8000624207147,85.1284961844413,107.));
#42070=CARTESIAN_POINT('Ctrl Pts',(-37.7155004275651,85.0723295959512,107.));
#42071=CARTESIAN_POINT('Ctrl Pts',(-37.6283645341542,85.0207197688895,107.));
#42072=CARTESIAN_POINT('Ctrl Pts',(-37.5429608768295,84.9701359301014,107.));
#42073=CARTESIAN_POINT('Ctrl Pts',(-37.4550839747521,84.9239288015609,107.));
#42074=CARTESIAN_POINT('Ctrl Pts',(-37.3649665022594,84.8824247956419,107.));
#42075=CARTESIAN_POINT('Ctrl Pts',(-37.3246172470079,84.8638417652653,107.));
#42076=CARTESIAN_POINT('Ctrl Pts',(-37.2838184192053,84.8462021227698,107.));
#42077=CARTESIAN_POINT('Ctrl Pts',(-37.2425891498101,84.8295381139694,107.));
#42078=CARTESIAN_POINT('Ctrl Pts',(-37.2121695076316,84.817243130517,107.));
#42079=CARTESIAN_POINT('Ctrl Pts',(-37.1815155207895,84.8054792999133,107.));
#42080=CARTESIAN_POINT('Ctrl Pts',(-37.1506394582515,84.7942439414617,107.));
#42081=CARTESIAN_POINT('Ctrl Pts',(-35.5611267921506,84.7993326348266,107.));
#42082=CARTESIAN_POINT('Ctrl Pts',(-35.4662928667291,84.8340233083661,107.));
#42083=CARTESIAN_POINT('Ctrl Pts',(-35.373502094942,84.8737048604511,107.));
#42084=CARTESIAN_POINT('Ctrl Pts',(-35.2829954003415,84.9180569417674,107.));
#42085=CARTESIAN_POINT('Ctrl Pts',(-35.1912158404665,84.9630327805242,107.));
#42086=CARTESIAN_POINT('Ctrl Pts',(-35.1017843865515,85.0128121445763,107.));
#42087=CARTESIAN_POINT('Ctrl Pts',(-35.0149862950964,85.0671016605279,107.));
#42088=CARTESIAN_POINT('Ctrl Pts',(-34.9904732710836,85.0824337972818,107.));
#42089=CARTESIAN_POINT('Ctrl Pts',(-34.9661705183484,85.098125863753,107.));
#42090=CARTESIAN_POINT('Ctrl Pts',(-34.9420850585175,85.1141717075186,107.));
#42091=CARTESIAN_POINT('Ctrl Pts',(-34.9227555338565,85.1270491254692,107.));
#42092=CARTESIAN_POINT('Ctrl Pts',(-34.9035638566542,85.1401560264525,107.));
#42093=CARTESIAN_POINT('Ctrl Pts',(-34.8845329423808,85.1534754654736,107.));
#42094=CARTESIAN_POINT('Ctrl Pts',(-34.8018258386928,85.211360872783,107.));
#42095=CARTESIAN_POINT('Ctrl Pts',(-34.7220735941393,85.2733084226108,107.));
#42096=CARTESIAN_POINT('Ctrl Pts',(-34.6455425705562,85.3390207553953,107.));
#42097=CARTESIAN_POINT('Ctrl Pts',(-34.5865493779202,85.3896744658125,107.));
#42098=CARTESIAN_POINT('Ctrl Pts',(-34.5294708526726,85.442566101346,107.));
#42099=CARTESIAN_POINT('Ctrl Pts',(-34.4744465628682,85.4975712321909,107.));
#42100=CARTESIAN_POINT('Ctrl Pts',(-34.4451578114394,85.5268497855414,107.));
#42101=CARTESIAN_POINT('Ctrl Pts',(-34.4164513632894,85.5567273046795,107.));
#42102=CARTESIAN_POINT('Ctrl Pts',(-34.388350288722,85.5871858552371,107.));
#42103=CARTESIAN_POINT('Ctrl Pts',(-34.3787142836071,85.5976302511715,107.));
#42104=CARTESIAN_POINT('Ctrl Pts',(-34.3691501941652,85.6081422590004,107.));
#42105=CARTESIAN_POINT('Ctrl Pts',(-34.3596655870238,85.6187135430261,107.));
#42106=CARTESIAN_POINT('Ctrl Pts',(-34.2938683933846,85.6920492976525,107.));
#42107=CARTESIAN_POINT('Ctrl Pts',(-34.2318033500797,85.7683316754912,107.));
#42108=CARTESIAN_POINT('Ctrl Pts',(-34.1737142259206,85.8472821195271,107.));
#42109=CARTESIAN_POINT('Ctrl Pts',(-34.1161515595356,85.9255170410685,107.));
#42110=CARTESIAN_POINT('Ctrl Pts',(-34.0624926380258,86.0063726715474,107.));
#42111=CARTESIAN_POINT('Ctrl Pts',(-34.0130204055193,86.0896003448039,107.));
#42112=CARTESIAN_POINT('Ctrl Pts',(-33.964962467509,86.170448735092,107.));
#42113=CARTESIAN_POINT('Ctrl Pts',(-33.92085505662,86.2535361835536,107.));
#42114=CARTESIAN_POINT('Ctrl Pts',(-33.8810053242648,86.3386450701133,107.));
#42115=CARTESIAN_POINT('Ctrl Pts',(-33.8602009063501,86.3830780120577,107.));
#42116=CARTESIAN_POINT('Ctrl Pts',(-33.8405577745803,86.4280620243428,107.));
#42117=CARTESIAN_POINT('Ctrl Pts',(-33.8221253291101,86.4735663764393,107.));
#42118=CARTESIAN_POINT('Ctrl Pts',(-33.8150672434759,86.4909907390581,107.));
#42119=CARTESIAN_POINT('Ctrl Pts',(-33.8081867174046,86.5084913952829,107.));
#42120=CARTESIAN_POINT('Ctrl Pts',(-33.8014866864851,86.5260666110052,107.));
#42121=CARTESIAN_POINT('Ctrl Pts',(-33.7962449527397,86.5398164880495,107.));
#42122=CARTESIAN_POINT('Ctrl Pts',(-33.791113595039,86.5536125010622,107.));
#42123=CARTESIAN_POINT('Ctrl Pts',(-33.7860991485526,86.5674391067525,107.));
#42124=CARTESIAN_POINT('Ctrl Pts',(-33.7544154646644,86.6548022494497,107.));
#42125=CARTESIAN_POINT('Ctrl Pts',(-33.7273406062928,86.7435263402015,107.));
#42126=CARTESIAN_POINT('Ctrl Pts',(-33.705125829678,86.8333878288782,107.));
#42127=CARTESIAN_POINT('Ctrl Pts',(-33.7001418550498,86.8535486158801,107.));
#42128=CARTESIAN_POINT('Ctrl Pts',(-33.6954027145293,86.8737666931234,107.));
#42129=CARTESIAN_POINT('Ctrl Pts',(-33.6909116062639,86.8940395916533,107.));
#42130=CARTESIAN_POINT('Ctrl Pts',(-33.6705458557277,86.9859707520051,107.));
#42131=CARTESIAN_POINT('Ctrl Pts',(-33.6552763187112,87.0790295393631,107.));
#42132=CARTESIAN_POINT('Ctrl Pts',(-33.6449931699608,87.1728243655036,107.));
#42133=CARTESIAN_POINT('Ctrl Pts',(-33.6342593131593,87.2707301973596,107.));
#42134=CARTESIAN_POINT('Ctrl Pts',(-33.6289585408132,87.3694392403859,107.));
#42135=CARTESIAN_POINT('Ctrl Pts',(-33.6290234054697,87.4684914760975,107.));
#42136=CARTESIAN_POINT('Ctrl Pts',(-33.6290487774748,87.5072360553908,107.));
#42137=CARTESIAN_POINT('Ctrl Pts',(-33.6298956946779,87.5460328865882,107.));
#42138=CARTESIAN_POINT('Ctrl Pts',(-33.6315623444562,87.5848532118375,107.));
#42139=CARTESIAN_POINT('Ctrl Pts',(-33.6320953845293,87.5972690110524,107.));
#42140=CARTESIAN_POINT('Ctrl Pts',(-33.6327122710738,87.6096859021259,107.));
#42141=CARTESIAN_POINT('Ctrl Pts',(-33.6334122429631,87.6220932757044,107.));
#42142=CARTESIAN_POINT('Ctrl Pts',(-33.638651466045,87.7149612880346,107.));
#42143=CARTESIAN_POINT('Ctrl Pts',(-33.648547110654,87.807446071697,107.));
#42144=CARTESIAN_POINT('Ctrl Pts',(-33.6629757175006,87.8991760479908,107.));
#42145=CARTESIAN_POINT('Ctrl Pts',(-33.6773703353928,87.9906899392528,107.));
#42146=CARTESIAN_POINT('Ctrl Pts',(-33.696276994312,88.0814535204309,107.));
#42147=CARTESIAN_POINT('Ctrl Pts',(-33.7196217814369,88.1710808801793,107.));
#42148=CARTESIAN_POINT('Ctrl Pts',(-33.7425704165735,88.2591872983752,107.));
#42149=CARTESIAN_POINT('Ctrl Pts',(-33.7698082987973,88.3461965157412,107.));
#42150=CARTESIAN_POINT('Ctrl Pts',(-33.8013056556184,88.4317128384291,107.));
#42151=CARTESIAN_POINT('Ctrl Pts',(-33.8171471032868,88.4747228712503,107.));
#42152=CARTESIAN_POINT('Ctrl Pts',(-33.8340666009129,88.5173547357403,107.));
#42153=CARTESIAN_POINT('Ctrl Pts',(-33.8520637782135,88.5595543004123,107.));
#42154=CARTESIAN_POINT('Ctrl Pts',(-33.8576294800274,88.5726046910218,107.));
#42155=CARTESIAN_POINT('Ctrl Pts',(-33.8632982646163,88.5856137165589,107.));
#42156=CARTESIAN_POINT('Ctrl Pts',(-33.8690701619053,88.5985797184015,107.));
#42157=CARTESIAN_POINT('Ctrl Pts',(-33.8747496320563,88.6113380917329,107.));
#42158=CARTESIAN_POINT('Ctrl Pts',(-33.8805254577359,88.6240469437888,107.));
#42159=CARTESIAN_POINT('Ctrl Pts',(-33.886395849193,88.6367017889012,107.));
#42160=CARTESIAN_POINT('Ctrl Pts',(-33.9238756556946,88.7174972775129,107.));
#42161=CARTESIAN_POINT('Ctrl Pts',(-33.9652256181719,88.7961359866757,107.));
#42162=CARTESIAN_POINT('Ctrl Pts',(-34.0103760601782,88.8722703240689,107.));
#42163=CARTESIAN_POINT('Ctrl Pts',(-34.0547690647657,88.9471274426035,107.));
#42164=CARTESIAN_POINT('Ctrl Pts',(-34.1028365599303,89.0195641800131,107.));
#42165=CARTESIAN_POINT('Ctrl Pts',(-34.1545485303629,89.0892159682587,107.));
#42166=CARTESIAN_POINT('Ctrl Pts',(-34.2046829766307,89.1567429606752,107.));
#42167=CARTESIAN_POINT('Ctrl Pts',(-34.2582433760492,89.2216527685488,107.));
#42168=CARTESIAN_POINT('Ctrl Pts',(-34.3152300879658,89.2835728963379,107.));
#42169=CARTESIAN_POINT('Ctrl Pts',(-34.3361977081016,89.3063557113939,107.));
#42170=CARTESIAN_POINT('Ctrl Pts',(-34.3576294231801,89.3287333523195,107.));
#42171=CARTESIAN_POINT('Ctrl Pts',(-34.3795260622952,89.3506856545374,107.));
#42172=CARTESIAN_POINT('Ctrl Pts',(-34.3986034990632,89.3698115877581,107.));
#42173=CARTESIAN_POINT('Ctrl Pts',(-34.4180338691283,89.3886146337316,107.));
#42174=CARTESIAN_POINT('Ctrl Pts',(-34.4378070356397,89.4070896639596,107.));
#42175=CARTESIAN_POINT('Origin',(-36.3549260746835,87.7685555885722,124.208423447177));
#42176=CARTESIAN_POINT('Ctrl Pts',(-39.4317255112881,87.7704831500192,121.708423447178));
#42177=CARTESIAN_POINT('Ctrl Pts',(-39.4326481971992,87.8937580425098,121.702019850418));
#42178=CARTESIAN_POINT('Ctrl Pts',(-39.3701217699364,89.029664773114,121.642966745928));
#42179=CARTESIAN_POINT('Ctrl Pts',(-37.9573947132227,91.0220940158023,121.531264133707));
#42180=CARTESIAN_POINT('Ctrl Pts',(-34.5067287733102,90.8887185705161,121.373315610515));
#42181=CARTESIAN_POINT('Ctrl Pts',(-32.7318387507372,87.9267773779968,121.215367087322));
#42182=CARTESIAN_POINT('Ctrl Pts',(-34.2418569809606,84.8211911081587,121.05741856413));
#42183=CARTESIAN_POINT('Ctrl Pts',(-37.6677476301795,84.3879830560575,120.899470040937));
#42184=CARTESIAN_POINT('Ctrl Pts',(-39.314294541848,86.3263542158685,120.783138335287));
#42185=CARTESIAN_POINT('Ctrl Pts',(-39.4311721662448,87.5529959287177,120.719456137367));
#42186=CARTESIAN_POINT('Ctrl Pts',(-39.4292403360613,87.7658718692203,120.708423447177));
#42187=CARTESIAN_POINT('Ctrl Pts',(-39.4252046869538,87.7655406593158,121.791576552823));
#42188=CARTESIAN_POINT('Ctrl Pts',(-39.4202197564572,88.4585591084465,121.755752019753));
#42189=CARTESIAN_POINT('Ctrl Pts',(-38.8478323893262,90.1797487563936,121.667277978953));
#42190=CARTESIAN_POINT('Ctrl Pts',(-36.0033917073514,91.3774170351665,121.526154430422));
#42191=CARTESIAN_POINT('Ctrl Pts',(-33.1409989526284,89.4482950386239,121.36820590723));
#42192=CARTESIAN_POINT('Ctrl Pts',(-33.1913893007143,85.9950129878222,121.210257384038));
#42193=CARTESIAN_POINT('Ctrl Pts',(-36.1106392417851,84.1503274667491,121.052308860845));
#42194=CARTESIAN_POINT('Ctrl Pts',(-38.8854864734731,85.418769658119,120.912748583773));
#42195=CARTESIAN_POINT('Ctrl Pts',(-39.4210162770085,87.1075071559934,120.825837814433));
#42196=CARTESIAN_POINT('Ctrl Pts',(-39.4253674987814,87.7707064726519,120.791576552823));
#42197=CARTESIAN_POINT('Ctrl Pts',(-34.4414600780185,89.4045427919472,122.));
#42198=CARTESIAN_POINT('Ctrl Pts',(-33.9002646916968,88.7715555857257,121.947350492269));
#42199=CARTESIAN_POINT('Ctrl Pts',(-33.5049255901432,86.9365247300264,121.842051476807));
#42200=CARTESIAN_POINT('Ctrl Pts',(-35.4957255906178,84.923355640163,121.684102953615));
#42201=CARTESIAN_POINT('Ctrl Pts',(-38.2666279976808,85.4956008231392,121.526154430423));
#42202=CARTESIAN_POINT('Ctrl Pts',(-39.3037452232225,88.1258670336349,121.36820590723));
#42203=CARTESIAN_POINT('Ctrl Pts',(-37.6675061291889,90.4335248387924,121.210257384038));
#42204=CARTESIAN_POINT('Ctrl Pts',(-34.841069980261,90.3242771786304,121.052308860845));
#42205=CARTESIAN_POINT('Ctrl Pts',(-33.3872597860761,87.8981548580944,120.894360337653));
#42206=CARTESIAN_POINT('Ctrl Pts',(-34.6241138269375,85.3543730346626,120.73641181446));
#42207=CARTESIAN_POINT('Ctrl Pts',(-37.4302565662928,84.9995328618419,120.578463291268));
#42208=CARTESIAN_POINT('Ctrl Pts',(-39.2614231073442,87.1552445435626,120.420514768075));
#42209=CARTESIAN_POINT('Ctrl Pts',(-38.4573604664392,89.8670446085888,120.262566244883));
#42210=CARTESIAN_POINT('Ctrl Pts',(-35.747082910027,90.6761997920055,120.10461772169));
#42211=CARTESIAN_POINT('Ctrl Pts',(-33.5879190399563,88.8490866434182,119.946669198498));
#42212=CARTESIAN_POINT('Ctrl Pts',(-33.9375159163837,86.0422867908315,119.788720675305));
#42213=CARTESIAN_POINT('Ctrl Pts',(-36.4789052445403,84.8006433564885,119.630772152113));
#42214=CARTESIAN_POINT('Ctrl Pts',(-38.9078863408608,86.2499151910518,119.47282362892));
#42215=CARTESIAN_POINT('Ctrl Pts',(-39.0221760519813,89.0760923234738,119.314875105728));
#42216=CARTESIAN_POINT('Ctrl Pts',(-36.7181513083396,90.7167655501525,119.156926582536));
#42217=CARTESIAN_POINT('Ctrl Pts',(-34.084801302592,89.6843865264073,118.998978059343));
#42218=CARTESIAN_POINT('Ctrl Pts',(-33.5097043799898,86.9149818314663,118.841029536151));
#42219=CARTESIAN_POINT('Ctrl Pts',(-35.5142834368846,84.9194865150593,118.683081012958));
#42220=CARTESIAN_POINT('Ctrl Pts',(-38.2810476053028,85.5071554706503,118.525132489766));
#42221=CARTESIAN_POINT('Ctrl Pts',(-39.3014559628199,88.1451671389155,118.367183966573));
#42222=CARTESIAN_POINT('Ctrl Pts',(-37.6503352851408,90.4417165670853,118.209235443381));
#42223=CARTESIAN_POINT('Ctrl Pts',(-34.8247064745657,90.3145922372931,118.051286920188));
#42224=CARTESIAN_POINT('Ctrl Pts',(-33.3864812358262,87.8790539119505,117.893338396996));
#42225=CARTESIAN_POINT('Ctrl Pts',(-34.6396546513419,85.3433301176302,117.735389873803));
#42226=CARTESIAN_POINT('Ctrl Pts',(-37.4480124987638,85.0064844978296,117.577441350611));
#42227=CARTESIAN_POINT('Ctrl Pts',(-39.2653021302004,87.1739247314519,117.419492827418));
#42228=CARTESIAN_POINT('Ctrl Pts',(-38.4438423071828,89.8804986783248,117.261544304226));
#42229=CARTESIAN_POINT('Ctrl Pts',(-35.7284256676752,90.6722380575748,117.103595781034));
#42230=CARTESIAN_POINT('Ctrl Pts',(-33.5810378930527,88.8312968536853,116.945647257841));
#42231=CARTESIAN_POINT('Ctrl Pts',(-33.9486501687198,86.0268004665349,116.787698734649));
#42232=CARTESIAN_POINT('Ctrl Pts',(-36.4979596247505,84.8015004754471,116.629750211456));
#42233=CARTESIAN_POINT('Ctrl Pts',(-38.9175849111044,86.2663391165282,116.471801688264));
#42234=CARTESIAN_POINT('Ctrl Pts',(-39.0137253702208,89.0931917449628,116.313853165071));
#42235=CARTESIAN_POINT('Ctrl Pts',(-36.6992133717988,90.7190370573856,116.155904641879));
#42236=CARTESIAN_POINT('Ctrl Pts',(-34.0725465521072,89.669770556873,115.997956118686));
#42237=CARTESIAN_POINT('Ctrl Pts',(-33.5152438301002,86.8967302674414,115.840007595494));
#42238=CARTESIAN_POINT('Ctrl Pts',(-35.5325946342255,84.9141474813107,115.682059072301));
#42239=CARTESIAN_POINT('Ctrl Pts',(-38.2955283453338,85.5195697131357,115.524110549109));
#42240=CARTESIAN_POINT('Ctrl Pts',(-39.2989769983936,88.1640790384055,115.366162025916));
#42241=CARTESIAN_POINT('Ctrl Pts',(-37.6331442181869,90.4499792810135,115.208213502724));
#42242=CARTESIAN_POINT('Ctrl Pts',(-34.8083899225131,90.3047142135001,115.050264979531));
#42243=CARTESIAN_POINT('Ctrl Pts',(-33.3858329202414,87.8599912545425,114.892316456339));
#42244=CARTESIAN_POINT('Ctrl Pts',(-34.6552623802161,85.3323663581397,114.734367933147));
#42245=CARTESIAN_POINT('Ctrl Pts',(-37.4657252190298,85.0135601436239,114.576419409954));
#42246=CARTESIAN_POINT('Ctrl Pts',(-39.2690602570936,87.192624509644,114.418470886762));
#42247=CARTESIAN_POINT('Ctrl Pts',(-38.430238461351,89.8938680687762,114.260522363569));
#42248=CARTESIAN_POINT('Ctrl Pts',(-35.7097940423901,90.6681554405648,114.102573840377));
#42249=CARTESIAN_POINT('Ctrl Pts',(-33.5742712163058,88.8134638138948,113.944625317184));
#42250=CARTESIAN_POINT('Ctrl Pts',(-33.959883580518,86.0113856787719,113.786676793992));
#42251=CARTESIAN_POINT('Ctrl Pts',(-36.5170081322653,84.802480058958,113.628728270799));
#42252=CARTESIAN_POINT('Ctrl Pts',(-38.9271778119062,86.2828249127359,113.470779747607));
#42253=CARTESIAN_POINT('Ctrl Pts',(-39.0051650729075,89.1102365838387,113.312831224414));
#42254=CARTESIAN_POINT('Ctrl Pts',(-36.6802612375947,90.7211869019163,113.154882701222));
#42255=CARTESIAN_POINT('Ctrl Pts',(-34.060385904692,89.655076208407,112.996934178029));
#42256=CARTESIAN_POINT('Ctrl Pts',(-33.5209003586359,86.8785146448246,112.838985654837));
#42257=CARTESIAN_POINT('Ctrl Pts',(-35.5509397363243,84.9089261355665,112.681037131644));
#42258=CARTESIAN_POINT('Ctrl Pts',(-38.3099290748638,85.5320766796504,112.523088608452));
#42259=CARTESIAN_POINT('Ctrl Pts',(-39.2963766518683,88.1829746310225,112.365140085259));
#42260=CARTESIAN_POINT('Ctrl Pts',(-37.6159004507148,90.4581314405903,112.207191562067));
#42261=CARTESIAN_POINT('Ctrl Pts',(-34.7921371336156,90.2947316248854,112.049243038875));
#42262=CARTESIAN_POINT('Ctrl Pts',(-33.385307019306,87.8409248272262,111.891294515682));
#42263=CARTESIAN_POINT('Ctrl Pts',(-34.6709401856254,85.321503041891,111.73334599249));
#42264=CARTESIAN_POINT('Ctrl Pts',(-37.4833921414399,85.0207493768912,111.575397469297));
#42265=CARTESIAN_POINT('Ctrl Pts',(-39.272698235267,87.2113480332777,111.417448946105));
#42266=CARTESIAN_POINT('Ctrl Pts',(-38.4165490511289,89.907149833341,111.259500422912));
#42267=CARTESIAN_POINT('Ctrl Pts',(-35.6911890156619,90.6639532740908,111.10155189972));
#42268=CARTESIAN_POINT('Ctrl Pts',(-33.5676191849894,88.795587692891,110.943603376527));
#42269=CARTESIAN_POINT('Ctrl Pts',(-33.9712157390344,85.9960433385363,110.785654853335));
#42270=CARTESIAN_POINT('Ctrl Pts',(-36.5360499572654,84.8035819326398,110.627706330142));
#42271=CARTESIAN_POINT('Ctrl Pts',(-38.9366646595351,86.2993719652391,110.46975780695));
#42272=CARTESIAN_POINT('Ctrl Pts',(-38.9964955074805,89.1272261053812,110.311809283757));
#42273=CARTESIAN_POINT('Ctrl Pts',(-36.6612956893197,90.7232150111251,110.153860760565));
#42274=CARTESIAN_POINT('Ctrl Pts',(-34.0483198616244,89.6403040780895,109.995912237372));
#42275=CARTESIAN_POINT('Ctrl Pts',(-33.5266737304351,86.8603357209029,109.83796371418));
#42276=CARTESIAN_POINT('Ctrl Pts',(-35.569317991866,84.9038226859369,109.680015190988));
#42277=CARTESIAN_POINT('Ctrl Pts',(-38.3242491892674,85.5446758664894,109.522066667795));
#42278=CARTESIAN_POINT('Ctrl Pts',(-39.2936550530951,88.2018531144783,109.364118144603));
#42279=CARTESIAN_POINT('Ctrl Pts',(-37.5986046470003,90.4661727568194,109.20616962141));
#42280=CARTESIAN_POINT('Ctrl Pts',(-34.775948874024,90.284644786456,109.048221098218));
#42281=CARTESIAN_POINT('Ctrl Pts',(-33.3849033571381,87.8218556145483,108.890272575025));
#42282=CARTESIAN_POINT('Ctrl Pts',(-34.686687827486,85.3107402087474,108.732324051833));
#42283=CARTESIAN_POINT('Ctrl Pts',(-37.5010117020144,85.0280527402971,108.57437552864));
#42284=CARTESIAN_POINT('Ctrl Pts',(-39.276217633105,87.2300928048423,108.416427005448));
#42285=CARTESIAN_POINT('Ctrl Pts',(-38.4027711070691,89.9203469730075,108.258478482255));
#42286=CARTESIAN_POINT('Ctrl Pts',(-35.6726186219733,90.6596244337072,108.100529959063));
#42287=CARTESIAN_POINT('Ctrl Pts',(-33.5610671278939,88.7776842354716,107.94258143587));
#42288=CARTESIAN_POINT('Ctrl Pts',(-33.9826769125213,85.9807432147986,107.784632912678));
#42289=CARTESIAN_POINT('Ctrl Pts',(-36.5550211069366,84.8048695224416,107.626684389486));
#42290=CARTESIAN_POINT('Ctrl Pts',(-38.9461750506382,86.3158490632487,107.468735866293));
#42291=CARTESIAN_POINT('Ctrl Pts',(-38.987449710725,89.144428091839,107.3107873431));
#42292=CARTESIAN_POINT('Ctrl Pts',(-36.6428674306544,90.7245693543756,107.152838819908));
#42293=CARTESIAN_POINT('Ctrl Pts',(-34.0352179374292,89.6266035901596,106.994890296715));
#42294=CARTESIAN_POINT('Ctrl Pts',(-33.5349383123317,86.8398752713272,106.836941773523));
#42295=CARTESIAN_POINT('Ctrl Pts',(-34.9001756782213,85.551559245903,106.731642758061));
#42296=CARTESIAN_POINT('Ctrl Pts',(-35.7047260767084,85.3364687865372,106.678993250331));
#42297=CARTESIAN_POINT('Ctrl Pts',(-34.3005945243415,89.5249809097991,122.10700224989));
#42298=CARTESIAN_POINT('Ctrl Pts',(-33.7195574121284,88.8453944468204,122.054352742159));
#42299=CARTESIAN_POINT('Ctrl Pts',(-33.2951142337176,86.8752722762228,121.949053726697));
#42300=CARTESIAN_POINT('Ctrl Pts',(-35.4324729631248,84.7138976896414,121.791105203505));
#42301=CARTESIAN_POINT('Ctrl Pts',(-38.4073636837697,85.328270422665,121.633156680312));
#42302=CARTESIAN_POINT('Ctrl Pts',(-39.5208314127741,88.1521715901997,121.47520815712));
#42303=CARTESIAN_POINT('Ctrl Pts',(-37.7641356572001,90.6297145644623,121.317259633928));
#42304=CARTESIAN_POINT('Ctrl Pts',(-34.7296229112774,90.5124243092589,121.159311110735));
#42305=CARTESIAN_POINT('Ctrl Pts',(-33.1687861076298,87.9076956980619,121.001362587543));
#42306=CARTESIAN_POINT('Ctrl Pts',(-34.4966948782785,85.176645725828,120.84341406435));
#42307=CARTESIAN_POINT('Ctrl Pts',(-37.5094202542551,84.7956829265805,120.685465541158));
#42308=CARTESIAN_POINT('Ctrl Pts',(-39.4753936270609,87.1100938065847,120.527517017965));
#42309=CARTESIAN_POINT('Ctrl Pts',(-38.6121374968021,90.0215311885463,120.369568494773));
#42310=CARTESIAN_POINT('Ctrl Pts',(-35.7023347075049,90.8902547641484,120.21161997158));
#42311=CARTESIAN_POINT('Ctrl Pts',(-33.3842174959234,88.9286331864827,120.053671448388));
#42312=CARTESIAN_POINT('Ctrl Pts',(-33.7595509977455,85.9152023219081,119.895722925195));
#42313=CARTESIAN_POINT('Ctrl Pts',(-36.4880323439696,84.5821515721737,119.737774402003));
#42314=CARTESIAN_POINT('Ctrl Pts',(-39.0958301883279,86.1381159112078,119.57982587881));
#42315=CARTESIAN_POINT('Ctrl Pts',(-39.2185336802339,89.1723505723458,119.421877355618));
#42316=CARTESIAN_POINT('Ctrl Pts',(-36.7448912262361,90.9338068925739,119.263928832425));
#42317=CARTESIAN_POINT('Ctrl Pts',(-33.9176792405883,89.8254261823407,119.105980309233));
#42318=CARTESIAN_POINT('Ctrl Pts',(-33.3002448285499,86.8521434323996,118.94803178604));
#42319=CARTESIAN_POINT('Ctrl Pts',(-35.4523970010533,84.7097437272575,118.790083262848));
#42320=CARTESIAN_POINT('Ctrl Pts',(-38.4228448341706,85.3406757003008,118.632134739656));
#42321=CARTESIAN_POINT('Ctrl Pts',(-39.5183736215825,88.1728925307714,118.474186216463));
#42322=CARTESIAN_POINT('Ctrl Pts',(-37.7457007298299,90.6385093514682,118.316237693271));
#42323=CARTESIAN_POINT('Ctrl Pts',(-34.7120547569007,90.5020263818399,118.158289170078));
#42324=CARTESIAN_POINT('Ctrl Pts',(-33.1679502420619,87.8871885783255,118.000340646886));
#42325=CARTESIAN_POINT('Ctrl Pts',(-34.5133797872072,85.1647898512491,117.842392123693));
#42326=CARTESIAN_POINT('Ctrl Pts',(-37.5284833430919,84.803146328157,117.684443600501));
#42327=CARTESIAN_POINT('Ctrl Pts',(-39.4795582158498,87.130149192682,117.526495077308));
#42328=CARTESIAN_POINT('Ctrl Pts',(-38.5976241575991,90.0359757200862,117.368546554116));
#42329=CARTESIAN_POINT('Ctrl Pts',(-35.6823039561497,90.8860013747233,117.210598030923));
#42330=CARTESIAN_POINT('Ctrl Pts',(-33.3768297726969,88.9095337478797,117.052649507731));
#42331=CARTESIAN_POINT('Ctrl Pts',(-33.7715049315512,85.8985759252767,116.894700984538));
#42332=CARTESIAN_POINT('Ctrl Pts',(-36.5084894696809,84.5830717905218,116.736752461346));
#42333=CARTESIAN_POINT('Ctrl Pts',(-39.1062427479862,86.1557489333497,116.578803938153));
#42334=CARTESIAN_POINT('Ctrl Pts',(-39.2094608761219,89.1907088191703,116.420855414961));
#42335=CARTESIAN_POINT('Ctrl Pts',(-36.724559116545,90.9362456236433,116.262906891769));
#42336=CARTESIAN_POINT('Ctrl Pts',(-33.9045223197931,89.8097342142547,116.104958368576));
#42337=CARTESIAN_POINT('Ctrl Pts',(-33.306192081939,86.8325482246015,115.947009845384));
#42338=CARTESIAN_POINT('Ctrl Pts',(-35.4720562322533,84.7040116444835,115.789061322191));
#42339=CARTESIAN_POINT('Ctrl Pts',(-38.4383916174267,85.3540038545799,115.631112798999));
#42340=CARTESIAN_POINT('Ctrl Pts',(-39.5157121607349,88.1931966866157,115.473164275806));
#42341=CARTESIAN_POINT('Ctrl Pts',(-37.7272440907837,90.6473803499308,115.315215752614));
#42342=CARTESIAN_POINT('Ctrl Pts',(-34.6945370128002,90.4914211576192,115.157267229421));
#42343=CARTESIAN_POINT('Ctrl Pts',(-33.1672541987757,87.8667225660659,114.999318706229));
#42344=CARTESIAN_POINT('Ctrl Pts',(-34.5301365259792,85.1530189616324,114.841370183036));
#42345=CARTESIAN_POINT('Ctrl Pts',(-37.5475000385275,84.8107428688949,114.683421659844));
#42346=CARTESIAN_POINT('Ctrl Pts',(-39.483593008556,87.1502256112813,114.525473136651));
#42347=CARTESIAN_POINT('Ctrl Pts',(-38.5830188237458,90.0503293384212,114.367524613459));
#42348=CARTESIAN_POINT('Ctrl Pts',(-35.6623007077386,90.8816182035847,114.209576090267));
#42349=CARTESIAN_POINT('Ctrl Pts',(-33.369564946692,88.890387875236,114.051627567074));
#42350=CARTESIAN_POINT('Ctrl Pts',(-33.7835653247409,85.8820263315559,113.893679043881));
#42351=CARTESIAN_POINT('Ctrl Pts',(-36.5289402903607,84.5841234890188,113.735730520689));
#42352=CARTESIAN_POINT('Ctrl Pts',(-39.1165418590291,86.1734483810226,113.577781997497));
#42353=CARTESIAN_POINT('Ctrl Pts',(-39.2002703867787,89.2090084651187,113.419833474304));
#42354=CARTESIAN_POINT('Ctrl Pts',(-36.7042117639871,90.9385537354442,113.261884951112));
#42355=CARTESIAN_POINT('Ctrl Pts',(-33.8914664297479,89.7939580971363,113.103936427919));
#42356=CARTESIAN_POINT('Ctrl Pts',(-33.3122650328336,86.8129916041461,112.945987904727));
#42357=CARTESIAN_POINT('Ctrl Pts',(-35.491751864212,84.6984059136703,112.788039381534));
#42358=CARTESIAN_POINT('Ctrl Pts',(-38.4538524999681,85.3674315590464,112.630090858342));
#42359=CARTESIAN_POINT('Ctrl Pts',(-39.5129203818802,88.2134833351076,112.472142335149));
#42360=CARTESIAN_POINT('Ctrl Pts',(-37.7087308715124,90.6561326552505,112.314193811957));
#42361=CARTESIAN_POINT('Ctrl Pts',(-34.6770877259713,90.4807036707234,112.156245288764));
#42362=CARTESIAN_POINT('Ctrl Pts',(-33.1666895820614,87.8462525063644,111.998296765572));
#42363=CARTESIAN_POINT('Ctrl Pts',(-34.5469685001814,85.1413559096893,111.840348242379));
#42364=CARTESIAN_POINT('Ctrl Pts',(-37.5664675645602,84.8184613591891,111.682399719187));
#42365=CARTESIAN_POINT('Ctrl Pts',(-39.4874988074331,87.1703275234143,111.524451195995));
#42366=CARTESIAN_POINT('Ctrl Pts',(-38.5683216264223,90.0645888800265,111.366502672802));
#42367=CARTESIAN_POINT('Ctrl Pts',(-35.6423260160173,90.8771066819885,111.20855414961));
#42368=CARTESIAN_POINT('Ctrl Pts',(-33.3624232060857,88.8711957498261,111.050605626417));
#42369=CARTESIAN_POINT('Ctrl Pts',(-33.7957317341856,85.8655545188049,110.892657103225));
#42370=CARTESIAN_POINT('Ctrl Pts',(-36.5493839365723,84.5853064804455,110.734708580032));
#42371=CARTESIAN_POINT('Ctrl Pts',(-39.1267271094758,86.1912135945574,110.57676005684));
#42372=CARTESIAN_POINT('Ctrl Pts',(-39.190962585221,89.2272487213821,110.418811533647));
#42373=CARTESIAN_POINT('Ctrl Pts',(-36.683850009841,90.9407311500115,110.260863010455));
#42374=CARTESIAN_POINT('Ctrl Pts',(-33.8785121086339,89.7780984720215,110.102914487262));
#42375=CARTESIAN_POINT('Ctrl Pts',(-33.3184634287599,86.7934743840708,109.94496596407));
#42376=CARTESIAN_POINT('Ctrl Pts',(-35.511483090304,84.6929267582488,109.787017440877));
#42377=CARTESIAN_POINT('Ctrl Pts',(-38.4692268326581,85.380958272914,109.629068917685));
#42378=CARTESIAN_POINT('Ctrl Pts',(-39.5099984244287,88.233751614896,109.471120394493));
#42379=CARTESIAN_POINT('Ctrl Pts',(-37.6901617851941,90.6647659571563,109.3131718713));
#42380=CARTESIAN_POINT('Ctrl Pts',(-34.6597077189672,90.4698742593489,109.155223348108));
#42381=CARTESIAN_POINT('Ctrl Pts',(-33.1662562030891,87.8257794562487,108.997274824915));
#42382=CARTESIAN_POINT('Ctrl Pts',(-34.5638754520551,85.1298007382167,108.839326301723));
#42383=CARTESIAN_POINT('Ctrl Pts',(-37.5853842420734,84.8263023816555,108.68137777853));
#42384=CARTESIAN_POINT('Ctrl Pts',(-39.4912772963268,87.1904522477083,108.523429255338));
#42385=CARTESIAN_POINT('Ctrl Pts',(-38.5535293775764,90.0787575668171,108.365480732145));
#42386=CARTESIAN_POINT('Ctrl Pts',(-35.6223885069509,90.8724591610021,108.207532208953));
#42387=CARTESIAN_POINT('Ctrl Pts',(-33.3553887996033,88.8519742755479,108.04958368576));
#42388=CARTESIAN_POINT('Ctrl Pts',(-33.8080366564257,85.8491280304466,107.891635162568));
#42389=CARTESIAN_POINT('Ctrl Pts',(-36.5697517044782,84.5866888600426,107.733686639375));
#42390=CARTESIAN_POINT('Ctrl Pts',(-39.1369376366204,86.2089037036881,107.575738116183));
#42391=CARTESIAN_POINT('Ctrl Pts',(-39.1812508549341,89.2457170838043,107.41778959299));
#42392=CARTESIAN_POINT('Ctrl Pts',(-36.6640650994951,90.9421851973131,107.259841069798));
#42393=CARTESIAN_POINT('Ctrl Pts',(-33.8644456468879,89.7633893814714,107.101892546605));
#42394=CARTESIAN_POINT('Ctrl Pts',(-33.3273364327067,86.7715076769693,106.943944023413));
#42395=CARTESIAN_POINT('Ctrl Pts',(-34.7930798529405,85.3883483930034,106.838645007951));
#42396=CARTESIAN_POINT('Ctrl Pts',(-35.6568596485225,85.1574234026336,106.78599550022));
#42397=CARTESIAN_POINT('Ctrl Pts',(-34.1597289706644,89.645419027651,122.21400449978));
#42398=CARTESIAN_POINT('Ctrl Pts',(-33.53885013256,88.919233307915,122.161354992049));
#42399=CARTESIAN_POINT('Ctrl Pts',(-33.085302877292,86.8140198224193,122.056055976587));
#42400=CARTESIAN_POINT('Ctrl Pts',(-35.3692203356319,84.5044397391195,121.898107453395));
#42401=CARTESIAN_POINT('Ctrl Pts',(-38.5480993698586,85.160940022191,121.740158930202));
#42402=CARTESIAN_POINT('Ctrl Pts',(-39.7379176023256,88.1784761467643,121.58221040701));
#42403=CARTESIAN_POINT('Ctrl Pts',(-37.8607651852114,90.8259042901323,121.424261883817));
#42404=CARTESIAN_POINT('Ctrl Pts',(-34.6181758422938,90.7005714398875,121.266313360625));
#42405=CARTESIAN_POINT('Ctrl Pts',(-32.9503124291835,87.9172365380294,121.108364837432));
#42406=CARTESIAN_POINT('Ctrl Pts',(-34.3692759296196,84.9989184169933,120.95041631424));
#42407=CARTESIAN_POINT('Ctrl Pts',(-37.5885839422172,84.5918329913191,120.792467791047));
#42408=CARTESIAN_POINT('Ctrl Pts',(-39.6893641467774,87.0649430696068,120.634519267855));
#42409=CARTESIAN_POINT('Ctrl Pts',(-38.7669145271651,90.1760177685039,120.476570744663));
#42410=CARTESIAN_POINT('Ctrl Pts',(-35.6575865049826,91.1043097362912,120.31862222147));
#42411=CARTESIAN_POINT('Ctrl Pts',(-33.1805159518906,89.0081797295473,120.160673698278));
#42412=CARTESIAN_POINT('Ctrl Pts',(-33.5815860791074,85.7881178529846,120.002725175085));
#42413=CARTESIAN_POINT('Ctrl Pts',(-36.497159443399,84.3636597878589,119.844776651893));
#42414=CARTESIAN_POINT('Ctrl Pts',(-39.2837740357949,86.0263166313638,119.6868281287));
#42415=CARTESIAN_POINT('Ctrl Pts',(-39.4148913084864,89.2686088212177,119.528879605508));
#42416=CARTESIAN_POINT('Ctrl Pts',(-36.7716311441325,91.1508482349954,119.370931082315));
#42417=CARTESIAN_POINT('Ctrl Pts',(-33.7505571785846,89.9664658382739,119.212982559123));
#42418=CARTESIAN_POINT('Ctrl Pts',(-33.09078527711,86.789305033333,119.05503403593));
#42419=CARTESIAN_POINT('Ctrl Pts',(-35.3905105652219,84.5000009394557,118.897085512738));
#42420=CARTESIAN_POINT('Ctrl Pts',(-38.5646420630384,85.1741959299512,118.739136989545));
#42421=CARTESIAN_POINT('Ctrl Pts',(-39.735291280345,88.2006179226272,118.581188466353));
#42422=CARTESIAN_POINT('Ctrl Pts',(-37.8410661745189,90.8353021358514,118.42323994316));
#42423=CARTESIAN_POINT('Ctrl Pts',(-34.5994030392356,90.6894605263865,118.265291419968));
#42424=CARTESIAN_POINT('Ctrl Pts',(-32.9494192482977,87.8953232447007,118.107342896775));
#42425=CARTESIAN_POINT('Ctrl Pts',(-34.3871049230724,84.9862495848679,117.949394373583));
#42426=CARTESIAN_POINT('Ctrl Pts',(-37.6089541874201,84.5998081584843,117.791445850391));
#42427=CARTESIAN_POINT('Ctrl Pts',(-39.6938143014992,87.0863736539122,117.633497327198));
#42428=CARTESIAN_POINT('Ctrl Pts',(-38.7514060080155,90.1914527618476,117.475548804006));
#42429=CARTESIAN_POINT('Ctrl Pts',(-35.6361822446241,91.0997646918721,117.317600280813));
#42430=CARTESIAN_POINT('Ctrl Pts',(-33.1726216523412,88.9877706420741,117.159651757621));
#42431=CARTESIAN_POINT('Ctrl Pts',(-33.5943596943826,85.7703513840185,117.001703234428));
#42432=CARTESIAN_POINT('Ctrl Pts',(-36.5190193146114,84.3646431055967,116.843754711236));
#42433=CARTESIAN_POINT('Ctrl Pts',(-39.294900584868,86.0451587501709,116.685806188043));
#42434=CARTESIAN_POINT('Ctrl Pts',(-39.4051963820231,89.2882258933781,116.527857664851));
#42435=CARTESIAN_POINT('Ctrl Pts',(-36.7499048612913,91.1534541899008,116.369909141658));
#42436=CARTESIAN_POINT('Ctrl Pts',(-33.736498087479,89.9496978716363,116.211960618466));
#42437=CARTESIAN_POINT('Ctrl Pts',(-33.0971403337776,86.7683661817615,116.054012095273));
#42438=CARTESIAN_POINT('Ctrl Pts',(-35.4115178302812,84.4938758076564,115.896063572081));
#42439=CARTESIAN_POINT('Ctrl Pts',(-38.5812548895196,85.1884379960241,115.738115048888));
#42440=CARTESIAN_POINT('Ctrl Pts',(-39.7324473230763,88.2223143348259,115.580166525696));
#42441=CARTESIAN_POINT('Ctrl Pts',(-37.8213439633806,90.844781418848,115.422218002504));
#42442=CARTESIAN_POINT('Ctrl Pts',(-34.5806841030873,90.6781281017385,115.264269479311));
#42443=CARTESIAN_POINT('Ctrl Pts',(-32.94867547731,87.873453877589,115.106320956119));
#42444=CARTESIAN_POINT('Ctrl Pts',(-34.4050106717424,84.9736715651254,114.948372432926));
#42445=CARTESIAN_POINT('Ctrl Pts',(-37.6292748580252,84.6079255941658,114.790423909734));
#42446=CARTESIAN_POINT('Ctrl Pts',(-39.6981257600185,87.1078267129187,114.632475386541));
#42447=CARTESIAN_POINT('Ctrl Pts',(-38.7357991861407,90.2067906080661,114.474526863349));
#42448=CARTESIAN_POINT('Ctrl Pts',(-35.6148073730872,91.0950809666047,114.316578340156));
#42449=CARTESIAN_POINT('Ctrl Pts',(-33.1648586770783,88.9673119365771,114.158629816964));
#42450=CARTESIAN_POINT('Ctrl Pts',(-33.6072470689639,85.7526669843399,114.000681293771));
#42451=CARTESIAN_POINT('Ctrl Pts',(-36.5408724484561,84.3657669190797,113.842732770579));
#42452=CARTESIAN_POINT('Ctrl Pts',(-39.3059059061521,86.0640718493091,113.684784247386));
#42453=CARTESIAN_POINT('Ctrl Pts',(-39.39537570065,89.307780346399,113.526835724194));
#42454=CARTESIAN_POINT('Ctrl Pts',(-36.7281622903795,91.155920568972,113.368887201001));
#42455=CARTESIAN_POINT('Ctrl Pts',(-33.7225469548038,89.9328399858657,113.210938677809));
#42456=CARTESIAN_POINT('Ctrl Pts',(-33.1036297070312,86.7474685634676,113.052990154616));
#42457=CARTESIAN_POINT('Ctrl Pts',(-35.4325639920998,84.4878856917742,112.895041631424));
#42458=CARTESIAN_POINT('Ctrl Pts',(-38.5977759250725,85.2027864384426,112.737093108232));
#42459=CARTESIAN_POINT('Ctrl Pts',(-39.7294641118921,88.2439920391926,112.579144585039));
#42460=CARTESIAN_POINT('Ctrl Pts',(-37.8015612923099,90.8541338699109,112.421196061847));
#42461=CARTESIAN_POINT('Ctrl Pts',(-34.562038318327,90.6666757165611,112.263247538654));
#42462=CARTESIAN_POINT('Ctrl Pts',(-32.9480721448167,87.8515801855026,112.105299015462));
#42463=CARTESIAN_POINT('Ctrl Pts',(-34.4229968147373,84.9612087774874,111.947350492269));
#42464=CARTESIAN_POINT('Ctrl Pts',(-37.6495429876806,84.616173341487,111.789401969077));
#42465=CARTESIAN_POINT('Ctrl Pts',(-39.7022993795991,87.1293070135509,111.631453445884));
#42466=CARTESIAN_POINT('Ctrl Pts',(-38.7200942017158,90.2220279267117,111.473504922692));
#42467=CARTESIAN_POINT('Ctrl Pts',(-35.5934630163727,91.0902600898865,111.315556399499));
#42468=CARTESIAN_POINT('Ctrl Pts',(-33.157227227182,88.9468038067609,111.157607876307));
#42469=CARTESIAN_POINT('Ctrl Pts',(-33.6202477293367,85.7350656990739,110.999659353114));
#42470=CARTESIAN_POINT('Ctrl Pts',(-36.5627179158792,84.3670310282509,110.841710829922));
#42471=CARTESIAN_POINT('Ctrl Pts',(-39.3167895594165,86.0830552238758,110.683762306729));
#42472=CARTESIAN_POINT('Ctrl Pts',(-39.3854296629615,89.3272713373828,110.525813783537));
#42473=CARTESIAN_POINT('Ctrl Pts',(-36.7064043303624,91.1582472888979,110.367865260345));
#42474=CARTESIAN_POINT('Ctrl Pts',(-33.7087043556433,89.9158928659535,110.209916737152));
#42475=CARTESIAN_POINT('Ctrl Pts',(-33.1102531270847,86.7266130472388,110.05196821396));
#42476=CARTESIAN_POINT('Ctrl Pts',(-35.4536481887421,84.4820308305605,109.894019690767));
#42477=CARTESIAN_POINT('Ctrl Pts',(-38.6142044760489,85.2172406793387,109.736071167575));
#42478=CARTESIAN_POINT('Ctrl Pts',(-39.7263417957622,88.2656501153136,109.578122644382));
#42479=CARTESIAN_POINT('Ctrl Pts',(-37.7817189233878,90.8633591574933,109.42017412119));
#42480=CARTESIAN_POINT('Ctrl Pts',(-34.5434665639104,90.6551037322417,109.262225597997));
#42481=CARTESIAN_POINT('Ctrl Pts',(-32.9476090490401,87.8297032979492,109.104277074805));
#42482=CARTESIAN_POINT('Ctrl Pts',(-34.4410630766242,84.948861267686,108.946328551612));
#42483=CARTESIAN_POINT('Ctrl Pts',(-37.6697567821324,84.6245520230139,108.78838002842));
#42484=CARTESIAN_POINT('Ctrl Pts',(-39.7063369595486,87.1508116905743,108.630431505227));
#42485=CARTESIAN_POINT('Ctrl Pts',(-38.7042876480837,90.2371681606266,108.472482982035));
#42486=CARTESIAN_POINT('Ctrl Pts',(-35.5721583919285,91.0852938882971,108.314534458842));
#42487=CARTESIAN_POINT('Ctrl Pts',(-33.1497104713126,88.9262643156241,108.15658593565));
#42488=CARTESIAN_POINT('Ctrl Pts',(-33.6333964003301,85.7175128460946,107.998637412458));
#42489=CARTESIAN_POINT('Ctrl Pts',(-36.5844823020197,84.3685081976436,107.840688889265));
#42490=CARTESIAN_POINT('Ctrl Pts',(-39.3277002226027,86.1019583441278,107.682740366073));
#42491=CARTESIAN_POINT('Ctrl Pts',(-39.3750519991432,89.3470060757694,107.52479184288));
#42492=CARTESIAN_POINT('Ctrl Pts',(-36.6852627683359,91.1598010402508,107.366843319688));
#42493=CARTESIAN_POINT('Ctrl Pts',(-33.6936733563466,89.9001751727833,107.208894796495));
#42494=CARTESIAN_POINT('Ctrl Pts',(-33.1197345530817,86.7031400826113,107.050946273303));
#42495=CARTESIAN_POINT('Ctrl Pts',(-34.6859840276597,85.2251375401038,106.945647257841));
#42496=CARTESIAN_POINT('Ctrl Pts',(-35.6089932203365,84.9783780187301,106.89299775011));
#42497=CARTESIAN_POINT('Ctrl Pts',(-34.0188634169874,89.7658571455029,122.321006749669));
#42498=CARTESIAN_POINT('Ctrl Pts',(-33.3581428529915,88.9930721690097,122.268357241939));
#42499=CARTESIAN_POINT('Ctrl Pts',(-32.8754915208664,86.7527673686156,122.163058226477));
#42500=CARTESIAN_POINT('Ctrl Pts',(-35.3059677081389,84.2949817885978,122.005109703285));
#42501=CARTESIAN_POINT('Ctrl Pts',(-38.6888350559476,84.9936096217169,121.847161180092));
#42502=CARTESIAN_POINT('Ctrl Pts',(-39.9550037918771,88.204780703329,121.6892126569));
#42503=CARTESIAN_POINT('Ctrl Pts',(-37.9573947132227,91.0220940158023,121.531264133707));
#42504=CARTESIAN_POINT('Ctrl Pts',(-34.5067287733102,90.8887185705161,121.373315610515));
#42505=CARTESIAN_POINT('Ctrl Pts',(-32.7318387507372,87.9267773779968,121.215367087322));
#42506=CARTESIAN_POINT('Ctrl Pts',(-34.2418569809606,84.8211911081587,121.05741856413));
#42507=CARTESIAN_POINT('Ctrl Pts',(-37.6677476301795,84.3879830560575,120.899470040937));
#42508=CARTESIAN_POINT('Ctrl Pts',(-39.903334666494,87.019792332629,120.741521517745));
#42509=CARTESIAN_POINT('Ctrl Pts',(-38.921691557528,90.3305043484613,120.583572994552));
#42510=CARTESIAN_POINT('Ctrl Pts',(-35.6128383024604,91.3183647084341,120.42562447136));
#42511=CARTESIAN_POINT('Ctrl Pts',(-32.9768144078577,89.0877262726116,120.267675948167));
#42512=CARTESIAN_POINT('Ctrl Pts',(-33.4036211604692,85.6610333840612,120.109727424975));
#42513=CARTESIAN_POINT('Ctrl Pts',(-36.5062865428284,84.1451680035439,119.951778901782));
#42514=CARTESIAN_POINT('Ctrl Pts',(-39.4717178832619,85.9145173515199,119.79383037859));
#42515=CARTESIAN_POINT('Ctrl Pts',(-39.611248936739,89.3648670700897,119.635881855398));
#42516=CARTESIAN_POINT('Ctrl Pts',(-36.7983710620289,91.3678895774169,119.477933332205));
#42517=CARTESIAN_POINT('Ctrl Pts',(-33.583435116581,90.1075054942073,119.319984809013));
#42518=CARTESIAN_POINT('Ctrl Pts',(-32.8813257256701,86.7264666342663,119.16203628582));
#42519=CARTESIAN_POINT('Ctrl Pts',(-35.3286241293906,84.2902581516539,119.004087762628));
#42520=CARTESIAN_POINT('Ctrl Pts',(-38.7064392919062,85.0077161596018,118.846139239435));
#42521=CARTESIAN_POINT('Ctrl Pts',(-39.9522089391075,88.2283433144829,118.688190716243));
#42522=CARTESIAN_POINT('Ctrl Pts',(-37.936431619208,91.0320949202345,118.53024219305));
#42523=CARTESIAN_POINT('Ctrl Pts',(-34.4867513215705,90.8768946709331,118.372293669858));
#42524=CARTESIAN_POINT('Ctrl Pts',(-32.7308882545334,87.903457911076,118.214345146665));
#42525=CARTESIAN_POINT('Ctrl Pts',(-34.2608300589376,84.8077093184867,118.056396623473));
#42526=CARTESIAN_POINT('Ctrl Pts',(-37.6894250317483,84.3964699888117,117.89844810028));
#42527=CARTESIAN_POINT('Ctrl Pts',(-39.9080703871487,87.0425981151423,117.740499577088));
#42528=CARTESIAN_POINT('Ctrl Pts',(-38.9051878584318,90.346929803609,117.582551053895));
#42529=CARTESIAN_POINT('Ctrl Pts',(-35.5900605330986,91.3135280090206,117.424602530703));
#42530=CARTESIAN_POINT('Ctrl Pts',(-32.9684135319854,89.0660075362686,117.26665400751));
#42531=CARTESIAN_POINT('Ctrl Pts',(-33.417214457214,85.6421268427602,117.108705484318));
#42532=CARTESIAN_POINT('Ctrl Pts',(-36.5295491595418,84.1462144206715,116.950756961126));
#42533=CARTESIAN_POINT('Ctrl Pts',(-39.4835584217499,85.9345685669924,116.792808437933));
#42534=CARTESIAN_POINT('Ctrl Pts',(-39.6009318879243,89.3857429675857,116.634859914741));
#42535=CARTESIAN_POINT('Ctrl Pts',(-36.7752506060375,91.3706627561583,116.476911391548));
#42536=CARTESIAN_POINT('Ctrl Pts',(-33.5684738551649,90.0896615290181,116.318962868356));
#42537=CARTESIAN_POINT('Ctrl Pts',(-32.8880885856163,86.7041841389216,116.161014345163));
#42538=CARTESIAN_POINT('Ctrl Pts',(-35.3509794283091,84.2837399708291,116.003065821971));
#42539=CARTESIAN_POINT('Ctrl Pts',(-38.7241181616125,85.0228721374683,115.845117298778));
#42540=CARTESIAN_POINT('Ctrl Pts',(-39.9491824854176,88.251431983036,115.687168775586));
#42541=CARTESIAN_POINT('Ctrl Pts',(-37.9154438359774,91.0421824877652,115.529220252393));
#42542=CARTESIAN_POINT('Ctrl Pts',(-34.4668311933744,90.8648350458576,115.371271729201));
#42543=CARTESIAN_POINT('Ctrl Pts',(-32.7300967558443,87.8801851891123,115.213323206008));
#42544=CARTESIAN_POINT('Ctrl Pts',(-34.2798848175055,84.7943241686182,115.055374682816));
#42545=CARTESIAN_POINT('Ctrl Pts',(-37.7110496775229,84.4051083194366,114.897426159624));
#42546=CARTESIAN_POINT('Ctrl Pts',(-39.9126585114809,87.065427814556,114.739477636431));
#42547=CARTESIAN_POINT('Ctrl Pts',(-38.8885795485355,90.3632518777111,114.581529113238));
#42548=CARTESIAN_POINT('Ctrl Pts',(-35.5673140384357,91.3085437296246,114.423580590046));
#42549=CARTESIAN_POINT('Ctrl Pts',(-32.9601524074645,89.0442359979183,114.265632066854));
#42550=CARTESIAN_POINT('Ctrl Pts',(-33.4309288131869,85.623307637124,114.107683543661));
#42551=CARTESIAN_POINT('Ctrl Pts',(-36.5528046065515,84.1474103491404,113.949735020469));
#42552=CARTESIAN_POINT('Ctrl Pts',(-39.495269953275,85.9546953175959,113.791786497276));
#42553=CARTESIAN_POINT('Ctrl Pts',(-39.5904810145212,89.406552227679,113.633837974084));
#42554=CARTESIAN_POINT('Ctrl Pts',(-36.7521128167719,91.3732874025,113.475889450891));
#42555=CARTESIAN_POINT('Ctrl Pts',(-33.5536274798598,90.071721874595,113.317940927699));
#42556=CARTESIAN_POINT('Ctrl Pts',(-32.8949943812288,86.6819455227893,113.159992404506));
#42557=CARTESIAN_POINT('Ctrl Pts',(-35.3733761199876,84.2773654698779,113.002043881314));
#42558=CARTESIAN_POINT('Ctrl Pts',(-38.7416993501767,85.0381413178388,112.844095358121));
#42559=CARTESIAN_POINT('Ctrl Pts',(-39.946007841904,88.2745007432776,112.686146834929));
#42560=CARTESIAN_POINT('Ctrl Pts',(-37.8943917131075,91.0521350845713,112.528198311736));
#42561=CARTESIAN_POINT('Ctrl Pts',(-34.4469889106826,90.8526477623989,112.370249788544));
#42562=CARTESIAN_POINT('Ctrl Pts',(-32.7294547075721,87.8569078646409,112.212301265352));
#42563=CARTESIAN_POINT('Ctrl Pts',(-34.2990251292932,84.7810616452854,112.054352742159));
#42564=CARTESIAN_POINT('Ctrl Pts',(-37.732618410801,84.413885323785,111.896404218967));
#42565=CARTESIAN_POINT('Ctrl Pts',(-39.9170999517652,87.0882865036874,111.738455695774));
#42566=CARTESIAN_POINT('Ctrl Pts',(-38.8718667770092,90.3794669733972,111.580507172582));
#42567=CARTESIAN_POINT('Ctrl Pts',(-35.544600016728,91.3034134977843,111.422558649389));
#42568=CARTESIAN_POINT('Ctrl Pts',(-32.9520312482784,89.0224118636959,111.264610126197));
#42569=CARTESIAN_POINT('Ctrl Pts',(-33.4447637244879,85.6045768793427,111.106661603004));
#42570=CARTESIAN_POINT('Ctrl Pts',(-36.5760518951862,84.1487555760565,110.948713079812));
#42571=CARTESIAN_POINT('Ctrl Pts',(-39.5068520093573,85.9748968531942,110.790764556619));
#42572=CARTESIAN_POINT('Ctrl Pts',(-39.579896740702,89.4272939533835,110.632816033427));
#42573=CARTESIAN_POINT('Ctrl Pts',(-36.7289586508838,91.3757634277843,110.474867510234));
#42574=CARTESIAN_POINT('Ctrl Pts',(-33.5388966026528,90.0536872598855,110.316918987042));
#42575=CARTESIAN_POINT('Ctrl Pts',(-32.9020428254094,86.6597517104068,110.158970463849));
#42576=CARTESIAN_POINT('Ctrl Pts',(-35.3958132871802,84.2711349028723,110.001021940657));
#42577=CARTESIAN_POINT('Ctrl Pts',(-38.7591821194396,85.0535230857633,109.843073417464));
#42578=CARTESIAN_POINT('Ctrl Pts',(-39.9426851670958,88.2975486157311,109.685124894272));
#42579=CARTESIAN_POINT('Ctrl Pts',(-37.8732760615816,91.0619523578304,109.527176371079));
#42580=CARTESIAN_POINT('Ctrl Pts',(-34.4272254088536,90.8403332051346,109.369227847887));
#42581=CARTESIAN_POINT('Ctrl Pts',(-32.7289618949911,87.8336271396496,109.211279324695));
#42582=CARTESIAN_POINT('Ctrl Pts',(-34.3182507011933,84.7679217971554,109.053330801502));
#42583=CARTESIAN_POINT('Ctrl Pts',(-37.7541293221915,84.4228016643723,108.89538227831));
#42584=CARTESIAN_POINT('Ctrl Pts',(-39.9213966227703,87.1111711334404,108.737433755117));
#42585=CARTESIAN_POINT('Ctrl Pts',(-38.855045918591,90.3955787544361,108.579485231925));
#42586=CARTESIAN_POINT('Ctrl Pts',(-35.521928276906,91.298128615592,108.421536708732));
#42587=CARTESIAN_POINT('Ctrl Pts',(-32.944032143022,89.0005543557004,108.26358818554));
#42588=CARTESIAN_POINT('Ctrl Pts',(-33.4587561442345,85.5858976617427,108.105639662347));
#42589=CARTESIAN_POINT('Ctrl Pts',(-36.5992128995613,84.1503275352445,107.947691139155));
#42590=CARTESIAN_POINT('Ctrl Pts',(-39.5184628085849,85.9950129845674,107.789742615962));
#42591=CARTESIAN_POINT('Ctrl Pts',(-39.5688531433523,89.4482950677345,107.63179409277));
#42592=CARTESIAN_POINT('Ctrl Pts',(-36.7064604371766,91.3774168831885,107.473845569577));
#42593=CARTESIAN_POINT('Ctrl Pts',(-33.5229010658053,90.036960964095,107.315897046385));
#42594=CARTESIAN_POINT('Ctrl Pts',(-32.9121326734567,86.6347724882534,107.157948523192));
#42595=CARTESIAN_POINT('Ctrl Pts',(-34.578888202379,85.0619266872042,107.052649507731));
#42596=CARTESIAN_POINT('Ctrl Pts',(-35.5611267921506,84.7993326348266,107.));
#42597=CARTESIAN_POINT('Ctrl Pts',(-34.4414600780185,89.4045427919472,122.));
#42598=CARTESIAN_POINT('Ctrl Pts',(-34.3798518540623,89.3466461894736,122.));
#42599=CARTESIAN_POINT('Ctrl Pts',(-34.3216127823397,89.2855988291107,122.));
#42600=CARTESIAN_POINT('Ctrl Pts',(-34.2667404771132,89.2217855293614,122.));
#42601=CARTESIAN_POINT('Ctrl Pts',(-34.2104152444954,89.1562825595543,122.));
#42602=CARTESIAN_POINT('Ctrl Pts',(-34.1576369947234,89.0878648044825,122.));
#42603=CARTESIAN_POINT('Ctrl Pts',(-34.1084286552735,89.0168999163865,122.));
#42604=CARTESIAN_POINT('Ctrl Pts',(-34.057870758409,88.9439887892591,122.));
#42605=CARTESIAN_POINT('Ctrl Pts',(-34.0110807367076,88.86838834465,122.));
#42606=CARTESIAN_POINT('Ctrl Pts',(-33.9681175240201,88.7904543421215,122.));
#42607=CARTESIAN_POINT('Ctrl Pts',(-33.9492075685674,88.7561522398373,122.));
#42608=CARTESIAN_POINT('Ctrl Pts',(-33.9310394493789,88.7213975690564,122.));
#42609=CARTESIAN_POINT('Ctrl Pts',(-33.9136206166358,88.6862185871068,122.));
#42610=CARTESIAN_POINT('Ctrl Pts',(-33.9036897724251,88.6661623069653,122.));
#42611=CARTESIAN_POINT('Ctrl Pts',(-33.8940025031947,88.6459680887744,122.));
#42612=CARTESIAN_POINT('Ctrl Pts',(-33.8845604238774,88.6256410205665,122.));
#42613=CARTESIAN_POINT('Ctrl Pts',(-33.8760548331441,88.6073300408371,122.));
#42614=CARTESIAN_POINT('Ctrl Pts',(-33.8677458327171,88.5889055291902,122.));
#42615=CARTESIAN_POINT('Ctrl Pts',(-33.8596482636109,88.5704029596064,122.));
#42616=CARTESIAN_POINT('Ctrl Pts',(-33.8230866066973,88.4868612704561,122.));
#42617=CARTESIAN_POINT('Ctrl Pts',(-33.7907851307286,88.4016360383248,122.));
#42618=CARTESIAN_POINT('Ctrl Pts',(-33.7627688719189,88.3151260404377,122.));
#42619=CARTESIAN_POINT('Ctrl Pts',(-33.7342895213475,88.227186084768,122.));
#42620=CARTESIAN_POINT('Ctrl Pts',(-33.7102377294814,88.1379177844905,122.));
#42621=CARTESIAN_POINT('Ctrl Pts',(-33.6906788696645,88.0477028957553,122.));
#42622=CARTESIAN_POINT('Ctrl Pts',(-33.6717103782297,87.9602110705522,122.));
#42623=CARTESIAN_POINT('Ctrl Pts',(-33.6569675246869,87.8718280211553,122.));
#42624=CARTESIAN_POINT('Ctrl Pts',(-33.6465506821664,87.7828801024266,122.));
#42625=CARTESIAN_POINT('Ctrl Pts',(-33.6421818440549,87.7455752227077,122.));
#42626=CARTESIAN_POINT('Ctrl Pts',(-33.638574456279,87.7081707917553,122.));
#42627=CARTESIAN_POINT('Ctrl Pts',(-33.6357382583831,87.6706902671327,122.));
#42628=CARTESIAN_POINT('Ctrl Pts',(-33.6339591268603,87.6471789377781,122.));
#42629=CARTESIAN_POINT('Ctrl Pts',(-33.6324834856474,87.6236376602105,122.));
#42630=CARTESIAN_POINT('Ctrl Pts',(-33.6313140348496,87.6000721918068,122.));
#42631=CARTESIAN_POINT('Ctrl Pts',(-33.6306296486946,87.5862812051798,122.));
#42632=CARTESIAN_POINT('Ctrl Pts',(-33.630050417326,87.5724868801265,122.));
#42633=CARTESIAN_POINT('Ctrl Pts',(-33.6295768415433,87.5586982075279,122.));
#42634=CARTESIAN_POINT('Ctrl Pts',(-33.6262494419034,87.461817357796,122.));
#42635=CARTESIAN_POINT('Ctrl Pts',(-33.6281279592553,87.3651015105385,122.));
#42636=CARTESIAN_POINT('Ctrl Pts',(-33.6352767760794,87.268970431256,122.));
#42637=CARTESIAN_POINT('Ctrl Pts',(-33.6424255929035,87.1728393519736,122.));
#42638=CARTESIAN_POINT('Ctrl Pts',(-33.6548442788849,87.0772919966335,122.));
#42639=CARTESIAN_POINT('Ctrl Pts',(-33.6726496794354,86.9827293452592,122.));
#42640=CARTESIAN_POINT('Ctrl Pts',(-33.6897076975519,86.8921359651379,122.));
#42641=CARTESIAN_POINT('Ctrl Pts',(-33.7117095737827,86.8024453892223,122.));
#42642=CARTESIAN_POINT('Ctrl Pts',(-33.738380698432,86.7138969574772,122.));
#42643=CARTESIAN_POINT('Ctrl Pts',(-33.7472500404817,86.684450642804,122.));
#42644=CARTESIAN_POINT('Ctrl Pts',(-33.756636166633,86.6551306692652,122.));
#42645=CARTESIAN_POINT('Ctrl Pts',(-33.7665302267902,86.6259460129984,122.));
#42646=CARTESIAN_POINT('Ctrl Pts',(-33.7758505040486,86.598453852674,122.));
#42647=CARTESIAN_POINT('Ctrl Pts',(-33.7856215168716,86.5710817688634,122.));
#42648=CARTESIAN_POINT('Ctrl Pts',(-33.7958363420113,86.5438373897669,122.));
#42649=CARTESIAN_POINT('Ctrl Pts',(-33.8009941567469,86.5300807705352,122.));
#42650=CARTESIAN_POINT('Ctrl Pts',(-33.8062620516302,86.5163649848821,122.));
#42651=CARTESIAN_POINT('Ctrl Pts',(-33.8116373565419,86.5026943515934,122.));
#42652=CARTESIAN_POINT('Ctrl Pts',(-33.845888676196,86.4155853897129,122.));
#42653=CARTESIAN_POINT('Ctrl Pts',(-33.8845134961369,86.3302652389299,122.));
#42654=CARTESIAN_POINT('Ctrl Pts',(-33.927181830165,86.2469683145023,122.));
#42655=CARTESIAN_POINT('Ctrl Pts',(-33.9714116396017,86.1606230850008,122.));
#42656=CARTESIAN_POINT('Ctrl Pts',(-34.0199864581995,86.076451143434,122.));
#42657=CARTESIAN_POINT('Ctrl Pts',(-34.0725945744941,85.9947170694416,122.));
#42658=CARTESIAN_POINT('Ctrl Pts',(-34.1257656479925,85.9121083626172,122.));
#42659=CARTESIAN_POINT('Ctrl Pts',(-34.1830572163906,85.8319891559087,122.));
#42660=CARTESIAN_POINT('Ctrl Pts',(-34.2441989619735,85.7546479784666,122.));
#42661=CARTESIAN_POINT('Ctrl Pts',(-34.2668877934898,85.7259477683643,122.));
#42662=CARTESIAN_POINT('Ctrl Pts',(-34.2901072857831,85.697630319848,122.));
#42663=CARTESIAN_POINT('Ctrl Pts',(-34.3138452200131,85.6697112650143,122.));
#42664=CARTESIAN_POINT('Ctrl Pts',(-34.3346002693604,85.645300490463,122.));
#42665=CARTESIAN_POINT('Ctrl Pts',(-34.3557516672241,85.6211942822015,122.));
#42666=CARTESIAN_POINT('Ctrl Pts',(-34.3772917361037,85.5974034716814,122.));
#42667=CARTESIAN_POINT('Ctrl Pts',(-34.3890554697408,85.5844105346794,122.));
#42668=CARTESIAN_POINT('Ctrl Pts',(-34.4009304534246,85.5715169185705,122.));
#42669=CARTESIAN_POINT('Ctrl Pts',(-34.4129093606097,85.5587302471734,122.));
#42670=CARTESIAN_POINT('Ctrl Pts',(-34.4819201604098,85.4850658964735,122.));
#42671=CARTESIAN_POINT('Ctrl Pts',(-34.554433357923,85.4148860760258,122.));
#42672=CARTESIAN_POINT('Ctrl Pts',(-34.6301404311514,85.3484820008986,122.));
#42673=CARTESIAN_POINT('Ctrl Pts',(-34.6923345902646,85.2939303528409,122.));
#42674=CARTESIAN_POINT('Ctrl Pts',(-34.7566853223865,85.2419269392842,122.));
#42675=CARTESIAN_POINT('Ctrl Pts',(-34.8230438595686,85.1926465506592,122.));
#42676=CARTESIAN_POINT('Ctrl Pts',(-34.8476613986356,85.1743646242677,122.));
#42677=CARTESIAN_POINT('Ctrl Pts',(-34.8725554416842,85.1564575983159,122.));
#42678=CARTESIAN_POINT('Ctrl Pts',(-34.8977190002205,85.1389349616694,122.));
#42679=CARTESIAN_POINT('Ctrl Pts',(-34.9145299551421,85.1272286581135,122.));
#42680=CARTESIAN_POINT('Ctrl Pts',(-34.9314623353314,85.1156932828469,122.));
#42681=CARTESIAN_POINT('Ctrl Pts',(-34.9484989961695,85.1043414885822,122.));
#42682=CARTESIAN_POINT('Ctrl Pts',(-35.033409495634,85.0477642913257,122.));
#42683=CARTESIAN_POINT('Ctrl Pts',(-35.1209892714876,84.995686394659,122.));
#42684=CARTESIAN_POINT('Ctrl Pts',(-35.2109479651256,84.9484157153952,122.));
#42685=CARTESIAN_POINT('Ctrl Pts',(-35.2944060214804,84.904560932112,122.));
#42686=CARTESIAN_POINT('Ctrl Pts',(-35.3799124172306,84.8648434346886,122.));
#42687=CARTESIAN_POINT('Ctrl Pts',(-35.4672630109208,84.8295381485711,122.));
#42688=CARTESIAN_POINT('Ctrl Pts',(-35.4976931912937,84.8172389050366,122.));
#42689=CARTESIAN_POINT('Ctrl Pts',(-35.5283473918442,84.8054754204773,122.));
#42690=CARTESIAN_POINT('Ctrl Pts',(-35.5592127063051,84.7942439724069,122.));
#42691=CARTESIAN_POINT('Ctrl Pts',(-38.8730930351581,87.7663573574127,120.387416697508));
#42692=CARTESIAN_POINT('Ctrl Pts',(-38.8746753948415,87.5919909412047,120.398449387697));
#42693=CARTESIAN_POINT('Ctrl Pts',(-38.8580898013711,87.4179235704137,120.409482077886));
#42694=CARTESIAN_POINT('Ctrl Pts',(-38.8222182436848,87.2479259407801,120.420514768075));
#42695=CARTESIAN_POINT('Ctrl Pts',(-38.6510342603271,86.436673982989,120.473164275806));
#42696=CARTESIAN_POINT('Ctrl Pts',(-38.04064541331,85.7181034224155,120.525813783537));
#42697=CARTESIAN_POINT('Ctrl Pts',(-37.2677605332422,85.4179581709321,120.578463291268));
#42698=CARTESIAN_POINT('Ctrl Pts',(-36.4948756531744,85.1178129194488,120.631112798999));
#42699=CARTESIAN_POINT('Ctrl Pts',(-35.5594947400559,85.2360929770557,120.683762306729));
#42700=CARTESIAN_POINT('Ctrl Pts',(-34.8856619433531,85.7191966430978,120.73641181446));
#42701=CARTESIAN_POINT('Ctrl Pts',(-34.2118291466503,86.2023003091399,120.789061322191));
#42702=CARTESIAN_POINT('Ctrl Pts',(-33.7995444663632,87.0502275836171,120.841710829922));
#42703=CARTESIAN_POINT('Ctrl Pts',(-33.8357038252505,87.8785449409451,120.894360337653));
#42704=CARTESIAN_POINT('Ctrl Pts',(-33.8718631841377,88.7068622982731,120.947009845384));
#42705=CARTESIAN_POINT('Ctrl Pts',(-34.3564665821994,89.5155697384517,120.999659353114));
#42706=CARTESIAN_POINT('Ctrl Pts',(-35.0698409727182,89.9381314019014,121.052308860845));
#42707=CARTESIAN_POINT('Ctrl Pts',(-35.783215363237,90.360693065351,121.104958368576));
#42708=CARTESIAN_POINT('Ctrl Pts',(-36.725360746213,90.3971089520717,121.157607876307));
#42709=CARTESIAN_POINT('Ctrl Pts',(-37.4691399533732,90.0307072612391,121.210257384038));
#42710=CARTESIAN_POINT('Ctrl Pts',(-38.2129191605335,89.6643055704066,121.262906891768));
#42711=CARTESIAN_POINT('Ctrl Pts',(-38.758332191878,88.8950863020207,121.315556399499));
#42712=CARTESIAN_POINT('Ctrl Pts',(-38.8581858366267,88.0720989660786,121.36820590723));
#42713=CARTESIAN_POINT('Ctrl Pts',(-38.8703307265502,87.9720015622371,121.374609503989));
#42714=CARTESIAN_POINT('Ctrl Pts',(-38.8758844099473,87.8711087617585,121.381013100749));
#42715=CARTESIAN_POINT('Ctrl Pts',(-38.8751286390733,87.7701344517389,121.387416697508));
#42716=CARTESIAN_POINT('Ctrl Pts',(-37.1487253572165,84.7993326348266,122.));
#42717=CARTESIAN_POINT('Ctrl Pts',(-38.1309639469882,85.0619266872043,121.947350492269));
#42718=CARTESIAN_POINT('Ctrl Pts',(-39.7977194028581,86.634772993702,121.842051476808));
#42719=CARTESIAN_POINT('Ctrl Pts',(-39.186951146607,90.036960832952,121.684102953615));
#42720=CARTESIAN_POINT('Ctrl Pts',(-36.0033917073514,91.3774170351665,121.526154430422));
#42721=CARTESIAN_POINT('Ctrl Pts',(-33.1409989526284,89.4482950386239,121.36820590723));
#42722=CARTESIAN_POINT('Ctrl Pts',(-33.1913893007143,85.9950129878222,121.210257384038));
#42723=CARTESIAN_POINT('Ctrl Pts',(-36.1106392417851,84.1503274667491,121.052308860845));
#42724=CARTESIAN_POINT('Ctrl Pts',(-39.2510960503128,85.5858976381881,120.894360337653));
#42725=CARTESIAN_POINT('Ctrl Pts',(-39.765820054418,89.0005543692986,120.73641181446));
#42726=CARTESIAN_POINT('Ctrl Pts',(-37.1879238856457,91.2981286694523,120.578463291268));
#42727=CARTESIAN_POINT('Ctrl Pts',(-33.854806193682,90.395578791602,120.420514768075));
#42728=CARTESIAN_POINT('Ctrl Pts',(-32.7884554748253,87.1111711244642,120.262566244883));
#42729=CARTESIAN_POINT('Ctrl Pts',(-34.9557228065637,84.4228016151801,120.10461772169));
#42730=CARTESIAN_POINT('Ctrl Pts',(-38.3916014780163,84.7679217534951,119.946669198498));
#42731=CARTESIAN_POINT('Ctrl Pts',(-39.9808903072863,87.8336271405144,119.788720675305));
#42732=CARTESIAN_POINT('Ctrl Pts',(-38.2826267686962,90.8403332500451,119.630772152113));
#42733=CARTESIAN_POINT('Ctrl Pts',(-34.8365760655942,91.0619524059114,119.47282362892));
#42734=CARTESIAN_POINT('Ctrl Pts',(-32.7671669298757,88.2975486234688,119.314875105728));
#42735=CARTESIAN_POINT('Ctrl Pts',(-33.9506699948071,85.0535230461015,119.156926582536));
#42736=CARTESIAN_POINT('Ctrl Pts',(-37.3140388761979,84.2711348517919,118.998978059343));
#42737=CARTESIAN_POINT('Ctrl Pts',(-39.8078093743896,86.65975169421,118.841029536151));
#42738=CARTESIAN_POINT('Ctrl Pts',(-39.1709555878457,90.0536872932633,118.683081012958));
#42739=CARTESIAN_POINT('Ctrl Pts',(-35.9808934930197,91.3757634804708,118.525132489766));
#42740=CARTESIAN_POINT('Ctrl Pts',(-33.1299553615612,89.4272939776113,118.367183966573));
#42741=CARTESIAN_POINT('Ctrl Pts',(-33.2030000939727,85.9748968269957,118.209235443381));
#42742=CARTESIAN_POINT('Ctrl Pts',(-36.1338002509514,84.1487555231856,118.051286920188));
#42743=CARTESIAN_POINT('Ctrl Pts',(-39.2650884673852,85.6045768477356,117.893338396996));
#42744=CARTESIAN_POINT('Ctrl Pts',(-39.7578209507915,89.0224118820099,117.735389873803));
#42745=CARTESIAN_POINT('Ctrl Pts',(-37.1652521444745,91.3034135494146,117.577441350611));
#42746=CARTESIAN_POINT('Ctrl Pts',(-33.8379853355952,90.3794670115321,117.419492827418));
#42747=CARTESIAN_POINT('Ctrl Pts',(-32.7927521455727,87.0882864937512,117.261544304226));
#42748=CARTESIAN_POINT('Ctrl Pts',(-34.9772337184436,84.4138852747866,117.103595781033));
#42749=CARTESIAN_POINT('Ctrl Pts',(-38.4108270501026,84.7810616016501,116.945647257841));
#42750=CARTESIAN_POINT('Ctrl Pts',(-39.9803974947487,87.8569078659315,116.787698734648));
#42751=CARTESIAN_POINT('Ctrl Pts',(-38.2628632665517,90.8526478074454,116.629750211456));
#42752=CARTESIAN_POINT('Ctrl Pts',(-34.8154604137739,91.0521351325312,116.471801688264));
#42753=CARTESIAN_POINT('Ctrl Pts',(-32.7638442550116,88.2745007506674,116.313853165071));
#42754=CARTESIAN_POINT('Ctrl Pts',(-33.9681527643291,85.0381412779581,116.155904641879));
#42755=CARTESIAN_POINT('Ctrl Pts',(-37.3364760437162,84.2773654188855,115.997956118686));
#42756=CARTESIAN_POINT('Ctrl Pts',(-39.8148578186742,86.6819455069184,115.840007595494));
#42757=CARTESIAN_POINT('Ctrl Pts',(-39.1562247104231,90.0717219082352,115.682059072301));
#42758=CARTESIAN_POINT('Ctrl Pts',(-35.9577393267937,91.3732874551507,115.524110549109));
#42759=CARTESIAN_POINT('Ctrl Pts',(-33.1193710875871,89.4065522516036,115.366162025916));
#42760=CARTESIAN_POINT('Ctrl Pts',(-33.2145821502242,85.9546952911023,115.208213502724));
#42761=CARTESIAN_POINT('Ctrl Pts',(-36.1570475399255,84.14741029625,115.050264979531));
#42762=CARTESIAN_POINT('Ctrl Pts',(-39.2789233788883,85.6233076057904,114.892316456339));
#42763=CARTESIAN_POINT('Ctrl Pts',(-39.7496997914867,89.0442360165511,114.734367933146));
#42764=CARTESIAN_POINT('Ctrl Pts',(-37.1425381224351,91.3085437813298,114.576419409954));
#42765=CARTESIAN_POINT('Ctrl Pts',(-33.8212725638248,90.3632519156092,114.418470886762));
#42766=CARTESIAN_POINT('Ctrl Pts',(-32.7971935859219,87.0654278042858,114.260522363569));
#42767=CARTESIAN_POINT('Ctrl Pts',(-34.9988024520367,84.4051082703102,114.102573840377));
#42768=CARTESIAN_POINT('Ctrl Pts',(-38.4299673621699,84.7943241251765,113.944625317184));
#42769=CARTESIAN_POINT('Ctrl Pts',(-39.9797554464671,87.8801851907431,113.786676793992));
#42770=CARTESIAN_POINT('Ctrl Pts',(-38.2430209835701,90.864835091082,113.628728270799));
#42771=CARTESIAN_POINT('Ctrl Pts',(-34.7944082905965,91.0421825355799,113.470779747607));
#42772=CARTESIAN_POINT('Ctrl Pts',(-32.7606696114516,88.2514319900887,113.312831224414));
#42773=CARTESIAN_POINT('Ctrl Pts',(-33.9857339531502,85.0228720973646,113.154882701222));
#42774=CARTESIAN_POINT('Ctrl Pts',(-37.3588727357218,84.2837399199298,112.996934178029));
#42775=CARTESIAN_POINT('Ctrl Pts',(-39.8217636143875,86.7041841233756,112.838985654837));
#42776=CARTESIAN_POINT('Ctrl Pts',(-39.1413783349011,90.0896615629203,112.681037131644));
#42777=CARTESIAN_POINT('Ctrl Pts',(-35.93460153719,91.3706628087708,112.523088608452));
#42778=CARTESIAN_POINT('Ctrl Pts',(-33.1089202140314,89.3857429912062,112.365140085259));
#42779=CARTESIAN_POINT('Ctrl Pts',(-33.2262936819204,85.934568540205,112.207191562067));
#42780=CARTESIAN_POINT('Ctrl Pts',(-36.1803029872748,84.1462143677634,112.049243038875));
#42781=CARTESIAN_POINT('Ctrl Pts',(-39.2926377350615,85.6421268117017,111.891294515682));
#42782=CARTESIAN_POINT('Ctrl Pts',(-39.741438666845,89.0660075552192,111.733345992489));
#42783=CARTESIAN_POINT('Ctrl Pts',(-37.11979162744,91.3135280607988,111.575397469297));
#42784=CARTESIAN_POINT('Ctrl Pts',(-33.8046642536859,90.3469298412686,111.417448946105));
#42785=CARTESIAN_POINT('Ctrl Pts',(-32.8017817103211,87.0425981045389,111.259500422912));
#42786=CARTESIAN_POINT('Ctrl Pts',(-35.0204270981272,84.3964699395587,111.10155189972));
#42787=CARTESIAN_POINT('Ctrl Pts',(-38.449022121016,84.8077092752406,110.943603376527));
#42788=CARTESIAN_POINT('Ctrl Pts',(-39.9789639477665,87.9034579130465,110.785654853335));
#42789=CARTESIAN_POINT('Ctrl Pts',(-38.223100855083,90.8768947163338,110.627706330142));
#42790=CARTESIAN_POINT('Ctrl Pts',(-34.7734205070594,91.0320949679017,110.46975780695));
#42791=CARTESIAN_POINT('Ctrl Pts',(-32.7576431577175,88.2283433211983,110.311809283757));
#42792=CARTESIAN_POINT('Ctrl Pts',(-34.0034128231148,85.0077161192772,110.153860760565));
#42793=CARTESIAN_POINT('Ctrl Pts',(-37.3812280349669,84.2902581008489,109.995912237372));
#42794=CARTESIAN_POINT('Ctrl Pts',(-39.8285264744325,86.7264666190477,109.83796371418));
#42795=CARTESIAN_POINT('Ctrl Pts',(-39.1264170732664,90.1075055283665,109.680015190987));
#42796=CARTESIAN_POINT('Ctrl Pts',(-35.9114810808611,91.3678896299961,109.522066667795));
#42797=CARTESIAN_POINT('Ctrl Pts',(-33.0986031650656,89.3648670933915,109.364118144603));
#42798=CARTESIAN_POINT('Ctrl Pts',(-33.2381342205824,85.9145173244662,109.20616962141));
#42799=CARTESIAN_POINT('Ctrl Pts',(-36.2035656043253,84.1451679505691,109.048221098218));
#42800=CARTESIAN_POINT('Ctrl Pts',(-39.3062310320116,85.6610333533782,108.890272575025));
#42801=CARTESIAN_POINT('Ctrl Pts',(-39.7330377908336,89.0877262916886,108.732324051833));
#42802=CARTESIAN_POINT('Ctrl Pts',(-37.0970138577844,91.3183647606488,108.57437552864));
#42803=CARTESIAN_POINT('Ctrl Pts',(-33.7881605542584,90.3305043851839,108.416427005448));
#42804=CARTESIAN_POINT('Ctrl Pts',(-32.8065174312516,87.0197923230117,108.258478482255));
#42805=CARTESIAN_POINT('Ctrl Pts',(-35.0421044995447,84.3879830042027,108.100529959063));
#42806=CARTESIAN_POINT('Ctrl Pts',(-38.4679952003212,84.8211910697221,107.94258143587));
#42807=CARTESIAN_POINT('Ctrl Pts',(-39.9780134492052,87.9267773718166,107.784632912678));
#42808=CARTESIAN_POINT('Ctrl Pts',(-38.2031234082454,90.8887186315066,107.626684389485));
#42809=CARTESIAN_POINT('Ctrl Pts',(-34.7524574012803,91.0220940358159,107.468735866293));
#42810=CARTESIAN_POINT('Ctrl Pts',(-32.7548483299835,88.204780757559,107.3107873431));
#42811=CARTESIAN_POINT('Ctrl Pts',(-34.0210170033453,84.9936094992121,107.152838819908));
#42812=CARTESIAN_POINT('Ctrl Pts',(-37.4038845674691,84.2949818609618,106.994890296715));
#42813=CARTESIAN_POINT('Ctrl Pts',(-39.8343602819912,86.7527669934546,106.836941773523));
#42814=CARTESIAN_POINT('Ctrl Pts',(-39.3517092963754,88.9930721690098,106.731642758061));
#42815=CARTESIAN_POINT('Ctrl Pts',(-38.6909887323795,89.7658571455031,106.678993250331));
#42816=CARTESIAN_POINT('Ctrl Pts',(-37.1008589290306,84.9783780187301,122.10700224989));
#42817=CARTESIAN_POINT('Ctrl Pts',(-38.0238681217074,85.2251375401039,122.054352742159));
#42818=CARTESIAN_POINT('Ctrl Pts',(-39.5901175276382,86.7031405575811,121.949053726697));
#42819=CARTESIAN_POINT('Ctrl Pts',(-39.016178852264,89.9001750495482,121.791105203505));
#42820=CARTESIAN_POINT('Ctrl Pts',(-36.024589376484,91.1598011830645,121.633156680313));
#42821=CARTESIAN_POINT('Ctrl Pts',(-33.3348001000567,89.3470060484142,121.47520815712));
#42822=CARTESIAN_POINT('Ctrl Pts',(-33.3821518891126,86.1019583471864,121.317259633927));
#42823=CARTESIAN_POINT('Ctrl Pts',(-36.1253698398103,84.3685081332785,121.159311110735));
#42824=CARTESIAN_POINT('Ctrl Pts',(-39.0764557914928,85.7175128239604,121.001362587543));
#42825=CARTESIAN_POINT('Ctrl Pts',(-39.5601417232285,88.9262643284023,120.84341406435));
#42826=CARTESIAN_POINT('Ctrl Pts',(-37.1376937698282,91.0852939389096,120.685465541158));
#42827=CARTESIAN_POINT('Ctrl Pts',(-34.0055644664261,90.2371681955513,120.527517017965));
#42828=CARTESIAN_POINT('Ctrl Pts',(-33.0035151411689,87.1508116821394,120.369568494773));
#42829=CARTESIAN_POINT('Ctrl Pts',(-35.0400953478657,84.6245519767882,120.21161997158));
#42830=CARTESIAN_POINT('Ctrl Pts',(-38.2687891007858,84.9488612266584,120.053671448388));
#42831=CARTESIAN_POINT('Ctrl Pts',(-39.7622431500468,87.8297032987619,119.895722925195));
#42832=CARTESIAN_POINT('Ctrl Pts',(-38.16638561194,90.6551037744441,119.737774402003));
#42833=CARTESIAN_POINT('Ctrl Pts',(-34.928133205126,90.863359202675,119.57982587881));
#42834=CARTESIAN_POINT('Ctrl Pts',(-32.9835103043688,88.2656501225846,119.421877355618));
#42835=CARTESIAN_POINT('Ctrl Pts',(-34.0956476403156,85.2172406420686,119.263928832425));
#42836=CARTESIAN_POINT('Ctrl Pts',(-37.2562039737911,84.4820307825603,119.105980309233));
#42837=CARTESIAN_POINT('Ctrl Pts',(-39.5995990696733,86.7266130320189,118.94803178604));
#42838=CARTESIAN_POINT('Ctrl Pts',(-39.0011478323748,89.9158928973185,118.790083262848));
#42839=CARTESIAN_POINT('Ctrl Pts',(-36.0034478138706,91.1582473384075,118.632134739656));
#42840=CARTESIAN_POINT('Ctrl Pts',(-33.324422442142,89.3272713601495,118.474186216463));
#42841=CARTESIAN_POINT('Ctrl Pts',(-33.3930625466895,86.0830551992572,118.316237693271));
#42842=CARTESIAN_POINT('Ctrl Pts',(-36.147134230453,84.3670309785681,118.158289170078));
#42843=CARTESIAN_POINT('Ctrl Pts',(-39.0896044599732,85.7350656693728,118.000340646886));
#42844=CARTESIAN_POINT('Ctrl Pts',(-39.5526249688907,88.9468038239705,117.842392123693));
#42845=CARTESIAN_POINT('Ctrl Pts',(-37.1163891441162,91.0902601384036,117.684443600501));
#42846=CARTESIAN_POINT('Ctrl Pts',(-33.9897579131054,90.222027962547,117.526495077308));
#42847=CARTESIAN_POINT('Ctrl Pts',(-33.0075527208761,87.1293070042139,117.368546554116));
#42848=CARTESIAN_POINT('Ctrl Pts',(-35.0603091427774,84.6161732954432,117.210598030923));
#42849=CARTESIAN_POINT('Ctrl Pts',(-38.2868553628477,84.9612087364832,117.052649507731));
#42850=CARTESIAN_POINT('Ctrl Pts',(-39.7617800543109,87.8515801867154,116.894700984538));
#42851=CARTESIAN_POINT('Ctrl Pts',(-38.147813857227,90.6666757588912,116.736752461346));
#42852=CARTESIAN_POINT('Ctrl Pts',(-34.9082908359274,90.8541339149789,116.578803938153));
#42853=CARTESIAN_POINT('Ctrl Pts',(-32.9803879881863,88.2439920461367,116.420855414961));
#42854=CARTESIAN_POINT('Ctrl Pts',(-34.1120761915356,85.2027864009668,116.262906891768));
#42855=CARTESIAN_POINT('Ctrl Pts',(-37.2772881707395,84.4878856438566,116.104958368576));
#42856=CARTESIAN_POINT('Ctrl Pts',(-39.6062224898245,86.7474685485538,115.947009845384));
#42857=CARTESIAN_POINT('Ctrl Pts',(-38.9873052330117,89.9328400174774,115.789061322191));
#42858=CARTESIAN_POINT('Ctrl Pts',(-35.9816898535359,91.155920618448,115.631112798999));
#42859=CARTESIAN_POINT('Ctrl Pts',(-33.3144764043081,89.3077803688807,115.473164275806));
#42860=CARTESIAN_POINT('Ctrl Pts',(-33.403946200113,86.0640718244132,115.315215752614));
#42861=CARTESIAN_POINT('Ctrl Pts',(-36.1689796981952,84.3657668693785,115.157267229421));
#42862=CARTESIAN_POINT('Ctrl Pts',(-39.1026051205359,85.7526669548959,114.999318706229));
#42863=CARTESIAN_POINT('Ctrl Pts',(-39.544993518883,88.9673119540864,114.841370183036));
#42864=CARTESIAN_POINT('Ctrl Pts',(-37.09504478709,91.095081015192,114.683421659844));
#42865=CARTESIAN_POINT('Ctrl Pts',(-33.9740529284511,90.206790643679,114.525473136651));
#42866=CARTESIAN_POINT('Ctrl Pts',(-33.0117263405178,87.1078267032678,114.367524613459));
#42867=CARTESIAN_POINT('Ctrl Pts',(-35.0805772727288,84.6079255480015,114.209576090266));
#42868=CARTESIAN_POINT('Ctrl Pts',(-38.3048415061054,84.9736715243033,114.051627567074));
#42869=CARTESIAN_POINT('Ctrl Pts',(-39.7611767218088,87.8734538791213,113.893679043882));
#42870=CARTESIAN_POINT('Ctrl Pts',(-38.1291680721943,90.678128144236,113.735730520689));
#42871=CARTESIAN_POINT('Ctrl Pts',(-34.8885081645678,90.8447814637793,113.577781997497));
#42872=CARTESIAN_POINT('Ctrl Pts',(-32.9774047769586,88.2223143414533,113.419833474304));
#42873=CARTESIAN_POINT('Ctrl Pts',(-34.1285972273298,85.1884379583387,113.261884951112));
#42874=CARTESIAN_POINT('Ctrl Pts',(-37.2983343328655,84.4938757598263,113.103936427919));
#42875=CARTESIAN_POINT('Ctrl Pts',(-39.6127118631728,86.7683661671529,112.945987904727));
#42876=CARTESIAN_POINT('Ctrl Pts',(-38.9733541001328,89.9496979034943,112.788039381534));
#42877=CARTESIAN_POINT('Ctrl Pts',(-35.9599472823065,91.1534542393407,112.630090858342));
#42878=CARTESIAN_POINT('Ctrl Pts',(-33.3046557227915,89.2882259155742,112.472142335149));
#42879=CARTESIAN_POINT('Ctrl Pts',(-33.4149515215578,86.0451587249989,112.314193811957));
#42880=CARTESIAN_POINT('Ctrl Pts',(-36.190832832359,84.3646430558789,112.156245288764));
#42881=CARTESIAN_POINT('Ctrl Pts',(-39.1154924953055,85.7703513548328,111.998296765572));
#42882=CARTESIAN_POINT('Ctrl Pts',(-39.5372305435066,88.9877706598821,111.840348242379));
#42883=CARTESIAN_POINT('Ctrl Pts',(-37.0736699152408,91.0997647405279,111.682399719187));
#42884=CARTESIAN_POINT('Ctrl Pts',(-33.9584461063484,90.1914527972364,111.524451195994));
#42885=CARTESIAN_POINT('Ctrl Pts',(-33.0160377990999,87.0863736439481,111.366502672802));
#42886=CARTESIAN_POINT('Ctrl Pts',(-35.1008979436308,84.5998081122014,111.20855414961));
#42887=CARTESIAN_POINT('Ctrl Pts',(-38.3227472550368,84.9862495442295,111.050605626417));
#42888=CARTESIAN_POINT('Ctrl Pts',(-39.7604329508104,87.8953232465526,110.892657103225));
#42889=CARTESIAN_POINT('Ctrl Pts',(-38.1104491357725,90.6894605690494,110.734708580032));
#42890=CARTESIAN_POINT('Ctrl Pts',(-34.8687859531413,90.8353021806444,110.57676005684));
#42891=CARTESIAN_POINT('Ctrl Pts',(-32.9745608196483,88.2006179289376,110.418811533647));
#42892=CARTESIAN_POINT('Ctrl Pts',(-34.1452100540536,85.1741958920582,110.260863010455));
#42893=CARTESIAN_POINT('Ctrl Pts',(-37.3193415982316,84.5000008917143,110.102914487262));
#42894=CARTESIAN_POINT('Ctrl Pts',(-39.6190669199333,86.789305019032,109.94496596407));
#42895=CARTESIAN_POINT('Ctrl Pts',(-38.9592950088217,89.9664658703735,109.787017440877));
#42896=CARTESIAN_POINT('Ctrl Pts',(-35.9382209991481,91.1508482844039,109.629068917685));
#42897=CARTESIAN_POINT('Ctrl Pts',(-33.2949607961862,89.2686088431145,109.471120394492));
#42898=CARTESIAN_POINT('Ctrl Pts',(-33.4260780707944,86.0263166059414,109.3131718713));
#42899=CARTESIAN_POINT('Ctrl Pts',(-36.2126927038881,84.3636597380785,109.155223348107));
#42900=CARTESIAN_POINT('Ctrl Pts',(-39.1282661107737,85.7881178241517,108.997274824915));
#42901=CARTESIAN_POINT('Ctrl Pts',(-39.5293362438264,89.0081797474739,108.839326301723));
#42902=CARTESIAN_POINT('Ctrl Pts',(-37.0522656546062,91.1043097853572,108.68137777853));
#42903=CARTESIAN_POINT('Ctrl Pts',(-33.9429375868874,90.1760178030121,108.523429255338));
#42904=CARTESIAN_POINT('Ctrl Pts',(-33.0204879540809,87.0649430605694,108.365480732145));
#42905=CARTESIAN_POINT('Ctrl Pts',(-35.1212681886914,84.591832942591,108.207532208953));
#42906=CARTESIAN_POINT('Ctrl Pts',(-38.3405762497377,84.9989183808745,108.04958368576));
#42907=CARTESIAN_POINT('Ctrl Pts',(-39.7595397677092,87.9172365322217,107.891635162568));
#42908=CARTESIAN_POINT('Ctrl Pts',(-38.0916763373207,90.7005714972004,107.733686639375));
#42909=CARTESIAN_POINT('Ctrl Pts',(-34.8490869313939,90.825904308939,107.575738116183));
#42910=CARTESIAN_POINT('Ctrl Pts',(-32.9719345211937,88.1784761977243,107.41778959299));
#42911=CARTESIAN_POINT('Ctrl Pts',(-34.1617526948657,85.1609399070733,107.259841069798));
#42912=CARTESIAN_POINT('Ctrl Pts',(-37.3406319323637,84.50443980712,107.101892546605));
#42913=CARTESIAN_POINT('Ctrl Pts',(-39.6245489464603,86.8140194698805,106.943944023413));
#42914=CARTESIAN_POINT('Ctrl Pts',(-39.171002016807,88.9192333079152,106.838645007951));
#42915=CARTESIAN_POINT('Ctrl Pts',(-38.5501231787025,89.6454190276512,106.78599550022));
#42916=CARTESIAN_POINT('Ctrl Pts',(-37.0529925008447,85.1574234026337,122.21400449978));
#42917=CARTESIAN_POINT('Ctrl Pts',(-37.9167722964266,85.3883483930035,122.161354992049));
#42918=CARTESIAN_POINT('Ctrl Pts',(-39.3825156524183,86.7715081214603,122.056055976587));
#42919=CARTESIAN_POINT('Ctrl Pts',(-38.845406557921,89.7633892661443,121.898107453395));
#42920=CARTESIAN_POINT('Ctrl Pts',(-36.0457870456165,90.9421853309626,121.740158930202));
#42921=CARTESIAN_POINT('Ctrl Pts',(-33.528601247485,89.2457170582044,121.58221040701));
#42922=CARTESIAN_POINT('Ctrl Pts',(-33.5729144775109,86.2089037065505,121.424261883817));
#42923=CARTESIAN_POINT('Ctrl Pts',(-36.1401004378356,84.5866887998078,121.266313360625));
#42924=CARTESIAN_POINT('Ctrl Pts',(-38.9018155326728,85.8491280097327,121.108364837432));
#42925=CARTESIAN_POINT('Ctrl Pts',(-39.354463392039,88.8519742875062,120.95041631424));
#42926=CARTESIAN_POINT('Ctrl Pts',(-37.0874636540108,90.8724592083668,120.792467791047));
#42927=CARTESIAN_POINT('Ctrl Pts',(-34.1563227391702,90.0787575995008,120.634519267855));
#42928=CARTESIAN_POINT('Ctrl Pts',(-33.2185748075125,87.1904522398145,120.476570744663));
#42929=CARTESIAN_POINT('Ctrl Pts',(-35.1244678891676,84.8263023383961,120.31862222147));
#42930=CARTESIAN_POINT('Ctrl Pts',(-38.1459767235555,85.1298006998218,120.160673698278));
#42931=CARTESIAN_POINT('Ctrl Pts',(-39.5435959928072,87.8257794570092,120.002725175085));
#42932=CARTESIAN_POINT('Ctrl Pts',(-38.0501444551837,90.4698742988431,119.844776651893));
#42933=CARTESIAN_POINT('Ctrl Pts',(-35.0196903446579,90.6647659994386,119.6868281287));
#42934=CARTESIAN_POINT('Ctrl Pts',(-33.1998536788618,88.2337516217006,119.528879605508));
#42935=CARTESIAN_POINT('Ctrl Pts',(-34.2406252858241,85.3809582380354,119.370931082315));
#42936=CARTESIAN_POINT('Ctrl Pts',(-37.1983690713843,84.6929267133288,119.212982559123));
#42937=CARTESIAN_POINT('Ctrl Pts',(-39.391388764957,86.7934743698275,119.05503403593));
#42938=CARTESIAN_POINT('Ctrl Pts',(-38.8313400769042,89.7780985013739,118.897085512738));
#42939=CARTESIAN_POINT('Ctrl Pts',(-36.0260021347214,90.940731196344,118.739136989545));
#42940=CARTESIAN_POINT('Ctrl Pts',(-33.5188895227229,89.2272487426878,118.581188466353));
#42941=CARTESIAN_POINT('Ctrl Pts',(-33.5831249994063,86.1912135715186,118.42323994316));
#42942=CARTESIAN_POINT('Ctrl Pts',(-36.1604682099547,84.5853064339508,118.265291419968));
#42943=CARTESIAN_POINT('Ctrl Pts',(-38.9141204525613,85.8655544910099,118.107342896776));
#42944=CARTESIAN_POINT('Ctrl Pts',(-39.3474289869899,88.8711957659313,117.949394373583));
#42945=CARTESIAN_POINT('Ctrl Pts',(-37.0675261437579,90.8771067273923,117.791445850391));
#42946=CARTESIAN_POINT('Ctrl Pts',(-34.1415304906156,90.0645889135622,117.633497327198));
#42947=CARTESIAN_POINT('Ctrl Pts',(-33.2223532961796,87.1703275146764,117.475548804006));
#42948=CARTESIAN_POINT('Ctrl Pts',(-35.1433845671111,84.8184613160999,117.317600280813));
#42949=CARTESIAN_POINT('Ctrl Pts',(-38.162883675593,85.1413558713164,117.159651757621));
#42950=CARTESIAN_POINT('Ctrl Pts',(-39.5431626138732,87.8462525074993,117.001703234428));
#42951=CARTESIAN_POINT('Ctrl Pts',(-38.0327644479022,90.4807037103371,116.843754711236));
#42952=CARTESIAN_POINT('Ctrl Pts',(-35.0011212580808,90.6561326974266,116.685806188043));
#42953=CARTESIAN_POINT('Ctrl Pts',(-33.1969317213611,88.2134833416061,116.527857664851));
#42954=CARTESIAN_POINT('Ctrl Pts',(-34.255999618742,85.3674315239755,116.369909141658));
#42955=CARTESIAN_POINT('Ctrl Pts',(-37.2181002977627,84.6984058688277,116.211960618466));
#42956=CARTESIAN_POINT('Ctrl Pts',(-39.3975871609747,86.8129915901892,116.054012095273));
#42957=CARTESIAN_POINT('Ctrl Pts',(-38.8183857556004,89.7939581267197,115.896063572081));
#42958=CARTESIAN_POINT('Ctrl Pts',(-36.0056403802781,90.9385537817452,115.738115048888));
#42959=CARTESIAN_POINT('Ctrl Pts',(-33.5095817210291,89.209008486158,115.580166525696));
#42960=CARTESIAN_POINT('Ctrl Pts',(-33.5933102500017,86.1734483577242,115.422218002503));
#42961=CARTESIAN_POINT('Ctrl Pts',(-36.1809118564649,84.584123442507,115.264269479311));
#42962=CARTESIAN_POINT('Ctrl Pts',(-38.9262868621835,85.8820263040013,115.106320956119));
#42963=CARTESIAN_POINT('Ctrl Pts',(-39.3402872462792,88.8903878916216,114.948372432926));
#42964=CARTESIAN_POINT('Ctrl Pts',(-37.0475514517448,90.8816182490542,114.790423909734));
#42965=CARTESIAN_POINT('Ctrl Pts',(-34.1268332930775,90.0503293717488,114.632475386541));
#42966=CARTESIAN_POINT('Ctrl Pts',(-33.2262590951137,87.1502256022498,114.474526863349));
#42967=CARTESIAN_POINT('Ctrl Pts',(-35.1623520934209,84.8107428256929,114.316578340156));
#42968=CARTESIAN_POINT('Ctrl Pts',(-38.1797156500409,85.1530189234301,114.158629816964));
#42969=CARTESIAN_POINT('Ctrl Pts',(-39.5425979971506,87.8667225674997,114.000681293771));
#42970=CARTESIAN_POINT('Ctrl Pts',(-38.0153151608184,90.4914211973897,113.842732770579));
#42971=CARTESIAN_POINT('Ctrl Pts',(-34.9826080385391,90.6473803919789,113.684784247386));
#42972=CARTESIAN_POINT('Ctrl Pts',(-33.1941399424655,88.1931966928179,113.526835724194));
#42973=CARTESIAN_POINT('Ctrl Pts',(-34.2714605015093,85.3540038193127,113.368887201001));
#42974=CARTESIAN_POINT('Ctrl Pts',(-37.2377959300091,84.7040115997228,113.210938677809));
#42975=CARTESIAN_POINT('Ctrl Pts',(-39.4036601119581,86.8325482109303,113.052990154616));
#42976=CARTESIAN_POINT('Ctrl Pts',(-38.8053298653645,89.8097342440683,112.895041631424));
#42977=CARTESIAN_POINT('Ctrl Pts',(-35.985293027423,90.9362456699106,112.737093108231));
#42978=CARTESIAN_POINT('Ctrl Pts',(-33.5003912315516,89.1907088399423,112.579144585039));
#42979=CARTESIAN_POINT('Ctrl Pts',(-33.6036093611951,86.1557489097928,112.421196061847));
#42980=CARTESIAN_POINT('Ctrl Pts',(-36.2013626774433,84.5830717439945,112.263247538654));
#42981=CARTESIAN_POINT('Ctrl Pts',(-38.9383472555495,85.8985758979639,112.105299015462));
#42982=CARTESIAN_POINT('Ctrl Pts',(-39.3330224201682,88.909533764545,111.947350492269));
#42983=CARTESIAN_POINT('Ctrl Pts',(-37.0275482030416,90.886001420257,111.789401969077));
#42984=CARTESIAN_POINT('Ctrl Pts',(-34.1122279590109,90.0359757532041,111.631453445884));
#42985=CARTESIAN_POINT('Ctrl Pts',(-33.2302938878788,87.1301491833573,111.473504922692));
#42986=CARTESIAN_POINT('Ctrl Pts',(-35.1813687891343,84.803146284844,111.315556399499));
#42987=CARTESIAN_POINT('Ctrl Pts',(-38.1964723890577,85.1647898132184,111.157607876307));
#42988=CARTESIAN_POINT('Ctrl Pts',(-39.5419019538542,87.8871885800586,110.999659353114));
#42989=CARTESIAN_POINT('Ctrl Pts',(-37.9977974164621,90.502026421765,110.841710829922));
#42990=CARTESIAN_POINT('Ctrl Pts',(-34.9641513992233,90.6385093933869,110.683762306729));
#42991=CARTESIAN_POINT('Ctrl Pts',(-33.1914784815791,88.1728925366768,110.525813783537));
#42992=CARTESIAN_POINT('Ctrl Pts',(-34.2870072849925,85.3406756648394,110.367865260344));
#42993=CARTESIAN_POINT('Ctrl Pts',(-37.2574551614964,84.7097436825796,110.209916737152));
#42994=CARTESIAN_POINT('Ctrl Pts',(-39.409607365434,86.8521434190164,110.05196821396));
#42995=CARTESIAN_POINT('Ctrl Pts',(-38.792172944377,89.8254262123803,109.894019690767));
#42996=CARTESIAN_POINT('Ctrl Pts',(-35.9649609174351,90.9338069388119,109.736071167575));
#42997=CARTESIAN_POINT('Ctrl Pts',(-33.4913184273068,89.1723505928374,109.578122644382));
#42998=CARTESIAN_POINT('Ctrl Pts',(-33.6140219210065,86.1381158874167,109.42017412119));
#42999=CARTESIAN_POINT('Ctrl Pts',(-36.221819803451,84.5821515255878,109.262225597997));
#43000=CARTESIAN_POINT('Ctrl Pts',(-38.9503011895357,85.9152022949253,109.104277074805));
#43001=CARTESIAN_POINT('Ctrl Pts',(-39.3256346968193,88.9286332032591,108.946328551612));
#43002=CARTESIAN_POINT('Ctrl Pts',(-37.0075174514281,90.8902548100658,108.78838002842));
#43003=CARTESIAN_POINT('Ctrl Pts',(-34.0977146195165,90.0215312208402,108.630431505227));
#43004=CARTESIAN_POINT('Ctrl Pts',(-33.2344584769103,87.1100937981272,108.472482982035));
#43005=CARTESIAN_POINT('Ctrl Pts',(-35.2004318778381,84.7956828809793,108.314534458842));
#43006=CARTESIAN_POINT('Ctrl Pts',(-38.2131572991543,85.1766456920269,108.15658593565));
#43007=CARTESIAN_POINT('Ctrl Pts',(-39.5410660862132,87.907695692627,107.998637412457));
#43008=CARTESIAN_POINT('Ctrl Pts',(-37.9802292663962,90.5124243628941,107.840688889265));
#43009=CARTESIAN_POINT('Ctrl Pts',(-34.9457164615075,90.6297145820622,107.682740366073));
#43010=CARTESIAN_POINT('Ctrl Pts',(-33.1890207124038,88.1521716378895,107.52479184288));
#43011=CARTESIAN_POINT('Ctrl Pts',(-34.3024883863861,85.3282703149345,107.366843319688));
#43012=CARTESIAN_POINT('Ctrl Pts',(-37.2773792972584,84.7138977532781,107.208894796495));
#43013=CARTESIAN_POINT('Ctrl Pts',(-39.4147376109293,86.8752719463065,107.050946273303));
#43014=CARTESIAN_POINT('Ctrl Pts',(-38.9902947372386,88.8453944468205,106.945647257841));
#43015=CARTESIAN_POINT('Ctrl Pts',(-38.4092576250255,89.5249809097992,106.89299775011));
#43016=CARTESIAN_POINT('Ctrl Pts',(-37.0051260726588,85.3364687865372,122.321006749669));
#43017=CARTESIAN_POINT('Ctrl Pts',(-37.8096764711459,85.551559245903,122.268357241939));
#43018=CARTESIAN_POINT('Ctrl Pts',(-39.1749137771984,86.8398756853395,122.163058226477));
#43019=CARTESIAN_POINT('Ctrl Pts',(-38.674634263578,89.6266034827405,122.005109703284));
#43020=CARTESIAN_POINT('Ctrl Pts',(-36.0669847147491,90.7245694788604,121.847161180092));
#43021=CARTESIAN_POINT('Ctrl Pts',(-33.7224023949133,89.1444280679948,121.6892126569));
#43022=CARTESIAN_POINT('Ctrl Pts',(-33.7636770659093,86.3158490659145,121.531264133707));
#43023=CARTESIAN_POINT('Ctrl Pts',(-36.1548310358608,84.8048694663372,121.373315610515));
#43024=CARTESIAN_POINT('Ctrl Pts',(-38.7271752738528,85.980743195505,121.215367087322));
#43025=CARTESIAN_POINT('Ctrl Pts',(-39.1487850608496,88.7776842466098,121.05741856413));
#43026=CARTESIAN_POINT('Ctrl Pts',(-37.0372335381933,90.6596244778241,120.899470040937));
#43027=CARTESIAN_POINT('Ctrl Pts',(-34.3070810119143,89.9203470034502,120.741521517745));
#43028=CARTESIAN_POINT('Ctrl Pts',(-33.4336344738561,87.2300927974898,120.583572994552));
#43029=CARTESIAN_POINT('Ctrl Pts',(-35.2088404304695,85.028052700004,120.42562447136));
#43030=CARTESIAN_POINT('Ctrl Pts',(-38.023164346325,85.3107401729852,120.267675948167));
#43031=CARTESIAN_POINT('Ctrl Pts',(-39.3249488355677,87.8218556152566,120.109727424975));
#43032=CARTESIAN_POINT('Ctrl Pts',(-37.9339032984275,90.2846448232422,119.951778901782));
#43033=CARTESIAN_POINT('Ctrl Pts',(-35.1112474841897,90.4661727962024,119.79383037859));
#43034=CARTESIAN_POINT('Ctrl Pts',(-33.4161970533549,88.2018531208163,119.635881855397));
#43035=CARTESIAN_POINT('Ctrl Pts',(-34.3856029313326,85.5446758340026,119.477933332205));
#43036=CARTESIAN_POINT('Ctrl Pts',(-37.1405341689775,84.903822644097,119.319984809013));
#43037=CARTESIAN_POINT('Ctrl Pts',(-39.1831784602407,86.8603357076363,119.16203628582));
#43038=CARTESIAN_POINT('Ctrl Pts',(-38.6615323214334,89.6403041054291,119.004087762628));
#43039=CARTESIAN_POINT('Ctrl Pts',(-36.0485564555722,90.7232150542806,118.846139239435));
#43040=CARTESIAN_POINT('Ctrl Pts',(-33.7133566033038,89.1272261252261,118.688190716243));
#43041=CARTESIAN_POINT('Ctrl Pts',(-33.7731874521231,86.2993719437801,118.53024219305));
#43042=CARTESIAN_POINT('Ctrl Pts',(-36.1738021894563,84.8035818893332,118.372293669858));
#43043=CARTESIAN_POINT('Ctrl Pts',(-38.7386364451493,85.9960433126471,118.214345146665));
#43044=CARTESIAN_POINT('Ctrl Pts',(-39.1422330050891,88.7955877078919,118.056396623473));
#43045=CARTESIAN_POINT('Ctrl Pts',(-37.0186631433996,90.6639533163812,117.89844810028));
#43046=CARTESIAN_POINT('Ctrl Pts',(-34.2933030681259,89.9071498645772,117.740499577088));
#43047=CARTESIAN_POINT('Ctrl Pts',(-33.4371538714831,87.2113480251391,117.582551053896));
#43048=CARTESIAN_POINT('Ctrl Pts',(-35.2264599914449,85.0207493367565,117.424602530703));
#43049=CARTESIAN_POINT('Ctrl Pts',(-38.0389119883381,85.3215030061496,117.266654007511));
#43050=CARTESIAN_POINT('Ctrl Pts',(-39.3245451734354,87.8409248282832,117.108705484318));
#43051=CARTESIAN_POINT('Ctrl Pts',(-37.9177150385775,90.2947316617829,116.950756961126));
#43052=CARTESIAN_POINT('Ctrl Pts',(-35.0939516802342,90.4581314798742,116.792808437933));
#43053=CARTESIAN_POINT('Ctrl Pts',(-33.4134754545358,88.1829746370754,116.634859914741));
#43054=CARTESIAN_POINT('Ctrl Pts',(-34.3999230459485,85.5320766469841,116.476911391548));
#43055=CARTESIAN_POINT('Ctrl Pts',(-37.158912424786,84.9089260937988,116.318962868356));
#43056=CARTESIAN_POINT('Ctrl Pts',(-39.188951832125,86.8785146318246,116.161014345163));
#43057=CARTESIAN_POINT('Ctrl Pts',(-38.6494662781891,89.6550762359618,116.003065821971));
#43058=CARTESIAN_POINT('Ctrl Pts',(-36.0295909070203,90.7211869450424,115.845117298778));
#43059=CARTESIAN_POINT('Ctrl Pts',(-33.70468703775,89.1102366034352,115.687168775586));
#43060=CARTESIAN_POINT('Ctrl Pts',(-33.7826742998905,86.2828248910351,115.529220252393));
#43061=CARTESIAN_POINT('Ctrl Pts',(-36.1928440147345,84.8024800156354,115.371271729201));
#43062=CARTESIAN_POINT('Ctrl Pts',(-38.7499686038312,86.0113856531068,115.213323206008));
#43063=CARTESIAN_POINT('Ctrl Pts',(-39.1355809736756,88.8134638291569,115.055374682816));
#43064=CARTESIAN_POINT('Ctrl Pts',(-37.0000581163997,90.6681554829164,114.897426159623));
#43065=CARTESIAN_POINT('Ctrl Pts',(-34.2796136577039,89.8938680998186,114.739477636431));
#43066=CARTESIAN_POINT('Ctrl Pts',(-33.4407918497096,87.1926245012317,114.581529113239));
#43067=CARTESIAN_POINT('Ctrl Pts',(-35.2441269141131,85.0135601033844,114.423580590046));
#43068=CARTESIAN_POINT('Ctrl Pts',(-38.0545897939765,85.3323663225568,114.265632066854));
#43069=CARTESIAN_POINT('Ctrl Pts',(-39.3240192724923,87.8599912558781,114.107683543661));
#43070=CARTESIAN_POINT('Ctrl Pts',(-37.9014622494426,90.3047142505435,113.949735020469));
#43071=CARTESIAN_POINT('Ctrl Pts',(-35.0767079125104,90.4499793201784,113.791786497276));
#43072=CARTESIAN_POINT('Ctrl Pts',(-33.4108751079725,88.1640790441824,113.633837974084));
#43073=CARTESIAN_POINT('Ctrl Pts',(-34.4143237756889,85.5195696802868,113.475889450891));
#43074=CARTESIAN_POINT('Ctrl Pts',(-37.1772575271527,84.9141474396192,113.317940927699));
#43075=CARTESIAN_POINT('Ctrl Pts',(-39.1946083607433,86.8967302547077,113.159992404506));
#43076=CARTESIAN_POINT('Ctrl Pts',(-38.6373056305963,89.6697705846423,113.002043881314));
#43077=CARTESIAN_POINT('Ctrl Pts',(-36.0106387725394,90.7190371004805,112.844095358121));
#43078=CARTESIAN_POINT('Ctrl Pts',(-33.6961267403118,89.0931917643103,112.686146834929));
#43079=CARTESIAN_POINT('Ctrl Pts',(-33.7922672008325,86.2663390945867,112.528198311736));
#43080=CARTESIAN_POINT('Ctrl Pts',(-36.2118925225276,84.8015004321101,112.370249788544));
#43081=CARTESIAN_POINT('Ctrl Pts',(-38.7612020157935,86.026800441095,112.212301265352));
#43082=CARTESIAN_POINT('Ctrl Pts',(-39.1288142968298,88.8312968692079,112.054352742159));
#43083=CARTESIAN_POINT('Ctrl Pts',(-36.9814264908424,90.6722380999861,111.896404218967));
#43084=CARTESIAN_POINT('Ctrl Pts',(-34.2660098116734,89.8804987091719,111.738455695774));
#43085=CARTESIAN_POINT('Ctrl Pts',(-33.4445499766577,87.1739247227665,111.580507172582));
#43086=CARTESIAN_POINT('Ctrl Pts',(-35.2618396346379,85.0064844574867,111.422558649389));
#43087=CARTESIAN_POINT('Ctrl Pts',(-38.0701975230785,85.3433300822074,111.264610126197));
#43088=CARTESIAN_POINT('Ctrl Pts',(-39.3233709568981,87.8790539135646,111.106661603004));
#43089=CARTESIAN_POINT('Ctrl Pts',(-37.8851456971516,90.3145922744807,110.948713079812));
#43090=CARTESIAN_POINT('Ctrl Pts',(-35.0595168453053,90.4417166061294,110.790764556619));
#43091=CARTESIAN_POINT('Ctrl Pts',(-33.40839614351,88.1451671444161,110.632816033427));
#43092=CARTESIAN_POINT('Ctrl Pts',(-34.4288045159315,85.5071554376204,110.474867510234));
#43093=CARTESIAN_POINT('Ctrl Pts',(-37.1955687247611,84.919486473445,110.316918987042));
#43094=CARTESIAN_POINT('Ctrl Pts',(-39.2001478109348,86.9149818190007,110.158970463849));
#43095=CARTESIAN_POINT('Ctrl Pts',(-38.6250508799324,89.6843865543872,110.001021940657));
#43096=CARTESIAN_POINT('Ctrl Pts',(-35.9917008357221,90.7167655932198,109.843073417465));
#43097=CARTESIAN_POINT('Ctrl Pts',(-33.6876760584274,89.0760923425604,109.685124894272));
#43098=CARTESIAN_POINT('Ctrl Pts',(-33.8019657712185,86.2499151688921,109.52717637108));
#43099=CARTESIAN_POINT('Ctrl Pts',(-36.2309469030138,84.8006433130971,109.369227847887));
#43100=CARTESIAN_POINT('Ctrl Pts',(-38.7723362682978,86.042286765699,109.211279324695));
#43101=CARTESIAN_POINT('Ctrl Pts',(-39.1219331498121,88.8490866590441,109.053330801502));
#43102=CARTESIAN_POINT('Ctrl Pts',(-36.9627692482499,90.6761998347745,108.89538227831));
#43103=CARTESIAN_POINT('Ctrl Pts',(-34.2524916521456,89.8670446386682,108.737433755117));
#43104=CARTESIAN_POINT('Ctrl Pts',(-33.4484289997396,87.1552445356851,108.579485231925));
#43105=CARTESIAN_POINT('Ctrl Pts',(-35.2795955669848,84.9995328193676,108.421536708732));
#43106=CARTESIAN_POINT('Ctrl Pts',(-38.0857383485708,85.3543730031793,108.26358818554));
#43107=CARTESIAN_POINT('Ctrl Pts',(-39.3225924047172,87.8981548530322,108.105639662347));
#43108=CARTESIAN_POINT('Ctrl Pts',(-37.8687821954715,90.3242772285877,107.947691139155));
#43109=CARTESIAN_POINT('Ctrl Pts',(-35.0423459916211,90.4335248551855,107.789742615962));
#43110=CARTESIAN_POINT('Ctrl Pts',(-33.406106903614,88.1258670780547,107.63179409277));
#43111=CARTESIAN_POINT('Ctrl Pts',(-34.4432240779066,85.4956007227958,107.473845569577));
#43112=CARTESIAN_POINT('Ctrl Pts',(-37.2141266621531,84.9233556994363,107.315897046385));
#43113=CARTESIAN_POINT('Ctrl Pts',(-39.2049262753984,86.9365244227325,107.157948523192));
#43114=CARTESIAN_POINT('Ctrl Pts',(-38.8095874576701,88.7715555857258,107.052649507731));
#43115=CARTESIAN_POINT('Ctrl Pts',(-38.2683920713485,89.4045427919473,107.));
#43116=CARTESIAN_POINT('Ctrl Pts',(-38.8699207989934,87.7703173750275,121.112583302492));
#43117=CARTESIAN_POINT('Ctrl Pts',(-38.8718336645079,88.0618702234686,121.094195056371));
#43118=CARTESIAN_POINT('Ctrl Pts',(-38.8249623706359,88.3528282219475,121.07580681025));
#43119=CARTESIAN_POINT('Ctrl Pts',(-38.7265915092407,88.6251841099614,121.05741856413));
#43120=CARTESIAN_POINT('Ctrl Pts',(-38.4449345532975,89.4049976570146,121.004769056399));
#43121=CARTESIAN_POINT('Ctrl Pts',(-37.7410840457454,90.0323110674193,120.952119548668));
#43122=CARTESIAN_POINT('Ctrl Pts',(-36.9341333709228,90.2227548602261,120.899470040937));
#43123=CARTESIAN_POINT('Ctrl Pts',(-36.1271826961003,90.4131986530328,120.846820533206));
#43124=CARTESIAN_POINT('Ctrl Pts',(-35.2171318540073,90.1667728282415,120.794171025476));
#43125=CARTESIAN_POINT('Ctrl Pts',(-34.6165320099511,89.5951842148525,120.741521517745));
#43126=CARTESIAN_POINT('Ctrl Pts',(-34.0159321658949,89.0235956014634,120.688872010014));
#43127=CARTESIAN_POINT('Ctrl Pts',(-33.7247833198755,88.1268441994766,120.636222502283));
#43128=CARTESIAN_POINT('Ctrl Pts',(-33.8750765563014,87.3114618155689,120.583572994552));
#43129=CARTESIAN_POINT('Ctrl Pts',(-34.0253697927272,86.4960794316612,120.530923486822));
#43130=CARTESIAN_POINT('Ctrl Pts',(-34.6171051115984,85.7620660658326,120.478273979091));
#43131=CARTESIAN_POINT('Ctrl Pts',(-35.3820267570099,85.4421739617485,120.42562447136));
#43132=CARTESIAN_POINT('Ctrl Pts',(-36.1469484024214,85.1222818576644,120.372974963629));
#43133=CARTESIAN_POINT('Ctrl Pts',(-37.0850563743732,85.2165110153248,120.320325455898));
#43134=CARTESIAN_POINT('Ctrl Pts',(-37.7710744418896,85.6821448345336,120.267675948167));
#43135=CARTESIAN_POINT('Ctrl Pts',(-38.4446885721246,86.1393594983833,120.215978399609));
#43136=CARTESIAN_POINT('Ctrl Pts',(-38.8752464913585,86.9546694615518,120.16428085105));
#43137=CARTESIAN_POINT('Ctrl Pts',(-38.8765117847785,87.7688288397063,120.112583302492));
#43138=CARTESIAN_POINT('Ctrl Pts',(-37.1487253572165,84.7993326348266,122.));
#43139=CARTESIAN_POINT('Ctrl Pts',(-37.2417753891008,84.8333707521416,122.));
#43140=CARTESIAN_POINT('Ctrl Pts',(-37.3327602562807,84.8721775720516,122.));
#43141=CARTESIAN_POINT('Ctrl Pts',(-37.4214714739468,84.9154247709244,122.));
#43142=CARTESIAN_POINT('Ctrl Pts',(-37.5121496630562,84.9596308790244,122.));
#43143=CARTESIAN_POINT('Ctrl Pts',(-37.6004529266836,85.0084770764388,122.));
#43144=CARTESIAN_POINT('Ctrl Pts',(-37.6861296852363,85.0616582541536,122.));
#43145=CARTESIAN_POINT('Ctrl Pts',(-37.7685611201985,85.1128249983916,122.));
#43146=CARTESIAN_POINT('Ctrl Pts',(-37.8485615426075,85.1680054118964,122.));
#43147=CARTESIAN_POINT('Ctrl Pts',(-37.9258739256416,85.2269578069965,122.));
#43148=CARTESIAN_POINT('Ctrl Pts',(-37.9935222607964,85.2785411527092,122.));
#43149=CARTESIAN_POINT('Ctrl Pts',(-38.059112275569,85.3330131191914,122.));
#43150=CARTESIAN_POINT('Ctrl Pts',(-38.1224471612445,85.3902244937864,122.));
#43151=CARTESIAN_POINT('Ctrl Pts',(-38.1365836289362,85.402994182086,122.));
#43152=CARTESIAN_POINT('Ctrl Pts',(-38.1506103907732,85.4159030811327,122.));
#43153=CARTESIAN_POINT('Ctrl Pts',(-38.1645056734731,85.428930998852,122.));
#43154=CARTESIAN_POINT('Ctrl Pts',(-38.236935765249,85.4968398925705,122.));
#43155=CARTESIAN_POINT('Ctrl Pts',(-38.3059001696468,85.5680707029916,122.));
#43156=CARTESIAN_POINT('Ctrl Pts',(-38.3711589370242,85.6423327060287,122.));
#43157=CARTESIAN_POINT('Ctrl Pts',(-38.4360586851855,85.7161861588099,122.));
#43158=CARTESIAN_POINT('Ctrl Pts',(-38.4972939435271,85.7930383408696,122.));
#43159=CARTESIAN_POINT('Ctrl Pts',(-38.5545850913186,85.8726300682051,122.));
#43160=CARTESIAN_POINT('Ctrl Pts',(-38.6097480011666,85.9492651409677,122.));
#43161=CARTESIAN_POINT('Ctrl Pts',(-38.6612545505178,86.0284407407527,122.));
#43162=CARTESIAN_POINT('Ctrl Pts',(-38.7088102913344,86.1099390932959,122.));
#43163=CARTESIAN_POINT('Ctrl Pts',(-38.7287566222569,86.144121992806,122.));
#43164=CARTESIAN_POINT('Ctrl Pts',(-38.7480073496925,86.1787136222189,122.));
#43165=CARTESIAN_POINT('Ctrl Pts',(-38.7665381634545,86.2136982099032,122.));
#43166=CARTESIAN_POINT('Ctrl Pts',(-38.7794207042811,86.2380193425275,122.));
#43167=CARTESIAN_POINT('Ctrl Pts',(-38.7919552805797,86.2625303934131,122.));
#43168=CARTESIAN_POINT('Ctrl Pts',(-38.8041332584856,86.2872260692728,122.));
#43169=CARTESIAN_POINT('Ctrl Pts',(-38.8120415994691,86.3032633643826,122.));
#43170=CARTESIAN_POINT('Ctrl Pts',(-38.8198006651,86.319381131767,122.));
#43171=CARTESIAN_POINT('Ctrl Pts',(-38.8273979149827,86.3355557323494,122.));
#43172=CARTESIAN_POINT('Ctrl Pts',(-38.8695182138971,86.4252301568939,122.));
#43173=CARTESIAN_POINT('Ctrl Pts',(-38.9067396802643,86.5167881682253,122.));
#43174=CARTESIAN_POINT('Ctrl Pts',(-38.9387710306477,86.6099574003158,122.));
#43175=CARTESIAN_POINT('Ctrl Pts',(-38.9686507850787,86.6968683092245,122.));
#43176=CARTESIAN_POINT('Ctrl Pts',(-38.9940140885018,86.7851820439995,122.));
#43177=CARTESIAN_POINT('Ctrl Pts',(-39.0145739632211,86.8746862171339,122.));
#43178=CARTESIAN_POINT('Ctrl Pts',(-39.0160544487227,86.8811312773528,122.));
#43179=CARTESIAN_POINT('Ctrl Pts',(-39.0175100048601,86.8875825114178,122.));
#43180=CARTESIAN_POINT('Ctrl Pts',(-39.0189405138548,86.8940398403423,122.));
#43181=CARTESIAN_POINT('Ctrl Pts',(-39.0395467338659,86.9870564805743,122.));
#43182=CARTESIAN_POINT('Ctrl Pts',(-39.0549599296115,87.0813387804123,122.));
#43183=CARTESIAN_POINT('Ctrl Pts',(-39.0652570210305,87.1764788744327,122.));
#43184=CARTESIAN_POINT('Ctrl Pts',(-39.0710535407633,87.2300358848478,122.));
#43185=CARTESIAN_POINT('Ctrl Pts',(-39.0752279006169,87.2838645309515,122.));
#43186=CARTESIAN_POINT('Ctrl Pts',(-39.0777870601897,87.3378894180018,122.));
#43187=CARTESIAN_POINT('Ctrl Pts',(-39.0784479432014,87.3518409239729,122.));
#43188=CARTESIAN_POINT('Ctrl Pts',(-39.07900098961,87.3658049179873,122.));
#43189=CARTESIAN_POINT('Ctrl Pts',(-39.0794460778701,87.3797667321621,122.));
#43190=CARTESIAN_POINT('Ctrl Pts',(-39.0824174908988,87.4729759229344,122.));
#43191=CARTESIAN_POINT('Ctrl Pts',(-39.0805897501033,87.5662433468626,122.));
#43192=CARTESIAN_POINT('Ctrl Pts',(-39.0740977497051,87.659193925161,122.));
#43193=CARTESIAN_POINT('Ctrl Pts',(-39.0675949549735,87.7522990535925,122.));
#43194=CARTESIAN_POINT('Ctrl Pts',(-39.0564119991282,87.845087261528,122.));
#43195=CARTESIAN_POINT('Ctrl Pts',(-39.0406335176743,87.9371695003463,122.));
#43196=CARTESIAN_POINT('Ctrl Pts',(-39.0250806320128,88.0279351761161,122.));
#43197=CARTESIAN_POINT('Ctrl Pts',(-39.0050622311029,88.1180157699776,122.));
#43198=CARTESIAN_POINT('Ctrl Pts',(-38.9806163469264,88.2070134839553,122.));
#43199=CARTESIAN_POINT('Ctrl Pts',(-38.9715175827602,88.2401384552168,122.));
#43200=CARTESIAN_POINT('Ctrl Pts',(-38.9618050679078,88.2731130950482,122.));
#43201=CARTESIAN_POINT('Ctrl Pts',(-38.9514794019202,88.3059156261388,122.));
#43202=CARTESIAN_POINT('Ctrl Pts',(-38.944484882208,88.328135786136,122.));
#43203=CARTESIAN_POINT('Ctrl Pts',(-38.9372089974467,88.3502769571618,122.));
#43204=CARTESIAN_POINT('Ctrl Pts',(-38.9296517548766,88.3723321568593,122.));
#43205=CARTESIAN_POINT('Ctrl Pts',(-38.9251356923547,88.3855119191658,122.));
#43206=CARTESIAN_POINT('Ctrl Pts',(-38.9205195020769,88.3986598081647,122.));
#43207=CARTESIAN_POINT('Ctrl Pts',(-38.9158066558644,88.4117651858116,122.));
#43208=CARTESIAN_POINT('Ctrl Pts',(-38.8841749038243,88.4997260564677,122.));
#43209=CARTESIAN_POINT('Ctrl Pts',(-38.8481539347597,88.5858891804725,122.));
#43210=CARTESIAN_POINT('Ctrl Pts',(-38.8078083123978,88.6698403149831,122.));
#43211=CARTESIAN_POINT('Ctrl Pts',(-38.7775490956264,88.7328036658661,122.));
#43212=CARTESIAN_POINT('Ctrl Pts',(-38.7448562140504,88.7945222807168,122.));
#43213=CARTESIAN_POINT('Ctrl Pts',(-38.7097409437031,88.8548058697244,122.));
#43214=CARTESIAN_POINT('Ctrl Pts',(-38.6962715801236,88.8779291881608,122.));
#43215=CARTESIAN_POINT('Ctrl Pts',(-38.6824456762413,88.900841209529,122.));
#43216=CARTESIAN_POINT('Ctrl Pts',(-38.6682633879976,88.9235305507161,122.));
#43217=CARTESIAN_POINT('Ctrl Pts',(-38.6581392015999,88.9397275927922,122.));
#43218=CARTESIAN_POINT('Ctrl Pts',(-38.6478325658439,88.9558122233299,122.));
#43219=CARTESIAN_POINT('Ctrl Pts',(-38.6373536122841,88.9717652973009,122.));
#43220=CARTESIAN_POINT('Ctrl Pts',(-38.5901670347616,89.04360176049,122.));
#43221=CARTESIAN_POINT('Ctrl Pts',(-38.5394455308257,89.112844773472,122.));
#43222=CARTESIAN_POINT('Ctrl Pts',(-38.4852219917805,89.1791423373427,122.));
#43223=CARTESIAN_POINT('Ctrl Pts',(-38.4364255687668,89.2388043223104,122.));
#43224=CARTESIAN_POINT('Ctrl Pts',(-38.3847924489325,89.2960808804698,122.));
#43225=CARTESIAN_POINT('Ctrl Pts',(-38.3303261109488,89.3506856727381,122.));
#43226=CARTESIAN_POINT('Ctrl Pts',(-38.3112435400582,89.369816751823,122.));
#43227=CARTESIAN_POINT('Ctrl Pts',(-38.2918130242121,89.3886195826515,122.));
#43228=CARTESIAN_POINT('Ctrl Pts',(-38.272045138338,89.4070896778011,122.));
#43229=CARTESIAN_POINT('Origin',(-36.3549260746835,87.7685555885722,114.));
#43230=CARTESIAN_POINT('Origin',(36.3549260746835,-87.7685555885722,107.));
#43231=CARTESIAN_POINT('Ctrl Pts',(34.441460078019,-86.1325683851967,107.));
#43232=CARTESIAN_POINT('Ctrl Pts',(34.3793224918267,-86.1909624581861,107.));
#43233=CARTESIAN_POINT('Ctrl Pts',(34.320560277281,-86.2526104359851,107.));
#43234=CARTESIAN_POINT('Ctrl Pts',(34.2651854154857,-86.3171358435518,107.));
#43235=CARTESIAN_POINT('Ctrl Pts',(34.2084554811663,-86.383240245703,107.));
#43236=CARTESIAN_POINT('Ctrl Pts',(34.1552802428995,-86.4523651183919,107.));
#43237=CARTESIAN_POINT('Ctrl Pts',(34.1057014708844,-86.5241519419432,107.));
#43238=CARTESIAN_POINT('Ctrl Pts',(34.0927636287905,-86.5428850922367,107.));
#43239=CARTESIAN_POINT('Ctrl Pts',(34.080070868449,-86.5617997318037,107.));
#43240=CARTESIAN_POINT('Ctrl Pts',(34.0676243075757,-86.5808899227627,107.));
#43241=CARTESIAN_POINT('Ctrl Pts',(34.0574544824683,-86.5964881193486,107.));
#43242=CARTESIAN_POINT('Ctrl Pts',(34.0474485842597,-86.612204424695,107.));
#43243=CARTESIAN_POINT('Ctrl Pts',(34.0376160702623,-86.6280210049421,107.));
#43244=CARTESIAN_POINT('Ctrl Pts',(33.9901718947115,-86.7043396971966,107.));
#43245=CARTESIAN_POINT('Ctrl Pts',(33.9467112825774,-86.783065746378,107.));
#43246=CARTESIAN_POINT('Ctrl Pts',(33.9072689218163,-86.8638066024608,107.));
#43247=CARTESIAN_POINT('Ctrl Pts',(33.8754404287267,-86.9289614190155,107.));
#43248=CARTESIAN_POINT('Ctrl Pts',(33.8462290730293,-86.9954293421335,107.));
#43249=CARTESIAN_POINT('Ctrl Pts',(33.819670241093,-87.0630218995359,107.));
#43250=CARTESIAN_POINT('Ctrl Pts',(33.8090685977204,-87.0900032136971,107.));
#43251=CARTESIAN_POINT('Ctrl Pts',(33.7988897945031,-87.1171638805078,107.));
#43252=CARTESIAN_POINT('Ctrl Pts',(33.7891368427985,-87.1444924579589,107.));
#43253=CARTESIAN_POINT('Ctrl Pts',(33.7838959378683,-87.1591779071067,107.));
#43254=CARTESIAN_POINT('Ctrl Pts',(33.7787783829148,-87.1739110234873,107.));
#43255=CARTESIAN_POINT('Ctrl Pts',(33.7737886445088,-87.1886775541965,107.));
#43256=CARTESIAN_POINT('Ctrl Pts',(33.744249812514,-87.2760941749241,107.));
#43257=CARTESIAN_POINT('Ctrl Pts',(33.7191464479123,-87.3647918982878,107.));
#43258=CARTESIAN_POINT('Ctrl Pts',(33.6985111208832,-87.4543729160899,107.));
#43259=CARTESIAN_POINT('Ctrl Pts',(33.6775543388031,-87.5453494179855,107.));
#43260=CARTESIAN_POINT('Ctrl Pts',(33.6612053831337,-87.6372377538553,107.));
#43261=CARTESIAN_POINT('Ctrl Pts',(33.6495401950691,-87.729654418924,107.));
#43262=CARTESIAN_POINT('Ctrl Pts',(33.6379657251133,-87.821352375899,107.));
#43263=CARTESIAN_POINT('Ctrl Pts',(33.631002112185,-87.9135714065299,107.));
#43264=CARTESIAN_POINT('Ctrl Pts',(33.6287704839946,-88.0059560939408,107.));
#43265=CARTESIAN_POINT('Ctrl Pts',(33.6276598722209,-88.0519330725417,107.));
#43266=CARTESIAN_POINT('Ctrl Pts',(33.6277220148865,-88.0979512931867,107.));
#43267=CARTESIAN_POINT('Ctrl Pts',(33.6289766402602,-88.1439676459876,107.));
#43268=CARTESIAN_POINT('Ctrl Pts',(33.6293464212451,-88.1575302381508,107.));
#43269=CARTESIAN_POINT('Ctrl Pts',(33.6298198132723,-88.1710926687391,107.));
#43270=CARTESIAN_POINT('Ctrl Pts',(33.6303973778168,-88.1846538340193,107.));
#43271=CARTESIAN_POINT('Ctrl Pts',(33.6310178764361,-88.199223087642,107.));
#43272=CARTESIAN_POINT('Ctrl Pts',(33.6317582082676,-88.2137810937379,107.));
#43273=CARTESIAN_POINT('Ctrl Pts',(33.6326184218729,-88.2283239261021,107.));
#43274=CARTESIAN_POINT('Ctrl Pts',(33.6382702188031,-88.3238736067939,107.));
#43275=CARTESIAN_POINT('Ctrl Pts',(33.6490946590568,-88.4188015746807,107.));
#43276=CARTESIAN_POINT('Ctrl Pts',(33.6651621993108,-88.5127121877848,107.));
#43277=CARTESIAN_POINT('Ctrl Pts',(33.6675425111235,-88.5266244940976,107.));
#43278=CARTESIAN_POINT('Ctrl Pts',(33.6700379786409,-88.5405145062868,107.));
#43279=CARTESIAN_POINT('Ctrl Pts',(33.6726489234542,-88.5543809687066,107.));
#43280=CARTESIAN_POINT('Ctrl Pts',(33.6895945630855,-88.6443775377394,107.));
#43281=CARTESIAN_POINT('Ctrl Pts',(33.7114000884911,-88.733381941817,107.));
#43282=CARTESIAN_POINT('Ctrl Pts',(33.737762949146,-88.8211619318416,107.));
#43283=CARTESIAN_POINT('Ctrl Pts',(33.7647217588965,-88.9109262439152,107.));
#43284=CARTESIAN_POINT('Ctrl Pts',(33.7964464848098,-88.9994108591658,107.));
#43285=CARTESIAN_POINT('Ctrl Pts',(33.8326678325411,-89.086363731768,107.));
#43286=CARTESIAN_POINT('Ctrl Pts',(33.845157910542,-89.1163473803409,107.));
#43287=CARTESIAN_POINT('Ctrl Pts',(33.8581831105127,-89.1461488154908,107.));
#43288=CARTESIAN_POINT('Ctrl Pts',(33.8717337628504,-89.1757573633716,107.));
#43289=CARTESIAN_POINT('Ctrl Pts',(33.8784247684257,-89.1903773944972,107.));
#43290=CARTESIAN_POINT('Ctrl Pts',(33.8852438980845,-89.2049503931226,107.));
#43291=CARTESIAN_POINT('Ctrl Pts',(33.8921900469341,-89.219475051693,107.));
#43292=CARTESIAN_POINT('Ctrl Pts',(33.8976838231309,-89.2309627444056,107.));
#43293=CARTESIAN_POINT('Ctrl Pts',(33.9032566146494,-89.2424191739447,107.));
#43294=CARTESIAN_POINT('Ctrl Pts',(33.9089032804855,-89.253834763427,107.));
#43295=CARTESIAN_POINT('Ctrl Pts',(33.9516272055465,-89.3402076432341,107.));
#43296=CARTESIAN_POINT('Ctrl Pts',(33.9986419909546,-89.424382211309,107.));
#43297=CARTESIAN_POINT('Ctrl Pts',(34.0496049802514,-89.506108829215,107.));
#43298=CARTESIAN_POINT('Ctrl Pts',(34.1015786903742,-89.5894562860063,107.));
#43299=CARTESIAN_POINT('Ctrl Pts',(34.1576590761245,-89.6702585036094,107.));
#43300=CARTESIAN_POINT('Ctrl Pts',(34.2175376968044,-89.7482436651937,107.));
#43301=CARTESIAN_POINT('Ctrl Pts',(34.2779031585332,-89.8268628824301,107.));
#43302=CARTESIAN_POINT('Ctrl Pts',(34.342129327908,-89.9026198862294,107.));
#43303=CARTESIAN_POINT('Ctrl Pts',(34.4099495107696,-89.9752168962673,107.));
#43304=CARTESIAN_POINT('Ctrl Pts',(34.4469502263334,-90.0148237095471,107.));
#43305=CARTESIAN_POINT('Ctrl Pts',(34.4850215078373,-90.0534895501217,107.));
#43306=CARTESIAN_POINT('Ctrl Pts',(34.5241253959326,-90.0911622835395,107.));
#43307=CARTESIAN_POINT('Ctrl Pts',(34.536092533356,-90.1026914383087,107.));
#43308=CARTESIAN_POINT('Ctrl Pts',(34.5481564062128,-90.1141275592007,107.));
#43309=CARTESIAN_POINT('Ctrl Pts',(34.560315989506,-90.1254690898891,107.));
#43310=CARTESIAN_POINT('Ctrl Pts',(34.5708617769609,-90.1353053950623,107.));
#43311=CARTESIAN_POINT('Ctrl Pts',(34.5814784435051,-90.145069435766,107.));
#43312=CARTESIAN_POINT('Ctrl Pts',(34.5921562070644,-90.154752216978,107.));
#43313=CARTESIAN_POINT('Ctrl Pts',(34.6677306685615,-90.2232844495778,107.));
#43314=CARTESIAN_POINT('Ctrl Pts',(34.746481851648,-90.2878603390861,107.));
#43315=CARTESIAN_POINT('Ctrl Pts',(34.82808240795,-90.3481981124324,107.));
#43316=CARTESIAN_POINT('Ctrl Pts',(34.9097871680395,-90.4086129370245,107.));
#43317=CARTESIAN_POINT('Ctrl Pts',(34.9943491566684,-90.46477965297,107.));
#43318=CARTESIAN_POINT('Ctrl Pts',(35.0814850443532,-90.5163896064528,107.));
#43319=CARTESIAN_POINT('Ctrl Pts',(35.1668886983011,-90.5669735704729,107.));
#43320=CARTESIAN_POINT('Ctrl Pts',(35.2547655959762,-90.613180823026,107.));
#43321=CARTESIAN_POINT('Ctrl Pts',(35.3448830612224,-90.6546849506116,107.));
#43322=CARTESIAN_POINT('Ctrl Pts',(35.3852331814247,-90.6732684353156,107.));
#43323=CARTESIAN_POINT('Ctrl Pts',(35.4260328929523,-90.6909084910784,107.));
#43324=CARTESIAN_POINT('Ctrl Pts',(35.4672630634612,-90.7075728698848,107.));
#43325=CARTESIAN_POINT('Ctrl Pts',(35.4976827134229,-90.7198678607583,107.));
#43326=CARTESIAN_POINT('Ctrl Pts',(35.5283367073931,-90.7316316981734,107.));
#43327=CARTESIAN_POINT('Ctrl Pts',(35.5592127764326,-90.7428670628568,107.));
#43328=CARTESIAN_POINT('Ctrl Pts',(37.1487253572158,-90.7377785423181,107.));
#43329=CARTESIAN_POINT('Ctrl Pts',(37.2435592465647,-90.703087881974,107.));
#43330=CARTESIAN_POINT('Ctrl Pts',(37.3363499820799,-90.6634063347566,107.));
#43331=CARTESIAN_POINT('Ctrl Pts',(37.4268566408666,-90.6190542519878,107.));
#43332=CARTESIAN_POINT('Ctrl Pts',(37.5186361899685,-90.5740783992404,107.));
#43333=CARTESIAN_POINT('Ctrl Pts',(37.6080676322742,-90.5242990120235,107.));
#43334=CARTESIAN_POINT('Ctrl Pts',(37.6948657117722,-90.4700094660602,107.));
#43335=CARTESIAN_POINT('Ctrl Pts',(37.7193787255217,-90.4546773251379,107.));
#43336=CARTESIAN_POINT('Ctrl Pts',(37.7436814680841,-90.4389852541544,107.));
#43337=CARTESIAN_POINT('Ctrl Pts',(37.7677669178499,-90.4229394055795,107.));
#43338=CARTESIAN_POINT('Ctrl Pts',(37.7870964822202,-90.4100619519335,107.));
#43339=CARTESIAN_POINT('Ctrl Pts',(37.8062881985499,-90.3969550139071,107.));
#43340=CARTESIAN_POINT('Ctrl Pts',(37.8253191512513,-90.3836355366237,107.));
#43341=CARTESIAN_POINT('Ctrl Pts',(37.9080262499151,-90.3257500834303,107.));
#43342=CARTESIAN_POINT('Ctrl Pts',(37.9877784886294,-90.263802481533,107.));
#43343=CARTESIAN_POINT('Ctrl Pts',(38.0643095059346,-90.1980900928801,107.));
#43344=CARTESIAN_POINT('Ctrl Pts',(38.1233026941829,-90.1474363390095,107.));
#43345=CARTESIAN_POINT('Ctrl Pts',(38.1803812147524,-90.0945446577292,107.));
#43346=CARTESIAN_POINT('Ctrl Pts',(38.2354054997586,-90.0395394799401,107.));
#43347=CARTESIAN_POINT('Ctrl Pts',(38.2646942393973,-90.0102609108346,107.));
#43348=CARTESIAN_POINT('Ctrl Pts',(38.2934006760903,-89.9803833759801,107.));
#43349=CARTESIAN_POINT('Ctrl Pts',(38.3215017395818,-89.9499248098952,107.));
#43350=CARTESIAN_POINT('Ctrl Pts',(38.3311377428159,-89.9394804065583,107.));
#43351=CARTESIAN_POINT('Ctrl Pts',(38.3407018304141,-89.9289683913002,107.));
#43352=CARTESIAN_POINT('Ctrl Pts',(38.3501864357286,-89.9183970998547,107.));
#43353=CARTESIAN_POINT('Ctrl Pts',(38.4159836260407,-89.8450612833374,107.));
#43354=CARTESIAN_POINT('Ctrl Pts',(38.4780486658794,-89.7687788430213,107.));
#43355=CARTESIAN_POINT('Ctrl Pts',(38.5361377867705,-89.6898283382125,107.));
#43356=CARTESIAN_POINT('Ctrl Pts',(38.5937004502349,-89.6115933560172,107.));
#43357=CARTESIAN_POINT('Ctrl Pts',(38.6473593689752,-89.5307376665252,107.));
#43358=CARTESIAN_POINT('Ctrl Pts',(38.6968315991878,-89.4475099381577,107.));
#43359=CARTESIAN_POINT('Ctrl Pts',(38.7448895391944,-89.3666614872271,107.));
#43360=CARTESIAN_POINT('Ctrl Pts',(38.7889969518342,-89.2835739814083,107.));
#43361=CARTESIAN_POINT('Ctrl Pts',(38.8288466859154,-89.1984650429878,107.));
#43362=CARTESIAN_POINT('Ctrl Pts',(38.8496511020266,-89.1540320797447,107.));
#43363=CARTESIAN_POINT('Ctrl Pts',(38.8692942322878,-89.1090480478038,107.));
#43364=CARTESIAN_POINT('Ctrl Pts',(38.8877266765946,-89.0635436780106,107.));
#43365=CARTESIAN_POINT('Ctrl Pts',(38.8947847579787,-89.046119318008,107.));
#43366=CARTESIAN_POINT('Ctrl Pts',(38.9016652800419,-89.0286186647692,107.));
#43367=CARTESIAN_POINT('Ctrl Pts',(38.9083653072029,-89.0110434524178,107.));
#43368=CARTESIAN_POINT('Ctrl Pts',(38.9136070431997,-88.9972935643921,107.));
#43369=CARTESIAN_POINT('Ctrl Pts',(38.9187384030901,-88.9834975405313,107.));
#43370=CARTESIAN_POINT('Ctrl Pts',(38.9237528516952,-88.9696709241645,107.));
#43371=CARTESIAN_POINT('Ctrl Pts',(38.9554365396406,-88.8823077397353,107.));
#43372=CARTESIAN_POINT('Ctrl Pts',(38.9825114019973,-88.7935836147519,107.));
#43373=CARTESIAN_POINT('Ctrl Pts',(39.0047261827264,-88.7037221014846,107.));
#43374=CARTESIAN_POINT('Ctrl Pts',(39.0097101548453,-88.6835613228504,107.));
#43375=CARTESIAN_POINT('Ctrl Pts',(39.0144492932001,-88.6633432545392,107.));
#43376=CARTESIAN_POINT('Ctrl Pts',(39.0189403996523,-88.6430703655259,107.));
#43377=CARTESIAN_POINT('Ctrl Pts',(39.0393061529012,-88.5511391989667,107.));
#43378=CARTESIAN_POINT('Ctrl Pts',(39.054575694401,-88.4580804162001,107.));
#43379=CARTESIAN_POINT('Ctrl Pts',(39.0648588490549,-88.3642856036222,107.));
#43380=CARTESIAN_POINT('Ctrl Pts',(39.0755927118845,-88.2663797871473,107.));
#43381=CARTESIAN_POINT('Ctrl Pts',(39.0808934919427,-88.1676707693011,107.));
#43382=CARTESIAN_POINT('Ctrl Pts',(39.0808286362865,-88.0686185665232,107.));
#43383=CARTESIAN_POINT('Ctrl Pts',(39.0808032678039,-88.0298740031761,107.));
#43384=CARTESIAN_POINT('Ctrl Pts',(39.0799563544502,-87.9910771891197,107.));
#43385=CARTESIAN_POINT('Ctrl Pts',(39.0782897088242,-87.9522568820768,107.));
#43386=CARTESIAN_POINT('Ctrl Pts',(39.0777566699434,-87.9398410855225,107.));
#43387=CARTESIAN_POINT('Ctrl Pts',(39.0771397845791,-87.9274241972147,107.));
#43388=CARTESIAN_POINT('Ctrl Pts',(39.0764398138567,-87.9150168265058,107.));
#43389=CARTESIAN_POINT('Ctrl Pts',(39.0712006005755,-87.822148854568,107.));
#43390=CARTESIAN_POINT('Ctrl Pts',(39.0613049669259,-87.7296641169378,107.));
#43391=CARTESIAN_POINT('Ctrl Pts',(39.0468763718403,-87.6379341904711,107.));
#43392=CARTESIAN_POINT('Ctrl Pts',(39.0324817650919,-87.5464203451715,107.));
#43393=CARTESIAN_POINT('Ctrl Pts',(39.0135751177459,-87.4556568137981,107.));
#43394=CARTESIAN_POINT('Ctrl Pts',(38.9902303422857,-87.3660295059385,107.));
#43395=CARTESIAN_POINT('Ctrl Pts',(38.9672817156295,-87.2779231272848,107.));
#43396=CARTESIAN_POINT('Ctrl Pts',(38.9400438408593,-87.190913951763,107.));
#43397=CARTESIAN_POINT('Ctrl Pts',(38.9085464901449,-87.1053976716856,107.));
#43398=CARTESIAN_POINT('Ctrl Pts',(38.8927050482775,-87.0623876677065,107.));
#43399=CARTESIAN_POINT('Ctrl Pts',(38.8757855564829,-87.0197558321219,107.));
#43400=CARTESIAN_POINT('Ctrl Pts',(38.8577883849998,-86.9775562961909,107.));
#43401=CARTESIAN_POINT('Ctrl Pts',(38.8522226745452,-86.9645058899906,107.));
#43402=CARTESIAN_POINT('Ctrl Pts',(38.8465538809276,-86.9514968490023,107.));
#43403=CARTESIAN_POINT('Ctrl Pts',(38.8407819742204,-86.9385308318502,107.));
#43404=CARTESIAN_POINT('Ctrl Pts',(38.8351025159904,-86.9257724910523,107.));
#43405=CARTESIAN_POINT('Ctrl Pts',(38.8293267026267,-86.9130636714118,107.));
#43406=CARTESIAN_POINT('Ctrl Pts',(38.8234563238127,-86.9004088584368,107.));
#43407=CARTESIAN_POINT('Ctrl Pts',(38.7859765239624,-86.8196134153368,107.));
#43408=CARTESIAN_POINT('Ctrl Pts',(38.7446265669885,-86.7409747507621,107.));
#43409=CARTESIAN_POINT('Ctrl Pts',(38.6994761290357,-86.6648404554994,107.));
#43410=CARTESIAN_POINT('Ctrl Pts',(38.6550831229752,-86.5899833691838,107.));
#43411=CARTESIAN_POINT('Ctrl Pts',(38.6070156240331,-86.5175466622143,107.));
#43412=CARTESIAN_POINT('Ctrl Pts',(38.5553036472175,-86.4478949012765,107.));
#43413=CARTESIAN_POINT('Ctrl Pts',(38.5051691862912,-86.380367923926,107.));
#43414=CARTESIAN_POINT('Ctrl Pts',(38.4516087686083,-86.3154581290589,107.));
#43415=CARTESIAN_POINT('Ctrl Pts',(38.3946220345055,-86.2535380111354,107.));
#43416=CARTESIAN_POINT('Ctrl Pts',(38.373654460502,-86.2307552587053,107.));
#43417=CARTESIAN_POINT('Ctrl Pts',(38.3522227934278,-86.2083776778821,107.));
#43418=CARTESIAN_POINT('Ctrl Pts',(38.3303262041782,-86.1864254330304,107.));
#43419=CARTESIAN_POINT('Ctrl Pts',(38.311248768753,-86.1672995075806,107.));
#43420=CARTESIAN_POINT('Ctrl Pts',(38.2918183998859,-86.1484964687257,107.));
#43421=CARTESIAN_POINT('Ctrl Pts',(38.2720452344324,-86.1300214449938,107.));
#43422=CARTESIAN_POINT('Origin',(36.3549260746835,-87.7685555885722,124.208423447177));
#43423=CARTESIAN_POINT('Ctrl Pts',(33.2781264274053,-87.766627982914,121.708423447177));
#43424=CARTESIAN_POINT('Ctrl Pts',(33.2772037481594,-87.6433530720069,121.702019850418));
#43425=CARTESIAN_POINT('Ctrl Pts',(33.3397302338269,-86.5074461871871,121.642966745928));
#43426=CARTESIAN_POINT('Ctrl Pts',(34.7524572651294,-84.5150170630276,121.531264133707));
#43427=CARTESIAN_POINT('Ctrl Pts',(38.2031235339731,-84.6483923074236,121.373315610515));
#43428=CARTESIAN_POINT('Ctrl Pts',(39.9780136468089,-87.6103338294361,121.215367087322));
#43429=CARTESIAN_POINT('Ctrl Pts',(38.4679953249988,-90.71592025761,121.05741856413));
#43430=CARTESIAN_POINT('Ctrl Pts',(35.0421044228056,-91.1491283755177,120.899470040937));
#43431=CARTESIAN_POINT('Ctrl Pts',(33.3955573955644,-89.2107570630753,120.783138335287));
#43432=CARTESIAN_POINT('Ctrl Pts',(33.2786797629631,-87.9841152617576,120.719456137367));
#43433=CARTESIAN_POINT('Ctrl Pts',(33.2806115932904,-87.7712393060438,120.708423447177));
#43434=CARTESIAN_POINT('Ctrl Pts',(33.2846473629325,-87.7715718261144,121.791576552823));
#43435=CARTESIAN_POINT('Ctrl Pts',(33.2896323807993,-87.078553038224,121.755752019753));
#43436=CARTESIAN_POINT('Ctrl Pts',(33.862020072503,-85.3573618548392,121.667277978953));
#43437=CARTESIAN_POINT('Ctrl Pts',(36.7064604149176,-84.1596949927803,121.526154430422));
#43438=CARTESIAN_POINT('Ctrl Pts',(39.5688528980205,-86.0888159753533,121.36820590723));
#43439=CARTESIAN_POINT('Ctrl Pts',(39.5184626244884,-89.5420982077003,121.210257384038));
#43440=CARTESIAN_POINT('Ctrl Pts',(36.5992128626851,-91.3867833270583,121.052308860845));
#43441=CARTESIAN_POINT('Ctrl Pts',(33.8243658940394,-90.1183413579956,120.912748583774));
#43442=CARTESIAN_POINT('Ctrl Pts',(33.2888361264505,-88.4296039786679,120.825837814433));
#43443=CARTESIAN_POINT('Ctrl Pts',(33.2844849022013,-87.7664047084671,120.791576552823));
#43444=CARTESIAN_POINT('Ctrl Pts',(38.2683920713486,-86.1325683851972,122.));
#43445=CARTESIAN_POINT('Ctrl Pts',(38.8095874576702,-86.7655555914187,121.947350492269));
#43446=CARTESIAN_POINT('Ctrl Pts',(39.2049251670254,-88.6005879544937,121.842051476808));
#43447=CARTESIAN_POINT('Ctrl Pts',(37.2141270656728,-90.6137552465961,121.684102953615));
#43448=CARTESIAN_POINT('Ctrl Pts',(34.4432237898319,-90.0415108461503,121.526154430423));
#43449=CARTESIAN_POINT('Ctrl Pts',(33.4061068154979,-87.4112439256985,121.36820590723));
#43450=CARTESIAN_POINT('Ctrl Pts',(35.0423458801,-85.1035862578228,121.210257384038));
#43451=CARTESIAN_POINT('Ctrl Pts',(37.868782298455,-85.2128337534358,121.052308860845));
#43452=CARTESIAN_POINT('Ctrl Pts',(39.3225925665741,-87.6389563438593,120.894360337653));
#43453=CARTESIAN_POINT('Ctrl Pts',(38.0857384506941,-90.1827382969836,120.73641181446));
#43454=CARTESIAN_POINT('Ctrl Pts',(35.2795955041279,-90.5375785237065,120.578463291268));
#43455=CARTESIAN_POINT('Ctrl Pts',(33.448428834545,-88.3818666722405,120.420514768075));
#43456=CARTESIAN_POINT('Ctrl Pts',(34.2524915318856,-85.670066420957,120.262566244883));
#43457=CARTESIAN_POINT('Ctrl Pts',(36.96276928306,-84.8609111752806,120.10461772169));
#43458=CARTESIAN_POINT('Ctrl Pts',(39.1219333076541,-86.6880244570525,119.946669198498));
#43459=CARTESIAN_POINT('Ctrl Pts',(38.7723364062652,-89.4948245096349,119.788720675306));
#43460=CARTESIAN_POINT('Ctrl Pts',(36.2309468959301,-90.7364680335706,119.630772152113));
#43461=CARTESIAN_POINT('Ctrl Pts',(33.8019656255414,-89.2871960948262,119.472823628921));
#43462=CARTESIAN_POINT('Ctrl Pts',(33.6876759062241,-86.4610187600149,119.314875105728));
#43463=CARTESIAN_POINT('Ctrl Pts',(35.9917008149959,-84.8203454156677,119.156926582536));
#43464=CARTESIAN_POINT('Ctrl Pts',(38.6250510094734,-85.8527245134451,118.998978059343));
#43465=CARTESIAN_POINT('Ctrl Pts',(39.2001479732925,-88.622129406846,118.841029536151));
#43466=CARTESIAN_POINT('Ctrl Pts',(37.1955687727307,-90.6176248662799,118.683081012958));
#43467=CARTESIAN_POINT('Ctrl Pts',(34.4288044060203,-90.0299558685653,118.525132489766));
#43468=CARTESIAN_POINT('Ctrl Pts',(33.4083959753712,-87.3919440112382,118.367183966573));
#43469=CARTESIAN_POINT('Ctrl Pts',(35.0595167713852,-85.095394418475,118.209235443381));
#43470=CARTESIAN_POINT('Ctrl Pts',(37.8851457844713,-85.2225187573788,118.051286920188));
#43471=CARTESIAN_POINT('Ctrl Pts',(39.3233711262874,-87.6580572572747,117.893338396996));
#43472=CARTESIAN_POINT('Ctrl Pts',(38.0701976209574,-90.1937812333288,117.735389873803));
#43473=CARTESIAN_POINT('Ctrl Pts',(35.2618395722624,-90.5306268772706,117.577441350611));
#43474=CARTESIAN_POINT('Ctrl Pts',(33.4445498105818,-88.3631864883094,117.419492827419));
#43475=CARTESIAN_POINT('Ctrl Pts',(34.2660096924731,-85.6566123474577,117.261544304226));
#43476=CARTESIAN_POINT('Ctrl Pts',(36.9814265265929,-84.8648729114648,117.103595781034));
#43477=CARTESIAN_POINT('Ctrl Pts',(39.1288144551173,-86.7058142472931,116.945647257841));
#43478=CARTESIAN_POINT('Ctrl Pts',(38.7612021531035,-89.5103108354403,116.787698734649));
#43479=CARTESIAN_POINT('Ctrl Pts',(36.2118925143652,-90.7356109143443,116.629750211456));
#43480=CARTESIAN_POINT('Ctrl Pts',(33.7922670545985,-89.2707721682791,116.471801688264));
#43481=CARTESIAN_POINT('Ctrl Pts',(33.6961265885919,-86.4439193372456,116.313853165071));
#43482=CARTESIAN_POINT('Ctrl Pts',(36.0106387528937,-84.8180739082996,116.155904641879));
#43483=CARTESIAN_POINT('Ctrl Pts',(38.6373057608367,-85.8673404840128,115.997956118686));
#43484=CARTESIAN_POINT('Ctrl Pts',(39.194608522785,-88.6403809721864,115.840007595494));
#43485=CARTESIAN_POINT('Ctrl Pts',(37.1772575740773,-90.6229639004075,115.682059072301));
#43486=CARTESIAN_POINT('Ctrl Pts',(34.4143236649513,-90.0175416251921,115.524110549109));
#43487=CARTESIAN_POINT('Ctrl Pts',(33.4108749399752,-87.3730321103917,115.366162025916));
#43488=CARTESIAN_POINT('Ctrl Pts',(35.0767078395714,-85.0871317039549,115.208213502724));
#43489=CARTESIAN_POINT('Ctrl Pts',(37.9014623376935,-85.2323967818796,115.050264979531));
#43490=CARTESIAN_POINT('Ctrl Pts',(39.3240194419186,-87.6771199160491,114.892316456339));
#43491=CARTESIAN_POINT('Ctrl Pts',(38.0545898909647,-90.2047449936051,114.734367933147));
#43492=CARTESIAN_POINT('Ctrl Pts',(35.2441268507267,-90.5235512309691,114.576419409954));
#43493=CARTESIAN_POINT('Ctrl Pts',(33.4407916834193,-88.3444867087769,114.418470886762));
#43494=CARTESIAN_POINT('Ctrl Pts',(34.27961353928,-85.6432429560481,114.260522363569));
#43495=CARTESIAN_POINT('Ctrl Pts',(37.0000581532135,-84.8689555287672,114.102573840377));
#43496=CARTESIAN_POINT('Ctrl Pts',(39.1355811323492,-86.7236472883622,113.944625317184));
#43497=CARTESIAN_POINT('Ctrl Pts',(38.7499687405001,-89.525725624308,113.786676793992));
#43498=CARTESIAN_POINT('Ctrl Pts',(36.1928440054851,-90.7346313307632,113.628728270799));
#43499=CARTESIAN_POINT('Ctrl Pts',(33.782674153109,-89.2542863708898,113.470779747607));
#43500=CARTESIAN_POINT('Ctrl Pts',(33.7046868865187,-86.426874497148,113.312831224414));
#43501=CARTESIAN_POINT('Ctrl Pts',(36.0295908884562,-84.815924063615,113.154882701222));
#43502=CARTESIAN_POINT('Ctrl Pts',(38.6494664091236,-85.882034833532,112.996934178029));
#43503=CARTESIAN_POINT('Ctrl Pts',(39.1889519938438,-88.658596596109,112.838985654837));
#43504=CARTESIAN_POINT('Ctrl Pts',(37.1589124706636,-90.6281852465259,112.681037131644));
#43505=CARTESIAN_POINT('Ctrl Pts',(34.3999229343891,-90.005034657781,112.523088608452));
#43506=CARTESIAN_POINT('Ctrl Pts',(33.4134752866869,-87.3541365164204,112.365140085259));
#43507=CARTESIAN_POINT('Ctrl Pts',(35.0939516082793,-85.0789795437939,112.207191562067));
#43508=CARTESIAN_POINT('Ctrl Pts',(37.9177151277559,-85.2423793712098,112.049243038874));
#43509=CARTESIAN_POINT('Ctrl Pts',(39.3245453428919,-87.6961863447321,111.891294515682));
#43510=CARTESIAN_POINT('Ctrl Pts',(38.0389120844315,-90.2156083106323,111.733345992489));
#43511=CARTESIAN_POINT('Ctrl Pts',(35.2264599270504,-90.5163619971867,111.575397469297));
#43512=CARTESIAN_POINT('Ctrl Pts',(33.4371537049852,-88.325763183801,111.417448946105));
#43513=CARTESIAN_POINT('Ctrl Pts',(34.2933029504833,-85.6299611905315,111.259500422912));
#43514=CARTESIAN_POINT('Ctrl Pts',(37.0186631812752,-84.8731576955424,111.10155189972));
#43515=CARTESIAN_POINT('Ctrl Pts',(39.1422331641425,-86.7415234106471,110.943603376527));
#43516=CARTESIAN_POINT('Ctrl Pts',(38.7386365811713,-89.5410679656435,110.785654853335));
#43517=CARTESIAN_POINT('Ctrl Pts',(36.1738021791204,-90.7335294570022,110.627706330142));
#43518=CARTESIAN_POINT('Ctrl Pts',(33.7731873047999,-89.2377393172008,110.46975780695));
#43519=CARTESIAN_POINT('Ctrl Pts',(33.7133564525678,-86.4098849743869,110.311809283757));
#43520=CARTESIAN_POINT('Ctrl Pts',(36.0485564380895,-84.8138959542623,110.153860760565));
#43521=CARTESIAN_POINT('Ctrl Pts',(38.6615324530581,-85.8968069649053,109.995912237372));
#43522=CARTESIAN_POINT('Ctrl Pts',(39.1831786216268,-88.6767755213396,109.83796371418));
#43523=CARTESIAN_POINT('Ctrl Pts',(37.1405342138127,-90.6332886965093,109.680015190987));
#43524=CARTESIAN_POINT('Ctrl Pts',(34.3856028189437,-89.9924354700622,109.522066667795));
#43525=CARTESIAN_POINT('Ctrl Pts',(33.4161968856849,-87.3352580315655,109.364118144603));
#43526=CARTESIAN_POINT('Ctrl Pts',(35.1112474131768,-85.0709382270786,109.20616962141));
#43527=CARTESIAN_POINT('Ctrl Pts',(37.9339033886155,-85.2524662101859,109.048221098218));
#43528=CARTESIAN_POINT('Ctrl Pts',(39.3249490048854,-87.7152555591209,108.890272575025));
#43529=CARTESIAN_POINT('Ctrl Pts',(38.0231644418222,-90.2263711438778,108.732324051833));
#43530=CARTESIAN_POINT('Ctrl Pts',(35.2088403645094,-90.5090586345567,108.57437552864));
#43531=CARTESIAN_POINT('Ctrl Pts',(33.4336343081817,-88.3070184083814,108.416427005448));
#43532=CARTESIAN_POINT('Ctrl Pts',(34.3070808932133,-85.6167640547538,108.258478482255));
#43533=CARTESIAN_POINT('Ctrl Pts',(37.0372335803832,-84.8774865269729,108.100529959063));
#43534=CARTESIAN_POINT('Ctrl Pts',(39.1487852146927,-86.7594268870025,107.94258143587));
#43535=CARTESIAN_POINT('Ctrl Pts',(38.7271754184244,-89.5563680570491,107.784632912678));
#43536=CARTESIAN_POINT('Ctrl Pts',(36.1548310102042,-90.7322419299408,107.626684389485));
#43537=CARTESIAN_POINT('Ctrl Pts',(33.7636769376747,-89.2212621009139,107.468735866293));
#43538=CARTESIAN_POINT('Ctrl Pts',(33.7224022240811,-86.3926832021283,107.3107873431));
#43539=CARTESIAN_POINT('Ctrl Pts',(36.0669846992798,-84.812541212222,107.152838819908));
#43540=CARTESIAN_POINT('Ctrl Pts',(38.6746344652086,-85.9105081134349,106.994890296715));
#43541=CARTESIAN_POINT('Ctrl Pts',(39.1749135435619,-88.6972338749877,106.836941773523));
#43542=CARTESIAN_POINT('Ctrl Pts',(37.8096764711453,-89.9855519312418,106.731642758061));
#43543=CARTESIAN_POINT('Ctrl Pts',(37.0051260726582,-90.2006423906074,106.678993250331));
#43544=CARTESIAN_POINT('Ctrl Pts',(38.4092576250256,-86.0121302673453,122.10700224989));
#43545=CARTESIAN_POINT('Ctrl Pts',(38.9902947372386,-86.6917167303241,122.054352742159));
#43546=CARTESIAN_POINT('Ctrl Pts',(39.4147364209601,-88.6618405192673,121.949053726697));
#43547=CARTESIAN_POINT('Ctrl Pts',(37.2773797304845,-90.8232131757403,121.791105203505));
#43548=CARTESIAN_POINT('Ctrl Pts',(34.302488077104,-90.2088412828551,121.633156680312));
#43549=CARTESIAN_POINT('Ctrl Pts',(33.1890206178008,-87.3849393530991,121.47520815712));
#43550=CARTESIAN_POINT('Ctrl Pts',(34.9457163417765,-84.9073965262243,121.317259633928));
#43551=CARTESIAN_POINT('Ctrl Pts',(37.980229376961,-85.0246866047652,121.159311110735));
#43552=CARTESIAN_POINT('Ctrl Pts',(39.5410662599857,-87.6294155057182,121.001362587543));
#43553=CARTESIAN_POINT('Ctrl Pts',(38.2131574087957,-90.3604656171925,120.84341406435));
#43554=CARTESIAN_POINT('Ctrl Pts',(35.2004318103538,-90.7414284743101,120.685465541158));
#43555=CARTESIAN_POINT('Ctrl Pts',(33.2344582995543,-88.4270174120644,120.527517017965));
#43556=CARTESIAN_POINT('Ctrl Pts',(34.0977144904032,-85.5155798301335,120.369568494773));
#43557=CARTESIAN_POINT('Ctrl Pts',(37.0075174888008,-84.6468561876885,120.21161997158));
#43558=CARTESIAN_POINT('Ctrl Pts',(39.3256348662813,-86.6084779083434,120.053671448388));
#43559=CARTESIAN_POINT('Ctrl Pts',(38.9503013376599,-89.6219089876371,119.895722925195));
#43560=CARTESIAN_POINT('Ctrl Pts',(36.2218197958458,-90.9549598335599,119.737774402003));
#43561=CARTESIAN_POINT('Ctrl Pts',(33.6140217646049,-89.3989953826749,119.57982587881));
#43562=CARTESIAN_POINT('Ctrl Pts',(33.4913182638986,-86.3647605042483,119.421877355618));
#43563=CARTESIAN_POINT('Ctrl Pts',(35.9649608951831,-84.6033040576888,119.263928832425));
#43564=CARTESIAN_POINT('Ctrl Pts',(38.7921730834546,-85.7116848474046,119.105980309233));
#43565=CARTESIAN_POINT('Ctrl Pts',(39.4096075397443,-88.6849678104158,118.948031786041));
#43566=CARTESIAN_POINT('Ctrl Pts',(37.2574552129974,-90.8273676691141,118.790083262848));
#43567=CARTESIAN_POINT('Ctrl Pts',(34.28700716699,-90.1964356508463,118.632134739656));
#43568=CARTESIAN_POINT('Ctrl Pts',(33.1914783010623,-87.3642186173953,118.474186216463));
#43569=CARTESIAN_POINT('Ctrl Pts',(34.9641513198614,-84.8986016199879,118.316237693271));
#43570=CARTESIAN_POINT('Ctrl Pts',(37.9977975102101,-85.0350845993988,118.158289170078));
#43571=CARTESIAN_POINT('Ctrl Pts',(39.5419021357137,-87.6499225903166,118.000340646886));
#43572=CARTESIAN_POINT('Ctrl Pts',(38.1964724941422,-90.3723215125058,117.842392123693));
#43573=CARTESIAN_POINT('Ctrl Pts',(35.1813687221669,-90.7339650615165,117.684443600501));
#43574=CARTESIAN_POINT('Ctrl Pts',(33.2302937095768,-88.4069620302165,117.526495077308));
#43575=CARTESIAN_POINT('Ctrl Pts',(34.1122278310353,-85.5011352945534,117.368546554116));
#43576=CARTESIAN_POINT('Ctrl Pts',(37.027548241424,-84.6511095789959,117.210598030923));
#43577=CARTESIAN_POINT('Ctrl Pts',(39.3330225901084,-86.6275773474915,117.052649507731));
#43578=CARTESIAN_POINT('Ctrl Pts',(38.938347402968,-89.6385353858884,116.894700984538));
#43579=CARTESIAN_POINT('Ctrl Pts',(36.20136266868,-90.9540396149241,116.736752461346));
#43580=CARTESIAN_POINT('Ctrl Pts',(33.6036092041957,-89.3813623593836,116.578803938154));
#43581=CARTESIAN_POINT('Ctrl Pts',(33.5003910686625,-86.3464022560491,116.420855414961));
#43582=CARTESIAN_POINT('Ctrl Pts',(35.9852930063309,-84.6008653264748,116.262906891769));
#43583=CARTESIAN_POINT('Ctrl Pts',(38.805330005193,-85.7273768166001,116.104958368576));
#43584=CARTESIAN_POINT('Ctrl Pts',(39.4036602859289,-88.7045630196262,115.947009845384));
#43585=CARTESIAN_POINT('Ctrl Pts',(37.2377959803882,-90.8330997522951,115.789061322191));
#43586=CARTESIAN_POINT('Ctrl Pts',(34.2714603826195,-90.1831074956138,115.631112798999));
#43587=CARTESIAN_POINT('Ctrl Pts',(33.1941397621006,-87.3439144600947,115.473164275806));
#43588=CARTESIAN_POINT('Ctrl Pts',(34.9826079602305,-84.8897306208901,115.315215752614));
#43589=CARTESIAN_POINT('Ctrl Pts',(38.0153152555662,-85.0456898243793,115.157267229421));
#43590=CARTESIAN_POINT('Ctrl Pts',(39.5425981790498,-87.6703886040434,114.999318706229));
#43591=CARTESIAN_POINT('Ctrl Pts',(38.1797157541692,-90.3840924029661,114.841370183036));
#43592=CARTESIAN_POINT('Ctrl Pts',(35.1623520253682,-90.7263685202339,114.683421659844));
#43593=CARTESIAN_POINT('Ctrl Pts',(33.2262589165814,-88.3868856101783,114.525473136651));
#43594=CARTESIAN_POINT('Ctrl Pts',(34.1268331659355,-85.4867816751897,114.367524613459));
#43595=CARTESIAN_POINT('Ctrl Pts',(37.0475514912688,-84.6554927504486,114.209576090266));
#43596=CARTESIAN_POINT('Ctrl Pts',(39.3402874166341,-86.6467232215078,114.051627567074));
#43597=CARTESIAN_POINT('Ctrl Pts',(38.9262870089137,-89.6550849807952,113.893679043881));
#43598=CARTESIAN_POINT('Ctrl Pts',(36.1809118465345,-90.9529879163518,113.735730520689));
#43599=CARTESIAN_POINT('Ctrl Pts',(33.5933100924145,-89.3636629104421,113.577781997497));
#43600=CARTESIAN_POINT('Ctrl Pts',(33.5095815586644,-86.3281026087889,113.419833474304));
#43601=CARTESIAN_POINT('Ctrl Pts',(36.0056403603473,-84.5985572145086,113.261884951112));
#43602=CARTESIAN_POINT('Ctrl Pts',(38.818385896174,-85.7431529348491,113.103936427919));
#43603=CARTESIAN_POINT('Ctrl Pts',(39.397587334599,-88.7241196414834,112.945987904727));
#43604=CARTESIAN_POINT('Ctrl Pts',(37.2181003470178,-90.83870548351,112.788039381534));
#43605=CARTESIAN_POINT('Ctrl Pts',(34.2559994989699,-90.1696797901849,112.630090858342));
#43606=CARTESIAN_POINT('Ctrl Pts',(33.1969315411555,-87.3236278101488,112.472142335149));
#43607=CARTESIAN_POINT('Ctrl Pts',(35.0011211808287,-84.8809783149429,112.314193811957));
#43608=CARTESIAN_POINT('Ctrl Pts',(38.0327645436458,-85.0564073120434,112.156245288764));
#43609=CARTESIAN_POINT('Ctrl Pts',(39.5431627958047,-87.6908586652121,111.998296765572));
#43610=CARTESIAN_POINT('Ctrl Pts',(38.1628837787605,-90.3957554557452,111.840348242379));
#43611=CARTESIAN_POINT('Ctrl Pts',(35.143384497976,-90.7186500293867,111.682399719187));
#43612=CARTESIAN_POINT('Ctrl Pts',(33.2223531174244,-88.3667836966043,111.524451195994));
#43613=CARTESIAN_POINT('Ctrl Pts',(34.1415303643124,-85.4725221325625,111.366502672802));
#43614=CARTESIAN_POINT('Ctrl Pts',(37.0675261844218,-84.6600042723681,111.208554149609));
#43615=CARTESIAN_POINT('Ctrl Pts',(39.3474291577524,-86.6659153482933,111.050605626417));
#43616=CARTESIAN_POINT('Ctrl Pts',(38.914120598597,-89.6715567947269,110.892657103225));
#43617=CARTESIAN_POINT('Ctrl Pts',(36.1604681988578,-90.9518049248403,110.734708580032));
#43618=CARTESIAN_POINT('Ctrl Pts',(33.5831248412375,-89.3458976956341,110.57676005684));
#43619=CARTESIAN_POINT('Ctrl Pts',(33.51888936089,-86.3098623512175,110.418811533647));
#43620=CARTESIAN_POINT('Ctrl Pts',(36.0260021159516,-84.5963797997868,110.260863010455));
#43621=CARTESIAN_POINT('Ctrl Pts',(38.8313402182188,-85.7590125610974,110.102914487262));
#43622=CARTESIAN_POINT('Ctrl Pts',(39.391388938224,-88.743636862964,109.94496596407));
#43623=CARTESIAN_POINT('Ctrl Pts',(37.1983691195202,-90.8441846393115,109.787017440877));
#43624=CARTESIAN_POINT('Ctrl Pts',(34.2406251651613,-90.1561530753728,109.629068917685));
#43625=CARTESIAN_POINT('Ctrl Pts',(33.1998534988484,-87.3033595288585,109.471120394492));
#43626=CARTESIAN_POINT('Ctrl Pts',(35.0196902684171,-84.8723450125151,109.3131718713));
#43627=CARTESIAN_POINT('Ctrl Pts',(38.0501445520112,-85.0672367240047,109.155223348108));
#43628=CARTESIAN_POINT('Ctrl Pts',(39.5435961745898,-87.7113317171647,108.997274824915));
#43629=CARTESIAN_POINT('Ctrl Pts',(38.1459768260829,-90.4073106273269,108.839326301723));
#43630=CARTESIAN_POINT('Ctrl Pts',(35.1244678183516,-90.7108090077533,108.68137777853));
#43631=CARTESIAN_POINT('Ctrl Pts',(33.2185746296415,-88.3466589681714,108.523429255338));
#43632=CARTESIAN_POINT('Ctrl Pts',(34.1563226117307,-85.458353449947,108.365480732145));
#43633=CARTESIAN_POINT('Ctrl Pts',(37.0874636993066,-84.6646517837423,108.207532208953));
#43634=CARTESIAN_POINT('Ctrl Pts',(39.3544635572078,-86.6851368429016,108.04958368576));
#43635=CARTESIAN_POINT('Ctrl Pts',(38.9018156878874,-89.6879832483728,107.891635162568));
#43636=CARTESIAN_POINT('Ctrl Pts',(36.1401004102902,-90.9504226126024,107.733686639375));
#43637=CARTESIAN_POINT('Ctrl Pts',(33.572914339836,-89.3282074595185,107.575738116183));
#43638=CARTESIAN_POINT('Ctrl Pts',(33.5286010640765,-86.2913942187635,107.41778959299));
#43639=CARTESIAN_POINT('Ctrl Pts',(36.0457870290084,-84.5949253243372,107.259841069798));
#43640=CARTESIAN_POINT('Ctrl Pts',(38.8454067743952,-85.7737223608792,107.101892546605));
#43641=CARTESIAN_POINT('Ctrl Pts',(39.3825154015819,-88.76560131984,106.943944023413));
#43642=CARTESIAN_POINT('Ctrl Pts',(37.916772296426,-90.1487627841414,106.838645007951));
#43643=CARTESIAN_POINT('Ctrl Pts',(37.052992500844,-90.379687774511,106.78599550022));
#43644=CARTESIAN_POINT('Ctrl Pts',(38.5501231787026,-85.8916921494934,122.21400449978));
#43645=CARTESIAN_POINT('Ctrl Pts',(39.1710020168071,-86.6178778692294,122.161354992049));
#43646=CARTESIAN_POINT('Ctrl Pts',(39.6245476748949,-88.7230930840409,122.056055976587));
#43647=CARTESIAN_POINT('Ctrl Pts',(37.3406323952962,-91.0326711048844,121.898107453395));
#43648=CARTESIAN_POINT('Ctrl Pts',(34.1617523643761,-90.37617171956,121.740158930202));
#43649=CARTESIAN_POINT('Ctrl Pts',(32.9719344201038,-87.3586347804996,121.58221040701));
#43650=CARTESIAN_POINT('Ctrl Pts',(34.8490868034529,-84.7112067946259,121.424261883817));
#43651=CARTESIAN_POINT('Ctrl Pts',(38.0916764554671,-84.8365394560944,121.266313360625));
#43652=CARTESIAN_POINT('Ctrl Pts',(39.7595399533973,-87.6198746675772,121.108364837432));
#43653=CARTESIAN_POINT('Ctrl Pts',(38.3405763668972,-90.5381929374012,120.95041631424));
#43654=CARTESIAN_POINT('Ctrl Pts',(35.1212681165797,-90.9452784249139,120.792467791047));
#43655=CARTESIAN_POINT('Ctrl Pts',(33.0204877645637,-88.4721681518882,120.634519267855));
#43656=CARTESIAN_POINT('Ctrl Pts',(33.9429374489209,-85.3610932393102,120.476570744662));
#43657=CARTESIAN_POINT('Ctrl Pts',(37.0522656945416,-84.4328012000962,120.31862222147));
#43658=CARTESIAN_POINT('Ctrl Pts',(39.5293364249085,-86.5289313596344,120.160673698277));
#43659=CARTESIAN_POINT('Ctrl Pts',(39.1282662690547,-89.7489934656392,120.002725175085));
#43660=CARTESIAN_POINT('Ctrl Pts',(36.2126926957615,-91.1734516335492,119.844776651893));
#43661=CARTESIAN_POINT('Ctrl Pts',(33.4260779036684,-89.5107946705236,119.6868281287));
#43662=CARTESIAN_POINT('Ctrl Pts',(33.2949606215731,-86.2685022484816,119.528879605508));
#43663=CARTESIAN_POINT('Ctrl Pts',(35.9382209753702,-84.38626269971,119.370931082315));
#43664=CARTESIAN_POINT('Ctrl Pts',(38.9592951574358,-85.5706451813641,119.212982559123));
#43665=CARTESIAN_POINT('Ctrl Pts',(39.619067106196,-88.7478062139855,119.05503403593));
#43666=CARTESIAN_POINT('Ctrl Pts',(37.3193416532641,-91.0371104719483,118.897085512738));
#43667=CARTESIAN_POINT('Ctrl Pts',(34.1452099279596,-90.3629154331271,118.739136989545));
#43668=CARTESIAN_POINT('Ctrl Pts',(32.9745606267535,-87.3364932235525,118.581188466353));
#43669=CARTESIAN_POINT('Ctrl Pts',(34.8687858683375,-84.7018088215008,118.42323994316));
#43670=CARTESIAN_POINT('Ctrl Pts',(38.1104492359489,-84.8476504414188,118.265291419968));
#43671=CARTESIAN_POINT('Ctrl Pts',(39.7604331451399,-87.6417879233585,118.107342896775));
#43672=CARTESIAN_POINT('Ctrl Pts',(38.322747367327,-90.5508617916828,117.949394373583));
#43673=CARTESIAN_POINT('Ctrl Pts',(35.1008978720714,-90.9373032457623,117.79144585039));
#43674=CARTESIAN_POINT('Ctrl Pts',(33.0160376085718,-88.4507375721237,117.633497327198));
#43675=CARTESIAN_POINT('Ctrl Pts',(33.9584459695975,-85.3456582416492,117.475548804005));
#43676=CARTESIAN_POINT('Ctrl Pts',(37.0736699562551,-84.4373462465268,117.317600280813));
#43677=CARTESIAN_POINT('Ctrl Pts',(39.5372307250997,-86.5493404476901,117.159651757621));
#43678=CARTESIAN_POINT('Ctrl Pts',(39.1154926528324,-89.7667599363363,117.001703234428));
#43679=CARTESIAN_POINT('Ctrl Pts',(36.190832822995,-91.172468315504,116.843754711236));
#43680=CARTESIAN_POINT('Ctrl Pts',(33.4149513537928,-89.491952550488,116.685806188043));
#43681=CARTESIAN_POINT('Ctrl Pts',(33.3046555487331,-86.2488851748525,116.527857664851));
#43682=CARTESIAN_POINT('Ctrl Pts',(35.9599472597682,-84.38365674465,116.369909141658));
#43683=CARTESIAN_POINT('Ctrl Pts',(38.9733542495494,-85.5874131491874,116.211960618466));
#43684=CARTESIAN_POINT('Ctrl Pts',(39.6127120490728,-88.7687450670661,116.054012095273));
#43685=CARTESIAN_POINT('Ctrl Pts',(37.2983343866991,-91.0432356041825,115.896063572081));
#43686=CARTESIAN_POINT('Ctrl Pts',(34.1285971002877,-90.3486733660357,115.738115048889));
#43687=CARTESIAN_POINT('Ctrl Pts',(32.977404584226,-87.3147968097978,115.580166525696));
#43688=CARTESIAN_POINT('Ctrl Pts',(34.8885080808896,-84.6923295378252,115.422218002504));
#43689=CARTESIAN_POINT('Ctrl Pts',(38.1291681734389,-84.858982866879,115.264269479311));
#43690=CARTESIAN_POINT('Ctrl Pts',(39.7611769161809,-87.6636572920377,115.106320956119));
#43691=CARTESIAN_POINT('Ctrl Pts',(38.3048416173737,-90.5634398123269,114.948372432926));
#43692=CARTESIAN_POINT('Ctrl Pts',(35.0805772000098,-90.9291858094989,114.790423909734));
#43693=CARTESIAN_POINT('Ctrl Pts',(33.0117261497435,-88.4292845115796,114.632475386541));
#43694=CARTESIAN_POINT('Ctrl Pts',(33.974052792591,-85.3303203943313,114.474526863349));
#43695=CARTESIAN_POINT('Ctrl Pts',(37.0950448293241,-84.4420299721299,114.316578340156));
#43696=CARTESIAN_POINT('Ctrl Pts',(39.5449937009191,-86.5697991546535,114.158629816964));
#43697=CARTESIAN_POINT('Ctrl Pts',(39.1026052773274,-89.7844443372823,114.000681293771));
#43698=CARTESIAN_POINT('Ctrl Pts',(36.1689796875839,-91.1713445019405,113.842732770579));
#43699=CARTESIAN_POINT('Ctrl Pts',(33.40394603172,-89.4730394499943,113.684784247386));
#43700=CARTESIAN_POINT('Ctrl Pts',(33.3144762308101,-86.2293307204299,113.526835724194));
#43701=CARTESIAN_POINT('Ctrl Pts',(35.9816898322384,-84.3811903654021,113.368887201001));
#43702=CARTESIAN_POINT('Ctrl Pts',(38.9873053832245,-85.6042710361663,113.210938677809));
#43703=CARTESIAN_POINT('Ctrl Pts',(39.6062226753541,-88.7896426868578,113.052990154617));
#43704=CARTESIAN_POINT('Ctrl Pts',(37.277288223372,-91.0492257204941,112.895041631424));
#43705=CARTESIAN_POINT('Ctrl Pts',(34.1120760635507,-90.3343249225886,112.737093108232));
#43706=CARTESIAN_POINT('Ctrl Pts',(32.980387795624,-87.2931191038772,112.579144585039));
#43707=CARTESIAN_POINT('Ctrl Pts',(34.9082907533782,-84.6829770860919,112.421196061847));
#43708=CARTESIAN_POINT('Ctrl Pts',(38.1478139595356,-84.8704352528771,112.263247538654));
#43709=CARTESIAN_POINT('Ctrl Pts',(39.7617802487174,-87.685530985692,112.105299015462));
#43710=CARTESIAN_POINT('Ctrl Pts',(38.2868554730895,-90.5759026008582,111.947350492269));
#43711=CARTESIAN_POINT('Ctrl Pts',(35.0603090689016,-90.9209380615865,111.789401969077));
#43712=CARTESIAN_POINT('Ctrl Pts',(33.0075525298637,-88.4078042094077,111.631453445884));
#43713=CARTESIAN_POINT('Ctrl Pts',(33.9897577781416,-85.3150830745935,111.473504922692));
#43714=CARTESIAN_POINT('Ctrl Pts',(37.1163891875685,-84.4468508491938,111.315556399499));
#43715=CARTESIAN_POINT('Ctrl Pts',(39.5526251513623,-86.5903072859396,111.157607876307));
#43716=CARTESIAN_POINT('Ctrl Pts',(39.0896046160226,-89.8020456238101,110.999659353114));
#43717=CARTESIAN_POINT('Ctrl Pts',(36.1471342185952,-91.1700803926785,110.841710829922));
#43718=CARTESIAN_POINT('Ctrl Pts',(33.393062377675,-89.4540560740673,110.683762306729));
#43719=CARTESIAN_POINT('Ctrl Pts',(33.3244222692122,-86.2098397280481,110.525813783537));
#43720=CARTESIAN_POINT('Ctrl Pts',(36.0034477938138,-84.3788636453113,110.367865260344));
#43721=CARTESIAN_POINT('Ctrl Pts',(39.0011479833795,-85.6212181572896,110.209916737152));
#43722=CARTESIAN_POINT('Ctrl Pts',(39.5995992548212,-88.8104982045884,110.05196821396));
#43723=CARTESIAN_POINT('Ctrl Pts',(37.2562040252276,-91.0550805821136,109.894019690767));
#43724=CARTESIAN_POINT('Ctrl Pts',(34.095647511379,-90.3198706806834,109.736071167575));
#43725=CARTESIAN_POINT('Ctrl Pts',(32.9835101120118,-87.2714610261512,109.578122644382));
#43726=CARTESIAN_POINT('Ctrl Pts',(34.9281331236574,-84.6737517979516,109.42017412119));
#43727=CARTESIAN_POINT('Ctrl Pts',(38.166385715407,-84.8820072378236,109.262225597997));
#43728=CARTESIAN_POINT('Ctrl Pts',(39.7622433442942,-87.7074078752085,109.104277074805));
#43729=CARTESIAN_POINT('Ctrl Pts',(38.2687892103436,-90.5882501107759,108.946328551612));
#43730=CARTESIAN_POINT('Ctrl Pts',(35.0400952721938,-90.91255938095,108.78838002842));
#43731=CARTESIAN_POINT('Ctrl Pts',(33.0035149511013,-88.3862995279612,108.630431505227));
#43732=CARTESIAN_POINT('Ctrl Pts',(34.0055643302481,-85.2999428451404,108.472482982035));
#43733=CARTESIAN_POINT('Ctrl Pts',(37.1376938182299,-84.4518170405117,108.314534458842));
#43734=CARTESIAN_POINT('Ctrl Pts',(39.5601418997229,-86.6108467988005,108.15658593565));
#43735=CARTESIAN_POINT('Ctrl Pts',(39.0764559573505,-89.8195984396968,107.998637412457));
#43736=CARTESIAN_POINT('Ctrl Pts',(36.1253698103761,-91.1686032952638,107.840688889265));
#43737=CARTESIAN_POINT('Ctrl Pts',(33.3821517419973,-89.4351528181232,107.682740366073));
#43738=CARTESIAN_POINT('Ctrl Pts',(33.3347999040718,-86.1901052353986,107.52479184288));
#43739=CARTESIAN_POINT('Ctrl Pts',(36.0245893587371,-84.3773094364523,107.366843319688));
#43740=CARTESIAN_POINT('Ctrl Pts',(39.0161790835818,-85.6369366083236,107.208894796495));
#43741=CARTESIAN_POINT('Ctrl Pts',(39.590117259602,-88.8339687646923,107.050946273303));
#43742=CARTESIAN_POINT('Ctrl Pts',(38.0238681217068,-90.311973637041,106.945647257841));
#43743=CARTESIAN_POINT('Ctrl Pts',(37.1008589290299,-90.5587331584145,106.89299775011));
#43744=CARTESIAN_POINT('Ctrl Pts',(38.6909887323796,-85.7712540316415,122.321006749669));
#43745=CARTESIAN_POINT('Ctrl Pts',(39.3517092963755,-86.5440390081348,122.268357241939));
#43746=CARTESIAN_POINT('Ctrl Pts',(39.8343589288296,-88.7843456488144,122.163058226477));
#43747=CARTESIAN_POINT('Ctrl Pts',(37.4038850601078,-91.2421290340287,122.005109703285));
#43748=CARTESIAN_POINT('Ctrl Pts',(34.0210166516482,-90.5435021562648,121.847161180092));
#43749=CARTESIAN_POINT('Ctrl Pts',(32.7548482224067,-87.3323302079001,121.6892126569));
#43750=CARTESIAN_POINT('Ctrl Pts',(34.7524572651294,-84.5150170630276,121.531264133707));
#43751=CARTESIAN_POINT('Ctrl Pts',(38.2031235339731,-84.6483923074236,121.373315610515));
#43752=CARTESIAN_POINT('Ctrl Pts',(39.9780136468089,-87.6103338294361,121.215367087322));
#43753=CARTESIAN_POINT('Ctrl Pts',(38.4679953249988,-90.71592025761,121.05741856413));
#43754=CARTESIAN_POINT('Ctrl Pts',(35.0421044228056,-91.1491283755177,120.899470040937));
#43755=CARTESIAN_POINT('Ctrl Pts',(32.806517229573,-88.517318891712,120.741521517745));
#43756=CARTESIAN_POINT('Ctrl Pts',(33.7881604074385,-85.2066066484868,120.583572994552));
#43757=CARTESIAN_POINT('Ctrl Pts',(37.0970139002824,-84.2187462125039,120.42562447136));
#43758=CARTESIAN_POINT('Ctrl Pts',(39.7330379835356,-86.4493848109254,120.267675948167));
#43759=CARTESIAN_POINT('Ctrl Pts',(39.3062312004495,-89.8760779436413,120.109727424975));
#43760=CARTESIAN_POINT('Ctrl Pts',(36.2035655956772,-91.3919434335384,119.951778901782));
#43761=CARTESIAN_POINT('Ctrl Pts',(33.2381340427318,-89.6225939583723,119.79383037859));
#43762=CARTESIAN_POINT('Ctrl Pts',(33.0986029792476,-86.1722439927149,119.635881855398));
#43763=CARTESIAN_POINT('Ctrl Pts',(35.9114810555574,-84.1692213417312,119.477933332205));
#43764=CARTESIAN_POINT('Ctrl Pts',(39.1264172314171,-85.4296055153237,119.319984809012));
#43765=CARTESIAN_POINT('Ctrl Pts',(39.8285266726477,-88.8106446175552,119.16203628582));
#43766=CARTESIAN_POINT('Ctrl Pts',(37.3812280935308,-91.2468532747826,119.004087762628));
#43767=CARTESIAN_POINT('Ctrl Pts',(34.0034126889292,-90.529395215408,118.846139239435));
#43768=CARTESIAN_POINT('Ctrl Pts',(32.7576429524446,-87.3087678297098,118.688190716243));
#43769=CARTESIAN_POINT('Ctrl Pts',(34.7734204168137,-84.5050160230137,118.53024219305));
#43770=CARTESIAN_POINT('Ctrl Pts',(38.2231009616876,-84.6602162834389,118.372293669858));
#43771=CARTESIAN_POINT('Ctrl Pts',(39.9789641545662,-87.6336532564003,118.214345146665));
#43772=CARTESIAN_POINT('Ctrl Pts',(38.4490222405119,-90.7294020708598,118.056396623473));
#43773=CARTESIAN_POINT('Ctrl Pts',(35.0204270219759,-91.1406414300081,117.89844810028));
#43774=CARTESIAN_POINT('Ctrl Pts',(32.8017815075667,-88.4945131140308,117.740499577088));
#43775=CARTESIAN_POINT('Ctrl Pts',(33.8046641081597,-85.1901811887448,117.582551053895));
#43776=CARTESIAN_POINT('Ctrl Pts',(37.1197916710861,-84.2235829140579,117.424602530703));
#43777=CARTESIAN_POINT('Ctrl Pts',(39.7414388600909,-86.4711035478885,117.26665400751));
#43778=CARTESIAN_POINT('Ctrl Pts',(39.2926379026969,-89.8949844867843,117.108705484318));
#43779=CARTESIAN_POINT('Ctrl Pts',(36.1803029773098,-91.3908970160839,116.950756961125));
#43780=CARTESIAN_POINT('Ctrl Pts',(33.22629350339,-89.6025427415926,116.792808437933));
#43781=CARTESIAN_POINT('Ctrl Pts',(33.1089200288037,-86.1513680936557,116.634859914741));
#43782=CARTESIAN_POINT('Ctrl Pts',(35.9346015132054,-84.1664481628253,116.476911391548));
#43783=CARTESIAN_POINT('Ctrl Pts',(39.1413784939057,-85.4474494817745,116.318962868356));
#43784=CARTESIAN_POINT('Ctrl Pts',(39.8217638122167,-88.8329271145059,116.161014345163));
#43785=CARTESIAN_POINT('Ctrl Pts',(37.35887279301,-91.2533714560701,116.003065821971));
#43786=CARTESIAN_POINT('Ctrl Pts',(33.9857338179559,-90.5142392364574,115.845117298778));
#43787=CARTESIAN_POINT('Ctrl Pts',(32.7606694063514,-87.2856791595006,115.687168775586));
#43788=CARTESIAN_POINT('Ctrl Pts',(34.7944082015486,-84.4949284547604,115.529220252393));
#43789=CARTESIAN_POINT('Ctrl Pts',(38.2430210913116,-84.6722759093786,115.371271729201));
#43790=CARTESIAN_POINT('Ctrl Pts',(39.979755653312,-87.6569259800321,115.213323206008));
#43791=CARTESIAN_POINT('Ctrl Pts',(38.4299674805782,-90.7427872216878,115.055374682816));
#43792=CARTESIAN_POINT('Ctrl Pts',(34.9988023746513,-91.1320030987637,114.897426159623));
#43793=CARTESIAN_POINT('Ctrl Pts',(32.7971933829057,-88.471683412981,114.739477636431));
#43794=CARTESIAN_POINT('Ctrl Pts',(33.8212724192465,-85.1738591134728,114.581529113239));
#43795=CARTESIAN_POINT('Ctrl Pts',(37.1425381673794,-84.2285671938113,114.423580590046));
#43796=CARTESIAN_POINT('Ctrl Pts',(39.749699985204,-86.4928750877993,114.265632066854));
#43797=CARTESIAN_POINT('Ctrl Pts',(39.278923545741,-89.9138036937695,114.107683543661));
#43798=CARTESIAN_POINT('Ctrl Pts',(36.1570475286333,-91.3897010875291,113.949735020469));
#43799=CARTESIAN_POINT('Ctrl Pts',(33.2145819710255,-89.5824159895466,113.791786497276));
#43800=CARTESIAN_POINT('Ctrl Pts',(33.1193709029558,-86.1305588320708,113.633837974084));
#43801=CARTESIAN_POINT('Ctrl Pts',(35.9577393041295,-84.1638235162957,113.475889450891));
#43802=CARTESIAN_POINT('Ctrl Pts',(39.1562248702749,-85.4653891374834,113.317940927699));
#43803=CARTESIAN_POINT('Ctrl Pts',(39.8148580161093,-88.8551657322322,113.159992404506));
#43804=CARTESIAN_POINT('Ctrl Pts',(37.3364760997262,-91.2597459574781,113.002043881314));
#43805=CARTESIAN_POINT('Ctrl Pts',(33.9681526281314,-90.4989700549925,112.844095358121));
#43806=CARTESIAN_POINT('Ctrl Pts',(32.7638440500926,-87.2626103976056,112.686146834929));
#43807=CARTESIAN_POINT('Ctrl Pts',(34.8154603259275,-84.484975857241,112.528198311736));
#43808=CARTESIAN_POINT('Ctrl Pts',(38.2628633754255,-84.6844631937108,112.370249788544));
#43809=CARTESIAN_POINT('Ctrl Pts',(39.9803977016302,-87.6802033061719,112.212301265351));
#43810=CARTESIAN_POINT('Ctrl Pts',(38.4108271674185,-90.7560497459711,112.054352742159));
#43811=CARTESIAN_POINT('Ctrl Pts',(34.9772336398273,-91.1232260937864,111.896404218966));
#43812=CARTESIAN_POINT('Ctrl Pts',(32.792751942303,-88.448824722211,111.738455695774));
#43813=CARTESIAN_POINT('Ctrl Pts',(33.8379851919707,-85.1576440166245,111.580507172582));
#43814=CARTESIAN_POINT('Ctrl Pts',(37.1652521907151,-84.2336974260193,111.422558649389));
#43815=CARTESIAN_POINT('Ctrl Pts',(39.7578211449723,-86.5146992235859,111.264610126197));
#43816=CARTESIAN_POINT('Ctrl Pts',(39.2650886334483,-89.9325344528934,111.106661603004));
#43817=CARTESIAN_POINT('Ctrl Pts',(36.1338002383326,-91.3883558605165,110.948713079812));
#43818=CARTESIAN_POINT('Ctrl Pts',(33.2029999141126,-89.5622144525007,110.790764556619));
#43819=CARTESIAN_POINT('Ctrl Pts',(33.1299551775344,-86.1098171048787,110.632816033427));
#43820=CARTESIAN_POINT('Ctrl Pts',(35.9808934716759,-84.1613474908357,110.474867510234));
#43821=CARTESIAN_POINT('Ctrl Pts',(39.1709557485403,-85.4834237534817,110.316918987042));
#43822=CARTESIAN_POINT('Ctrl Pts',(39.8078095714184,-88.8773595462129,110.158970463849));
#43823=CARTESIAN_POINT('Ctrl Pts',(37.3140389309351,-91.2659765249159,110.001021940657));
#43824=CARTESIAN_POINT('Ctrl Pts',(33.9506698575966,-90.4835882859939,109.843073417465));
#43825=CARTESIAN_POINT('Ctrl Pts',(32.7671667251752,-87.2395625234441,109.685124894272));
#43826=CARTESIAN_POINT('Ctrl Pts',(34.8365759788977,-84.4751585833882,109.527176371079));
#43827=CARTESIAN_POINT('Ctrl Pts',(38.2826268788027,-84.6967777516425,109.369227847887));
#43828=CARTESIAN_POINT('Ctrl Pts',(39.9808905139985,-87.7034840332521,109.211279324694));
#43829=CARTESIAN_POINT('Ctrl Pts',(38.3916015946044,-90.7691895942252,109.053330801502));
#43830=CARTESIAN_POINT('Ctrl Pts',(34.9557227260359,-91.1143097541466,108.89538227831));
#43831=CARTESIAN_POINT('Ctrl Pts',(32.7884552725611,-88.4259400877512,108.737433755117));
#43832=CARTESIAN_POINT('Ctrl Pts',(33.8548060487655,-85.1415322403337,108.579485231925));
#43833=CARTESIAN_POINT('Ctrl Pts',(37.1879239371534,-84.238982297281,108.421536708732));
#43834=CARTESIAN_POINT('Ctrl Pts',(39.7658202422379,-86.5365567546996,108.26358818554));
#43835=CARTESIAN_POINT('Ctrl Pts',(39.2510962268136,-89.9512136310206,108.105639662347));
#43836=CARTESIAN_POINT('Ctrl Pts',(36.1106392104622,-91.3867839779253,107.947691139155));
#43837=CARTESIAN_POINT('Ctrl Pts',(33.1913891441585,-89.5420981767279,107.789742615962));
#43838=CARTESIAN_POINT('Ctrl Pts',(33.1409987440672,-86.0888162520338,107.63179409277));
#43839=CARTESIAN_POINT('Ctrl Pts',(36.0033916884657,-84.1596935485673,107.473845569577));
#43840=CARTESIAN_POINT('Ctrl Pts',(39.1869513927685,-85.500150855768,107.315897046385));
#43841=CARTESIAN_POINT('Ctrl Pts',(39.797719117622,-88.9023362095446,107.157948523192));
#43842=CARTESIAN_POINT('Ctrl Pts',(38.1309639469875,-90.4751844899406,107.052649507731));
#43843=CARTESIAN_POINT('Ctrl Pts',(37.1487253572158,-90.7377785423181,107.));
#43844=CARTESIAN_POINT('Ctrl Pts',(38.2683920713486,-86.1325683851972,122.));
#43845=CARTESIAN_POINT('Ctrl Pts',(38.3300002507757,-86.1904649458245,122.));
#43846=CARTESIAN_POINT('Ctrl Pts',(38.3882392757579,-86.251512267457,122.));
#43847=CARTESIAN_POINT('Ctrl Pts',(38.4431115334664,-86.315325530903,122.));
#43848=CARTESIAN_POINT('Ctrl Pts',(38.4994367220781,-86.3808284689928,122.));
#43849=CARTESIAN_POINT('Ctrl Pts',(38.5522149264209,-86.4492461953977,122.));
#43850=CARTESIAN_POINT('Ctrl Pts',(38.6014232205322,-86.5202110570223,122.));
#43851=CARTESIAN_POINT('Ctrl Pts',(38.651981111331,-86.5931222153823,122.));
#43852=CARTESIAN_POINT('Ctrl Pts',(38.6987711210245,-86.6687226978473,122.));
#43853=CARTESIAN_POINT('Ctrl Pts',(38.7417343172596,-86.7466567430807,122.));
#43854=CARTESIAN_POINT('Ctrl Pts',(38.7606443000318,-86.7809589268538,122.));
#43855=CARTESIAN_POINT('Ctrl Pts',(38.7788124429666,-86.8157136817185,122.));
#43856=CARTESIAN_POINT('Ctrl Pts',(38.7962312959641,-86.850892750047,122.));
#43857=CARTESIAN_POINT('Ctrl Pts',(38.8061621411259,-86.8709490580347,122.));
#43858=CARTESIAN_POINT('Ctrl Pts',(38.815849410692,-86.8911433045237,122.));
#43859=CARTESIAN_POINT('Ctrl Pts',(38.8252914897478,-86.9114704014436,122.));
#43860=CARTESIAN_POINT('Ctrl Pts',(38.8337970736902,-86.9297813929251,122.));
#43861=CARTESIAN_POINT('Ctrl Pts',(38.8421060671472,-86.9482059164998,122.));
#43862=CARTESIAN_POINT('Ctrl Pts',(38.8502036291305,-86.9667084981428,122.));
#43863=CARTESIAN_POINT('Ctrl Pts',(38.8867652309718,-87.0502501893895,122.));
#43864=CARTESIAN_POINT('Ctrl Pts',(38.9190666540545,-87.1354754242206,122.));
#43865=CARTESIAN_POINT('Ctrl Pts',(38.947082863758,-87.2219854243391,122.));
#43866=CARTESIAN_POINT('Ctrl Pts',(38.9755621712229,-87.3099254033098,122.));
#43867=CARTESIAN_POINT('Ctrl Pts',(38.9996139217682,-87.3991937270396,122.));
#43868=CARTESIAN_POINT('Ctrl Pts',(39.0191727436887,-87.4894086379833,122.));
#43869=CARTESIAN_POINT('Ctrl Pts',(39.0381412062379,-87.5769005210103,122.));
#43870=CARTESIAN_POINT('Ctrl Pts',(39.0528840306109,-87.6652836278016,122.));
#43871=CARTESIAN_POINT('Ctrl Pts',(39.0633008450673,-87.7542316018242,122.));
#43872=CARTESIAN_POINT('Ctrl Pts',(39.0676696750207,-87.791536535576,122.));
#43873=CARTESIAN_POINT('Ctrl Pts',(39.0712770535737,-87.8289410203567,122.));
#43874=CARTESIAN_POINT('Ctrl Pts',(39.0741132412595,-87.8664215984214,122.));
#43875=CARTESIAN_POINT('Ctrl Pts',(39.0758923650537,-87.8899329438063,122.));
#43876=CARTESIAN_POINT('Ctrl Pts',(39.0773679986009,-87.9134742372075,122.));
#43877=CARTESIAN_POINT('Ctrl Pts',(39.0785374418203,-87.9370397212164,122.));
#43878=CARTESIAN_POINT('Ctrl Pts',(39.0792218231253,-87.950830708611,122.));
#43879=CARTESIAN_POINT('Ctrl Pts',(39.0798010498032,-87.964625034357,122.));
#43880=CARTESIAN_POINT('Ctrl Pts',(39.0802746210619,-87.9784137075555,122.));
#43881=CARTESIAN_POINT('Ctrl Pts',(39.0836019902155,-88.0752945993602,122.));
#43882=CARTESIAN_POINT('Ctrl Pts',(39.0817234464995,-88.172010484153,122.));
#43883=CARTESIAN_POINT('Ctrl Pts',(39.074574609124,-88.2681415945912,122.));
#43884=CARTESIAN_POINT('Ctrl Pts',(39.0674257717486,-88.3642727050294,122.));
#43885=CARTESIAN_POINT('Ctrl Pts',(39.0550070710252,-88.4598200851495,122.));
#43886=CARTESIAN_POINT('Ctrl Pts',(39.0372016632323,-88.5543827530839,122.));
#43887=CARTESIAN_POINT('Ctrl Pts',(39.0201436337382,-88.6449761726466,122.));
#43888=CARTESIAN_POINT('Ctrl Pts',(38.9981417504386,-88.7346667799934,122.));
#43889=CARTESIAN_POINT('Ctrl Pts',(38.9714706220827,-88.8232152361145,122.));
#43890=CARTESIAN_POINT('Ctrl Pts',(38.9626012728804,-88.852661578548,122.));
#43891=CARTESIAN_POINT('Ctrl Pts',(38.9532151392587,-88.8819815788975,122.));
#43892=CARTESIAN_POINT('Ctrl Pts',(38.9433210712961,-88.9111662610406,122.));
#43893=CARTESIAN_POINT('Ctrl Pts',(38.9340007339025,-88.9386586014335,122.));
#43894=CARTESIAN_POINT('Ctrl Pts',(38.9242296555423,-88.9660308631234,122.));
#43895=CARTESIAN_POINT('Ctrl Pts',(38.9140147595642,-88.9932754177916,122.));
#43896=CARTESIAN_POINT('Ctrl Pts',(38.9088570148167,-89.007031843607,122.));
#43897=CARTESIAN_POINT('Ctrl Pts',(38.9035891933686,-89.0207474361896,122.));
#43898=CARTESIAN_POINT('Ctrl Pts',(38.8982139648971,-89.034417877811,122.));
#43899=CARTESIAN_POINT('Ctrl Pts',(38.8639626423259,-89.121526864554,122.));
#43900=CARTESIAN_POINT('Ctrl Pts',(38.8253378210354,-89.2068470331141,122.));
#43901=CARTESIAN_POINT('Ctrl Pts',(38.7826694863704,-89.2901439691626,122.));
#43902=CARTESIAN_POINT('Ctrl Pts',(38.7384396869984,-89.3764891897729,122.));
#43903=CARTESIAN_POINT('Ctrl Pts',(38.6898648813373,-89.4606611168872,122.));
#43904=CARTESIAN_POINT('Ctrl Pts',(38.6372567796703,-89.5423951719936,122.));
#43905=CARTESIAN_POINT('Ctrl Pts',(38.5840857288504,-89.6250038474651,122.));
#43906=CARTESIAN_POINT('Ctrl Pts',(38.5267941860822,-89.7051230190292,122.));
#43907=CARTESIAN_POINT('Ctrl Pts',(38.4656524677661,-89.7824641587497,122.));
#43908=CARTESIAN_POINT('Ctrl Pts',(38.4429635855522,-89.8111644317832,122.));
#43909=CARTESIAN_POINT('Ctrl Pts',(38.4197440399425,-89.8394819408235,122.));
#43910=CARTESIAN_POINT('Ctrl Pts',(38.3960060498082,-89.867401053708,122.));
#43911=CARTESIAN_POINT('Ctrl Pts',(38.3752506128797,-89.8918122773753,122.));
#43912=CARTESIAN_POINT('Ctrl Pts',(38.3540988125212,-89.9159189229224,122.));
#43913=CARTESIAN_POINT('Ctrl Pts',(38.3325583266211,-89.9397101583158,122.));
#43914=CARTESIAN_POINT('Ctrl Pts',(38.3207950958777,-89.9527025203685,122.));
#43915=CARTESIAN_POINT('Ctrl Pts',(38.3089206259342,-89.9655955686881,122.));
#43916=CARTESIAN_POINT('Ctrl Pts',(38.2969422410122,-89.9783816819787,122.));
#43917=CARTESIAN_POINT('Ctrl Pts',(38.2279314720012,-90.0520459962072,122.));
#43918=CARTESIAN_POINT('Ctrl Pts',(38.1554183053285,-90.1222257786201,122.));
#43919=CARTESIAN_POINT('Ctrl Pts',(38.0797112616787,-90.1886298153968,122.));
#43920=CARTESIAN_POINT('Ctrl Pts',(38.0175171475697,-90.2431814137882,122.));
#43921=CARTESIAN_POINT('Ctrl Pts',(37.9531664610367,-90.2951847791595,122.));
#43922=CARTESIAN_POINT('Ctrl Pts',(37.8868079691602,-90.3444651219269,122.));
#43923=CARTESIAN_POINT('Ctrl Pts',(37.8621903721155,-90.3627470868445,122.));
#43924=CARTESIAN_POINT('Ctrl Pts',(37.8372962693708,-90.3806541493651,122.));
#43925=CARTESIAN_POINT('Ctrl Pts',(37.8121326494392,-90.39817682058,122.));
#43926=CARTESIAN_POINT('Ctrl Pts',(37.7953218298329,-90.4098830244416,122.));
#43927=CARTESIAN_POINT('Ctrl Pts',(37.7783895868136,-90.4214183026613,122.));
#43928=CARTESIAN_POINT('Ctrl Pts',(37.7613530646459,-90.4327700028003,122.));
#43929=CARTESIAN_POINT('Ctrl Pts',(37.6764426037664,-90.4893471657374,122.));
#43930=CARTESIAN_POINT('Ctrl Pts',(37.5888628636194,-90.5414250307333,122.));
#43931=CARTESIAN_POINT('Ctrl Pts',(37.4989042014469,-90.5886956823262,122.));
#43932=CARTESIAN_POINT('Ctrl Pts',(37.4154461624309,-90.6325504461663,122.));
#43933=CARTESIAN_POINT('Ctrl Pts',(37.3299397797897,-90.6722679264133,122.));
#43934=CARTESIAN_POINT('Ctrl Pts',(37.2425891939653,-90.7075731985908,122.));
#43935=CARTESIAN_POINT('Ctrl Pts',(37.2121590204155,-90.7198724356188,122.));
#43936=CARTESIAN_POINT('Ctrl Pts',(37.1815048261116,-90.7316359142083,122.));
#43937=CARTESIAN_POINT('Ctrl Pts',(37.1506395173467,-90.742867356818,122.));
#43938=CARTESIAN_POINT('Ctrl Pts',(33.8367589339947,-87.7707538181913,120.387416697508));
#43939=CARTESIAN_POINT('Ctrl Pts',(33.8351765741934,-87.9451202468588,120.398449387697));
#43940=CARTESIAN_POINT('Ctrl Pts',(33.851762168828,-88.119187630204,120.409482077886));
#43941=CARTESIAN_POINT('Ctrl Pts',(33.8876337290323,-88.2891852722709,120.420514768075));
#43942=CARTESIAN_POINT('Ctrl Pts',(34.058817724406,-89.1004372893958,120.473164275806));
#43943=CARTESIAN_POINT('Ctrl Pts',(34.669206614267,-89.8190079065511,120.525813783537));
#43944=CARTESIAN_POINT('Ctrl Pts',(35.4420915502918,-90.1191531773417,120.578463291268));
#43945=CARTESIAN_POINT('Ctrl Pts',(36.2149764863167,-90.4192984481322,120.631112798999));
#43946=CARTESIAN_POINT('Ctrl Pts',(37.1503574685054,-90.3010183725579,120.683762306729));
#43947=CARTESIAN_POINT('Ctrl Pts',(37.8241903122464,-89.8179146759167,120.73641181446));
#43948=CARTESIAN_POINT('Ctrl Pts',(38.4980231559875,-89.3348109792755,120.789061322191));
#43949=CARTESIAN_POINT('Ctrl Pts',(38.9103078612808,-88.4868836615674,120.841710829922));
#43950=CARTESIAN_POINT('Ctrl Pts',(38.8741485025743,-87.6585662376428,120.894360337653));
#43951=CARTESIAN_POINT('Ctrl Pts',(38.8379891438677,-86.8302488137182,120.947009845384));
#43952=CARTESIAN_POINT('Ctrl Pts',(38.3533857211613,-86.021541283577,120.999659353114));
#43953=CARTESIAN_POINT('Ctrl Pts',(37.6400112734157,-85.5989796025709,121.052308860845));
#43954=CARTESIAN_POINT('Ctrl Pts',(36.92663682567,-85.1764179215648,121.104958368576));
#43955=CARTESIAN_POINT('Ctrl Pts',(35.984491352885,-85.1400020896938,121.157607876307));
#43956=CARTESIAN_POINT('Ctrl Pts',(35.2407121057255,-85.5064037850709,121.210257384038));
#43957=CARTESIAN_POINT('Ctrl Pts',(34.496932858566,-85.872805480448,121.262906891769));
#43958=CARTESIAN_POINT('Ctrl Pts',(33.9515198370319,-86.6420247030733,121.315556399499));
#43959=CARTESIAN_POINT('Ctrl Pts',(33.8516661553206,-87.4650121344612,121.36820590723));
#43960=CARTESIAN_POINT('Ctrl Pts',(33.8395212609014,-87.5651095499113,121.374609503989));
#43961=CARTESIAN_POINT('Ctrl Pts',(33.8339675723167,-87.6660023640875,121.381013100749));
#43962=CARTESIAN_POINT('Ctrl Pts',(33.8347233377312,-87.7669766891919,121.387416697508));
#43963=CARTESIAN_POINT('Ctrl Pts',(35.5611267921506,-90.7377785423179,122.));
#43964=CARTESIAN_POINT('Ctrl Pts',(34.5788882023789,-90.4751844899402,121.947350492269));
#43965=CARTESIAN_POINT('Ctrl Pts',(32.9121323375455,-88.9023410125859,121.842051476808));
#43966=CARTESIAN_POINT('Ctrl Pts',(33.5229013557052,-85.5001496093779,121.684102953615));
#43967=CARTESIAN_POINT('Ctrl Pts',(36.7064604149176,-84.1596949927803,121.526154430422));
#43968=CARTESIAN_POINT('Ctrl Pts',(39.5688528980205,-86.0888159753533,121.36820590723));
#43969=CARTESIAN_POINT('Ctrl Pts',(39.5184626244884,-89.5420982077003,121.210257384038));
#43970=CARTESIAN_POINT('Ctrl Pts',(36.5992128626851,-91.3867833270583,121.052308860845));
#43971=CARTESIAN_POINT('Ctrl Pts',(33.4587563518577,-89.9512134072174,120.894360337653));
#43972=CARTESIAN_POINT('Ctrl Pts',(32.944032363916,-86.5365568838997,120.73641181446));
#43973=CARTESIAN_POINT('Ctrl Pts',(35.5219283374979,-84.238982809065,120.578463291268));
#43974=CARTESIAN_POINT('Ctrl Pts',(38.8550457481358,-85.1415325934838,120.420514768075));
#43975=CARTESIAN_POINT('Ctrl Pts',(39.921396384874,-88.4259400024622,120.262566244883));
#43976=CARTESIAN_POINT('Ctrl Pts',(37.7541292274747,-91.1143092867255,120.10461772169));
#43977=CARTESIAN_POINT('Ctrl Pts',(34.3182508383241,-90.7691891793635,119.946669198498));
#43978=CARTESIAN_POINT('Ctrl Pts',(32.7289621381221,-87.7034840414673,119.788720675305));
#43979=CARTESIAN_POINT('Ctrl Pts',(34.4272255383588,-84.6967781783805,119.630772152113));
#43980=CARTESIAN_POINT('Ctrl Pts',(37.8732759596097,-84.4751590402537,119.47282362892));
#43981=CARTESIAN_POINT('Ctrl Pts',(39.9426849263303,-87.2395625969708,119.314875105728));
#43982=CARTESIAN_POINT('Ctrl Pts',(38.7591819580553,-90.4835879091297,119.156926582536));
#43983=CARTESIAN_POINT('Ctrl Pts',(35.3958133515618,-91.2659760395494,118.998978059343));
#43984=CARTESIAN_POINT('Ctrl Pts',(32.9020430571518,-88.877359392311,118.841029536151));
#43985=CARTESIAN_POINT('Ctrl Pts',(33.5388967916589,-85.4834240706333,118.683081012958));
#43986=CARTESIAN_POINT('Ctrl Pts',(36.7289586257789,-84.1613479914634,118.525132489766));
#43987=CARTESIAN_POINT('Ctrl Pts',(39.5798965242524,-86.1098173350916,118.367183966573));
#43988=CARTESIAN_POINT('Ctrl Pts',(39.506851797809,-89.5622142035652,118.209235443381));
#43989=CARTESIAN_POINT('Ctrl Pts',(36.5760518803447,-91.3883553581382,118.051286920188));
#43990=CARTESIAN_POINT('Ctrl Pts',(33.444763919809,-89.9325341525616,117.893338396996));
#43991=CARTESIAN_POINT('Ctrl Pts',(32.9520314766706,-86.5146993976035,117.735389873803));
#43992=CARTESIAN_POINT('Ctrl Pts',(35.544600071115,-84.2336979166091,117.577441350611));
#43993=CARTESIAN_POINT('Ctrl Pts',(38.87186660808,-85.1576443789841,117.419492827418));
#43994=CARTESIAN_POINT('Ctrl Pts',(39.9170997126827,-88.4488246277999,117.261544304226));
#43995=CARTESIAN_POINT('Ctrl Pts',(37.7326183183341,-91.1232256282042,117.103595781033));
#43996=CARTESIAN_POINT('Ctrl Pts',(34.2990252672788,-90.7560493313473,116.945647257841));
#43997=CARTESIAN_POINT('Ctrl Pts',(32.7294549509029,-87.6802033184331,116.787698734649));
#43998=CARTESIAN_POINT('Ctrl Pts',(34.446989038738,-84.6844636217403,116.629750211456));
#43999=CARTESIAN_POINT('Ctrl Pts',(37.8943916097836,-84.4849763129574,116.471801688264));
#44000=CARTESIAN_POINT('Ctrl Pts',(39.9460076008814,-87.2626104678248,116.313853165071));
#44001=CARTESIAN_POINT('Ctrl Pts',(38.7416991899834,-90.4989696760488,116.155904641879));
#44002=CARTESIAN_POINT('Ctrl Pts',(35.3733761858658,-91.2597454729484,115.997956118686));
#44003=CARTESIAN_POINT('Ctrl Pts',(32.8949946134489,-88.8551655814247,115.840007595494));
#44004=CARTESIAN_POINT('Ctrl Pts',(33.5536276678748,-85.4653894571308,115.682059072301));
#44005=CARTESIAN_POINT('Ctrl Pts',(36.7521127901144,-84.1638240165833,115.524110549109));
#44006=CARTESIAN_POINT('Ctrl Pts',(39.5904807973608,-86.1305590594033,115.366162025916));
#44007=CARTESIAN_POINT('Ctrl Pts',(39.4952697425043,-89.5824157378083,115.208213502724));
#44008=CARTESIAN_POINT('Ctrl Pts',(36.55280459327,-91.3897005849636,115.050264979531));
#44009=CARTESIAN_POINT('Ctrl Pts',(33.4309290094365,-89.9138033960376,114.892316456339));
#44010=CARTESIAN_POINT('Ctrl Pts',(32.9601526353117,-86.4928752648455,114.734367933146));
#44011=CARTESIAN_POINT('Ctrl Pts',(35.5673140912984,-84.2285676851132,114.576419409954));
#44012=CARTESIAN_POINT('Ctrl Pts',(38.8885793784847,-85.1738594735819,114.418470886761));
#44013=CARTESIAN_POINT('Ctrl Pts',(39.9126582726965,-88.4716833153973,114.260522363569));
#44014=CARTESIAN_POINT('Ctrl Pts',(37.7110495865035,-91.1320026319635,114.102573840377));
#44015=CARTESIAN_POINT('Ctrl Pts',(34.2798849567756,-90.7427868089045,113.944625317184));
#44016=CARTESIAN_POINT('Ctrl Pts',(32.730096999132,-87.6569259955238,113.786676793992));
#44017=CARTESIAN_POINT('Ctrl Pts',(34.4668313200981,-84.6722763390996,113.628728270799));
#44018=CARTESIAN_POINT('Ctrl Pts',(37.9154437312407,-84.4949289090955,113.470779747607));
#44019=CARTESIAN_POINT('Ctrl Pts',(39.949182244182,-87.2856792265183,113.312831224414));
#44020=CARTESIAN_POINT('Ctrl Pts',(38.724118002599,-90.5142388553946,113.154882701222));
#44021=CARTESIAN_POINT('Ctrl Pts',(35.3509794956904,-91.2533709724249,112.996934178029));
#44022=CARTESIAN_POINT('Ctrl Pts',(32.8880888182999,-88.832926966785,112.838985654837));
#44023=CARTESIAN_POINT('Ctrl Pts',(33.5684740421835,-85.4474498039115,112.681037131644));
#44024=CARTESIAN_POINT('Ctrl Pts',(36.7752505778273,-84.1664486627489,112.523088608452));
#44025=CARTESIAN_POINT('Ctrl Pts',(39.6009316700625,-86.1513683181001,112.365140085259));
#44026=CARTESIAN_POINT('Ctrl Pts',(39.4835582117651,-89.6025424870611,112.207191562067));
#44027=CARTESIAN_POINT('Ctrl Pts',(36.5295491478211,-91.3908965133523,112.049243038874));
#44028=CARTESIAN_POINT('Ctrl Pts',(33.417214654384,-89.8949841916642,111.891294515682));
#44029=CARTESIAN_POINT('Ctrl Pts',(32.9684137592783,-86.4711037279564,111.73334599249));
#44030=CARTESIAN_POINT('Ctrl Pts',(35.5900605844347,-84.2235834060515,111.575397469297));
#44031=CARTESIAN_POINT('Ctrl Pts',(38.9051876872665,-85.1901815465887,111.417448946105));
#44032=CARTESIAN_POINT('Ctrl Pts',(39.9080701486722,-88.4945130132787,111.259500422912));
#44033=CARTESIAN_POINT('Ctrl Pts',(37.6894249421801,-91.1406409620089,111.10155189972));
#44034=CARTESIAN_POINT('Ctrl Pts',(34.2608301994864,-90.7294016599341,110.943603376527));
#44035=CARTESIAN_POINT('Ctrl Pts',(32.730888497768,-87.6336532751223,110.785654853335));
#44036=CARTESIAN_POINT('Ctrl Pts',(34.4867514469574,-84.660216714833,110.627706330142));
#44037=CARTESIAN_POINT('Ctrl Pts',(37.9364315130628,-84.5050164759499,110.46975780695));
#44038=CARTESIAN_POINT('Ctrl Pts',(39.9522086976689,-87.3087678935207,110.311809283757));
#44039=CARTESIAN_POINT('Ctrl Pts',(38.7064391340791,-90.5293948322461,110.153860760565));
#44040=CARTESIAN_POINT('Ctrl Pts',(35.3286241982722,-91.2468527920333,109.995912237372));
#44041=CARTESIAN_POINT('Ctrl Pts',(32.8813259588075,-88.8106444729439,109.83796371418));
#44042=CARTESIAN_POINT('Ctrl Pts',(33.5834353025955,-85.4296058399034,109.680015190987));
#44043=CARTESIAN_POINT('Ctrl Pts',(36.7983710322676,-84.1692218413362,109.522066667795));
#44044=CARTESIAN_POINT('Ctrl Pts',(39.611248718183,-86.1722442141325,109.364118144603));
#44045=CARTESIAN_POINT('Ctrl Pts',(39.4717176740767,-89.6225937013098,109.20616962141));
#44046=CARTESIAN_POINT('Ctrl Pts',(36.506286532656,-91.3919429301732,109.048221098218));
#44047=CARTESIAN_POINT('Ctrl Pts',(33.4036213585832,-89.8760776520892,108.890272575025));
#44048=CARTESIAN_POINT('Ctrl Pts',(32.9768146345105,-86.4493849921911,108.732324051833));
#44049=CARTESIAN_POINT('Ctrl Pts',(35.6128383524474,-84.2187467086474,108.57437552864));
#44050=CARTESIAN_POINT('Ctrl Pts',(38.9216913848391,-85.2066069974257,108.416427005448));
#44051=CARTESIAN_POINT('Ctrl Pts',(39.9033344292869,-88.5173188003331,108.258478482255));
#44052=CARTESIAN_POINT('Ctrl Pts',(37.6677475399111,-91.14912788279,108.100529959063));
#44053=CARTESIAN_POINT('Ctrl Pts',(34.2418571276214,-90.7159198923917,107.94258143587));
#44054=CARTESIAN_POINT('Ctrl Pts',(32.7318389831201,-87.6103337706953,107.784632912678));
#44055=CARTESIAN_POINT('Ctrl Pts',(34.5067289212608,-84.6483928869776,107.626684389485));
#44056=CARTESIAN_POINT('Ctrl Pts',(37.9573945529429,-84.5150172531596,107.468735866293));
#44057=CARTESIAN_POINT('Ctrl Pts',(39.9550036656341,-87.3323307232591,107.3107873431));
#44058=CARTESIAN_POINT('Ctrl Pts',(38.68883464176,-90.5435009921344,107.152838819908));
#44059=CARTESIAN_POINT('Ctrl Pts',(35.3059682889895,-91.2421297218218,106.994890296715));
#44060=CARTESIAN_POINT('Ctrl Pts',(32.8754899278038,-88.7843420838406,106.836941773523));
#44061=CARTESIAN_POINT('Ctrl Pts',(33.3581428529919,-86.544039008134,106.731642758061));
#44062=CARTESIAN_POINT('Ctrl Pts',(34.018863416988,-85.7712540316409,106.678993250331));
#44063=CARTESIAN_POINT('Ctrl Pts',(35.6089932203365,-90.5587331584144,122.10700224989));
#44064=CARTESIAN_POINT('Ctrl Pts',(34.6859840276597,-90.3119736370406,122.054352742159));
#44065=CARTESIAN_POINT('Ctrl Pts',(33.1197342374261,-88.8339732781081,121.949053726697));
#44066=CARTESIAN_POINT('Ctrl Pts',(33.6936736287654,-85.6369354370915,121.791105203505));
#44067=CARTESIAN_POINT('Ctrl Pts',(36.6852627474191,-84.3773107935785,121.633156680312));
#44068=CARTESIAN_POINT('Ctrl Pts',(39.375051768605,-86.1901049754021,121.47520815712));
#44069=CARTESIAN_POINT('Ctrl Pts',(39.3277000496072,-89.435152847228,121.317259633928));
#44070=CARTESIAN_POINT('Ctrl Pts',(36.5844822673672,-91.1686026836444,121.159311110735));
#44071=CARTESIAN_POINT('Ctrl Pts',(33.6333965954336,-89.8195982293889,121.001362587543));
#44072=CARTESIAN_POINT('Ctrl Pts',(33.1497106788866,-86.6108469202099,120.84341406435));
#44073=CARTESIAN_POINT('Ctrl Pts',(35.5721584488666,-84.4518175214348,120.685465541157));
#44074=CARTESIAN_POINT('Ctrl Pts',(38.704287487907,-85.2999431769956,120.527517017965));
#44075=CARTESIAN_POINT('Ctrl Pts',(39.7063367359976,-88.3862994478151,120.369568494773));
#44076=CARTESIAN_POINT('Ctrl Pts',(37.6697566931271,-90.9125589417146,120.21161997158));
#44077=CARTESIAN_POINT('Ctrl Pts',(34.441063205486,-90.5882497209306,120.053671448388));
#44078=CARTESIAN_POINT('Ctrl Pts',(32.9476092775101,-87.7074078829283,119.895722925195));
#44079=CARTESIAN_POINT('Ctrl Pts',(34.5434666856064,-84.882007638829,119.737774402003));
#44080=CARTESIAN_POINT('Ctrl Pts',(37.7817188275649,-84.673752227268,119.57982587881));
#44081=CARTESIAN_POINT('Ctrl Pts',(39.726341569515,-87.2714610952442,119.421877355618));
#44082=CARTESIAN_POINT('Ctrl Pts',(38.6142043243961,-90.3198703265441,119.263928832425));
#44083=CARTESIAN_POINT('Ctrl Pts',(35.4536482492415,-91.0550801260151,119.105980309233));
#44084=CARTESIAN_POINT('Ctrl Pts',(33.1102533448528,-88.8104980599669,118.94803178604));
#44085=CARTESIAN_POINT('Ctrl Pts',(33.7087045332523,-85.6212184553168,118.790083262848));
#44086=CARTESIAN_POINT('Ctrl Pts',(36.7064043067714,-84.378864115751,118.632134739655));
#44087=CARTESIAN_POINT('Ctrl Pts',(39.3854294595639,-86.209839944379,118.474186216463));
#44088=CARTESIAN_POINT('Ctrl Pts',(39.3167893606247,-89.4540558401428,118.31623769327));
#44089=CARTESIAN_POINT('Ctrl Pts',(36.5627179019327,-91.1700799205937,118.158289170078));
#44090=CARTESIAN_POINT('Ctrl Pts',(33.6202479128799,-89.8020453415885,118.000340646886));
#44091=CARTESIAN_POINT('Ctrl Pts',(33.1572274418021,-86.5903074494638,117.842392123693));
#44092=CARTESIAN_POINT('Ctrl Pts',(35.5934630674801,-84.4468513102008,117.684443600501));
#44093=CARTESIAN_POINT('Ctrl Pts',(38.7200940429731,-85.3150834151026,117.526495077308));
#44094=CARTESIAN_POINT('Ctrl Pts',(39.7022991549334,-88.4078041206896,117.368546554116));
#44095=CARTESIAN_POINT('Ctrl Pts',(37.6495429007895,-90.920937624079,117.210598030923));
#44096=CARTESIAN_POINT('Ctrl Pts',(34.4229969444023,-90.5759022112363,117.052649507731));
#44097=CARTESIAN_POINT('Ctrl Pts',(32.9480723734746,-87.6855309972138,116.894700984538));
#44098=CARTESIAN_POINT('Ctrl Pts',(34.5620384386605,-84.8704356550963,116.736752461346));
#44099=CARTESIAN_POINT('Ctrl Pts',(37.8015611952165,-84.6829775143284,116.578803938153));
#44100=CARTESIAN_POINT('Ctrl Pts',(39.7294638854033,-87.2931191698622,116.420855414961));
#44101=CARTESIAN_POINT('Ctrl Pts',(38.5977757745388,-90.3343245664954,116.262906891769));
#44102=CARTESIAN_POINT('Ctrl Pts',(35.4325640540056,-91.0492252651816,116.104958368576));
#44103=CARTESIAN_POINT('Ctrl Pts',(33.1036299252483,-88.7896425451441,115.947009845384));
#44104=CARTESIAN_POINT('Ctrl Pts',(33.7225471314815,-85.6042713365387,115.789061322191));
#44105=CARTESIAN_POINT('Ctrl Pts',(36.7281622653295,-84.3811908355222,115.631112798999));
#44106=CARTESIAN_POINT('Ctrl Pts',(39.3953754965844,-86.229330934054,115.473164275806));
#44107=CARTESIAN_POINT('Ctrl Pts',(39.305905708091,-89.473039213436,115.315215752614));
#44108=CARTESIAN_POINT('Ctrl Pts',(36.5408724359755,-91.1713440296798,115.157267229421));
#44109=CARTESIAN_POINT('Ctrl Pts',(33.6072472533796,-89.7844440575038,114.999318706229));
#44110=CARTESIAN_POINT('Ctrl Pts',(33.1648588911862,-86.5697993210237,114.841370183036));
#44111=CARTESIAN_POINT('Ctrl Pts',(35.6148074227622,-84.4420304338062,114.683421659844));
#44112=CARTESIAN_POINT('Ctrl Pts',(38.735799026344,-85.3303207327256,114.525473136651));
#44113=CARTESIAN_POINT('Ctrl Pts',(39.6981255356329,-88.4292844198803,114.367524613459));
#44114=CARTESIAN_POINT('Ctrl Pts',(37.6292747724943,-90.9291853708469,114.209576090266));
#44115=CARTESIAN_POINT('Ctrl Pts',(34.4050108026144,-90.5634394244347,114.051627567074));
#44116=CARTESIAN_POINT('Ctrl Pts',(32.9486757059274,-87.6636573065954,113.893679043881));
#44117=CARTESIAN_POINT('Ctrl Pts',(34.5806842221695,-84.8589832706875,113.735730520689));
#44118=CARTESIAN_POINT('Ctrl Pts',(37.8213438649595,-84.6923299647638,113.577781997497));
#44119=CARTESIAN_POINT('Ctrl Pts',(39.7324470963873,-87.3147968727741,113.419833474304));
#44120=CARTESIAN_POINT('Ctrl Pts',(38.5812547400947,-90.348673007951,113.261884951112));
#44121=CARTESIAN_POINT('Ctrl Pts',(35.4115178935994,-91.0432351497015,113.103936427919));
#44122=CARTESIAN_POINT('Ctrl Pts',(33.0971405524303,-88.7687449282526,112.945987904727));
#44123=CARTESIAN_POINT('Ctrl Pts',(33.7364982632203,-85.5874134518995,112.788039381534));
#44124=CARTESIAN_POINT('Ctrl Pts',(36.7499048347821,-84.3836572144279,112.630090858342));
#44125=CARTESIAN_POINT('Ctrl Pts',(39.4051961772984,-86.2488853857627,112.472142335149));
#44126=CARTESIAN_POINT('Ctrl Pts',(39.2949003875455,-89.4919523113047,112.314193811957));
#44127=CARTESIAN_POINT('Ctrl Pts',(36.5190193035974,-91.1724678430876,112.156245288764));
#44128=CARTESIAN_POINT('Ctrl Pts',(33.5943598796632,-89.766759659012,111.998296765572));
#44129=CARTESIAN_POINT('Ctrl Pts',(33.1726218659282,-86.5493406168999,111.840348242379));
#44130=CARTESIAN_POINT('Ctrl Pts',(35.6361822928647,-84.437346708853,111.682399719187));
#44131=CARTESIAN_POINT('Ctrl Pts',(38.7514058471714,-85.3456585779148,111.524451195994));
#44132=CARTESIAN_POINT('Ctrl Pts',(39.693814077403,-88.4507374774469,111.366502672802));
#44133=CARTESIAN_POINT('Ctrl Pts',(37.6089541032529,-90.9373028059837,111.208554149609));
#44134=CARTESIAN_POINT('Ctrl Pts',(34.3871050551461,-90.5508614055361,111.050605626417));
#44135=CARTESIAN_POINT('Ctrl Pts',(32.9494194768651,-87.6417879409515,110.892657103225));
#44136=CARTESIAN_POINT('Ctrl Pts',(34.5994031570616,-84.8476508467996,110.734708580032));
#44137=CARTESIAN_POINT('Ctrl Pts',(37.8410660747743,-84.7018092471248,110.57676005684));
#44138=CARTESIAN_POINT('Ctrl Pts',(39.7352910534652,-87.3364932835156,110.418811533647));
#44139=CARTESIAN_POINT('Ctrl Pts',(38.5646419147283,-90.3629150730701,110.260863010455));
#44140=CARTESIAN_POINT('Ctrl Pts',(35.39051062995,-91.0371100183091,110.102914487262));
#44141=CARTESIAN_POINT('Ctrl Pts',(33.0907854961891,-88.7478060780943,109.94496596407));
#44142=CARTESIAN_POINT('Ctrl Pts',(33.7505573533824,-85.5706454863716,109.787017440877));
#44143=CARTESIAN_POINT('Ctrl Pts',(36.7716311161658,-84.3862631691886,109.629068917685));
#44144=CARTESIAN_POINT('Ctrl Pts',(39.4148911031094,-86.2685024565476,109.471120394492));
#44145=CARTESIAN_POINT('Ctrl Pts',(39.2837738392237,-89.510794428962,109.3131718713));
#44146=CARTESIAN_POINT('Ctrl Pts',(36.49715943384,-91.173451160537,109.155223348107));
#44147=CARTESIAN_POINT('Ctrl Pts',(33.581586265275,-89.7489931916678,108.997274824915));
#44148=CARTESIAN_POINT('Ctrl Pts',(33.1805161648761,-86.5289315299698,108.839326301722));
#44149=CARTESIAN_POINT('Ctrl Pts',(35.6575865519554,-84.4328016663219,108.68137777853));
#44150=CARTESIAN_POINT('Ctrl Pts',(38.7669143648894,-85.361093567208,108.523429255338));
#44151=CARTESIAN_POINT('Ctrl Pts',(39.689363923874,-88.4721680660194,108.365480732145));
#44152=CARTESIAN_POINT('Ctrl Pts',(37.5885838573921,-90.9452779618979,108.207532208953));
#44153=CARTESIAN_POINT('Ctrl Pts',(34.3692760674367,-90.5381925942059,108.04958368576));
#44154=CARTESIAN_POINT('Ctrl Pts',(32.9503126475537,-87.6198746123785,107.891635162568));
#44155=CARTESIAN_POINT('Ctrl Pts',(34.6181759813229,-84.836540000701,107.733686639375));
#44156=CARTESIAN_POINT('Ctrl Pts',(37.8607650345966,-84.7112069732929,107.575738116183));
#44157=CARTESIAN_POINT('Ctrl Pts',(39.7379174836951,-87.3586352647822,107.41778959299));
#44158=CARTESIAN_POINT('Ctrl Pts',(38.5480989806468,-90.3761706256272,107.259841069798));
#44159=CARTESIAN_POINT('Ctrl Pts',(35.3692208814569,-91.0326717512034,107.101892546605));
#44160=CARTESIAN_POINT('Ctrl Pts',(33.0853013802918,-88.7230897340364,106.943944023413));
#44161=CARTESIAN_POINT('Ctrl Pts',(33.5388501325603,-86.6178778692287,106.838645007951));
#44162=CARTESIAN_POINT('Ctrl Pts',(34.159728970665,-85.8916921494928,106.78599550022));
#44163=CARTESIAN_POINT('Ctrl Pts',(35.6568596485224,-90.3796877745108,122.21400449978));
#44164=CARTESIAN_POINT('Ctrl Pts',(34.7930798529405,-90.1487627841411,122.161354992049));
#44165=CARTESIAN_POINT('Ctrl Pts',(33.3273361373066,-88.7656055436304,122.056055976587));
#44166=CARTESIAN_POINT('Ctrl Pts',(33.8644459018257,-85.7737212648049,121.898107453395));
#44167=CARTESIAN_POINT('Ctrl Pts',(36.6640650799205,-84.5949265943767,121.740158930202));
#44168=CARTESIAN_POINT('Ctrl Pts',(39.1812506391896,-86.2913939754508,121.58221040701));
#44169=CARTESIAN_POINT('Ctrl Pts',(39.1369374747261,-89.3282074867557,121.424261883817));
#44170=CARTESIAN_POINT('Ctrl Pts',(36.5697516720493,-90.9504220402305,121.266313360625));
#44171=CARTESIAN_POINT('Ctrl Pts',(33.8080368390094,-89.6879830515605,121.108364837433));
#44172=CARTESIAN_POINT('Ctrl Pts',(33.3553889938573,-86.6851369565202,120.95041631424));
#44173=CARTESIAN_POINT('Ctrl Pts',(35.6223885602353,-84.6646522338046,120.792467791047));
#44174=CARTESIAN_POINT('Ctrl Pts',(38.5535292276782,-85.4583537605072,120.634519267855));
#44175=CARTESIAN_POINT('Ctrl Pts',(39.491277087121,-88.3466588931682,120.476570744662));
#44176=CARTESIAN_POINT('Ctrl Pts',(37.5853841587796,-90.7108085967037,120.31862222147));
#44177=CARTESIAN_POINT('Ctrl Pts',(34.5638755726478,-90.4073102624978,120.160673698277));
#44178=CARTESIAN_POINT('Ctrl Pts',(33.1662564168983,-87.7113317243892,120.002725175085));
#44179=CARTESIAN_POINT('Ctrl Pts',(34.659707832854,-85.0672370992777,119.844776651893));
#44180=CARTESIAN_POINT('Ctrl Pts',(37.6901616955201,-84.8723454142823,119.6868281287));
#44181=CARTESIAN_POINT('Ctrl Pts',(39.5099982126997,-87.3033595935177,119.528879605508));
#44182=CARTESIAN_POINT('Ctrl Pts',(38.4692266907368,-90.1561527439587,119.370931082315));
#44183=CARTESIAN_POINT('Ctrl Pts',(35.5114831469213,-90.8441842124806,119.212982559123));
#44184=CARTESIAN_POINT('Ctrl Pts',(33.3184636325538,-88.7436367276228,119.05503403593));
#44185=CARTESIAN_POINT('Ctrl Pts',(33.8785122748457,-85.7590128400003,118.897085512738));
#44186=CARTESIAN_POINT('Ctrl Pts',(36.6838499877638,-84.5963802400384,118.739136989545));
#44187=CARTESIAN_POINT('Ctrl Pts',(39.1909623948755,-86.3098625536665,118.581188466353));
#44188=CARTESIAN_POINT('Ctrl Pts',(39.1267269234404,-89.3458974767205,118.42323994316));
#44189=CARTESIAN_POINT('Ctrl Pts',(36.5493839235208,-90.9518044830492,118.265291419968));
#44190=CARTESIAN_POINT('Ctrl Pts',(33.7957319059508,-89.6715565306153,118.107342896775));
#44191=CARTESIAN_POINT('Ctrl Pts',(33.3624234069336,-86.6659155013242,117.949394373583));
#44192=CARTESIAN_POINT('Ctrl Pts',(35.6423260638452,-84.6600047037924,117.79144585039));
#44193=CARTESIAN_POINT('Ctrl Pts',(38.5683214778662,-85.4725224512211,117.633497327198));
#44194=CARTESIAN_POINT('Ctrl Pts',(39.4874985971841,-88.3667836135794,117.475548804005));
#44195=CARTESIAN_POINT('Ctrl Pts',(37.5664674832449,-90.718649619954,117.317600280813));
#44196=CARTESIAN_POINT('Ctrl Pts',(34.5469686215258,-90.3957550911254,117.159651757621));
#44197=CARTESIAN_POINT('Ctrl Pts',(33.1666897960462,-87.6908586759945,117.001703234428));
#44198=CARTESIAN_POINT('Ctrl Pts',(34.6770878385831,-85.0564076884523,116.843754711236));
#44199=CARTESIAN_POINT('Ctrl Pts',(37.7087307806494,-84.8809787156995,116.685806188043));
#44200=CARTESIAN_POINT('Ctrl Pts',(39.5129201699252,-87.3236278718996,116.527857664851));
#44201=CARTESIAN_POINT('Ctrl Pts',(38.4538523590942,-90.169679456942,116.369909141658));
#44202=CARTESIAN_POINT('Ctrl Pts',(35.4917519221453,-90.8387050574149,116.211960618466));
#44203=CARTESIAN_POINT('Ctrl Pts',(33.3122652370477,-88.7241195088633,116.054012095273));
#44204=CARTESIAN_POINT('Ctrl Pts',(33.8914665950882,-85.7431532159467,115.896063572081));
#44205=CARTESIAN_POINT('Ctrl Pts',(36.7042117405445,-84.5985576544611,115.738115048888));
#44206=CARTESIAN_POINT('Ctrl Pts',(39.200270195808,-86.3281028087049,115.580166525696));
#44207=CARTESIAN_POINT('Ctrl Pts',(39.1165416736776,-89.3636626890636,115.422218002503));
#44208=CARTESIAN_POINT('Ctrl Pts',(36.528940278681,-90.9529874743961,115.264269479311));
#44209=CARTESIAN_POINT('Ctrl Pts',(33.7835654973227,-89.6550847189701,115.106320956118));
#44210=CARTESIAN_POINT('Ctrl Pts',(33.3695651470607,-86.6467233772021,114.948372432926));
#44211=CARTESIAN_POINT('Ctrl Pts',(35.662300754226,-84.6554931824991,114.790423909734));
#44212=CARTESIAN_POINT('Ctrl Pts',(38.5830186742033,-85.4867819918694,114.632475386541));
#44213=CARTESIAN_POINT('Ctrl Pts',(39.4835927985692,-88.3868855243633,114.474526863349));
#44214=CARTESIAN_POINT('Ctrl Pts',(37.5474999584851,-90.7263681097303,114.316578340156));
#44215=CARTESIAN_POINT('Ctrl Pts',(34.5301366484532,-90.3840920399647,114.158629816964));
#44216=CARTESIAN_POINT('Ctrl Pts',(33.1672544127228,-87.6703886176669,114.000681293771));
#44217=CARTESIAN_POINT('Ctrl Pts',(34.6945371242409,-85.0456902022755,113.842732770579));
#44218=CARTESIAN_POINT('Ctrl Pts',(37.7272439986783,-84.889731020432,113.684784247386));
#44219=CARTESIAN_POINT('Ctrl Pts',(39.5157119485926,-87.3439145190299,113.526835724194));
#44220=CARTESIAN_POINT('Ctrl Pts',(38.4383914775904,-90.1831071605076,113.368887201001));
#44221=CARTESIAN_POINT('Ctrl Pts',(35.4720562915084,-90.8330993269778,113.210938677809));
#44222=CARTESIAN_POINT('Ctrl Pts',(33.3061922865607,-88.7045628897205,113.052990154617));
#44223=CARTESIAN_POINT('Ctrl Pts',(33.9045224842572,-85.7273770998871,112.895041631424));
#44224=CARTESIAN_POINT('Ctrl Pts',(36.724559091737,-84.6008657661072,112.737093108232));
#44225=CARTESIAN_POINT('Ctrl Pts',(39.2094606845344,-86.3464024534252,112.579144585039));
#44226=CARTESIAN_POINT('Ctrl Pts',(39.1062425633258,-89.3813621355486,112.421196061847));
#44227=CARTESIAN_POINT('Ctrl Pts',(36.5084894593737,-90.9540391728226,112.263247538654));
#44228=CARTESIAN_POINT('Ctrl Pts',(33.7715051049423,-89.6385351263598,112.105299015462));
#44229=CARTESIAN_POINT('Ctrl Pts',(33.3768299725781,-86.6275775058433,111.947350492269));
#44230=CARTESIAN_POINT('Ctrl Pts',(35.6823040012946,-84.6511100116545,111.789401969077));
#44231=CARTESIAN_POINT('Ctrl Pts',(38.5976240070764,-85.5011356092412,111.631453445884));
#44232=CARTESIAN_POINT('Ctrl Pts',(39.4795580061338,-88.4069619416151,111.473504922692));
#44233=CARTESIAN_POINT('Ctrl Pts',(37.5284832643257,-90.7339646499585,111.315556399499));
#44234=CARTESIAN_POINT('Ctrl Pts',(34.5133799108057,-90.3723211511379,111.157607876307));
#44235=CARTESIAN_POINT('Ctrl Pts',(33.1679504559622,-87.6499226067807,110.999659353114));
#44236=CARTESIAN_POINT('Ctrl Pts',(34.7120548671658,-85.0350849787663,110.841710829922));
#44237=CARTESIAN_POINT('Ctrl Pts',(37.7457006364858,-84.8986020182997,110.683762306729));
#44238=CARTESIAN_POINT('Ctrl Pts',(39.5183734092616,-87.3642186735107,110.525813783537));
#44239=CARTESIAN_POINT('Ctrl Pts',(38.4228446953775,-90.1964353138941,110.367865260344));
#44240=CARTESIAN_POINT('Ctrl Pts',(35.4523970616278,-90.8273672445848,110.209916737152));
#44241=CARTESIAN_POINT('Ctrl Pts',(33.3002450335707,-88.6849676832447,110.051968213959));
#44242=CARTESIAN_POINT('Ctrl Pts',(33.9176794041694,-85.7116851328398,109.894019690767));
#44243=CARTESIAN_POINT('Ctrl Pts',(36.744891200064,-84.6033044970411,109.736071167575));
#44244=CARTESIAN_POINT('Ctrl Pts',(39.2185334880359,-86.3647606989627,109.578122644382));
#44245=CARTESIAN_POINT('Ctrl Pts',(39.0958300043706,-89.3989951566143,109.42017412119));
#44246=CARTESIAN_POINT('Ctrl Pts',(36.488032335024,-90.9549593909009,109.262225597997));
#44247=CARTESIAN_POINT('Ctrl Pts',(33.7595511719668,-89.6219087312464,109.104277074805));
#44248=CARTESIAN_POINT('Ctrl Pts',(33.3842176952418,-86.6084780677483,108.946328551612));
#44249=CARTESIAN_POINT('Ctrl Pts',(35.7023347514634,-84.6468566239965,108.78838002842));
#44250=CARTESIAN_POINT('Ctrl Pts',(38.6121373449396,-85.5155801369902,108.630431505227));
#44251=CARTESIAN_POINT('Ctrl Pts',(39.4753934184612,-88.4270173317057,108.472482982035));
#44252=CARTESIAN_POINT('Ctrl Pts',(37.5094201748731,-90.741428041006,108.314534458842));
#44253=CARTESIAN_POINT('Ctrl Pts',(34.496695007252,-90.3604652960198,108.15658593565));
#44254=CARTESIAN_POINT('Ctrl Pts',(33.1687863119872,-87.6294154540617,107.998637412457));
#44255=CARTESIAN_POINT('Ctrl Pts',(34.7296230413851,-85.0246871144243,107.840688889265));
#44256=CARTESIAN_POINT('Ctrl Pts',(37.7641355162503,-84.9073966934263,107.682740366073));
#44257=CARTESIAN_POINT('Ctrl Pts',(39.5208313017561,-87.3849398063052,107.52479184288));
#44258=CARTESIAN_POINT('Ctrl Pts',(38.4073633195336,-90.2088402591199,107.366843319688));
#44259=CARTESIAN_POINT('Ctrl Pts',(35.4324734739243,-90.823213780585,107.208894796495));
#44260=CARTESIAN_POINT('Ctrl Pts',(33.2951128327798,-88.6618373842322,107.050946273303));
#44261=CARTESIAN_POINT('Ctrl Pts',(33.7195574121287,-86.6917167303234,106.945647257841));
#44262=CARTESIAN_POINT('Ctrl Pts',(34.300594524342,-86.0121302673448,106.89299775011));
#44263=CARTESIAN_POINT('Ctrl Pts',(35.7047260767084,-90.2006423906073,122.321006749669));
#44264=CARTESIAN_POINT('Ctrl Pts',(34.9001756782213,-89.9855519312415,122.268357241939));
#44265=CARTESIAN_POINT('Ctrl Pts',(33.5349380371872,-88.6972378091528,122.163058226477));
#44266=CARTESIAN_POINT('Ctrl Pts',(34.0352181748859,-85.9105070925183,122.005109703285));
#44267=CARTESIAN_POINT('Ctrl Pts',(36.642867412422,-84.8125423951751,121.847161180092));
#44268=CARTESIAN_POINT('Ctrl Pts',(38.9874495097741,-86.3926829754995,121.6892126569));
#44269=CARTESIAN_POINT('Ctrl Pts',(38.9461748998449,-89.2212621262834,121.531264133707));
#44270=CARTESIAN_POINT('Ctrl Pts',(36.5550210767314,-90.7322413968164,121.373315610515));
#44271=CARTESIAN_POINT('Ctrl Pts',(33.9826770825852,-89.5563678737322,121.215367087322));
#44272=CARTESIAN_POINT('Ctrl Pts',(33.5610673088279,-86.7594269928302,121.05741856413));
#44273=CARTESIAN_POINT('Ctrl Pts',(35.672618671604,-84.8774869461745,120.899470040937));
#44274=CARTESIAN_POINT('Ctrl Pts',(38.4027709674495,-85.6167643440188,120.741521517745));
#44275=CARTESIAN_POINT('Ctrl Pts',(39.2762174382445,-88.3070183385212,120.583572994552));
#44276=CARTESIAN_POINT('Ctrl Pts',(37.5010116244319,-90.5090582516927,120.42562447136));
#44277=CARTESIAN_POINT('Ctrl Pts',(34.6866879398097,-90.2263708040651,120.267675948167));
#44278=CARTESIAN_POINT('Ctrl Pts',(33.3849035562864,-87.71525556585,120.109727424975));
#44279=CARTESIAN_POINT('Ctrl Pts',(34.7759489801016,-85.2524665597263,119.951778901782));
#44280=CARTESIAN_POINT('Ctrl Pts',(37.5986045634753,-85.0709386012965,119.79383037859));
#44281=CARTESIAN_POINT('Ctrl Pts',(39.2936548558844,-87.3352580917912,119.635881855397));
#44282=CARTESIAN_POINT('Ctrl Pts',(38.3242490570776,-89.9924351613731,119.477933332205));
#44283=CARTESIAN_POINT('Ctrl Pts',(35.569318044601,-90.6332882989464,119.319984809013));
#44284=CARTESIAN_POINT('Ctrl Pts',(33.5266739202549,-88.6767753952787,119.16203628582));
#44285=CARTESIAN_POINT('Ctrl Pts',(34.048320016439,-85.8968072246837,119.004087762628));
#44286=CARTESIAN_POINT('Ctrl Pts',(36.6612956687563,-84.8138963643259,118.846139239435));
#44287=CARTESIAN_POINT('Ctrl Pts',(38.996495330187,-86.4098851629539,118.688190716243));
#44288=CARTESIAN_POINT('Ctrl Pts',(38.9366644862561,-89.2377391132981,118.53024219305));
#44289=CARTESIAN_POINT('Ctrl Pts',(36.5360499451088,-90.7335290455047,118.372293669858));
#44290=CARTESIAN_POINT('Ctrl Pts',(33.9712158990217,-89.5410677196422,118.214345146665));
#44291=CARTESIAN_POINT('Ctrl Pts',(33.5676193720652,-86.7415235531845,118.056396623473));
#44292=CARTESIAN_POINT('Ctrl Pts',(35.6911890602102,-84.873158097384,117.89844810028));
#44293=CARTESIAN_POINT('Ctrl Pts',(38.4165489127592,-85.6299614873397,117.740499577088));
#44294=CARTESIAN_POINT('Ctrl Pts',(39.2726980394348,-88.3257631064689,117.582551053895));
#44295=CARTESIAN_POINT('Ctrl Pts',(37.4833920657004,-90.5163616158289,117.424602530703));
#44296=CARTESIAN_POINT('Ctrl Pts',(34.6709402986493,-90.2156079710144,117.26665400751));
#44297=CARTESIAN_POINT('Ctrl Pts',(33.3853072186179,-87.6961863547752,117.108705484318));
#44298=CARTESIAN_POINT('Ctrl Pts',(34.7921372385056,-85.2423797218082,116.950756961126));
#44299=CARTESIAN_POINT('Ctrl Pts',(37.6159003660824,-85.0789799170705,116.792808437933));
#44300=CARTESIAN_POINT('Ctrl Pts',(39.2963764544471,-87.3541365739369,116.634859914741));
#44301=CARTESIAN_POINT('Ctrl Pts',(38.3099289436496,-90.0050343473886,116.476911391548));
#44302=CARTESIAN_POINT('Ctrl Pts',(35.5509397902851,-90.6281848496482,116.318962868356));
#44303=CARTESIAN_POINT('Ctrl Pts',(33.5209005488471,-88.6585964725826,116.161014345163));
#44304=CARTESIAN_POINT('Ctrl Pts',(34.0603860586949,-85.8820350953548,116.003065821971));
#44305=CARTESIAN_POINT('Ctrl Pts',(36.6802612157596,-84.8159244733999,115.845117298778));
#44306=CARTESIAN_POINT('Ctrl Pts',(39.0051648950316,-86.4268746833558,115.687168775586));
#44307=CARTESIAN_POINT('Ctrl Pts',(38.9271776392642,-89.2542861646912,115.529220252393));
#44308=CARTESIAN_POINT('Ctrl Pts',(36.5170081213865,-90.7346309191124,115.371271729201));
#44309=CARTESIAN_POINT('Ctrl Pts',(33.9598837412658,-89.5257253804362,115.213323206008));
#44310=CARTESIAN_POINT('Ctrl Pts',(33.5742714029352,-86.7236474333804,115.055374682816));
#44311=CARTESIAN_POINT('Ctrl Pts',(35.7097940856898,-84.8689559311919,114.897426159624));
#44312=CARTESIAN_POINT('Ctrl Pts',(38.4302383220626,-85.6432432510131,114.739477636431));
#44313=CARTESIAN_POINT('Ctrl Pts',(39.2690600615056,-88.3444866288462,114.581529113239));
#44314=CARTESIAN_POINT('Ctrl Pts',(37.4657251444759,-90.5235508486137,114.423580590046));
#44315=CARTESIAN_POINT('Ctrl Pts',(34.655262494292,-90.2047446554949,114.265632066854));
#44316=CARTESIAN_POINT('Ctrl Pts',(33.3858331195181,-87.6771199287383,114.107683543661));
#44317=CARTESIAN_POINT('Ctrl Pts',(34.8083900263124,-85.2323971338635,113.949735020469));
#44318=CARTESIAN_POINT('Ctrl Pts',(37.6331441323971,-85.0871320761002,113.791786497276));
#44319=CARTESIAN_POINT('Ctrl Pts',(39.2989768007979,-87.3730321652858,113.633837974084));
#44320=CARTESIAN_POINT('Ctrl Pts',(38.2955282150861,-90.0175413130639,113.475889450891));
#44321=CARTESIAN_POINT('Ctrl Pts',(35.5325946894174,-90.6229635042544,113.317940927699));
#44322=CARTESIAN_POINT('Ctrl Pts',(33.5152440206911,-88.6403808511882,113.159992404506));
#44323=CARTESIAN_POINT('Ctrl Pts',(34.072546705294,-85.8673407478749,113.002043881314));
#44324=CARTESIAN_POINT('Ctrl Pts',(36.6992133486918,-84.8180743177863,112.844095358121));
#44325=CARTESIAN_POINT('Ctrl Pts',(39.0137251917704,-86.4439195210878,112.686146834929));
#44326=CARTESIAN_POINT('Ctrl Pts',(38.9175847391062,-89.2707719597925,112.528198311736));
#44327=CARTESIAN_POINT('Ctrl Pts',(36.49795961515,-90.7356105025577,112.370249788544));
#44328=CARTESIAN_POINT('Ctrl Pts',(33.9486503302215,-89.5103105937078,112.212301265351));
#44329=CARTESIAN_POINT('Ctrl Pts',(33.581038079228,-86.7058143947865,112.054352742159));
#44330=CARTESIAN_POINT('Ctrl Pts',(35.7284257097246,-84.8648733144562,111.896404218967));
#44331=CARTESIAN_POINT('Ctrl Pts',(38.4438421669814,-85.6566126405671,111.738455695774));
#44332=CARTESIAN_POINT('Ctrl Pts',(39.2653019348646,-88.3631864057835,111.580507172582));
#44333=CARTESIAN_POINT('Ctrl Pts',(37.4480124253985,-90.5306264939331,111.422558649389));
#44334=CARTESIAN_POINT('Ctrl Pts',(34.6396547664653,-90.1937808967399,111.264610126197));
#44335=CARTESIAN_POINT('Ctrl Pts',(33.3864814350593,-87.6580572726099,111.106661603004));
#44336=CARTESIAN_POINT('Ctrl Pts',(34.82470657727,-85.2225191107331,110.948713079812));
#44337=CARTESIAN_POINT('Ctrl Pts',(37.6503351981973,-85.0953947894745,110.790764556619));
#44338=CARTESIAN_POINT('Ctrl Pts',(39.3014557650579,-87.3919440635056,110.632816033427));
#44339=CARTESIAN_POINT('Ctrl Pts',(38.2810474760267,-90.029955554718,110.474867510234));
#44340=CARTESIAN_POINT('Ctrl Pts',(35.5142834933055,-90.6176244708606,110.316918987042));
#44341=CARTESIAN_POINT('Ctrl Pts',(33.5097045709523,-88.622129288395,110.158970463849));
#44342=CARTESIAN_POINT('Ctrl Pts',(34.0848014549563,-85.8527247793081,110.001021940657));
#44343=CARTESIAN_POINT('Ctrl Pts',(36.7181512839622,-84.8203458248934,109.843073417464));
#44344=CARTESIAN_POINT('Ctrl Pts',(39.0221758729624,-86.4610189413778,109.685124894272));
#44345=CARTESIAN_POINT('Ctrl Pts',(38.9078861695176,-89.2871958842667,109.527176371079));
#44346=CARTESIAN_POINT('Ctrl Pts',(36.4789052362081,-90.7364676212647,109.369227847887));
#44347=CARTESIAN_POINT('Ctrl Pts',(33.9375160786586,-89.4948242708249,109.211279324695));
#44348=CARTESIAN_POINT('Ctrl Pts',(33.5879192256074,-86.6880246055271,109.053330801502));
#44349=CARTESIAN_POINT('Ctrl Pts',(35.7470829509713,-84.860911581671,108.89538227831));
#44350=CARTESIAN_POINT('Ctrl Pts',(38.4573603249899,-85.6700667067725,108.737433755117));
#44351=CARTESIAN_POINT('Ctrl Pts',(39.2614229130483,-88.3818665973921,108.579485231925));
#44352=CARTESIAN_POINT('Ctrl Pts',(37.4302564923541,-90.5375781201139,108.421536708732));
#44353=CARTESIAN_POINT('Ctrl Pts',(34.6241139470672,-90.1827379978339,108.26358818554));
#44354=CARTESIAN_POINT('Ctrl Pts',(33.3872599764207,-87.6389562957449,108.105639662347));
#44355=CARTESIAN_POINT('Ctrl Pts',(34.8410701014472,-85.2128342281477,107.947691139155));
#44356=CARTESIAN_POINT('Ctrl Pts',(37.667505997904,-85.1035864135597,107.789742615962));
#44357=CARTESIAN_POINT('Ctrl Pts',(39.3037451198171,-87.4112443478284,107.63179409277));
#44358=CARTESIAN_POINT('Ctrl Pts',(38.2666276584204,-90.0415098926125,107.473845569578));
#44359=CARTESIAN_POINT('Ctrl Pts',(35.4957260663917,-90.6137558099667,107.315897046385));
#44360=CARTESIAN_POINT('Ctrl Pts',(33.5049242852677,-88.6005850344281,107.157948523192));
#44361=CARTESIAN_POINT('Ctrl Pts',(33.9002646916971,-86.7655555914181,107.052649507731));
#44362=CARTESIAN_POINT('Ctrl Pts',(34.441460078019,-86.1325683851967,107.));
#44363=CARTESIAN_POINT('Ctrl Pts',(33.8399315564717,-87.7667938053724,121.112583302492));
#44364=CARTESIAN_POINT('Ctrl Pts',(33.8380186898685,-87.4752409773549,121.094195056371));
#44365=CARTESIAN_POINT('Ctrl Pts',(33.8848899787242,-87.1842829992347,121.07580681025));
#44366=CARTESIAN_POINT('Ctrl Pts',(33.9832608315835,-86.9119271318713,121.05741856413));
#44367=CARTESIAN_POINT('Ctrl Pts',(34.2649177630866,-86.132113643945,121.004769056399));
#44368=CARTESIAN_POINT('Ctrl Pts',(34.9687682173453,-85.5048002950597,120.952119548668));
#44369=CARTESIAN_POINT('Ctrl Pts',(35.7757188271156,-85.3143565202578,120.899470040937));
#44370=CARTESIAN_POINT('Ctrl Pts',(36.5826694368858,-85.1239127454559,120.846820533206));
#44371=CARTESIAN_POINT('Ctrl Pts',(37.4927202021677,-85.3703385447374,120.794171025476));
#44372=CARTESIAN_POINT('Ctrl Pts',(38.0933199966077,-85.9419271101285,120.741521517745));
#44373=CARTESIAN_POINT('Ctrl Pts',(38.6939197910478,-86.5135156755196,120.688872010014));
#44374=CARTESIAN_POINT('Ctrl Pts',(38.9850686146462,-87.4102670070204,120.636222502283));
#44375=CARTESIAN_POINT('Ctrl Pts',(38.8347753908099,-88.225649324966,120.583572994552));
#44376=CARTESIAN_POINT('Ctrl Pts',(38.6844821669737,-89.0410316429117,120.530923486821));
#44377=CARTESIAN_POINT('Ctrl Pts',(38.0927468957028,-89.7750449473022,120.478273979091));
#44378=CARTESIAN_POINT('Ctrl Pts',(37.3278253126303,-90.0949370248928,120.42562447136));
#44379=CARTESIAN_POINT('Ctrl Pts',(36.5629037295579,-90.4148291024835,120.372974963629));
#44380=CARTESIAN_POINT('Ctrl Pts',(35.6247958346838,-90.3205999532743,120.320325455898));
#44381=CARTESIAN_POINT('Ctrl Pts',(34.9387778233262,-89.8549661723005,120.267675948167));
#44382=CARTESIAN_POINT('Ctrl Pts',(34.2651637482346,-89.3977515459945,120.215978399609));
#44383=CARTESIAN_POINT('Ctrl Pts',(33.8346058639746,-88.5824416490861,120.16428085105));
#44384=CARTESIAN_POINT('Ctrl Pts',(33.8333405706013,-87.7682823373648,120.112583302492));
#44385=CARTESIAN_POINT('Ctrl Pts',(35.5611267921506,-90.7377785423179,122.));
#44386=CARTESIAN_POINT('Ctrl Pts',(35.4680767052966,-90.7037404048947,122.));
#44387=CARTESIAN_POINT('Ctrl Pts',(35.3770917836601,-90.664933572561,122.));
#44388=CARTESIAN_POINT('Ctrl Pts',(35.2883805128425,-90.6216863669008,122.));
#44389=CARTESIAN_POINT('Ctrl Pts',(35.197702296709,-90.5774802651747,122.));
#44390=CARTESIAN_POINT('Ctrl Pts',(35.1093990059899,-90.5286340828183,122.));
#44391=CARTESIAN_POINT('Ctrl Pts',(35.0237222209495,-90.4754529263978,122.));
#44392=CARTESIAN_POINT('Ctrl Pts',(34.9412907936686,-90.424286223234,122.));
#44393=CARTESIAN_POINT('Ctrl Pts',(34.861290377545,-90.3691058598076,122.));
#44394=CARTESIAN_POINT('Ctrl Pts',(34.7839779997226,-90.3101535213279,122.));
#44395=CARTESIAN_POINT('Ctrl Pts',(34.7163296691279,-90.2585702251582,122.));
#44396=CARTESIAN_POINT('Ctrl Pts',(34.6507396580929,-90.2040983132303,122.));
#44397=CARTESIAN_POINT('Ctrl Pts',(34.5874047755446,-90.1468869965436,122.));
#44398=CARTESIAN_POINT('Ctrl Pts',(34.5732683536243,-90.1341173618848,122.));
#44399=CARTESIAN_POINT('Ctrl Pts',(34.5592416368608,-90.1212085175659,122.));
#44400=CARTESIAN_POINT('Ctrl Pts',(34.5453463983788,-90.1081806554779,122.));
#44401=CARTESIAN_POINT('Ctrl Pts',(34.4729162970605,-90.040271826693,122.));
#44402=CARTESIAN_POINT('Ctrl Pts',(34.403951882981,-89.9690410838559,122.));
#44403=CARTESIAN_POINT('Ctrl Pts',(34.3386931062104,-89.8947791484553,122.));
#44404=CARTESIAN_POINT('Ctrl Pts',(34.2737933595084,-89.8209257752296,122.));
#44405=CARTESIAN_POINT('Ctrl Pts',(34.2125581016922,-89.7440736737795,122.));
#44406=CARTESIAN_POINT('Ctrl Pts',(34.1552669537762,-89.6644820254102,122.));
#44407=CARTESIAN_POINT('Ctrl Pts',(34.1001040339643,-89.5878470150046,122.));
#44408=CARTESIAN_POINT('Ctrl Pts',(34.0485974753497,-89.5086714751506,122.));
#44409=CARTESIAN_POINT('Ctrl Pts',(34.0010417263708,-89.4271731777542,122.));
#44410=CARTESIAN_POINT('Ctrl Pts',(33.9810953973884,-89.392990310566,122.));
#44411=CARTESIAN_POINT('Ctrl Pts',(33.9618446717128,-89.3583987128521,122.));
#44412=CARTESIAN_POINT('Ctrl Pts',(33.9433138595418,-89.3234141560505,122.));
#44413=CARTESIAN_POINT('Ctrl Pts',(33.9304313294793,-89.2990930631293,122.));
#44414=CARTESIAN_POINT('Ctrl Pts',(33.9178967633415,-89.274582051837,122.));
#44415=CARTESIAN_POINT('Ctrl Pts',(33.9057187949769,-89.2498864153828,122.));
#44416=CARTESIAN_POINT('Ctrl Pts',(33.8978104365748,-89.2338490979749,122.));
#44417=CARTESIAN_POINT('Ctrl Pts',(33.8900513541417,-89.2177313077059,122.));
#44418=CARTESIAN_POINT('Ctrl Pts',(33.8824540881418,-89.2015566837388,122.));
#44419=CARTESIAN_POINT('Ctrl Pts',(33.8403337819923,-89.1118823043832,122.));
#44420=CARTESIAN_POINT('Ctrl Pts',(33.8031123102296,-89.0203243302145,122.));
#44421=CARTESIAN_POINT('Ctrl Pts',(33.7710809567661,-88.9271551245399,122.));
#44422=CARTESIAN_POINT('Ctrl Pts',(33.7412012053114,-88.8402442572872,122.));
#44423=CARTESIAN_POINT('Ctrl Pts',(33.7158379051123,-88.7519305553683,122.));
#44424=CARTESIAN_POINT('Ctrl Pts',(33.6952780341048,-88.662426403845,122.));
#44425=CARTESIAN_POINT('Ctrl Pts',(33.6937975445556,-88.6559813263984,122.));
#44426=CARTESIAN_POINT('Ctrl Pts',(33.6923419845185,-88.6495300750113,122.));
#44427=CARTESIAN_POINT('Ctrl Pts',(33.6909114717731,-88.6430727286702,122.));
#44428=CARTESIAN_POINT('Ctrl Pts',(33.6703052539739,-88.5500560914257,122.));
#44429=CARTESIAN_POINT('Ctrl Pts',(33.6548920629776,-88.4557737818519,122.));
#44430=CARTESIAN_POINT('Ctrl Pts',(33.6445949784327,-88.3606336675157,122.));
#44431=CARTESIAN_POINT('Ctrl Pts',(33.6387984637639,-88.3070766566996,122.));
#44432=CARTESIAN_POINT('Ctrl Pts',(33.6346241089796,-88.2532480069532,122.));
#44433=CARTESIAN_POINT('Ctrl Pts',(33.6320649544127,-88.1992231133509,122.));
#44434=CARTESIAN_POINT('Ctrl Pts',(33.6314040725555,-88.1852716027681,122.));
#44435=CARTESIAN_POINT('Ctrl Pts',(33.6308510273416,-88.1713076039324,122.));
#44436=CARTESIAN_POINT('Ctrl Pts',(33.6304059403149,-88.15734578475,122.));
#44437=CARTESIAN_POINT('Ctrl Pts',(33.627434535562,-88.0641365618572,122.));
#44438=CARTESIAN_POINT('Ctrl Pts',(33.6292622862227,-87.9708690974207,122.));
#44439=CARTESIAN_POINT('Ctrl Pts',(33.6357542976629,-87.877918472349,122.));
#44440=CARTESIAN_POINT('Ctrl Pts',(33.6422571034003,-87.7848132978462,122.));
#44441=CARTESIAN_POINT('Ctrl Pts',(33.6534400713544,-87.6920250375438,122.));
#44442=CARTESIAN_POINT('Ctrl Pts',(33.6692185656195,-87.5999427421327,122.));
#44443=CARTESIAN_POINT('Ctrl Pts',(33.6847714619004,-87.5091770223002,122.));
#44444=CARTESIAN_POINT('Ctrl Pts',(33.7047898729604,-87.4190963800901,122.));
#44445=CARTESIAN_POINT('Ctrl Pts',(33.7292357664442,-87.3300986153128,122.));
#44446=CARTESIAN_POINT('Ctrl Pts',(33.7383345299043,-87.2969736403256,122.));
#44447=CARTESIAN_POINT('Ctrl Pts',(33.7480470433711,-87.2639989962916,122.));
#44448=CARTESIAN_POINT('Ctrl Pts',(33.7583727072738,-87.2311964605871,122.));
#44449=CARTESIAN_POINT('Ctrl Pts',(33.7653671455383,-87.2089765517205,122.));
#44450=CARTESIAN_POINT('Ctrl Pts',(33.7726429420923,-87.1868356298293,122.));
#44451=CARTESIAN_POINT('Ctrl Pts',(33.7802000896882,-87.1647806770501,122.));
#44452=CARTESIAN_POINT('Ctrl Pts',(33.784716145434,-87.1516009164385,122.));
#44453=CARTESIAN_POINT('Ctrl Pts',(33.7893323288939,-87.1384530285915,122.));
#44454=CARTESIAN_POINT('Ctrl Pts',(33.7940451680849,-87.1253476520519,122.));
#44455=CARTESIAN_POINT('Ctrl Pts',(33.8256769306868,-87.0373866284082,122.));
#44456=CARTESIAN_POINT('Ctrl Pts',(33.8616979180992,-86.9512233528443,122.));
#44457=CARTESIAN_POINT('Ctrl Pts',(33.9020435658716,-86.8672720713196,122.));
#44458=CARTESIAN_POINT('Ctrl Pts',(33.9323028017008,-86.8043086101762,122.));
#44459=CARTESIAN_POINT('Ctrl Pts',(33.9649957063116,-86.7425898876219,122.));
#44460=CARTESIAN_POINT('Ctrl Pts',(34.0001110034215,-86.6823061948472,122.));
#44461=CARTESIAN_POINT('Ctrl Pts',(34.0135802871606,-86.6591829912964,122.));
#44462=CARTESIAN_POINT('Ctrl Pts',(34.0274061069814,-86.6362710825671,122.));
#44463=CARTESIAN_POINT('Ctrl Pts',(34.0415883069323,-86.6135818516236,122.));
#44464=CARTESIAN_POINT('Ctrl Pts',(34.051712699879,-86.5973844569652,122.));
#44465=CARTESIAN_POINT('Ctrl Pts',(34.0620195498418,-86.5812994784565,122.));
#44466=CARTESIAN_POINT('Ctrl Pts',(34.0724987247553,-86.5653460621708,122.));
#44467=CARTESIAN_POINT('Ctrl Pts',(34.1196853014102,-86.4935095763133,122.));
#44468=CARTESIAN_POINT('Ctrl Pts',(34.1704068011088,-86.4242665432395,122.));
#44469=CARTESIAN_POINT('Ctrl Pts',(34.2246303322527,-86.3579689632954,122.));
#44470=CARTESIAN_POINT('Ctrl Pts',(34.2734267450191,-86.2983069676984,122.));
#44471=CARTESIAN_POINT('Ctrl Pts',(34.3250598512736,-86.2410304018568,122.));
#44472=CARTESIAN_POINT('Ctrl Pts',(34.3795261720882,-86.1864256058779,122.));
#44473=CARTESIAN_POINT('Ctrl Pts',(34.3986087445119,-86.1672945179254,122.));
#44474=CARTESIAN_POINT('Ctrl Pts',(34.4180392617253,-86.1484916789768,122.));
#44475=CARTESIAN_POINT('Ctrl Pts',(34.4378071488064,-86.1300215764195,122.));
#44476=CARTESIAN_POINT('Origin',(36.3549260746835,-87.7685555885722,114.));
#44477=CARTESIAN_POINT('Origin',(-87.7685555885722,-36.3549260746835,107.));
#44478=CARTESIAN_POINT('Ctrl Pts',(-89.6820215852368,-34.718938871308,107.));
#44479=CARTESIAN_POINT('Ctrl Pts',(-89.7441591022264,-34.7773328792639,
107.));
#44480=CARTESIAN_POINT('Ctrl Pts',(-89.8029212433459,-34.8389807974981,
107.));
#44481=CARTESIAN_POINT('Ctrl Pts',(-89.858296029888,-34.9035061497367,107.));
#44482=CARTESIAN_POINT('Ctrl Pts',(-89.9150258984937,-34.9696105084677,
107.));
#44483=CARTESIAN_POINT('Ctrl Pts',(-89.9682010676987,-35.038735343394,107.));
#44484=CARTESIAN_POINT('Ctrl Pts',(-90.0177797698294,-35.1105221332789,
107.));
#44485=CARTESIAN_POINT('Ctrl Pts',(-90.0307174577489,-35.1292550779578,
107.));
#44486=CARTESIAN_POINT('Ctrl Pts',(-90.0434100690099,-35.1481695083757,
107.));
#44487=CARTESIAN_POINT('Ctrl Pts',(-90.0558564859775,-35.1672594868097,
107.));
#44488=CARTESIAN_POINT('Ctrl Pts',(-90.0660265385985,-35.1828580390446,
107.));
#44489=CARTESIAN_POINT('Ctrl Pts',(-90.0760326568071,-35.1985747060449,
107.));
#44490=CARTESIAN_POINT('Ctrl Pts',(-90.0858653827356,-35.2143916528229,
107.));
#44491=CARTESIAN_POINT('Ctrl Pts',(-90.1333094775083,-35.2907103387503,
107.));
#44492=CARTESIAN_POINT('Ctrl Pts',(-90.1767700081504,-35.3694363854873,
107.));
#44493=CARTESIAN_POINT('Ctrl Pts',(-90.2162122893232,-35.4501772412122,
107.));
#44494=CARTESIAN_POINT('Ctrl Pts',(-90.2480407463799,-35.5153321151888,
107.));
#44495=CARTESIAN_POINT('Ctrl Pts',(-90.2772520626476,-35.5818000994126,
107.));
#44496=CARTESIAN_POINT('Ctrl Pts',(-90.3038108530357,-35.6493927201715,
107.));
#44497=CARTESIAN_POINT('Ctrl Pts',(-90.3144122571216,-35.6763734928431,
107.));
#44498=CARTESIAN_POINT('Ctrl Pts',(-90.3245908384771,-35.7035336109894,
107.));
#44499=CARTESIAN_POINT('Ctrl Pts',(-90.3343435860193,-35.7308616332299,
107.));
#44500=CARTESIAN_POINT('Ctrl Pts',(-90.3395845428334,-35.745547236826,107.));
#44501=CARTESIAN_POINT('Ctrl Pts',(-90.3447021475068,-35.7602805096407,
107.));
#44502=CARTESIAN_POINT('Ctrl Pts',(-90.3496919330262,-35.7750471974551,
107.));
#44503=CARTESIAN_POINT('Ctrl Pts',(-90.379230726078,-35.8624638075913,107.));
#44504=CARTESIAN_POINT('Ctrl Pts',(-90.4043340580788,-35.951161521916,107.));
#44505=CARTESIAN_POINT('Ctrl Pts',(-90.4249693616929,-36.0407425302748,
107.));
#44506=CARTESIAN_POINT('Ctrl Pts',(-90.4459261369105,-36.1317190960213,
107.));
#44507=CARTESIAN_POINT('Ctrl Pts',(-90.4622750877517,-36.2236074967956,
107.));
#44508=CARTESIAN_POINT('Ctrl Pts',(-90.4739402758961,-36.3160242249173,
107.));
#44509=CARTESIAN_POINT('Ctrl Pts',(-90.4855147505546,-36.4077222810838,
107.));
#44510=CARTESIAN_POINT('Ctrl Pts',(-90.492478369332,-36.4999414095043,107.));
#44511=CARTESIAN_POINT('Ctrl Pts',(-90.4947100072084,-36.5923261901315,
107.));
#44512=CARTESIAN_POINT('Ctrl Pts',(-90.4958206266717,-36.6383033339006,
107.));
#44513=CARTESIAN_POINT('Ctrl Pts',(-90.4957584865878,-36.6843217187953,
107.));
#44514=CARTESIAN_POINT('Ctrl Pts',(-90.494503858864,-36.7303382342054,107.));
#44515=CARTESIAN_POINT('Ctrl Pts',(-90.4941340858137,-36.7439005578688,
107.));
#44516=CARTESIAN_POINT('Ctrl Pts',(-90.4936607061271,-36.7574627198223,
107.));
#44517=CARTESIAN_POINT('Ctrl Pts',(-90.4930831583726,-36.7710236163914,
107.));
#44518=CARTESIAN_POINT('Ctrl Pts',(-90.4924626435032,-36.785593386418,107.));
#44519=CARTESIAN_POINT('Ctrl Pts',(-90.491722287192,-36.8001519099739,107.));
#44520=CARTESIAN_POINT('Ctrl Pts',(-90.4908620410004,-36.8146952575918,
107.));
#44521=CARTESIAN_POINT('Ctrl Pts',(-90.4852102271911,-36.9102449894035,
107.));
#44522=CARTESIAN_POINT('Ctrl Pts',(-90.4743857795999,-37.0051729993,107.));
#44523=CARTESIAN_POINT('Ctrl Pts',(-90.458318244262,-37.0990836424695,107.));
#44524=CARTESIAN_POINT('Ctrl Pts',(-90.4559379034287,-37.1129961271111,
107.));
#44525=CARTESIAN_POINT('Ctrl Pts',(-90.4534424042812,-37.1268863168099,
107.));
#44526=CARTESIAN_POINT('Ctrl Pts',(-90.4508314252251,-37.1407529558637,
107.));
#44527=CARTESIAN_POINT('Ctrl Pts',(-90.433885764654,-37.2307496021864,107.));
#44528=CARTESIAN_POINT('Ctrl Pts',(-90.4120802238171,-37.3197540702518,
107.));
#44529=CARTESIAN_POINT('Ctrl Pts',(-90.385717351839,-37.4075341124589,107.));
#44530=CARTESIAN_POINT('Ctrl Pts',(-90.3587585371945,-37.4972984556344,
107.));
#44531=CARTESIAN_POINT('Ctrl Pts',(-90.3270338130467,-37.5857830902758,
107.));
#44532=CARTESIAN_POINT('Ctrl Pts',(-90.2908124720421,-37.6727359721983,
107.));
#44533=CARTESIAN_POINT('Ctrl Pts',(-90.2783223243084,-37.7027197969535,
107.));
#44534=CARTESIAN_POINT('Ctrl Pts',(-90.2652970490218,-37.7325214049852,
107.));
#44535=CARTESIAN_POINT('Ctrl Pts',(-90.2517463158813,-37.7621301223255,
107.));
#44536=CARTESIAN_POINT('Ctrl Pts',(-90.245055229323,-37.7767503268968,107.));
#44537=CARTESIAN_POINT('Ctrl Pts',(-90.2382360157698,-37.7913234975559,
107.));
#44538=CARTESIAN_POINT('Ctrl Pts',(-90.2312897801449,-37.8058483267084,
107.));
#44539=CARTESIAN_POINT('Ctrl Pts',(-90.2257960066309,-37.8173360052153,
107.));
#44540=CARTESIAN_POINT('Ctrl Pts',(-90.220223218393,-37.8287924197308,107.));
#44541=CARTESIAN_POINT('Ctrl Pts',(-90.2145765560449,-37.840207994202,107.));
#44542=CARTESIAN_POINT('Ctrl Pts',(-90.1718526024324,-37.926580871506,107.));
#44543=CARTESIAN_POINT('Ctrl Pts',(-90.1248377921968,-38.0107554256567,
107.));
#44544=CARTESIAN_POINT('Ctrl Pts',(-90.0738747799873,-38.0924820198704,
107.));
#44545=CARTESIAN_POINT('Ctrl Pts',(-90.0219010618754,-38.1758294278385,
107.));
#44546=CARTESIAN_POINT('Ctrl Pts',(-89.9658206725573,-38.2566315879641,
107.));
#44547=CARTESIAN_POINT('Ctrl Pts',(-89.9059420505749,-38.3346166852078,
107.));
#44548=CARTESIAN_POINT('Ctrl Pts',(-89.8455766045364,-38.4132358154351,
107.));
#44549=CARTESIAN_POINT('Ctrl Pts',(-89.7813504553299,-38.4889927268592,
107.));
#44550=CARTESIAN_POINT('Ctrl Pts',(-89.7135302947394,-38.5615896410769,
107.));
#44551=CARTESIAN_POINT('Ctrl Pts',(-89.6765296427799,-38.6011963470019,
107.));
#44552=CARTESIAN_POINT('Ctrl Pts',(-89.6384584284845,-38.6398620818104,
107.));
#44553=CARTESIAN_POINT('Ctrl Pts',(-89.5993546106677,-38.6775347115697,
107.));
#44554=CARTESIAN_POINT('Ctrl Pts',(-89.5873868339339,-38.6890644712479,
107.));
#44555=CARTESIAN_POINT('Ctrl Pts',(-89.5753223113711,-38.7005011869721,
107.));
#44556=CARTESIAN_POINT('Ctrl Pts',(-89.5631620681302,-38.7118433021718,
107.));
#44557=CARTESIAN_POINT('Ctrl Pts',(-89.5526162948829,-38.7216795671767,
107.));
#44558=CARTESIAN_POINT('Ctrl Pts',(-89.5419996446347,-38.7314435662217,
107.));
#44559=CARTESIAN_POINT('Ctrl Pts',(-89.531321897357,-38.7411263062964,107.));
#44560=CARTESIAN_POINT('Ctrl Pts',(-89.4557474041478,-38.8096583809928,
107.));
#44561=CARTESIAN_POINT('Ctrl Pts',(-89.3769961916351,-38.8742341081678,
107.));
#44562=CARTESIAN_POINT('Ctrl Pts',(-89.2953956054652,-38.9345717165341,
107.));
#44563=CARTESIAN_POINT('Ctrl Pts',(-89.2136908377845,-38.9949863594351,
107.));
#44564=CARTESIAN_POINT('Ctrl Pts',(-89.1291288426842,-39.051152893352,107.));
#44565=CARTESIAN_POINT('Ctrl Pts',(-89.0419929468074,-39.102762666281,107.));
#44566=CARTESIAN_POINT('Ctrl Pts',(-88.9565892880383,-39.1533464514366,
107.));
#44567=CARTESIAN_POINT('Ctrl Pts',(-88.8687123840793,-39.1995535268664,
107.));
#44568=CARTESIAN_POINT('Ctrl Pts',(-88.7785949084889,-39.2410574806785,
107.));
#44569=CARTESIAN_POINT('Ctrl Pts',(-88.7382460236614,-39.2596403164856,
107.));
#44570=CARTESIAN_POINT('Ctrl Pts',(-88.6974475743233,-39.2772797819957,
107.));
#44571=CARTESIAN_POINT('Ctrl Pts',(-88.6562186908398,-39.2939436323372,
107.));
#44572=CARTESIAN_POINT('Ctrl Pts',(-88.6257990519939,-39.3062386126117,
107.));
#44573=CARTESIAN_POINT('Ctrl Pts',(-88.595145068204,-39.3180024402984,107.));
#44574=CARTESIAN_POINT('Ctrl Pts',(-88.5642690084499,-39.3292377960812,
107.));
#44575=CARTESIAN_POINT('Ctrl Pts',(-86.97475630604,-39.3241490284294,107.));
#44576=CARTESIAN_POINT('Ctrl Pts',(-86.8799223996403,-39.2894583618481,
107.));
#44577=CARTESIAN_POINT('Ctrl Pts',(-86.7871316469804,-39.2497768123283,
107.));
#44578=CARTESIAN_POINT('Ctrl Pts',(-86.6966249712659,-39.2054247302432,
107.));
#44579=CARTESIAN_POINT('Ctrl Pts',(-86.6048454170698,-39.1604488841048,
107.));
#44580=CARTESIAN_POINT('Ctrl Pts',(-86.515413969275,-39.1106695078317,107.));
#44581=CARTESIAN_POINT('Ctrl Pts',(-86.4286158841239,-39.0563799760475,
107.));
#44582=CARTESIAN_POINT('Ctrl Pts',(-86.4041028655354,-39.0410478371015,
107.));
#44583=CARTESIAN_POINT('Ctrl Pts',(-86.3798001181766,-39.0253557682571,
107.));
#44584=CARTESIAN_POINT('Ctrl Pts',(-86.3557146636652,-39.009309921962,107.));
#44585=CARTESIAN_POINT('Ctrl Pts',(-86.3363851178117,-38.9964324850188,
107.));
#44586=CARTESIAN_POINT('Ctrl Pts',(-86.3171934197275,-38.9833255643263,
107.));
#44587=CARTESIAN_POINT('Ctrl Pts',(-86.2981624849453,-38.9700061049476,
107.));
#44588=CARTESIAN_POINT('Ctrl Pts',(-86.215455383929,-38.912120673416,107.));
#44589=CARTESIAN_POINT('Ctrl Pts',(-86.1357031424774,-38.8501730961047,
107.));
#44590=CARTESIAN_POINT('Ctrl Pts',(-86.0591721222282,-38.7844607338344,
107.));
#44591=CARTESIAN_POINT('Ctrl Pts',(-86.0001789319485,-38.7338070005048,
107.));
#44592=CARTESIAN_POINT('Ctrl Pts',(-85.943100409209,-38.6809153408518,107.));
#44593=CARTESIAN_POINT('Ctrl Pts',(-85.8880761219746,-38.6259101852584,
107.));
#44594=CARTESIAN_POINT('Ctrl Pts',(-85.8587873766259,-38.5966316234449,
107.));
#44595=CARTESIAN_POINT('Ctrl Pts',(-85.8300809343862,-38.5667540958584,
107.));
#44596=CARTESIAN_POINT('Ctrl Pts',(-85.8019798655343,-38.5362955369464,
107.));
#44597=CARTESIAN_POINT('Ctrl Pts',(-85.7923438617004,-38.5258511374114,
107.));
#44598=CARTESIAN_POINT('Ctrl Pts',(-85.7827797735159,-38.5153391259719,
107.));
#44599=CARTESIAN_POINT('Ctrl Pts',(-85.7732951676183,-38.5047678383442,
107.));
#44600=CARTESIAN_POINT('Ctrl Pts',(-85.7074979757394,-38.4314320510738,
107.));
#44601=CARTESIAN_POINT('Ctrl Pts',(-85.6454329342682,-38.3551496402824,
107.));
#44602=CARTESIAN_POINT('Ctrl Pts',(-85.5873438118379,-38.276199164193,107.));
#44603=CARTESIAN_POINT('Ctrl Pts',(-85.5297811470021,-38.197964210666,107.));
#44604=CARTESIAN_POINT('Ctrl Pts',(-85.4761222269613,-38.1171085490677,
107.));
#44605=CARTESIAN_POINT('Ctrl Pts',(-85.4266499956721,-38.0338808467508,
107.));
#44606=CARTESIAN_POINT('Ctrl Pts',(-85.3785920566061,-37.9530324244677,
107.));
#44607=CARTESIAN_POINT('Ctrl Pts',(-85.3344846447919,-37.8699449457437,
107.));
#44608=CARTESIAN_POINT('Ctrl Pts',(-85.2946349115255,-37.7848360318206,
107.));
#44609=CARTESIAN_POINT('Ctrl Pts',(-85.273830494568,-37.7404030786508,107.));
#44610=CARTESIAN_POINT('Ctrl Pts',(-85.2541873635994,-37.6954190560072,
107.));
#44611=CARTESIAN_POINT('Ctrl Pts',(-85.2357549187479,-37.6499146945858,
107.));
#44612=CARTESIAN_POINT('Ctrl Pts',(-85.2286968353362,-37.6324903332981,
107.));
#44613=CARTESIAN_POINT('Ctrl Pts',(-85.2218163113607,-37.6149896785989,
107.));
#44614=CARTESIAN_POINT('Ctrl Pts',(-85.2151162824064,-37.597414464605,107.));
#44615=CARTESIAN_POINT('Ctrl Pts',(-85.2098745474931,-37.5836645818168,
107.));
#44616=CARTESIAN_POINT('Ctrl Pts',(-85.2047431886565,-37.5698685631309,
107.));
#44617=CARTESIAN_POINT('Ctrl Pts',(-85.1997287410707,-37.5560419518582,
107.));
#44618=CARTESIAN_POINT('Ctrl Pts',(-85.1680450550389,-37.4686787871323,
107.));
#44619=CARTESIAN_POINT('Ctrl Pts',(-85.1409701945636,-37.3799546783075,
107.));
#44620=CARTESIAN_POINT('Ctrl Pts',(-85.1187554157791,-37.2900931766429,
107.));
#44621=CARTESIAN_POINT('Ctrl Pts',(-85.1137714424873,-37.2699323941024,
107.));
#44622=CARTESIAN_POINT('Ctrl Pts',(-85.1090323031209,-37.2497143216185,
107.));
#44623=CARTESIAN_POINT('Ctrl Pts',(-85.1045411958224,-37.2294414281565,
107.));
#44624=CARTESIAN_POINT('Ctrl Pts',(-85.0841754438542,-37.1375102645286,
107.));
#44625=CARTESIAN_POINT('Ctrl Pts',(-85.0689059044723,-37.0444514795905,
107.));
#44626=CARTESIAN_POINT('Ctrl Pts',(-85.0586227526078,-36.950656660602,107.));
#44627=CARTESIAN_POINT('Ctrl Pts',(-85.0478888926271,-36.8527508368625,
107.));
#44628=CARTESIAN_POINT('Ctrl Pts',(-85.0425881162133,-36.7540418071215,
107.));
#44629=CARTESIAN_POINT('Ctrl Pts',(-85.0426529761227,-36.654989588785,107.));
#44630=CARTESIAN_POINT('Ctrl Pts',(-85.0426783462698,-36.6162450179075,
107.));
#44631=CARTESIAN_POINT('Ctrl Pts',(-85.0435252614424,-36.5774481957561,
107.));
#44632=CARTESIAN_POINT('Ctrl Pts',(-85.0451919090303,-36.5386278801149,
107.));
#44633=CARTESIAN_POINT('Ctrl Pts',(-85.045724948488,-36.5262120819881,107.));
#44634=CARTESIAN_POINT('Ctrl Pts',(-85.0463418344278,-36.5137951920582,
107.));
#44635=CARTESIAN_POINT('Ctrl Pts',(-85.0470418057235,-36.5013878196786,
107.));
#44636=CARTESIAN_POINT('Ctrl Pts',(-85.0522810236674,-36.4085198286572,
107.));
#44637=CARTESIAN_POINT('Ctrl Pts',(-85.062176662527,-36.3160350692795,107.));
#44638=CARTESIAN_POINT('Ctrl Pts',(-85.0766052632011,-36.2243051192734,
107.));
#44639=CARTESIAN_POINT('Ctrl Pts',(-85.0909998752463,-36.1327912522612,
107.));
#44640=CARTESIAN_POINT('Ctrl Pts',(-85.1099065280918,-36.0420276973609,
107.));
#44641=CARTESIAN_POINT('Ctrl Pts',(-85.1332513090946,-35.9524003649907,
107.));
#44642=CARTESIAN_POINT('Ctrl Pts',(-85.156199939792,-35.8642939676463,107.));
#44643=CARTESIAN_POINT('Ctrl Pts',(-85.1834378181195,-35.7772847723475,
107.));
#44644=CARTESIAN_POINT('Ctrl Pts',(-85.2149351717563,-35.6917684721328,
107.));
#44645=CARTESIAN_POINT('Ctrl Pts',(-85.230776616366,-35.6487584545708,107.));
#44646=CARTESIAN_POINT('Ctrl Pts',(-85.2476961109153,-35.6061266053731,
107.));
#44647=CARTESIAN_POINT('Ctrl Pts',(-85.2656932851445,-35.5639270559061,
107.));
#44648=CARTESIAN_POINT('Ctrl Pts',(-85.2712589917432,-35.5508766565523,
107.));
#44649=CARTESIAN_POINT('Ctrl Pts',(-85.2769277813298,-35.5378676223478,
107.));
#44650=CARTESIAN_POINT('Ctrl Pts',(-85.2826996838302,-35.5249016119162,
107.));
#44651=CARTESIAN_POINT('Ctrl Pts',(-85.2883791474132,-35.5121432564074,
107.));
#44652=CARTESIAN_POINT('Ctrl Pts',(-85.2941549663054,-35.499434422109,107.));
#44653=CARTESIAN_POINT('Ctrl Pts',(-85.3000253507934,-35.486779594601,107.));
#44654=CARTESIAN_POINT('Ctrl Pts',(-85.3375051537983,-35.4059841300047,
107.));
#44655=CARTESIAN_POINT('Ctrl Pts',(-85.3788551133841,-35.3273454443705,
107.));
#44656=CARTESIAN_POINT('Ctrl Pts',(-85.4240055532635,-35.2512111292096,
107.));
#44657=CARTESIAN_POINT('Ctrl Pts',(-85.4683985586388,-35.1763540276795,
107.));
#44658=CARTESIAN_POINT('Ctrl Pts',(-85.5164660558066,-35.103917306336,107.));
#44659=CARTESIAN_POINT('Ctrl Pts',(-85.5681780296166,-35.0342655325047,
107.));
#44660=CARTESIAN_POINT('Ctrl Pts',(-85.6183124836241,-34.9667385480481,
107.));
#44661=CARTESIAN_POINT('Ctrl Pts',(-85.6718728926839,-34.901828747048,107.));
#44662=CARTESIAN_POINT('Ctrl Pts',(-85.7288596163099,-34.8399086244755,
107.));
#44663=CARTESIAN_POINT('Ctrl Pts',(-85.7498272120257,-34.8171258425545,
107.));
#44664=CARTESIAN_POINT('Ctrl Pts',(-85.7712589016926,-34.7947482334293,
107.));
#44665=CARTESIAN_POINT('Ctrl Pts',(-85.7931555144105,-34.7727959615648,
107.));
#44666=CARTESIAN_POINT('Ctrl Pts',(-85.8122329504701,-34.7536700324426,
107.));
#44667=CARTESIAN_POINT('Ctrl Pts',(-85.8316633199033,-34.7348669902236,
107.));
#44668=CARTESIAN_POINT('Ctrl Pts',(-85.8514364858567,-34.7163919634216,
107.));
#44669=CARTESIAN_POINT('Origin',(-87.7685555885722,-36.3549260746835,124.208423447177));
#44670=CARTESIAN_POINT('Ctrl Pts',(-90.8453551362697,-36.3529984899081,
121.708423447177));
#44671=CARTESIAN_POINT('Ctrl Pts',(-90.8462778186642,-36.2297235877034,
121.702019850418));
#44672=CARTESIAN_POINT('Ctrl Pts',(-90.7837513605892,-35.0938167757587,
121.642966745928));
#44673=CARTESIAN_POINT('Ctrl Pts',(-89.3710243173134,-33.1013875956417,
121.531264133707));
#44674=CARTESIAN_POINT('Ctrl Pts',(-85.9203582039126,-33.2347629349336,
121.373315610515));
#44675=CARTESIAN_POINT('Ctrl Pts',(-84.1454681337529,-36.1967043012439,
121.215367087322));
#44676=CARTESIAN_POINT('Ctrl Pts',(-85.6554864122685,-39.3022906545617,
121.05741856413));
#44677=CARTESIAN_POINT('Ctrl Pts',(-89.0813771948967,-39.735498741376,120.899470040937));
#44678=CARTESIAN_POINT('Ctrl Pts',(-90.7279241675112,-37.7971275010703,
120.783138335286));
#44679=CARTESIAN_POINT('Ctrl Pts',(-90.8448017962344,-36.5704857415671,
120.719456137367));
#44680=CARTESIAN_POINT('Ctrl Pts',(-90.8428699659751,-36.357609793043,120.708423447177));
#44681=CARTESIAN_POINT('Ctrl Pts',(-90.8388341582581,-36.3579404435482,
121.791576552823));
#44682=CARTESIAN_POINT('Ctrl Pts',(-90.8338492651609,-35.6649221393835,
121.755752019753));
#44683=CARTESIAN_POINT('Ctrl Pts',(-90.2614620369657,-33.9437331486761,
121.667277978953));
#44684=CARTESIAN_POINT('Ctrl Pts',(-87.417021209647,-32.7460642638912,121.526154430423));
#44685=CARTESIAN_POINT('Ctrl Pts',(-84.5546283385357,-34.6751866943283,
121.36820590723));
#44686=CARTESIAN_POINT('Ctrl Pts',(-84.6050187185395,-38.1284686676829,
121.210257384038));
#44687=CARTESIAN_POINT('Ctrl Pts',(-87.5242687364515,-39.9731543606838,
121.052308860845));
#44688=CARTESIAN_POINT('Ctrl Pts',(-90.2991160808229,-38.7047120741592,
120.912748583773));
#44689=CARTESIAN_POINT('Ctrl Pts',(-90.8346458997654,-37.0159745254743,
120.825837814433));
#44690=CARTESIAN_POINT('Ctrl Pts',(-90.8389971204791,-36.3527751889037,
120.791576552823));
#44691=CARTESIAN_POINT('Ctrl Pts',(-85.855089591907,-34.7189388713087,122.));
#44692=CARTESIAN_POINT('Ctrl Pts',(-85.3138942055855,-35.3519260775303,
121.947350492269));
#44693=CARTESIAN_POINT('Ctrl Pts',(-84.9185558383608,-37.1869577282907,
121.842051476807));
#44694=CARTESIAN_POINT('Ctrl Pts',(-86.9093548370361,-39.2001258698145,
121.684102953615));
#44695=CARTESIAN_POINT('Ctrl Pts',(-89.6802577024474,-38.6278810997191,
121.526154430422));
#44696=CARTESIAN_POINT('Ctrl Pts',(-90.7173747954316,-35.9976145147108,
121.36820590723));
#44697=CARTESIAN_POINT('Ctrl Pts',(-89.081135716962,-33.6899567820244,121.210257384038));
#44698=CARTESIAN_POINT('Ctrl Pts',(-86.2546994259301,-33.7992043553666,
121.052308860845));
#44699=CARTESIAN_POINT('Ctrl Pts',(-84.8008891927669,-36.2253268182546,
120.894360337653));
#44700=CARTESIAN_POINT('Ctrl Pts',(-86.0377432731843,-38.7691087100644,
120.73641181446));
#44701=CARTESIAN_POINT('Ctrl Pts',(-88.8438861218152,-39.1239489113188,
120.578463291268));
#44702=CARTESIAN_POINT('Ctrl Pts',(-90.675052730646,-36.9682371400777,120.420514768075));
#44703=CARTESIAN_POINT('Ctrl Pts',(-89.8709900599802,-34.2564369768315,
120.262566244883));
#44704=CARTESIAN_POINT('Ctrl Pts',(-87.1607124008595,-33.4472817605808,
120.10461772169));
#44705=CARTESIAN_POINT('Ctrl Pts',(-85.0015484493013,-35.2743949794042,
119.946669198498));
#44706=CARTESIAN_POINT('Ctrl Pts',(-85.3511453388923,-38.0811949374583,
119.788720675305));
#44707=CARTESIAN_POINT('Ctrl Pts',(-87.892534763121,-39.3228384190479,119.630772152113));
#44708=CARTESIAN_POINT('Ctrl Pts',(-90.3215159512363,-37.8735665295443,
119.472823628921));
#44709=CARTESIAN_POINT('Ctrl Pts',(-90.4358056666791,-35.0473892903923,
119.314875105728));
#44710=CARTESIAN_POINT('Ctrl Pts',(-88.1317808359558,-33.4067160016613,
119.156926582536));
#44711=CARTESIAN_POINT('Ctrl Pts',(-85.4984307306815,-34.4390950644477,
118.998978059343));
#44712=CARTESIAN_POINT('Ctrl Pts',(-84.9233337863437,-37.2084998640467,
118.841029536151));
#44713=CARTESIAN_POINT('Ctrl Pts',(-86.9279129190018,-39.2039952558787,
118.683081012958));
#44714=CARTESIAN_POINT('Ctrl Pts',(-89.6946771919892,-38.6163262780736,
118.525132489766));
#44715=CARTESIAN_POINT('Ctrl Pts',(-90.7150855880725,-35.9783145101063,
118.367183966573));
#44716=CARTESIAN_POINT('Ctrl Pts',(-89.063964847989,-33.6817649951384,118.209235443381));
#44717=CARTESIAN_POINT('Ctrl Pts',(-86.2383359306196,-33.8088893297358,
118.051286920188));
#44718=CARTESIAN_POINT('Ctrl Pts',(-84.8001106375229,-36.2444277471294,
117.893338396996));
#44719=CARTESIAN_POINT('Ctrl Pts',(-86.0532841004025,-38.7801516372869,
117.735389873803));
#44720=CARTESIAN_POINT('Ctrl Pts',(-88.861642053966,-39.1169972698181,117.577441350611));
#44721=CARTESIAN_POINT('Ctrl Pts',(-90.6789317540865,-36.9495569542776,
117.419492827418));
#44722=CARTESIAN_POINT('Ctrl Pts',(-89.8574719000215,-34.2429829051099,
117.261544304226));
#44723=CARTESIAN_POINT('Ctrl Pts',(-87.1420551578849,-33.4512434959369,
117.103595781033));
#44724=CARTESIAN_POINT('Ctrl Pts',(-84.9946673021025,-35.2921847694046,
116.945647257841));
#44725=CARTESIAN_POINT('Ctrl Pts',(-85.3622795916639,-38.0966812625507,
116.787698734649));
#44726=CARTESIAN_POINT('Ctrl Pts',(-87.9115891440455,-39.3219812999482,
116.629750211456));
#44727=CARTESIAN_POINT('Ctrl Pts',(-90.3312145218488,-37.8571426035032,
116.471801688264));
#44728=CARTESIAN_POINT('Ctrl Pts',(-90.4273549845983,-35.0302898682282,
116.313853165071));
#44729=CARTESIAN_POINT('Ctrl Pts',(-88.1128428986993,-33.4044444943569,
116.155904641879));
#44730=CARTESIAN_POINT('Ctrl Pts',(-85.4861759797334,-34.453711034527,115.997956118686));
#44731=CARTESIAN_POINT('Ctrl Pts',(-84.9288732366636,-37.2267514287653,
115.840007595494));
#44732=CARTESIAN_POINT('Ctrl Pts',(-86.9462241170348,-39.2093342898272,
115.682059072301));
#44733=CARTESIAN_POINT('Ctrl Pts',(-89.7091579325677,-38.6039120351199,
115.524110549109));
#44734=CARTESIAN_POINT('Ctrl Pts',(-90.7126066235523,-35.959402609901,115.366162025916));
#44735=CARTESIAN_POINT('Ctrl Pts',(-89.0467737803853,-33.673502280898,115.208213502724));
#44736=CARTESIAN_POINT('Ctrl Pts',(-86.2220193779501,-33.818767353902,115.050264979531));
#44737=CARTESIAN_POINT('Ctrl Pts',(-84.7994623219137,-36.263490405258,114.892316456339));
#44738=CARTESIAN_POINT('Ctrl Pts',(-86.0688918298665,-38.7911153971918,
114.734367933147));
#44739=CARTESIAN_POINT('Ctrl Pts',(-88.8793547749015,-39.1099216237564,
114.576419409954));
#44740=CARTESIAN_POINT('Ctrl Pts',(-90.6826898811218,-36.9308571753786,
114.418470886762));
#44741=CARTESIAN_POINT('Ctrl Pts',(-89.8438680536754,-34.2296135141532,
114.260522363569));
#44742=CARTESIAN_POINT('Ctrl Pts',(-87.1234235318957,-33.455326113101,114.102573840377));
#44743=CARTESIAN_POINT('Ctrl Pts',(-84.9879006250997,-35.3100178098693,
113.944625317184));
#44744=CARTESIAN_POINT('Ctrl Pts',(-85.3735130038868,-38.1120960508962,
113.786676793992));
#44745=CARTESIAN_POINT('Ctrl Pts',(-87.9306376522803,-39.3210017164002,
113.628728270799));
#44746=CARTESIAN_POINT('Ctrl Pts',(-90.3408074230132,-37.8406568066725,
113.470779747607));
#44747=CARTESIAN_POINT('Ctrl Pts',(-90.4187946869615,-35.013245028708,113.312831224414));
#44748=CARTESIAN_POINT('Ctrl Pts',(-88.093890763779,-33.4022946497451,113.154882701222));
#44749=CARTESIAN_POINT('Ctrl Pts',(-85.4740153318585,-34.4684053835483,
112.996934178029));
#44750=CARTESIAN_POINT('Ctrl Pts',(-84.9345297654133,-37.2449670520707,
112.838985654837));
#44751=CARTESIAN_POINT('Ctrl Pts',(-86.9645692198269,-39.2145556357687,
112.681037131644));
#44752=CARTESIAN_POINT('Ctrl Pts',(-89.7235586626422,-38.5914050681325,
112.523088608452));
#44753=CARTESIAN_POINT('Ctrl Pts',(-90.7100062769287,-35.9405070165698,
112.365140085259));
#44754=CARTESIAN_POINT('Ctrl Pts',(-89.0295300122615,-33.6653501210131,
112.207191562067));
#44755=CARTESIAN_POINT('Ctrl Pts',(-86.2057665884384,-33.8287499428941,
112.049243038875));
#44756=CARTESIAN_POINT('Ctrl Pts',(-84.7989364209583,-36.282556833295,111.891294515682));
#44757=CARTESIAN_POINT('Ctrl Pts',(-86.0845696358685,-38.8019787138511,
111.73334599249));
#44758=CARTESIAN_POINT('Ctrl Pts',(-88.8970216979793,-39.1027323902174,
111.575397469297));
#44759=CARTESIAN_POINT('Ctrl Pts',(-90.6863278594327,-36.9121336510371,
111.417448946105));
#44760=CARTESIAN_POINT('Ctrl Pts',(-89.830178642936,-34.2163317490865,111.259500422912));
#44761=CARTESIAN_POINT('Ctrl Pts',(-87.1048185044643,-33.4595282797339,
111.10155189972));
#44762=CARTESIAN_POINT('Ctrl Pts',(-84.9812485935319,-35.3278939315487,
110.943603376527));
#44763=CARTESIAN_POINT('Ctrl Pts',(-85.3848451628316,-38.1274383917119,
110.785654853335));
#44764=CARTESIAN_POINT('Ctrl Pts',(-87.949679478,-39.3198998426766,110.627706330142));
#44765=CARTESIAN_POINT('Ctrl Pts',(-90.3502942710008,-37.824109753544,110.46975780695));
#44766=CARTESIAN_POINT('Ctrl Pts',(-90.4101251212064,-34.9962555065228,
110.311809283757));
#44767=CARTESIAN_POINT('Ctrl Pts',(-88.0749252147876,-33.4002665404604,
110.153860760565));
#44768=CARTESIAN_POINT('Ctrl Pts',(-85.4619492883336,-34.4831775144226,
109.995912237372));
#44769=CARTESIAN_POINT('Ctrl Pts',(-84.9403031374328,-37.2631459766827,
109.83796371418));
#44770=CARTESIAN_POINT('Ctrl Pts',(-86.982947476059,-39.219659085585,109.680015190988));
#44771=CARTESIAN_POINT('Ctrl Pts',(-89.737878777595,-38.5788058808295,109.522066667795));
#44772=CARTESIAN_POINT('Ctrl Pts',(-90.7072846780369,-35.9216285323762,
109.364118144603));
#44773=CARTESIAN_POINT('Ctrl Pts',(-89.0122342079233,-33.6573088045276,
109.20616962141));
#44774=CARTESIAN_POINT('Ctrl Pts',(-86.1895783281781,-33.8388367816117,
109.048221098218));
#44775=CARTESIAN_POINT('Ctrl Pts',(-84.7985327588824,-36.3016260468753,
108.890272575025));
#44776=CARTESIAN_POINT('Ctrl Pts',(-86.1003172781239,-38.8127415470481,
108.732324051833));
#44777=CARTESIAN_POINT('Ctrl Pts',(-88.914641259591,-39.0954290272211,108.57437552864));
#44778=CARTESIAN_POINT('Ctrl Pts',(-90.6898472567247,-36.8933888774387,
108.416427005448));
#44779=CARTESIAN_POINT('Ctrl Pts',(-89.8164006995781,-34.2031346114724,
108.258478482255));
#44780=CARTESIAN_POINT('Ctrl Pts',(-87.0862481079167,-33.463857115393,108.100529959063));
#44781=CARTESIAN_POINT('Ctrl Pts',(-84.9746965398898,-35.3457973989596,
107.94258143587));
#44782=CARTESIAN_POINT('Ctrl Pts',(-85.396306330652,-38.1427384983891,107.784632912678));
#44783=CARTESIAN_POINT('Ctrl Pts',(-87.9686506378239,-39.3186122859791,
107.626684389485));
#44784=CARTESIAN_POINT('Ctrl Pts',(-90.3598046494548,-37.8076325931292,
107.468735866293));
#44785=CARTESIAN_POINT('Ctrl Pts',(-90.401079337765,-34.9790536330783,107.3107873431));
#44786=CARTESIAN_POINT('Ctrl Pts',(-88.0564969547953,-33.3989119868201,
107.152838819908));
#44787=CARTESIAN_POINT('Ctrl Pts',(-85.4488473177177,-34.4968783509201,
106.994890296716));
#44788=CARTESIAN_POINT('Ctrl Pts',(-84.9485679810268,-37.2836053207636,
106.836941773523));
#44789=CARTESIAN_POINT('Ctrl Pts',(-86.3138051921105,-38.5719224173531,
106.731642758061));
#44790=CARTESIAN_POINT('Ctrl Pts',(-87.1183555905977,-38.7870128767187,
106.678993250331));
#44791=CARTESIAN_POINT('Ctrl Pts',(-85.71422403823,-34.5985007534569,122.10700224989));
#44792=CARTESIAN_POINT('Ctrl Pts',(-85.133186926017,-35.2780872164357,122.054352742159));
#44793=CARTESIAN_POINT('Ctrl Pts',(-84.708744535995,-37.2482102406252,121.949053726697));
#44794=CARTESIAN_POINT('Ctrl Pts',(-86.8461021898526,-39.4095838090522,
121.791105203505));
#44795=CARTESIAN_POINT('Ctrl Pts',(-89.8209934025883,-38.7952115193046,
121.633156680312));
#44796=CARTESIAN_POINT('Ctrl Pts',(-90.9344609892766,-35.9713099496867,
121.47520815712));
#44797=CARTESIAN_POINT('Ctrl Pts',(-89.1777652504124,-33.4937670532302,
121.317259633927));
#44798=CARTESIAN_POINT('Ctrl Pts',(-86.1432523519242,-33.6110572152223,
121.159311110735));
#44799=CARTESIAN_POINT('Ctrl Pts',(-84.5824155064289,-36.215785979251,121.001362587543));
#44800=CARTESIAN_POINT('Ctrl Pts',(-85.9103243195458,-38.9468360248968,
120.84341406435));
#44801=CARTESIAN_POINT('Ctrl Pts',(-88.9230498128423,-39.3277988546712,
120.685465541158));
#44802=CARTESIAN_POINT('Ctrl Pts',(-90.8890232584176,-37.0133878785563,
120.527517017965));
#44803=CARTESIAN_POINT('Ctrl Pts',(-90.0257670962068,-34.1019503911438,
120.369568494773));
#44804=CARTESIAN_POINT('Ctrl Pts',(-87.11596419664,-33.2332267802908,120.21161997158));
#44805=CARTESIAN_POINT('Ctrl Pts',(-84.7978468975721,-35.1948484333631,
120.053671448388));
#44806=CARTESIAN_POINT('Ctrl Pts',(-85.173180413527,-38.2082794111694,119.895722925195));
#44807=CARTESIAN_POINT('Ctrl Pts',(-87.9016618628959,-39.5413302116287,
119.737774402003));
#44808=CARTESIAN_POINT('Ctrl Pts',(-90.5094598058065,-37.9853658136096,
119.57982587881));
#44809=CARTESIAN_POINT('Ctrl Pts',(-90.632163302353,-34.9511310378844,119.421877355618));
#44810=CARTESIAN_POINT('Ctrl Pts',(-88.1585207548627,-33.1896746510356,
119.263928832425));
#44811=CARTESIAN_POINT('Ctrl Pts',(-85.3313086623614,-34.2980554031843,
119.105980309233));
#44812=CARTESIAN_POINT('Ctrl Pts',(-84.7138742269874,-37.2713382654881,
118.948031786041));
#44813=CARTESIAN_POINT('Ctrl Pts',(-86.8660264808315,-39.4137380516079,
118.790083262848));
#44814=CARTESIAN_POINT('Ctrl Pts',(-89.8364744262163,-38.7828060547151,
118.632134739655));
#44815=CARTESIAN_POINT('Ctrl Pts',(-90.9320032550333,-35.9505891172026,
118.474186216463));
#44816=CARTESIAN_POINT('Ctrl Pts',(-89.1593302962823,-33.4849722033175,
118.316237693271));
#44817=CARTESIAN_POINT('Ctrl Pts',(-86.1256842086968,-33.6214551781051,
118.158289170078));
#44818=CARTESIAN_POINT('Ctrl Pts',(-84.5815796354993,-36.2362930804469,
118.000340646886));
#44819=CARTESIAN_POINT('Ctrl Pts',(-85.9270092314952,-38.958691910416,117.842392123693));
#44820=CARTESIAN_POINT('Ctrl Pts',(-88.9421129013356,-39.3203354471759,
117.684443600501));
#44821=CARTESIAN_POINT('Ctrl Pts',(-90.8931878478337,-36.9933324947018,
117.526495077308));
#44822=CARTESIAN_POINT('Ctrl Pts',(-90.0112537562499,-34.0875058574723,
117.368546554116));
#44823=CARTESIAN_POINT('Ctrl Pts',(-87.0959334446163,-33.237480170709,117.210598030923));
#44824=CARTESIAN_POINT('Ctrl Pts',(-84.7904591740287,-35.2139478722533,
117.052649507731));
#44825=CARTESIAN_POINT('Ctrl Pts',(-85.1851343478002,-38.2249058086552,
116.894700984538));
#44826=CARTESIAN_POINT('Ctrl Pts',(-87.9221189893741,-39.5404099931289,
116.736752461346));
#44827=CARTESIAN_POINT('Ctrl Pts',(-90.5198723658608,-37.9677327908616,
116.578803938154));
#44828=CARTESIAN_POINT('Ctrl Pts',(-90.6230904978973,-34.9327727903349,
116.420855414961));
#44829=CARTESIAN_POINT('Ctrl Pts',(-88.1381886444035,-33.18723591989,116.262906891769));
#44830=CARTESIAN_POINT('Ctrl Pts',(-85.3181517410688,-34.3137473718554,
116.104958368576));
#44831=CARTESIAN_POINT('Ctrl Pts',(-84.7198214806012,-37.290933474031,115.947009845384));
#44832=CARTESIAN_POINT('Ctrl Pts',(-86.8856857127746,-39.4194701345965,
115.789061322191));
#44833=CARTESIAN_POINT('Ctrl Pts',(-89.8520212100601,-38.7694778999333,
115.631112798999));
#44834=CARTESIAN_POINT('Ctrl Pts',(-90.9293417940852,-35.9302849605903,
115.473164275806));
#44835=CARTESIAN_POINT('Ctrl Pts',(-89.1408736565385,-33.47610120452,115.315215752614));
#44836=CARTESIAN_POINT('Ctrl Pts',(-86.1081664639344,-33.6320604027263,
115.157267229421));
#44837=CARTESIAN_POINT('Ctrl Pts',(-84.5808835921868,-36.2567590934803,
114.999318706229));
#44838=CARTESIAN_POINT('Ctrl Pts',(-85.9437659709006,-38.9704628004774,
114.841370183036));
#44839=CARTESIAN_POINT('Ctrl Pts',(-88.9611295974899,-39.3127389061509,
114.683421659844));
#44840=CARTESIAN_POINT('Ctrl Pts',(-90.8972226406924,-36.9732560753437,
114.525473136651));
#44841=CARTESIAN_POINT('Ctrl Pts',(-89.9966484218447,-34.0731522385948,
114.367524613459));
#44842=CARTESIAN_POINT('Ctrl Pts',(-87.0759301954492,-33.2418633420133,
114.209576090267));
#44843=CARTESIAN_POINT('Ctrl Pts',(-84.7831943477492,-35.2330937456208,
114.051627567074));
#44844=CARTESIAN_POINT('Ctrl Pts',(-85.1971947414458,-38.2414554030014,
113.893679043882));
#44845=CARTESIAN_POINT('Ctrl Pts',(-87.9425698108267,-39.5393582945921,
113.735730520689));
#44846=CARTESIAN_POINT('Ctrl Pts',(-90.5301714772931,-37.9500333425197,
113.577781997497));
#44847=CARTESIAN_POINT('Ctrl Pts',(-90.6139000082066,-34.9144731436948,
113.419833474304));
#44848=CARTESIAN_POINT('Ctrl Pts',(-88.1178412910765,-33.1849278080018,
113.261884951112));
#44849=CARTESIAN_POINT('Ctrl Pts',(-85.3050958505301,-34.32952348957,113.103936427919));
#44850=CARTESIAN_POINT('Ctrl Pts',(-84.7258944317255,-37.3104900952256,
112.945987904727));
#44851=CARTESIAN_POINT('Ctrl Pts',(-86.9053813454777,-39.4250758656216,
112.788039381534));
#44852=CARTESIAN_POINT('Ctrl Pts',(-89.867482093186,-38.7560501949591,112.630090858342));
#44853=CARTESIAN_POINT('Ctrl Pts',(-90.9265500151248,-35.9099983113317,
112.472142335149));
#44854=CARTESIAN_POINT('Ctrl Pts',(-89.1223604365675,-33.4673488988693,
112.314193811957));
#44855=CARTESIAN_POINT('Ctrl Pts',(-86.0907171764458,-33.6427778900275,
112.156245288764));
#44856=CARTESIAN_POINT('Ctrl Pts',(-84.580318975451,-36.2772291539554,111.998296765572));
#44857=CARTESIAN_POINT('Ctrl Pts',(-85.960597945739,-38.9821258528616,111.840348242379));
#44858=CARTESIAN_POINT('Ctrl Pts',(-88.9800971242396,-39.3050204155649,
111.682399719187));
#44859=CARTESIAN_POINT('Ctrl Pts',(-90.901128439717,-36.9531541624509,111.524451195994));
#44860=CARTESIAN_POINT('Ctrl Pts',(-89.9819512239657,-34.0588926964507,
111.366502672802));
#44861=CARTESIAN_POINT('Ctrl Pts',(-87.0559555029728,-33.24637486378,111.208554149609));
#44862=CARTESIAN_POINT('Ctrl Pts',(-84.7760526068729,-35.2522858717561,
111.050605626417));
#44863=CARTESIAN_POINT('Ctrl Pts',(-85.2093611513503,-38.257927216375,110.892657103225));
#44864=CARTESIAN_POINT('Ctrl Pts',(-87.963013457811,-39.5381753031207,110.734708580032));
#44865=CARTESIAN_POINT('Ctrl Pts',(-90.5403567281249,-37.9322681283135,
110.57676005684));
#44866=CARTESIAN_POINT('Ctrl Pts',(-90.6045922062968,-34.8962328867416,
110.418811533647));
#44867=CARTESIAN_POINT('Ctrl Pts',(-88.0974795361613,-33.1827503933531,
110.260863010455));
#44868=CARTESIAN_POINT('Ctrl Pts',(-85.2921415289253,-34.3453831152826,
110.102914487262));
#44869=CARTESIAN_POINT('Ctrl Pts',(-84.7320928278883,-37.330007316042,109.94496596407));
#44870=CARTESIAN_POINT('Ctrl Pts',(-86.925112572311,-39.4305550212435,109.787017440877));
#44871=CARTESIAN_POINT('Ctrl Pts',(-89.8828564264658,-38.7425234805934,
109.629068917685));
#44872=CARTESIAN_POINT('Ctrl Pts',(-90.923628057546,-35.8897300307512,109.471120394492));
#44873=CARTESIAN_POINT('Ctrl Pts',(-89.1037913495795,-33.4587155966883,
109.3131718713));
#44874=CARTESIAN_POINT('Ctrl Pts',(-86.0733371687237,-33.6536073017113,
109.155223348107));
#44875=CARTESIAN_POINT('Ctrl Pts',(-84.5798855965776,-36.29770220504,108.997274824915));
#44876=CARTESIAN_POINT('Ctrl Pts',(-85.9775048980366,-38.9936810243913,
108.839326301722));
#44877=CARTESIAN_POINT('Ctrl Pts',(-88.9990138028663,-39.2971793935384,
108.68137777853));
#44878=CARTESIAN_POINT('Ctrl Pts',(-90.9049069280247,-36.9330294359731,
108.523429255337));
#44879=CARTESIAN_POINT('Ctrl Pts',(-89.9671589758732,-34.0447240118636,
108.365480732145));
#44880=CARTESIAN_POINT('Ctrl Pts',(-87.036017990837,-33.2510223796941,108.207532208953));
#44881=CARTESIAN_POINT('Ctrl Pts',(-84.769018204098,-35.2715073567614,108.04958368576));
#44882=CARTESIAN_POINT('Ctrl Pts',(-85.2216660675069,-38.274353686417,107.891635162568));
#44883=CARTESIAN_POINT('Ctrl Pts',(-87.9833812366168,-39.5367929590649,
107.733686639375));
#44884=CARTESIAN_POINT('Ctrl Pts',(-90.5505672416893,-37.9145779521832,
107.575738116183));
#44885=CARTESIAN_POINT('Ctrl Pts',(-90.5948804903041,-34.8777646456526,
107.41778959299));
#44886=CARTESIAN_POINT('Ctrl Pts',(-88.0776946243907,-33.181296120173,107.259841069798));
#44887=CARTESIAN_POINT('Ctrl Pts',(-85.2780750173411,-34.3600925800612,
107.101892546605));
#44888=CARTESIAN_POINT('Ctrl Pts',(-84.7409661127983,-37.3519728362644,
106.943944023413));
#44889=CARTESIAN_POINT('Ctrl Pts',(-86.2067093668298,-38.7351332702527,
106.838645007951));
#44890=CARTESIAN_POINT('Ctrl Pts',(-87.0704891624118,-38.9660582606223,
106.78599550022));
#44891=CARTESIAN_POINT('Ctrl Pts',(-85.573358484553,-34.478062635605,122.21400449978));
#44892=CARTESIAN_POINT('Ctrl Pts',(-84.9524796464486,-35.2042483553411,
122.161354992049));
#44893=CARTESIAN_POINT('Ctrl Pts',(-84.4989332336292,-37.3094627529595,
122.056055976587));
#44894=CARTESIAN_POINT('Ctrl Pts',(-86.782849542669,-39.6190417482899,121.898107453395));
#44895=CARTESIAN_POINT('Ctrl Pts',(-89.9617291027293,-38.9625419388902,
121.740158930202));
#44896=CARTESIAN_POINT('Ctrl Pts',(-91.1515471831214,-35.9450053846625,
121.58221040701));
#44897=CARTESIAN_POINT('Ctrl Pts',(-89.274394783863,-33.2975773244359,121.424261883817));
#44898=CARTESIAN_POINT('Ctrl Pts',(-86.0318052779183,-33.4229100750779,
121.266313360625));
#44899=CARTESIAN_POINT('Ctrl Pts',(-84.3639418200909,-36.2062451402475,
121.108364837432));
#44900=CARTESIAN_POINT('Ctrl Pts',(-85.7829053659071,-39.1245633397293,
120.95041631424));
#44901=CARTESIAN_POINT('Ctrl Pts',(-89.0022135038696,-39.5316487980236,
120.792467791047));
#44902=CARTESIAN_POINT('Ctrl Pts',(-91.1029937861889,-37.0585386170348,
120.634519267855));
#44903=CARTESIAN_POINT('Ctrl Pts',(-90.1805441324336,-33.9474638054562,
120.476570744663));
#44904=CARTESIAN_POINT('Ctrl Pts',(-87.0712159924203,-33.0191718000006,
120.31862222147));
#44905=CARTESIAN_POINT('Ctrl Pts',(-84.594145345843,-35.115301887322,120.160673698277));
#44906=CARTESIAN_POINT('Ctrl Pts',(-84.9952154881615,-38.3353638848805,
120.002725175085));
#44907=CARTESIAN_POINT('Ctrl Pts',(-87.9107889626707,-39.7598220042095,
119.844776651893));
#44908=CARTESIAN_POINT('Ctrl Pts',(-90.6974036603767,-38.0971650976748,
119.6868281287));
#44909=CARTESIAN_POINT('Ctrl Pts',(-90.8285209380269,-34.8548727853765,
119.528879605508));
#44910=CARTESIAN_POINT('Ctrl Pts',(-88.1852606737698,-32.9726333004099,
119.370931082315));
#44911=CARTESIAN_POINT('Ctrl Pts',(-85.1641865940414,-34.157015741921,119.212982559123));
#44912=CARTESIAN_POINT('Ctrl Pts',(-84.504414667631,-37.3341766669294,119.05503403593));
#44913=CARTESIAN_POINT('Ctrl Pts',(-86.8041400426611,-39.623480847337,118.897085512738));
#44914=CARTESIAN_POINT('Ctrl Pts',(-89.9782716604433,-38.9492858313566,
118.739136989545));
#44915=CARTESIAN_POINT('Ctrl Pts',(-91.1489209219942,-35.9228637242989,
118.581188466353));
#44916=CARTESIAN_POINT('Ctrl Pts',(-89.2546957445757,-33.2881794114966,
118.42323994316));
#44917=CARTESIAN_POINT('Ctrl Pts',(-86.0130324867741,-33.4340210264743,
118.265291419968));
#44918=CARTESIAN_POINT('Ctrl Pts',(-84.3630486334757,-36.2281584137643,
118.107342896775));
#44919=CARTESIAN_POINT('Ctrl Pts',(-85.8007343625879,-39.1372321835451,
117.949394373583));
#44920=CARTESIAN_POINT('Ctrl Pts',(-89.022583748705,-39.5236736245337,117.791445850391));
#44921=CARTESIAN_POINT('Ctrl Pts',(-91.107443941581,-37.0371080351261,117.633497327198));
#44922=CARTESIAN_POINT('Ctrl Pts',(-90.1650356124785,-33.9320288098347,
117.475548804006));
#44923=CARTESIAN_POINT('Ctrl Pts',(-87.0498117313475,-33.0237168454812,
117.317600280813));
#44924=CARTESIAN_POINT('Ctrl Pts',(-84.586251045955,-35.135710975102,117.159651757621));
#44925=CARTESIAN_POINT('Ctrl Pts',(-85.0079891039364,-38.3531303547597,
117.001703234428));
#44926=CARTESIAN_POINT('Ctrl Pts',(-87.9326488347025,-39.7588386863096,
116.843754711236));
#44927=CARTESIAN_POINT('Ctrl Pts',(-90.708530209873,-38.0783229782199,116.685806188043));
#44928=CARTESIAN_POINT('Ctrl Pts',(-90.8188260111962,-34.8352557124416,
116.527857664851));
#44929=CARTESIAN_POINT('Ctrl Pts',(-88.1635343901077,-32.970027345423,116.369909141658));
#44930=CARTESIAN_POINT('Ctrl Pts',(-85.1501275024042,-34.1737837091839,
116.211960618466));
#44931=CARTESIAN_POINT('Ctrl Pts',(-84.5107697245388,-37.3551155192967,
116.054012095273));
#44932=CARTESIAN_POINT('Ctrl Pts',(-86.8251473085145,-39.6296059793658,
115.896063572081));
#44933=CARTESIAN_POINT('Ctrl Pts',(-89.9948844875526,-38.9350437647466,
115.738115048888));
#44934=CARTESIAN_POINT('Ctrl Pts',(-91.146076964618,-35.9011673112796,115.580166525696));
#44935=CARTESIAN_POINT('Ctrl Pts',(-89.2349735326918,-33.278700128142,115.422218002504));
#44936=CARTESIAN_POINT('Ctrl Pts',(-85.9943135499183,-33.4453534515506,
115.264269479311));
#44937=CARTESIAN_POINT('Ctrl Pts',(-84.3623048624599,-36.2500277817027,
115.106320956119));
#44938=CARTESIAN_POINT('Ctrl Pts',(-85.8186401119347,-39.1498102037631,
114.948372432926));
#44939=CARTESIAN_POINT('Ctrl Pts',(-89.0429044200783,-39.5155561885454,
114.790423909734));
#44940=CARTESIAN_POINT('Ctrl Pts',(-91.1117554002631,-37.0156549753088,
114.632475386541));
#44941=CARTESIAN_POINT('Ctrl Pts',(-90.1494287900138,-33.9166909630364,
114.474526863349));
#44942=CARTESIAN_POINT('Ctrl Pts',(-87.0284368590026,-33.0284005709257,
114.316578340156));
#44943=CARTESIAN_POINT('Ctrl Pts',(-84.5784880703985,-35.1561696813723,
114.158629816964));
#44944=CARTESIAN_POINT('Ctrl Pts',(-85.0208764790048,-38.3708147551066,
114.000681293771));
#44945=CARTESIAN_POINT('Ctrl Pts',(-87.9545019693732,-39.757714872784,113.842732770579));
#44946=CARTESIAN_POINT('Ctrl Pts',(-90.7195355315731,-38.0594098783669,
113.684784247386));
#44947=CARTESIAN_POINT('Ctrl Pts',(-90.8090053294518,-34.8157012586816,
113.526835724194));
#44948=CARTESIAN_POINT('Ctrl Pts',(-88.1417918183741,-32.9675609662586,
113.368887201001));
#44949=CARTESIAN_POINT('Ctrl Pts',(-85.1361763692016,-34.1906415955917,
113.210938677809));
#44950=CARTESIAN_POINT('Ctrl Pts',(-84.5172590980378,-37.3760131383805,
113.052990154616));
#44951=CARTESIAN_POINT('Ctrl Pts',(-86.8461934711285,-39.6355960954744,
112.895041631424));
#44952=CARTESIAN_POINT('Ctrl Pts',(-90.0114055237299,-38.9206953217857,
112.737093108232));
#44953=CARTESIAN_POINT('Ctrl Pts',(-91.143093753321,-35.8794896060935,112.579144585039));
#44954=CARTESIAN_POINT('Ctrl Pts',(-89.2151908608736,-33.2693476767256,
112.421196061847));
#44955=CARTESIAN_POINT('Ctrl Pts',(-85.9756677644532,-33.4568058371609,
112.263247538654));
#44956=CARTESIAN_POINT('Ctrl Pts',(-84.3617015299438,-36.2719014746159,
112.105299015462));
#44957=CARTESIAN_POINT('Ctrl Pts',(-85.8366262556094,-39.1622729918721,
111.947350492269));
#44958=CARTESIAN_POINT('Ctrl Pts',(-89.0631725504999,-39.5073084409124,
111.789401969077));
#44959=CARTESIAN_POINT('Ctrl Pts',(-91.1159290200014,-36.9941746738646,
111.631453445884));
#44960=CARTESIAN_POINT('Ctrl Pts',(-90.1337238049953,-33.9014536438148,
111.473504922692));
#44961=CARTESIAN_POINT('Ctrl Pts',(-87.0070925014814,-33.0332214478261,
111.315556399499));
#44962=CARTESIAN_POINT('Ctrl Pts',(-84.5708566202139,-35.1766778119636,
111.157607876307));
#44963=CARTESIAN_POINT('Ctrl Pts',(-85.033877139869,-38.388416041038,110.999659353114));
#44964=CARTESIAN_POINT('Ctrl Pts',(-87.976347437622,-39.7564507635648,110.841710829922));
#44965=CARTESIAN_POINT('Ctrl Pts',(-90.7304191852489,-38.040426503083,110.683762306729));
#44966=CARTESIAN_POINT('Ctrl Pts',(-90.7990592913871,-34.7962102669604,
110.525813783537));
#44967=CARTESIAN_POINT('Ctrl Pts',(-88.1200338575352,-32.9652342462458,
110.367865260344));
#44968=CARTESIAN_POINT('Ctrl Pts',(-85.1223337695167,-34.2075887161425,
110.209916737152));
#44969=CARTESIAN_POINT('Ctrl Pts',(-84.5238825183441,-37.3968686554014,
110.051968213959));
#44970=CARTESIAN_POINT('Ctrl Pts',(-86.8672776685629,-39.641450956902,109.894019690767));
#44971=CARTESIAN_POINT('Ctrl Pts',(-90.0278340753366,-38.9062410803574,
109.736071167575));
#44972=CARTESIAN_POINT('Ctrl Pts',(-91.1399714370551,-35.8578315291262,
109.578122644382));
#44973=CARTESIAN_POINT('Ctrl Pts',(-89.1953484912358,-33.2601223888489,
109.42017412119));
#44974=CARTESIAN_POINT('Ctrl Pts',(-85.9570960092694,-33.4683778218109,
109.262225597997));
#44975=CARTESIAN_POINT('Ctrl Pts',(-84.3612384342726,-36.2937783632046,
109.104277074805));
#44976=CARTESIAN_POINT('Ctrl Pts',(-85.8546925179493,-39.1746205017346,
108.946328551612));
#44977=CARTESIAN_POINT('Ctrl Pts',(-89.0833863461416,-39.4989297598556,
108.78838002842));
#44978=CARTESIAN_POINT('Ctrl Pts',(-91.1199665993245,-36.9726699945077,
108.630431505227));
#44979=CARTESIAN_POINT('Ctrl Pts',(-90.1179172521685,-33.8863134122548,
108.472482982035));
#44980=CARTESIAN_POINT('Ctrl Pts',(-86.9857878737573,-33.0381876439953,
108.314534458842));
#44981=CARTESIAN_POINT('Ctrl Pts',(-84.5633398683062,-35.1972173145631,
108.15658593565));
#44982=CARTESIAN_POINT('Ctrl Pts',(-85.0470258043618,-38.4059688744449,
107.998637412457));
#44983=CARTESIAN_POINT('Ctrl Pts',(-87.9981118354098,-39.7549736321506,
107.840688889265));
#44984=CARTESIAN_POINT('Ctrl Pts',(-90.7413298339237,-38.0215233112373,
107.682740366072));
#44985=CARTESIAN_POINT('Ctrl Pts',(-90.7886816428431,-34.7764756582269,
107.52479184288));
#44986=CARTESIAN_POINT('Ctrl Pts',(-88.0988922939863,-32.963680253526,107.366843319688));
#44987=CARTESIAN_POINT('Ctrl Pts',(-85.1073027169643,-34.2233068092021,
107.208894796495));
#44988=CARTESIAN_POINT('Ctrl Pts',(-84.5333642445699,-37.4203403517654,
107.050946273303));
#44989=CARTESIAN_POINT('Ctrl Pts',(-86.099613541549,-38.8983441231523,106.945647257841));
#44990=CARTESIAN_POINT('Ctrl Pts',(-87.0226227342259,-39.1451036445258,
106.89299775011));
#44991=CARTESIAN_POINT('Ctrl Pts',(-85.4324929308759,-34.3576245177531,
122.321006749669));
#44992=CARTESIAN_POINT('Ctrl Pts',(-84.7717723668801,-35.1304094942464,
122.268357241939));
#44993=CARTESIAN_POINT('Ctrl Pts',(-84.2891219312635,-37.3707152652939,
122.163058226477));
#44994=CARTESIAN_POINT('Ctrl Pts',(-86.7195968954854,-39.8284996875276,
122.005109703284));
#44995=CARTESIAN_POINT('Ctrl Pts',(-90.1024648028703,-39.1298723584757,
121.847161180092));
#44996=CARTESIAN_POINT('Ctrl Pts',(-91.3686333769664,-35.9187008196384,
121.6892126569));
#44997=CARTESIAN_POINT('Ctrl Pts',(-89.3710243173134,-33.1013875956417,
121.531264133707));
#44998=CARTESIAN_POINT('Ctrl Pts',(-85.9203582039126,-33.2347629349336,
121.373315610515));
#44999=CARTESIAN_POINT('Ctrl Pts',(-84.1454681337529,-36.1967043012439,
121.215367087322));
#45000=CARTESIAN_POINT('Ctrl Pts',(-85.6554864122685,-39.3022906545617,
121.05741856413));
#45001=CARTESIAN_POINT('Ctrl Pts',(-89.0813771948967,-39.735498741376,120.899470040937));
#45002=CARTESIAN_POINT('Ctrl Pts',(-91.3169643139602,-37.1036893555134,
120.741521517745));
#45003=CARTESIAN_POINT('Ctrl Pts',(-90.3353211686605,-33.7929772197686,
120.583572994552));
#45004=CARTESIAN_POINT('Ctrl Pts',(-87.0264677882008,-32.8051168197105,
120.42562447136));
#45005=CARTESIAN_POINT('Ctrl Pts',(-84.3904437941137,-35.0357553412809,
120.267675948167));
#45006=CARTESIAN_POINT('Ctrl Pts',(-84.8172505627962,-38.4624483585915,
120.109727424975));
#45007=CARTESIAN_POINT('Ctrl Pts',(-87.9199160624454,-39.9783137967903,
119.951778901782));
#45008=CARTESIAN_POINT('Ctrl Pts',(-90.8853475149469,-38.20896438174,119.79383037859));
#45009=CARTESIAN_POINT('Ctrl Pts',(-91.0248785737008,-34.7586145328686,
119.635881855397));
#45010=CARTESIAN_POINT('Ctrl Pts',(-88.2120005926768,-32.7555919497842,
119.477933332205));
#45011=CARTESIAN_POINT('Ctrl Pts',(-84.9970645257212,-34.0159760806577,
119.319984809012));
#45012=CARTESIAN_POINT('Ctrl Pts',(-84.2949551082748,-37.3970150683708,
119.16203628582));
#45013=CARTESIAN_POINT('Ctrl Pts',(-86.7422536044908,-39.8332236430662,
119.004087762628));
#45014=CARTESIAN_POINT('Ctrl Pts',(-90.1200688946704,-39.1157656079981,
118.846139239435));
#45015=CARTESIAN_POINT('Ctrl Pts',(-91.3658385889551,-35.8951383313953,
118.688190716243));
#45016=CARTESIAN_POINT('Ctrl Pts',(-89.350061192869,-33.0913866196758,118.53024219305));
#45017=CARTESIAN_POINT('Ctrl Pts',(-85.9003807648513,-33.2465868748436,
118.372293669858));
#45018=CARTESIAN_POINT('Ctrl Pts',(-84.1445176314521,-36.2200237470817,
118.214345146665));
#45019=CARTESIAN_POINT('Ctrl Pts',(-85.6744594936806,-39.3157724566742,
118.056396623473));
#45020=CARTESIAN_POINT('Ctrl Pts',(-89.1030545960746,-39.7270118018916,
117.89844810028));
#45021=CARTESIAN_POINT('Ctrl Pts',(-91.3217000353283,-37.0808835755504,
117.740499577088));
#45022=CARTESIAN_POINT('Ctrl Pts',(-90.3188174687069,-33.7765517621971,
117.582551053895));
#45023=CARTESIAN_POINT('Ctrl Pts',(-87.0036900180789,-32.8099535202534,
117.424602530703));
#45024=CARTESIAN_POINT('Ctrl Pts',(-84.382042917881,-35.0574740779507,117.26665400751));
#45025=CARTESIAN_POINT('Ctrl Pts',(-84.8308438600728,-38.4813549008641,
117.108705484318));
#45026=CARTESIAN_POINT('Ctrl Pts',(-87.9431786800308,-39.9772673794902,
116.950756961126));
#45027=CARTESIAN_POINT('Ctrl Pts',(-90.8971880538853,-38.1889131655783,
116.792808437933));
#45028=CARTESIAN_POINT('Ctrl Pts',(-91.0145615244951,-34.7377386345482,
116.634859914741));
#45029=CARTESIAN_POINT('Ctrl Pts',(-88.1888801358119,-32.7528187709561,
116.476911391548));
#45030=CARTESIAN_POINT('Ctrl Pts',(-84.9821032637396,-34.0338200465123,
116.318962868356));
#45031=CARTESIAN_POINT('Ctrl Pts',(-84.3017179684765,-37.4192975645625,
116.161014345163));
#45032=CARTESIAN_POINT('Ctrl Pts',(-86.7646089042542,-39.839741824135,116.003065821971));
#45033=CARTESIAN_POINT('Ctrl Pts',(-90.1377477650451,-39.10060962956,115.845117298778));
#45034=CARTESIAN_POINT('Ctrl Pts',(-91.3628121351507,-35.8720496619689,
115.687168775586));
#45035=CARTESIAN_POINT('Ctrl Pts',(-89.3290734088453,-33.081299051764,115.529220252393));
#45036=CARTESIAN_POINT('Ctrl Pts',(-85.8804606359022,-33.2586465003749,
115.371271729201));
#45037=CARTESIAN_POINT('Ctrl Pts',(-84.1437261327331,-36.243296469925,115.213323206008));
#45038=CARTESIAN_POINT('Ctrl Pts',(-85.6935142529687,-39.3291576070487,
115.055374682816));
#45039=CARTESIAN_POINT('Ctrl Pts',(-89.1246792426668,-39.7183734709399,
114.897426159623));
#45040=CARTESIAN_POINT('Ctrl Pts',(-91.3262881598338,-37.0580538752739,
114.739477636431));
#45041=CARTESIAN_POINT('Ctrl Pts',(-90.3022091581829,-33.760229687478,114.581529113238));
#45042=CARTESIAN_POINT('Ctrl Pts',(-86.9809435225561,-32.814937799838,114.423580590046));
#45043=CARTESIAN_POINT('Ctrl Pts',(-84.3737817930479,-35.0792456171238,
114.265632066854));
#45044=CARTESIAN_POINT('Ctrl Pts',(-84.8445582165638,-38.5001741072118,
114.107683543661));
#45045=CARTESIAN_POINT('Ctrl Pts',(-87.9664341279196,-39.9760714509759,
113.949735020469));
#45046=CARTESIAN_POINT('Ctrl Pts',(-90.9088995858529,-38.1687864142141,
113.791786497276));
#45047=CARTESIAN_POINT('Ctrl Pts',(-91.0041106506971,-34.7169293736683,
113.633837974084));
#45048=CARTESIAN_POINT('Ctrl Pts',(-88.1657423456717,-32.7501941245154,
113.475889450891));
#45049=CARTESIAN_POINT('Ctrl Pts',(-84.9672568878733,-34.0517597016134,
113.317940927699));
#45050=CARTESIAN_POINT('Ctrl Pts',(-84.3086237643501,-37.4415361815354,
113.159992404506));
#45051=CARTESIAN_POINT('Ctrl Pts',(-86.7870055967793,-39.8461163253272,
113.002043881314));
#45052=CARTESIAN_POINT('Ctrl Pts',(-90.1553289542737,-39.0853404486122,
112.844095358121));
#45053=CARTESIAN_POINT('Ctrl Pts',(-91.3596374915171,-35.8489809008554,
112.686146834929));
#45054=CARTESIAN_POINT('Ctrl Pts',(-89.3080212851796,-33.0713464545818,
112.528198311736));
#45055=CARTESIAN_POINT('Ctrl Pts',(-85.8606183524605,-33.2708337842943,
112.370249788544));
#45056=CARTESIAN_POINT('Ctrl Pts',(-84.1430840844366,-36.2665737952763,
112.212301265351));
#45057=CARTESIAN_POINT('Ctrl Pts',(-85.7126545654799,-39.3424201308827,
112.054352742159));
#45058=CARTESIAN_POINT('Ctrl Pts',(-89.1462479767601,-39.7095964662598,
111.896404218967));
#45059=CARTESIAN_POINT('Ctrl Pts',(-91.3307296002859,-37.0351951852785,
111.738455695774));
#45060=CARTESIAN_POINT('Ctrl Pts',(-90.285496386025,-33.744014591179,111.580507172582));
#45061=CARTESIAN_POINT('Ctrl Pts',(-86.9582294999899,-32.8200680318722,
111.422558649389));
#45062=CARTESIAN_POINT('Ctrl Pts',(-84.3656606335548,-35.1010697521711,
111.264610126197));
#45063=CARTESIAN_POINT('Ctrl Pts',(-84.8583931283879,-38.5189048657011,
111.106661603004));
#45064=CARTESIAN_POINT('Ctrl Pts',(-87.9896814174328,-39.974726224009,110.948713079812));
#45065=CARTESIAN_POINT('Ctrl Pts',(-90.9204816423732,-38.1485848778524,
110.790764556619));
#45066=CARTESIAN_POINT('Ctrl Pts',(-90.9935263764774,-34.6961876471792,
110.632816033427));
#45067=CARTESIAN_POINT('Ctrl Pts',(-88.142588178909,-32.7477180991385,110.474867510234));
#45068=CARTESIAN_POINT('Ctrl Pts',(-84.9525260101083,-34.0697943170025,
110.316918987042));
#45069=CARTESIAN_POINT('Ctrl Pts',(-84.3156722087998,-37.4637299947607,
110.158970463849));
#45070=CARTESIAN_POINT('Ctrl Pts',(-86.8094427648148,-39.8523468925606,
110.001021940657));
#45071=CARTESIAN_POINT('Ctrl Pts',(-90.1728117242074,-39.0699586801214,
109.843073417464));
#45072=CARTESIAN_POINT('Ctrl Pts',(-91.3563148165642,-35.8259330275012,
109.685124894272));
#45073=CARTESIAN_POINT('Ctrl Pts',(-89.2869056328921,-33.0615291810096,
109.52717637108));
#45074=CARTESIAN_POINT('Ctrl Pts',(-85.840854849815,-33.2831483419104,109.369227847887));
#45075=CARTESIAN_POINT('Ctrl Pts',(-84.1425912719677,-36.2898545213693,
109.211279324695));
#45076=CARTESIAN_POINT('Ctrl Pts',(-85.731880137862,-39.3555599790778,109.053330801502));
#45077=CARTESIAN_POINT('Ctrl Pts',(-89.1677588894168,-39.7006801261729,
108.89538227831));
#45078=CARTESIAN_POINT('Ctrl Pts',(-91.3350262706245,-37.0123105530422,
108.737433755117));
#45079=CARTESIAN_POINT('Ctrl Pts',(-90.2686755284635,-33.727902812646,108.579485231925));
#45080=CARTESIAN_POINT('Ctrl Pts',(-86.9355577566776,-32.8253529082965,
108.421536708732));
#45081=CARTESIAN_POINT('Ctrl Pts',(-84.3576615325144,-35.1229272723648,
108.26358818554));
#45082=CARTESIAN_POINT('Ctrl Pts',(-84.8723855412168,-38.5375840624727,
108.105639662347));
#45083=CARTESIAN_POINT('Ctrl Pts',(-88.0128424342027,-39.9731543052364,
107.947691139155));
#45084=CARTESIAN_POINT('Ctrl Pts',(-90.9320924261582,-38.1284686702913,
107.789742615962));
#45085=CARTESIAN_POINT('Ctrl Pts',(-90.9824827953822,-34.6751866708012,
107.63179409277));
#45086=CARTESIAN_POINT('Ctrl Pts',(-88.1200899635817,-32.7460643868788,
107.473845569577));
#45087=CARTESIAN_POINT('Ctrl Pts',(-84.9365304165877,-34.0865210383432,
107.315897046385));
#45088=CARTESIAN_POINT('Ctrl Pts',(-84.3257623763415,-37.4887078672662,
107.157948523192));
#45089=CARTESIAN_POINT('Ctrl Pts',(-85.9925177162683,-39.0615549760519,
107.052649507731));
#45090=CARTESIAN_POINT('Ctrl Pts',(-86.97475630604,-39.3241490284294,107.));
#45091=CARTESIAN_POINT('Ctrl Pts',(-85.855089591907,-34.7189388713087,122.));
#45092=CARTESIAN_POINT('Ctrl Pts',(-85.7934813914369,-34.7768354517112,
122.));
#45093=CARTESIAN_POINT('Ctrl Pts',(-85.735242344367,-34.8378827916466,122.));
#45094=CARTESIAN_POINT('Ctrl Pts',(-85.6803700642034,-34.9016960722485,
122.));
#45095=CARTESIAN_POINT('Ctrl Pts',(-85.6240448547982,-34.9671990253247,
122.));
#45096=CARTESIAN_POINT('Ctrl Pts',(-85.5712666289892,-35.0356167652744,
122.));
#45097=CARTESIAN_POINT('Ctrl Pts',(-85.5220583134545,-35.1065816394062,
122.));
#45098=CARTESIAN_POINT('Ctrl Pts',(-85.4715004197893,-35.1794927830071,
122.));
#45099=CARTESIAN_POINT('Ctrl Pts',(-85.4247104044215,-35.2550932475831,
122.));
#45100=CARTESIAN_POINT('Ctrl Pts',(-85.3817472004119,-35.3330272726362,
122.));
#45101=CARTESIAN_POINT('Ctrl Pts',(-85.3628372305493,-35.3673294179019,
122.));
#45102=CARTESIAN_POINT('Ctrl Pts',(-85.3446690988358,-35.402084133033,122.));
#45103=CARTESIAN_POINT('Ctrl Pts',(-85.3272502554093,-35.4372631605433,
122.));
#45104=CARTESIAN_POINT('Ctrl Pts',(-85.3173194106968,-35.4573194553726,
122.));
#45105=CARTESIAN_POINT('Ctrl Pts',(-85.3076321412892,-35.4775136884896,
122.));
#45106=CARTESIAN_POINT('Ctrl Pts',(-85.2981900621096,-35.497840771842,122.));
#45107=CARTESIAN_POINT('Ctrl Pts',(-85.2896844749579,-35.5161517577706,
122.));
#45108=CARTESIAN_POINT('Ctrl Pts',(-85.281375478207,-35.5345762757094,122.));
#45109=CARTESIAN_POINT('Ctrl Pts',(-85.2732779128575,-35.5530788516544,
122.));
#45110=CARTESIAN_POINT('Ctrl Pts',(-85.2367162849915,-35.636620541911,122.));
#45111=CARTESIAN_POINT('Ctrl Pts',(-85.2044148369174,-35.7218457754668,
122.));
#45112=CARTESIAN_POINT('Ctrl Pts',(-85.1763986040086,-35.8083557745312,
122.));
#45113=CARTESIAN_POINT('Ctrl Pts',(-85.147919276174,-35.8962957424901,122.));
#45114=CARTESIAN_POINT('Ctrl Pts',(-85.1238675061027,-35.9855640551364,
122.));
#45115=CARTESIAN_POINT('Ctrl Pts',(-85.1043086662742,-36.0757789555843,
122.));
#45116=CARTESIAN_POINT('Ctrl Pts',(-85.0853401900751,-36.1632708112854,
122.));
#45117=CARTESIAN_POINT('Ctrl Pts',(-85.0705973519178,-36.2516538909537,
122.));
#45118=CARTESIAN_POINT('Ctrl Pts',(-85.0601805241994,-36.3406018388456,
122.));
#45119=CARTESIAN_POINT('Ctrl Pts',(-85.0558116903908,-36.3779067470632,
122.));
#45120=CARTESIAN_POINT('Ctrl Pts',(-85.0522043074793,-36.4153112064065,
122.));
#45121=CARTESIAN_POINT('Ctrl Pts',(-85.0493681149686,-36.4527917592161,
122.));
#45122=CARTESIAN_POINT('Ctrl Pts',(-85.0475889875222,-36.4763030970235,
122.));
#45123=CARTESIAN_POINT('Ctrl Pts',(-85.0461133503525,-36.4998443829401,
122.));
#45124=CARTESIAN_POINT('Ctrl Pts',(-85.0449439035519,-36.5234098595724,
122.));
#45125=CARTESIAN_POINT('Ctrl Pts',(-85.0442595199509,-36.5372008466837,
122.));
#45126=CARTESIAN_POINT('Ctrl Pts',(-85.0436802910536,-36.5509951721818,
122.));
#45127=CARTESIAN_POINT('Ctrl Pts',(-85.0432067176554,-36.5647838451762,
122.));
#45128=CARTESIAN_POINT('Ctrl Pts',(-85.0398793341044,-36.6616647170585,
122.));
#45129=CARTESIAN_POINT('Ctrl Pts',(-85.0417578653667,-36.7583805840727,
122.));
#45130=CARTESIAN_POINT('Ctrl Pts',(-85.0489066930308,-36.8545116797471,
122.));
#45131=CARTESIAN_POINT('Ctrl Pts',(-85.0560555206949,-36.9506427754215,
122.));
#45132=CARTESIAN_POINT('Ctrl Pts',(-85.0684742144477,-37.0461901437907,
122.));
#45133=CARTESIAN_POINT('Ctrl Pts',(-85.0862796188093,-37.1407528038591,
122.));
#45134=CARTESIAN_POINT('Ctrl Pts',(-85.1033376429253,-37.2313462047815,
122.));
#45135=CARTESIAN_POINT('Ctrl Pts',(-85.1253395228826,-37.3210367972729,
122.));
#45136=CARTESIAN_POINT('Ctrl Pts',(-85.1520106494849,-37.4095852418723,
122.));
#45137=CARTESIAN_POINT('Ctrl Pts',(-85.1608799953067,-37.4390315711875,
122.));
#45138=CARTESIAN_POINT('Ctrl Pts',(-85.1702661253978,-37.4683515588674,
122.));
#45139=CARTESIAN_POINT('Ctrl Pts',(-85.1801601896715,-37.4975362287825,
122.));
#45140=CARTESIAN_POINT('Ctrl Pts',(-85.1894804986475,-37.5250284840829,
122.));
#45141=CARTESIAN_POINT('Ctrl Pts',(-85.1992515460373,-37.5524006617149,
122.));
#45142=CARTESIAN_POINT('Ctrl Pts',(-85.2094664085399,-37.5796451334156,
122.));
#45143=CARTESIAN_POINT('Ctrl Pts',(-85.2146241863597,-37.593401650629,122.));
#45144=CARTESIAN_POINT('Ctrl Pts',(-85.2198920425091,-37.607117334446,122.));
#45145=CARTESIAN_POINT('Ctrl Pts',(-85.2252673071018,-37.6207878666389,
122.));
#45146=CARTESIAN_POINT('Ctrl Pts',(-85.2595186282914,-37.7078968416282,
122.));
#45147=CARTESIAN_POINT('Ctrl Pts',(-85.2981434489407,-37.793217001783,122.));
#45148=CARTESIAN_POINT('Ctrl Pts',(-85.3408117833009,-37.8765139323352,
122.));
#45149=CARTESIAN_POINT('Ctrl Pts',(-85.3850415874262,-37.9628591571441,
122.));
#45150=CARTESIAN_POINT('Ctrl Pts',(-85.4336163991975,-38.047031091085,122.));
#45151=CARTESIAN_POINT('Ctrl Pts',(-85.4862245077739,-38.1287651551131,
122.));
#45152=CARTESIAN_POINT('Ctrl Pts',(-85.5393955693074,-38.2113738453971,
122.));
#45153=CARTESIAN_POINT('Ctrl Pts',(-85.5966871241838,-38.2914930335655,
122.));
#45154=CARTESIAN_POINT('Ctrl Pts',(-85.6578288553816,-38.3688341911083,
122.));
#45155=CARTESIAN_POINT('Ctrl Pts',(-85.6805177136348,-38.3975344343995,
122.));
#45156=CARTESIAN_POINT('Ctrl Pts',(-85.7037372340462,-38.4258519148351,
122.));
#45157=CARTESIAN_POINT('Ctrl Pts',(-85.727475197759,-38.4537710002837,122.));
#45158=CARTESIAN_POINT('Ctrl Pts',(-85.7482304515194,-38.4781820117021,
122.));
#45159=CARTESIAN_POINT('Ctrl Pts',(-85.7693820616618,-38.5022884505914,
122.));
#45160=CARTESIAN_POINT('Ctrl Pts',(-85.790922350481,-38.5260794851929,122.));
#45161=CARTESIAN_POINT('Ctrl Pts',(-85.8026858188802,-38.5390721189532,
122.));
#45162=CARTESIAN_POINT('Ctrl Pts',(-85.8145605316052,-38.5519654355969,
122.));
#45163=CARTESIAN_POINT('Ctrl Pts',(-85.8265391633365,-38.5647518126357,
122.));
#45164=CARTESIAN_POINT('Ctrl Pts',(-85.8955499468916,-38.6384161440946,
122.));
#45165=CARTESIAN_POINT('Ctrl Pts',(-85.9680631281327,-38.7085959444771,
122.));
#45166=CARTESIAN_POINT('Ctrl Pts',(-86.0437701857546,-38.7749999993731,
122.));
#45167=CARTESIAN_POINT('Ctrl Pts',(-86.1059643211302,-38.8295516212355,
122.));
#45168=CARTESIAN_POINT('Ctrl Pts',(-86.1703150292066,-38.8815550093779,
122.));
#45169=CARTESIAN_POINT('Ctrl Pts',(-86.2366735424928,-38.9308353738164,
122.));
#45170=CARTESIAN_POINT('Ctrl Pts',(-86.26129111213,-38.9491173205212,122.));
#45171=CARTESIAN_POINT('Ctrl Pts',(-86.286185186655,-38.9670243657543,122.));
#45172=CARTESIAN_POINT('Ctrl Pts',(-86.3113487775637,-38.9845470206273,
122.));
#45173=CARTESIAN_POINT('Ctrl Pts',(-86.3281596610916,-38.9962532715847,
122.));
#45174=CARTESIAN_POINT('Ctrl Pts',(-86.3450919689086,-39.0077885956498,
122.));
#45175=CARTESIAN_POINT('Ctrl Pts',(-86.3621285565829,-39.0191403402542,
122.));
#45176=CARTESIAN_POINT('Ctrl Pts',(-86.447039035685,-39.0757175194072,122.));
#45177=CARTESIAN_POINT('Ctrl Pts',(-86.5346187926945,-39.1277953993686,
122.));
#45178=CARTESIAN_POINT('Ctrl Pts',(-86.6245774697256,-39.1750660640383,
122.));
#45179=CARTESIAN_POINT('Ctrl Pts',(-86.7080355169804,-39.218920837096,122.));
#45180=CARTESIAN_POINT('Ctrl Pts',(-86.7935419058644,-39.2586383254852,
122.));
#45181=CARTESIAN_POINT('Ctrl Pts',(-86.8808924954566,-39.2939436042708,
122.));
#45182=CARTESIAN_POINT('Ctrl Pts',(-86.9113226722305,-39.3062428443735,
122.));
#45183=CARTESIAN_POINT('Ctrl Pts',(-86.9419768694861,-39.3180063257841,
122.));
#45184=CARTESIAN_POINT('Ctrl Pts',(-86.9728421809426,-39.3292377709744,
122.));
#45185=CARTESIAN_POINT('Ctrl Pts',(-90.2867226440827,-36.3571243050301,
120.387416697508));
#45186=CARTESIAN_POINT('Ctrl Pts',(-90.2883050038283,-36.5314907278085,
120.398449387697));
#45187=CARTESIAN_POINT('Ctrl Pts',(-90.271719409744,-36.7055581052199,120.409482077886));
#45188=CARTESIAN_POINT('Ctrl Pts',(-90.2358478507299,-36.8755557414102,
120.420514768075));
#45189=CARTESIAN_POINT('Ctrl Pts',(-90.0646638610358,-37.6868077304914,
120.473164275806));
#45190=CARTESIAN_POINT('Ctrl Pts',(-89.4542749914255,-38.4053783209051,
120.525813783537));
#45191=CARTESIAN_POINT('Ctrl Pts',(-88.6813900818485,-38.7055235825695,
120.578463291268));
#45192=CARTESIAN_POINT('Ctrl Pts',(-87.9085051722716,-39.005668844234,120.631112798999));
#45193=CARTESIAN_POINT('Ctrl Pts',(-86.973124222728,-38.8873887771492,120.683762306729));
#45194=CARTESIAN_POINT('Ctrl Pts',(-86.2992914012199,-38.4042850949718,
120.73641181446));
#45195=CARTESIAN_POINT('Ctrl Pts',(-85.6254585797119,-37.9211814127945,
120.789061322191));
#45196=CARTESIAN_POINT('Ctrl Pts',(-85.2131738862394,-37.0732541155246,
120.841710829922));
#45197=CARTESIAN_POINT('Ctrl Pts',(-85.2493332450303,-36.2449367230749,
120.894360337653));
#45198=CARTESIAN_POINT('Ctrl Pts',(-85.2854926038213,-35.4166193306253,
120.947009845384));
#45199=CARTESIAN_POINT('Ctrl Pts',(-85.7700960148757,-34.6079118429959,
120.999659353114));
#45200=CARTESIAN_POINT('Ctrl Pts',(-86.4834704355749,-34.1853501702909,
121.052308860845));
#45201=CARTESIAN_POINT('Ctrl Pts',(-87.196844856274,-33.7627884975859,121.104958368576));
#45202=CARTESIAN_POINT('Ctrl Pts',(-88.138990286618,-33.7263726398051,121.157607876307));
#45203=CARTESIAN_POINT('Ctrl Pts',(-88.8827695148683,-34.0927743330292,
121.210257384038));
#45204=CARTESIAN_POINT('Ctrl Pts',(-89.6265487431185,-34.4591760262532,
121.262906891768));
#45205=CARTESIAN_POINT('Ctrl Pts',(-90.1719617692751,-35.228395270482,121.315556399499));
#45206=CARTESIAN_POINT('Ctrl Pts',(-90.2718154335226,-36.0513826567645,
121.36820590723));
#45207=CARTESIAN_POINT('Ctrl Pts',(-90.2839603258177,-36.1514800667287,
121.374609503989));
#45208=CARTESIAN_POINT('Ctrl Pts',(-90.2895140119517,-36.2523728744322,
121.381013100749));
#45209=CARTESIAN_POINT('Ctrl Pts',(-90.2887582439581,-36.3533471924086,
121.387416697508));
#45210=CARTESIAN_POINT('Ctrl Pts',(-88.5623548711056,-39.3241490284291,
122.));
#45211=CARTESIAN_POINT('Ctrl Pts',(-89.5445934608772,-39.0615549760513,
121.947350492269));
#45212=CARTESIAN_POINT('Ctrl Pts',(-91.2113487416866,-37.4887074581619,
121.842051476808));
#45213=CARTESIAN_POINT('Ctrl Pts',(-90.6005808115744,-34.0865211443674,
121.684102953615));
#45214=CARTESIAN_POINT('Ctrl Pts',(-87.417021209647,-32.7460642638912,121.526154430423));
#45215=CARTESIAN_POINT('Ctrl Pts',(-84.5546283385357,-34.6751866943283,
121.36820590723));
#45216=CARTESIAN_POINT('Ctrl Pts',(-84.6050187185395,-38.1284686676829,
121.210257384038));
#45217=CARTESIAN_POINT('Ctrl Pts',(-87.5242687364515,-39.9731543606838,
121.052308860845));
#45218=CARTESIAN_POINT('Ctrl Pts',(-90.6647256725097,-38.5375840815526,
120.894360337653));
#45219=CARTESIAN_POINT('Ctrl Pts',(-91.1794496835569,-35.1229272613484,
120.73641181446));
#45220=CARTESIAN_POINT('Ctrl Pts',(-88.6015534311407,-32.8253528646868,
120.578463291268));
#45221=CARTESIAN_POINT('Ctrl Pts',(-85.2684356186448,-33.7279027825514,
120.420514768075));
#45222=CARTESIAN_POINT('Ctrl Pts',(-84.2020848645994,-37.0123105603124,
120.262566244883));
#45223=CARTESIAN_POINT('Ctrl Pts',(-86.3693522710391,-39.7006801660047,
120.10461772169));
#45224=CARTESIAN_POINT('Ctrl Pts',(-89.8052310634475,-39.3555600144301,
119.946669198498));
#45225=CARTESIAN_POINT('Ctrl Pts',(-91.3945199480195,-36.2898545206677,
119.788720675305));
#45226=CARTESIAN_POINT('Ctrl Pts',(-89.6962563501485,-33.2831483055448,
119.630772152113));
#45227=CARTESIAN_POINT('Ctrl Pts',(-86.2502055262826,-33.0615291420779,
119.47282362892));
#45228=CARTESIAN_POINT('Ctrl Pts',(-84.1807963181542,-35.8259330212369,
119.314875105728));
#45229=CARTESIAN_POINT('Ctrl Pts',(-85.3642994245004,-39.0699587122372,
119.156926582536));
#45230=CARTESIAN_POINT('Ctrl Pts',(-88.7276684236758,-39.8523469339212,
118.998978059343));
#45231=CARTESIAN_POINT('Ctrl Pts',(-91.2214390091811,-37.4637300078743,
118.841029536151));
#45232=CARTESIAN_POINT('Ctrl Pts',(-90.5845852003404,-34.069794289975,118.683081012958));
#45233=CARTESIAN_POINT('Ctrl Pts',(-87.3945229938104,-32.7477180564772,
118.525132489766));
#45234=CARTESIAN_POINT('Ctrl Pts',(-84.5435847625254,-34.6961876275626,
118.367183966573));
#45235=CARTESIAN_POINT('Ctrl Pts',(-84.6166294974947,-38.1485848990669,
118.209235443381));
#45236=CARTESIAN_POINT('Ctrl Pts',(-87.5474297570977,-39.9747262668198,
118.051286920188));
#45237=CARTESIAN_POINT('Ctrl Pts',(-90.6787180831755,-38.518904891293,117.893338396996));
#45238=CARTESIAN_POINT('Ctrl Pts',(-91.1714505838346,-35.1010697373407,
117.735389873803));
#45239=CARTESIAN_POINT('Ctrl Pts',(-88.5788816867368,-32.8200679900657,
117.577441350611));
#45240=CARTESIAN_POINT('Ctrl Pts',(-85.2516147613512,-33.7440145603012,
117.419492827418));
#45241=CARTESIAN_POINT('Ctrl Pts',(-84.2063815347296,-37.0351951933252,
117.261544304226));
#45242=CARTESIAN_POINT('Ctrl Pts',(-86.390863184092,-39.7095965059354,117.103595781033));
#45243=CARTESIAN_POINT('Ctrl Pts',(-89.8244566359805,-39.3424201662145,
116.945647257841));
#45244=CARTESIAN_POINT('Ctrl Pts',(-91.3940271355856,-36.26657379423,116.787698734648));
#45245=CARTESIAN_POINT('Ctrl Pts',(-89.6764928472477,-33.2708337478186,
116.629750211456));
#45246=CARTESIAN_POINT('Ctrl Pts',(-86.2290898737567,-33.071346415748,116.471801688264));
#45247=CARTESIAN_POINT('Ctrl Pts',(-84.1774736431561,-35.848980894873,116.313853165071));
#45248=CARTESIAN_POINT('Ctrl Pts',(-85.3817821946438,-39.0853404809052,
116.155904641879));
#45249=CARTESIAN_POINT('Ctrl Pts',(-88.7501055919751,-39.8461163666165,
115.997956118686));
#45250=CARTESIAN_POINT('Ctrl Pts',(-91.2284874537149,-37.4415361943852,
115.840007595494));
#45251=CARTESIAN_POINT('Ctrl Pts',(-90.5698543224008,-34.0517596743733,
115.682059072301));
#45252=CARTESIAN_POINT('Ctrl Pts',(-87.3713688267741,-32.750194081883,115.524110549109));
#45253=CARTESIAN_POINT('Ctrl Pts',(-84.5330004881805,-34.7169293542972,
115.366162025916));
#45254=CARTESIAN_POINT('Ctrl Pts',(-84.628211554152,-38.1687864356674,115.208213502724));
#45255=CARTESIAN_POINT('Ctrl Pts',(-87.5706770468859,-39.9760714938026,
115.050264979531));
#45256=CARTESIAN_POINT('Ctrl Pts',(-90.6925529951631,-38.5001741325821,
114.892316456339));
#45257=CARTESIAN_POINT('Ctrl Pts',(-91.1633294242455,-35.0792456020353,
114.734367933146));
#45258=CARTESIAN_POINT('Ctrl Pts',(-88.556167663902,-32.8149377579708,114.576419409954));
#45259=CARTESIAN_POINT('Ctrl Pts',(-85.2349019889955,-33.760229656792,114.418470886761));
#45260=CARTESIAN_POINT('Ctrl Pts',(-84.2108229752343,-37.058053883591,114.260522363569));
#45261=CARTESIAN_POINT('Ctrl Pts',(-86.4124319184404,-39.7183735107193,
114.102573840377));
#45262=CARTESIAN_POINT('Ctrl Pts',(-89.8435969487181,-39.3291576422236,
113.944625317184));
#45263=CARTESIAN_POINT('Ctrl Pts',(-91.3933850872816,-36.2432964686034,
113.786676793992));
#45264=CARTESIAN_POINT('Ctrl Pts',(-89.6566505635712,-33.2586464637551,
113.628728270799));
#45265=CARTESIAN_POINT('Ctrl Pts',(-86.2080377498421,-33.081299013048,113.470779747607));
#45266=CARTESIAN_POINT('Ctrl Pts',(-84.1742989994849,-35.8720496562593,
113.312831224414));
#45267=CARTESIAN_POINT('Ctrl Pts',(-85.3993633840806,-39.1006096620336,
113.154882701222));
#45268=CARTESIAN_POINT('Ctrl Pts',(-88.7725022847651,-39.8397418653489,
112.996934178029));
#45269=CARTESIAN_POINT('Ctrl Pts',(-91.23539324967,-37.4192975771493,112.838985654837));
#45270=CARTESIAN_POINT('Ctrl Pts',(-90.555007946359,-34.0338200190599,112.681037131644));
#45271=CARTESIAN_POINT('Ctrl Pts',(-87.3482310363601,-32.7528187283548,
112.523088608452));
#45272=CARTESIAN_POINT('Ctrl Pts',(-84.5225496142588,-34.7377386154233,
112.365140085259));
#45273=CARTESIAN_POINT('Ctrl Pts',(-84.6399230862583,-38.1889131872696,
112.207191562067));
#45274=CARTESIAN_POINT('Ctrl Pts',(-87.5939324950497,-39.9772674223311,
112.049243038875));
#45275=CARTESIAN_POINT('Ctrl Pts',(-90.7062673518165,-38.4813549260119,
111.891294515682));
#45276=CARTESIAN_POINT('Ctrl Pts',(-91.1550682993145,-35.0574740626047,
111.733345992489));
#45277=CARTESIAN_POINT('Ctrl Pts',(-88.5334211681103,-32.8099534783274,
111.575397469297));
#45278=CARTESIAN_POINT('Ctrl Pts',(-85.218293678275,-33.7765517317041,111.417448946105));
#45279=CARTESIAN_POINT('Ctrl Pts',(-84.2154110997942,-37.0808835841375,
111.259500422912));
#45280=CARTESIAN_POINT('Ctrl Pts',(-86.4340565652882,-39.7270118417731,
111.10155189972));
#45281=CARTESIAN_POINT('Ctrl Pts',(-89.8626517082315,-39.3157724916908,
110.943603376527));
#45282=CARTESIAN_POINT('Ctrl Pts',(-91.3925935885532,-36.2200237454849,
110.785654853335));
#45283=CARTESIAN_POINT('Ctrl Pts',(-89.6367304343865,-33.2465868380812,
110.627706330142));
#45284=CARTESIAN_POINT('Ctrl Pts',(-86.18704996557,-33.091386581079,110.46975780695));
#45285=CARTESIAN_POINT('Ctrl Pts',(-84.1712725456449,-35.8951383259589,
110.311809283757));
#45286=CARTESIAN_POINT('Ctrl Pts',(-85.4170422546641,-39.1157656406506,
110.153860760565));
#45287=CARTESIAN_POINT('Ctrl Pts',(-88.794857584793,-39.8332236842038,109.995912237372));
#45288=CARTESIAN_POINT('Ctrl Pts',(-91.2421561099518,-37.3970150806926,
109.83796371418));
#45289=CARTESIAN_POINT('Ctrl Pts',(-90.5400466842003,-34.0159760529972,
109.680015190987));
#45290=CARTESIAN_POINT('Ctrl Pts',(-87.3251105792218,-32.7555919072101,
109.522066667795));
#45291=CARTESIAN_POINT('Ctrl Pts',(-84.5122325649308,-34.7586145140015,
109.364118144603));
#45292=CARTESIAN_POINT('Ctrl Pts',(-84.6517636253375,-38.2089644036472,
109.20616962141));
#45293=CARTESIAN_POINT('Ctrl Pts',(-87.6171951129081,-39.9783138396851,
109.048221098218));
#45294=CARTESIAN_POINT('Ctrl Pts',(-90.7198606492592,-38.4624483834354,
108.890272575025));
#45295=CARTESIAN_POINT('Ctrl Pts',(-91.1466674229692,-35.0357553258326,
108.732324051833));
#45296=CARTESIAN_POINT('Ctrl Pts',(-88.5106433977503,-32.8051167774314,
108.57437552864));
#45297=CARTESIAN_POINT('Ctrl Pts',(-85.2017899780534,-33.7929771900336,
108.416427005448));
#45298=CARTESIAN_POINT('Ctrl Pts',(-84.2201468213852,-37.1036893633033,
108.258478482255));
#45299=CARTESIAN_POINT('Ctrl Pts',(-86.4557339663443,-39.7354987833619,
108.100529959063));
#45300=CARTESIAN_POINT('Ctrl Pts',(-89.8816247907176,-39.3022906856884,
107.94258143587));
#45301=CARTESIAN_POINT('Ctrl Pts',(-91.3916430843464,-36.1967043062389,
107.784632912678));
#45302=CARTESIAN_POINT('Ctrl Pts',(-89.6167529992886,-33.2347628855613,
107.626684389485));
#45303=CARTESIAN_POINT('Ctrl Pts',(-86.1660868316116,-33.1013875794135,
107.468735866293));
#45304=CARTESIAN_POINT('Ctrl Pts',(-84.1684777778814,-35.918700775767,107.3107873431));
#45305=CARTESIAN_POINT('Ctrl Pts',(-85.434646301384,-39.1298724576138,107.152838819908));
#45306=CARTESIAN_POINT('Ctrl Pts',(-88.8175143837618,-39.8284996290504,
106.994890296716));
#45307=CARTESIAN_POINT('Ctrl Pts',(-91.2479889654302,-37.3707155689491,
106.836941773523));
#45308=CARTESIAN_POINT('Ctrl Pts',(-90.7653388102639,-35.1304094942453,
106.731642758061));
#45309=CARTESIAN_POINT('Ctrl Pts',(-90.1046182462678,-34.3576245177522,
106.678993250331));
#45310=CARTESIAN_POINT('Ctrl Pts',(-88.5144884429196,-39.1451036445255,
122.10700224989));
#45311=CARTESIAN_POINT('Ctrl Pts',(-89.4374976355964,-38.8983441231517,
122.054352742159));
#45312=CARTESIAN_POINT('Ctrl Pts',(-91.003746877023,-37.4203399673302,121.949053726697));
#45313=CARTESIAN_POINT('Ctrl Pts',(-90.4298085081212,-34.223306908833,121.791105203505));
#45314=CARTESIAN_POINT('Ctrl Pts',(-87.4382188794787,-32.9636801379545,
121.633156680312));
#45315=CARTESIAN_POINT('Ctrl Pts',(-84.7484294936813,-34.7764756803353,
121.47520815712));
#45316=CARTESIAN_POINT('Ctrl Pts',(-84.7957813127306,-38.0215233087861,
121.317259633928));
#45317=CARTESIAN_POINT('Ctrl Pts',(-87.5389993356358,-39.7549736842546,
121.159311110735));
#45318=CARTESIAN_POINT('Ctrl Pts',(-90.4900854071588,-38.4059688923743,
121.001362587543));
#45319=CARTESIAN_POINT('Ctrl Pts',(-90.9737713454176,-35.1972173042109,
120.84341406435));
#45320=CARTESIAN_POINT('Ctrl Pts',(-88.5513233134175,-33.0381876030153,
120.685465541158));
#45321=CARTESIAN_POINT('Ctrl Pts',(-85.4191938967511,-33.8863133839749,
120.527517017965));
#45322=CARTESIAN_POINT('Ctrl Pts',(-84.4171445384271,-36.9726700013395,
120.369568494773));
#45323=CARTESIAN_POINT('Ctrl Pts',(-86.4537248153207,-39.4989297972856,
120.21161997158));
#45324=CARTESIAN_POINT('Ctrl Pts',(-89.6824186819031,-39.1746205349551,
120.053671448388));
#45325=CARTESIAN_POINT('Ctrl Pts',(-91.175872783131,-36.2937783625453,119.895722925195));
#45326=CARTESIAN_POINT('Ctrl Pts',(-89.5800151893182,-33.4683777876381,
119.737774402003));
#45327=CARTESIAN_POINT('Ctrl Pts',(-86.3417626690224,-33.2601223522649,
119.57982587881));
#45328=CARTESIAN_POINT('Ctrl Pts',(-84.3971397002217,-35.8578315232397,
119.421877355618));
#45329=CARTESIAN_POINT('Ctrl Pts',(-85.5092770750858,-38.9062411105366,
119.263928832425));
#45330=CARTESIAN_POINT('Ctrl Pts',(-88.6698335192436,-39.6414509957686,
119.105980309233));
#45331=CARTESIAN_POINT('Ctrl Pts',(-91.0132286971742,-37.3968686677242,
118.94803178604));
#45332=CARTESIAN_POINT('Ctrl Pts',(-90.4147774389237,-34.2075886907448,
118.790083262848));
#45333=CARTESIAN_POINT('Ctrl Pts',(-87.4170773154511,-32.965234206157,118.632134739655));
#45334=CARTESIAN_POINT('Ctrl Pts',(-84.7380518499156,-34.7962102485267,
118.474186216463));
#45335=CARTESIAN_POINT('Ctrl Pts',(-84.8066919568667,-38.0404265230182,
118.316237693271));
#45336=CARTESIAN_POINT('Ctrl Pts',(-87.5607637370663,-39.7564508037941,
118.158289170078));
#45337=CARTESIAN_POINT('Ctrl Pts',(-90.5032340696187,-38.3884160650867,
118.000340646886));
#45338=CARTESIAN_POINT('Ctrl Pts',(-90.9662545947489,-35.1766777980275,
117.842392123693));
#45339=CARTESIAN_POINT('Ctrl Pts',(-88.5300186846675,-33.0332214085406,
117.684443600501));
#45340=CARTESIAN_POINT('Ctrl Pts',(-85.4033873441759,-33.9014536147989,
117.526495077308));
#45341=CARTESIAN_POINT('Ctrl Pts',(-84.4211821175544,-36.9941746814262,
117.368546554116));
#45342=CARTESIAN_POINT('Ctrl Pts',(-86.4739386113346,-39.5073084781955,
117.210598030923));
#45343=CARTESIAN_POINT('Ctrl Pts',(-89.7004849443846,-39.1622730250734,
117.052649507731));
#45344=CARTESIAN_POINT('Ctrl Pts',(-91.1754096874929,-36.2719014736327,
116.894700984538));
#45345=CARTESIAN_POINT('Ctrl Pts',(-89.5614434338944,-33.4568058028847,
116.736752461346));
#45346=CARTESIAN_POINT('Ctrl Pts',(-86.3219202991608,-33.2693476402335,
116.578803938153));
#45347=CARTESIAN_POINT('Ctrl Pts',(-84.3940173839133,-35.8794896004719,
116.420855414961));
#45348=CARTESIAN_POINT('Ctrl Pts',(-85.5257056268899,-38.9206953521314,
116.262906891768));
#45349=CARTESIAN_POINT('Ctrl Pts',(-88.6909177169257,-39.6355961342739,
116.104958368576));
#45350=CARTESIAN_POINT('Ctrl Pts',(-91.0198521175596,-37.3760131504555,
115.947009845384));
#45351=CARTESIAN_POINT('Ctrl Pts',(-90.4009348390746,-34.1906415699941,
115.789061322191));
#45352=CARTESIAN_POINT('Ctrl Pts',(-87.395319354355,-32.967560926197,115.631112798999));
#45353=CARTESIAN_POINT('Ctrl Pts',(-84.7281058117332,-34.8157012404785,
115.473164275806));
#45354=CARTESIAN_POINT('Ctrl Pts',(-84.8175756106714,-38.0594098985265,
115.315215752614));
#45355=CARTESIAN_POINT('Ctrl Pts',(-87.5826092055734,-39.7577149130283,
115.157267229421));
#45356=CARTESIAN_POINT('Ctrl Pts',(-90.5162347306368,-38.3708147789471,
114.999318706229));
#45357=CARTESIAN_POINT('Ctrl Pts',(-90.9586231444738,-35.1561696671936,
114.841370183036));
#45358=CARTESIAN_POINT('Ctrl Pts',(-88.508674326894,-33.0284005315831,114.683421659844));
#45359=CARTESIAN_POINT('Ctrl Pts',(-85.3876823589715,-33.9166909342007,
114.525473136651));
#45360=CARTESIAN_POINT('Ctrl Pts',(-84.4253557373423,-37.0156549831244,
114.367524613459));
#45361=CARTESIAN_POINT('Ctrl Pts',(-86.4942067419958,-39.515556225926,114.209576090266));
#45362=CARTESIAN_POINT('Ctrl Pts',(-89.7184710882722,-39.1498102368169,
114.051627567074));
#45363=CARTESIAN_POINT('Ctrl Pts',(-91.1748063549696,-36.2500277804607,
113.893679043881));
#45364=CARTESIAN_POINT('Ctrl Pts',(-89.5427976482087,-33.445353417139,113.735730520689));
#45365=CARTESIAN_POINT('Ctrl Pts',(-86.3021376271084,-33.2787000917606,
113.577781997497));
#45366=CARTESIAN_POINT('Ctrl Pts',(-84.3910341725811,-35.9011673059144,
113.419833474304));
#45367=CARTESIAN_POINT('Ctrl Pts',(-85.5422266632625,-38.935043795262,113.261884951112));
#45368=CARTESIAN_POINT('Ctrl Pts',(-88.7119638797888,-39.6296060180944,
113.103936427919));
#45369=CARTESIAN_POINT('Ctrl Pts',(-91.0263414911353,-37.3551155311246,
112.945987904727));
#45370=CARTESIAN_POINT('Ctrl Pts',(-90.3869837057071,-34.1737836833869,
112.788039381534));
#45371=CARTESIAN_POINT('Ctrl Pts',(-87.3735767823643,-32.9700273053906,
112.630090858342));
#45372=CARTESIAN_POINT('Ctrl Pts',(-84.7182851298726,-34.8352556944698,
112.472142335149));
#45373=CARTESIAN_POINT('Ctrl Pts',(-84.8285809325017,-38.0783229986033,
112.314193811957));
#45374=CARTESIAN_POINT('Ctrl Pts',(-87.6044623405025,-39.7588387265671,
112.156245288764));
#45375=CARTESIAN_POINT('Ctrl Pts',(-90.5291221058576,-38.353130378391,111.998296765572));
#45376=CARTESIAN_POINT('Ctrl Pts',(-90.9508601688256,-35.1357109606813,
111.840348242379));
#45377=CARTESIAN_POINT('Ctrl Pts',(-88.4872994542962,-33.0237168060833,
111.682399719187));
#45378=CARTESIAN_POINT('Ctrl Pts',(-85.3720755363224,-33.9320287811804,
111.524451195994));
#45379=CARTESIAN_POINT('Ctrl Pts',(-84.4296671960753,-37.0371080431954,
111.366502672802));
#45380=CARTESIAN_POINT('Ctrl Pts',(-86.5145274136095,-39.5236736620104,
111.20855414961));
#45381=CARTESIAN_POINT('Ctrl Pts',(-89.7363768378307,-39.1372322164502,
111.050605626417));
#45382=CARTESIAN_POINT('Ctrl Pts',(-91.1740625839451,-36.2281584122637,
110.892657103225));
#45383=CARTESIAN_POINT('Ctrl Pts',(-89.5240787111315,-33.4340209919287,
110.734708580032));
#45384=CARTESIAN_POINT('Ctrl Pts',(-86.2824154149913,-33.2881793752273,
110.57676005684));
#45385=CARTESIAN_POINT('Ctrl Pts',(-84.3881902151712,-35.9228637191904,
110.418811533647));
#45386=CARTESIAN_POINT('Ctrl Pts',(-85.5588394905682,-38.9492858620401,
110.260863010455));
#45387=CARTESIAN_POINT('Ctrl Pts',(-88.7329711458906,-39.623480885994,110.102914487262));
#45388=CARTESIAN_POINT('Ctrl Pts',(-91.0326965481183,-37.3341766785082,
109.94496596407));
#45389=CARTESIAN_POINT('Ctrl Pts',(-90.3729246139036,-34.1570157159285,
109.787017440877));
#45390=CARTESIAN_POINT('Ctrl Pts',(-87.3518504984453,-32.972633260403,109.629068917685));
#45391=CARTESIAN_POINT('Ctrl Pts',(-84.708590202927,-34.8548727676472,109.471120394492));
#45392=CARTESIAN_POINT('Ctrl Pts',(-84.8397074821303,-38.0971651182609,
109.3131718713));
#45393=CARTESIAN_POINT('Ctrl Pts',(-87.6263222127909,-39.7598220445177,
109.155223348107));
#45394=CARTESIAN_POINT('Ctrl Pts',(-90.5418957217887,-38.3353639082262,
108.997274824915));
#45395=CARTESIAN_POINT('Ctrl Pts',(-90.9429658688318,-35.1153018728052,
108.839326301722));
#45396=CARTESIAN_POINT('Ctrl Pts',(-88.4658951929996,-33.0191717602709,
108.68137777853));
#45397=CARTESIAN_POINT('Ctrl Pts',(-85.3565670161152,-33.9474637775143,
108.523429255337));
#45398=CARTESIAN_POINT('Ctrl Pts',(-84.4341173516769,-37.058538624355,108.365480732145));
#45399=CARTESIAN_POINT('Ctrl Pts',(-86.5348976583306,-39.5316488374778,
108.207532208953));
#45400=CARTESIAN_POINT('Ctrl Pts',(-89.7542058355207,-39.124563368979,108.04958368576));
#45401=CARTESIAN_POINT('Ctrl Pts',(-91.1731693955388,-36.2062451449413,
107.891635162568));
#45402=CARTESIAN_POINT('Ctrl Pts',(-89.5053059237116,-33.4229100286828,
107.733686639375));
#45403=CARTESIAN_POINT('Ctrl Pts',(-86.2627163667637,-33.2975773091863,
107.575738116183));
#45404=CARTESIAN_POINT('Ctrl Pts',(-84.3855639730709,-35.9450053434366,
107.41778959299));
#45405=CARTESIAN_POINT('Ctrl Pts',(-85.5753820059203,-38.9625420320502,
107.259841069798));
#45406=CARTESIAN_POINT('Ctrl Pts',(-88.7542617304213,-39.6190416933389,
107.101892546605));
#45407=CARTESIAN_POINT('Ctrl Pts',(-91.0381776799758,-37.3094630383042,
106.943944023413));
#45408=CARTESIAN_POINT('Ctrl Pts',(-90.5846315306955,-35.2042483553399,
106.838645007951));
#45409=CARTESIAN_POINT('Ctrl Pts',(-89.9637526925908,-34.4780626356041,
106.78599550022));
#45410=CARTESIAN_POINT('Ctrl Pts',(-88.4666220147337,-38.966058260622,122.21400449978));
#45411=CARTESIAN_POINT('Ctrl Pts',(-89.3304018103156,-38.7351332702521,
122.161354992049));
#45412=CARTESIAN_POINT('Ctrl Pts',(-90.7961450123593,-37.3519724764984,
122.056055976587));
#45413=CARTESIAN_POINT('Ctrl Pts',(-90.2590362046681,-34.3600926732987,
121.898107453395));
#45414=CARTESIAN_POINT('Ctrl Pts',(-87.4594165493103,-33.1812960120178,
121.740158930202));
#45415=CARTESIAN_POINT('Ctrl Pts',(-84.942230648827,-34.8777646663423,121.58221040701));
#45416=CARTESIAN_POINT('Ctrl Pts',(-84.9865439069216,-37.9145779498893,
121.424261883817));
#45417=CARTESIAN_POINT('Ctrl Pts',(-87.5537299348201,-39.5367930078253,
121.266313360625));
#45418=CARTESIAN_POINT('Ctrl Pts',(-90.3154451418077,-38.2743537031959,
121.108364837432));
#45419=CARTESIAN_POINT('Ctrl Pts',(-90.7680930072786,-35.2715073470735,
120.95041631424));
#45420=CARTESIAN_POINT('Ctrl Pts',(-88.5010931956941,-33.2510223413438,
120.792467791047));
#45421=CARTESIAN_POINT('Ctrl Pts',(-85.5699521748575,-34.0447239853984,
120.634519267855));
#45422=CARTESIAN_POINT('Ctrl Pts',(-84.6322042122549,-36.9330294423666,
120.476570744662));
#45423=CARTESIAN_POINT('Ctrl Pts',(-86.5380973596023,-39.2971794285665,
120.31862222147));
#45424=CARTESIAN_POINT('Ctrl Pts',(-89.5596063003586,-38.9936810554801,
120.160673698277));
#45425=CARTESIAN_POINT('Ctrl Pts',(-90.9572256182428,-36.297702204423,120.002725175085));
#45426=CARTESIAN_POINT('Ctrl Pts',(-89.4637740284878,-33.6536072697314,
119.844776651892));
#45427=CARTESIAN_POINT('Ctrl Pts',(-86.4333198117624,-33.4587155624518,
119.6868281287));
#45428=CARTESIAN_POINT('Ctrl Pts',(-84.613483082289,-35.8897300252424,119.528879605508));
#45429=CARTESIAN_POINT('Ctrl Pts',(-85.6542547256714,-38.7425235088361,
119.370931082315));
#45430=CARTESIAN_POINT('Ctrl Pts',(-88.6119986148113,-39.430555057616,119.212982559123));
#45431=CARTESIAN_POINT('Ctrl Pts',(-90.8050183851675,-37.3300073275741,
119.05503403593));
#45432=CARTESIAN_POINT('Ctrl Pts',(-90.244969677507,-34.3453830915146,118.897085512738));
#45433=CARTESIAN_POINT('Ctrl Pts',(-87.4396316370916,-33.1827503558368,
118.739136989545));
#45434=CARTESIAN_POINT('Ctrl Pts',(-84.932518937306,-34.8962328694908,118.581188466353));
#45435=CARTESIAN_POINT('Ctrl Pts',(-84.9967544162386,-37.9322681469695,
118.42323994316));
#45436=CARTESIAN_POINT('Ctrl Pts',(-87.5740977170349,-39.5381753407685,
118.265291419968));
#45437=CARTESIAN_POINT('Ctrl Pts',(-90.327750056062,-38.2579272388805,118.107342896775));
#45438=CARTESIAN_POINT('Ctrl Pts',(-90.761058605663,-35.2522858587143,117.949394373583));
#45439=CARTESIAN_POINT('Ctrl Pts',(-88.4811556825983,-33.2463748270155,
117.79144585039));
#45440=CARTESIAN_POINT('Ctrl Pts',(-85.5551599270005,-34.0588926692967,
117.633497327198));
#45441=CARTESIAN_POINT('Ctrl Pts',(-84.6359827003793,-36.9531541695272,
117.475548804006));
#45442=CARTESIAN_POINT('Ctrl Pts',(-86.5570140385773,-39.3050204504555,
117.317600280813));
#45443=CARTESIAN_POINT('Ctrl Pts',(-89.5765132527889,-38.9821258839323,
117.159651757621));
#45444=CARTESIAN_POINT('Ctrl Pts',(-90.9567922394001,-36.2772291530353,
117.001703234428));
#45445=CARTESIAN_POINT('Ctrl Pts',(-89.4463940205411,-33.6427778579508,
116.843754711236));
#45446=CARTESIAN_POINT('Ctrl Pts',(-86.4147507245648,-33.4673488647189,
116.685806188043));
#45447=CARTESIAN_POINT('Ctrl Pts',(-84.6105611246705,-35.9099983060708,
116.527857664851));
#45448=CARTESIAN_POINT('Ctrl Pts',(-85.6696290591357,-38.7560502233575,
116.369909141658));
#45449=CARTESIAN_POINT('Ctrl Pts',(-88.6317298418765,-39.4250759019314,
116.211960618466));
#45450=CARTESIAN_POINT('Ctrl Pts',(-90.8112167814044,-37.3104901065257,
116.054012095273));
#45451=CARTESIAN_POINT('Ctrl Pts',(-90.2320153557485,-34.329523465615,115.896063572081));
#45452=CARTESIAN_POINT('Ctrl Pts',(-87.4192698819359,-33.184927770511,115.738115048888));
#45453=CARTESIAN_POINT('Ctrl Pts',(-84.9232111352859,-34.9144731266598,
115.580166525696));
#45454=CARTESIAN_POINT('Ctrl Pts',(-85.006939667191,-37.9500333613858,115.422218002503));
#45455=CARTESIAN_POINT('Ctrl Pts',(-87.5945413642607,-39.5393583322538,
115.264269479311));
#45456=CARTESIAN_POINT('Ctrl Pts',(-90.3399164661106,-38.2414554253121,
115.106320956119));
#45457=CARTESIAN_POINT('Ctrl Pts',(-90.7539168647021,-35.2330937323519,
114.948372432926));
#45458=CARTESIAN_POINT('Ctrl Pts',(-88.4611809898858,-33.2418633051955,
114.790423909734));
#45459=CARTESIAN_POINT('Ctrl Pts',(-85.5404627289477,-34.0731522116095,
114.632475386541));
#45460=CARTESIAN_POINT('Ctrl Pts',(-84.6398884994501,-36.9732560826578,
114.474526863349));
#45461=CARTESIAN_POINT('Ctrl Pts',(-86.5759815655513,-39.3127389411328,
114.316578340156));
#45462=CARTESIAN_POINT('Ctrl Pts',(-89.5933452278263,-38.9704628314102,
114.158629816964));
#45463=CARTESIAN_POINT('Ctrl Pts',(-90.9562276226576,-36.2567590923181,
114.000681293771));
#45464=CARTESIAN_POINT('Ctrl Pts',(-89.4289447328463,-33.6320603705229,
113.842732770579));
#45465=CARTESIAN_POINT('Ctrl Pts',(-86.3962375043747,-33.4761011704732,
113.684784247386));
#45466=CARTESIAN_POINT('Ctrl Pts',(-84.6077693456771,-35.9302849555694,
113.526835724194));
#45467=CARTESIAN_POINT('Ctrl Pts',(-85.6850899424446,-38.7694779284905,
113.368887201001));
#45468=CARTESIAN_POINT('Ctrl Pts',(-88.6514254748125,-39.41947017084,113.210938677809));
#45469=CARTESIAN_POINT('Ctrl Pts',(-90.8172897326005,-37.2909334850999,
113.052990154616));
#45470=CARTESIAN_POINT('Ctrl Pts',(-90.2189594650554,-34.3137473477138,
112.895041631424));
#45471=CARTESIAN_POINT('Ctrl Pts',(-87.3989225283682,-33.1872358824264,
112.737093108232));
#45472=CARTESIAN_POINT('Ctrl Pts',(-84.9140206454866,-34.9327727735164,
112.579144585039));
#45473=CARTESIAN_POINT('Ctrl Pts',(-85.017238778745,-37.967732809937,112.421196061847));
#45474=CARTESIAN_POINT('Ctrl Pts',(-87.6149921859555,-39.5404100308031,
112.263247538654));
#45475=CARTESIAN_POINT('Ctrl Pts',(-90.3519768598988,-38.2249058307701,
112.105299015462));
#45476=CARTESIAN_POINT('Ctrl Pts',(-90.7466520383367,-35.213947858758,111.947350492269));
#45477=CARTESIAN_POINT('Ctrl Pts',(-88.441177740482,-33.2374801338393,111.789401969077));
#45478=CARTESIAN_POINT('Ctrl Pts',(-85.5258573943697,-34.0875058306568,
111.631453445884));
#45479=CARTESIAN_POINT('Ctrl Pts',(-84.6439232923566,-36.9933325022533,
111.473504922692));
#45480=CARTESIAN_POINT('Ctrl Pts',(-86.5949982619306,-39.3203354822477,
111.315556399499));
#45481=CARTESIAN_POINT('Ctrl Pts',(-89.6101019674299,-38.9586919412095,
111.157607876307));
#45482=CARTESIAN_POINT('Ctrl Pts',(-90.9555315793369,-36.2362930790426,
110.999659353114));
#45483=CARTESIAN_POINT('Ctrl Pts',(-89.4114269878765,-33.6214551457762,
110.841710829922));
#45484=CARTESIAN_POINT('Ctrl Pts',(-86.3777808644127,-33.4849721693756,
110.683762306729));
#45485=CARTESIAN_POINT('Ctrl Pts',(-84.6051078846975,-35.9505891124219,
110.525813783537));
#45486=CARTESIAN_POINT('Ctrl Pts',(-85.7006367264722,-38.7828060834297,
110.367865260344));
#45487=CARTESIAN_POINT('Ctrl Pts',(-88.6710847069883,-39.4137380877842,
110.209916737152));
#45488=CARTESIAN_POINT('Ctrl Pts',(-90.8232369862847,-37.2713382763238,
110.05196821396));
#45489=CARTESIAN_POINT('Ctrl Pts',(-90.2058025436072,-34.2980553788597,
109.894019690767));
#45490=CARTESIAN_POINT('Ctrl Pts',(-87.3785904176685,-33.1896746135959,
109.736071167575));
#45491=CARTESIAN_POINT('Ctrl Pts',(-84.9049478409233,-34.9511310212928,
109.578122644382));
#45492=CARTESIAN_POINT('Ctrl Pts',(-85.0276513389231,-37.9853658328746,
109.42017412119));
#45493=CARTESIAN_POINT('Ctrl Pts',(-87.6354493126737,-39.5413302493503,
109.262225597997));
#45494=CARTESIAN_POINT('Ctrl Pts',(-90.3639307943181,-38.208279433017,109.104277074805));
#45495=CARTESIAN_POINT('Ctrl Pts',(-90.7392643146943,-35.1948484197779,
108.946328551612));
#45496=CARTESIAN_POINT('Ctrl Pts',(-88.421146988249,-33.2332267431105,108.78838002842));
#45497=CARTESIAN_POINT('Ctrl Pts',(-85.511344054177,-34.1019503649949,108.630431505227));
#45498=CARTESIAN_POINT('Ctrl Pts',(-84.6480878819688,-37.0133878854068,
108.472482982035));
#45499=CARTESIAN_POINT('Ctrl Pts',(-86.6140613503167,-39.3277988915936,
108.314534458842));
#45500=CARTESIAN_POINT('Ctrl Pts',(-89.6267868803239,-38.9468360522697,
108.15658593565));
#45501=CARTESIAN_POINT('Ctrl Pts',(-90.9546957067312,-36.2157859836437,
107.998637412458));
#45502=CARTESIAN_POINT('Ctrl Pts',(-89.3938588481345,-33.6110571718043,
107.840688889265));
#45503=CARTESIAN_POINT('Ctrl Pts',(-86.3593459019159,-33.4937670389591,
107.682740366073));
#45504=CARTESIAN_POINT('Ctrl Pts',(-84.6026501682603,-35.9713099111062,
107.52479184288));
#45505=CARTESIAN_POINT('Ctrl Pts',(-85.7161177104565,-38.7952116064866,
107.366843319688));
#45506=CARTESIAN_POINT('Ctrl Pts',(-88.6910090770809,-39.4095837576274,
107.208894796495));
#45507=CARTESIAN_POINT('Ctrl Pts',(-90.8283663945213,-37.2482105076592,
107.050946273303));
#45508=CARTESIAN_POINT('Ctrl Pts',(-90.4039242511271,-35.2780872164347,
106.945647257841));
#45509=CARTESIAN_POINT('Ctrl Pts',(-89.8228871389138,-34.5985007534561,
106.89299775011));
#45510=CARTESIAN_POINT('Ctrl Pts',(-88.4187555865477,-38.7870128767185,
122.321006749669));
#45511=CARTESIAN_POINT('Ctrl Pts',(-89.2233059850348,-38.5719224173526,
122.268357241939));
#45512=CARTESIAN_POINT('Ctrl Pts',(-90.5885431476955,-37.2836049856667,
122.163058226477));
#45513=CARTESIAN_POINT('Ctrl Pts',(-90.0882639012151,-34.4968784377644,
122.005109703284));
#45514=CARTESIAN_POINT('Ctrl Pts',(-87.4806142191418,-33.3989118860811,
121.847161180092));
#45515=CARTESIAN_POINT('Ctrl Pts',(-85.1360318039727,-34.9790536523493,
121.689212656899));
#45516=CARTESIAN_POINT('Ctrl Pts',(-85.1773065011126,-37.8076325909925,
121.531264133707));
#45517=CARTESIAN_POINT('Ctrl Pts',(-87.5684605340043,-39.318612331396,121.373315610515));
#45518=CARTESIAN_POINT('Ctrl Pts',(-90.1408048764567,-38.1427385140175,
121.215367087322));
#45519=CARTESIAN_POINT('Ctrl Pts',(-90.5624146691395,-35.3457973899361,
121.05741856413));
#45520=CARTESIAN_POINT('Ctrl Pts',(-88.4508630779708,-33.4638570796724,
120.899470040937));
#45521=CARTESIAN_POINT('Ctrl Pts',(-85.7207104529639,-34.2031345868219,
120.741521517745));
#45522=CARTESIAN_POINT('Ctrl Pts',(-84.8472638860827,-36.8933888833937,
120.583572994552));
#45523=CARTESIAN_POINT('Ctrl Pts',(-86.6224699038839,-39.0954290598474,
120.42562447136));
#45524=CARTESIAN_POINT('Ctrl Pts',(-89.4367939188142,-38.8127415760051,
120.267675948167));
#45525=CARTESIAN_POINT('Ctrl Pts',(-90.7385784533545,-36.3016260463006,
120.109727424975));
#45526=CARTESIAN_POINT('Ctrl Pts',(-89.3475328676574,-33.8388367518247,
119.951778901782));
#45527=CARTESIAN_POINT('Ctrl Pts',(-86.5248769545022,-33.6573087726388,
119.79383037859));
#45528=CARTESIAN_POINT('Ctrl Pts',(-84.8298264643564,-35.9216285272452,
119.635881855397));
#45529=CARTESIAN_POINT('Ctrl Pts',(-85.7992323762569,-38.5788059071355,
119.477933332205));
#45530=CARTESIAN_POINT('Ctrl Pts',(-88.554163710379,-39.2196591194634,119.319984809013));
#45531=CARTESIAN_POINT('Ctrl Pts',(-90.5968080731607,-37.263145987424,119.16203628582));
#45532=CARTESIAN_POINT('Ctrl Pts',(-90.0751619160902,-34.4831774922844,
119.004087762628));
#45533=CARTESIAN_POINT('Ctrl Pts',(-87.4621859587324,-33.4002665055166,
118.846139239435));
#45534=CARTESIAN_POINT('Ctrl Pts',(-85.1269860246962,-34.9962554904548,
118.688190716243));
#45535=CARTESIAN_POINT('Ctrl Pts',(-85.1868168756106,-37.8241097709208,
118.53024219305));
#45536=CARTESIAN_POINT('Ctrl Pts',(-87.5874316970034,-39.3198998777429,
118.372293669858));
#45537=CARTESIAN_POINT('Ctrl Pts',(-90.1522660425053,-38.1274384126742,
118.214345146665));
#45538=CARTESIAN_POINT('Ctrl Pts',(-90.5558626165772,-35.3278939194011,
118.056396623473));
#45539=CARTESIAN_POINT('Ctrl Pts',(-88.4322926805291,-33.4595282454904,
117.89844810028));
#45540=CARTESIAN_POINT('Ctrl Pts',(-85.7069325098252,-34.2163317237944,
117.740499577088));
#45541=CARTESIAN_POINT('Ctrl Pts',(-84.8507832832042,-36.9121336576282,
117.582551053895));
#45542=CARTESIAN_POINT('Ctrl Pts',(-86.64008946582,-39.1027324227156,117.424602530703));
#45543=CARTESIAN_POINT('Ctrl Pts',(-89.4525415611931,-38.8019787427913,
117.26665400751));
#45544=CARTESIAN_POINT('Ctrl Pts',(-90.7381747913074,-36.2825568324379,
117.108705484318));
#45545=CARTESIAN_POINT('Ctrl Pts',(-89.3313446071879,-33.8287499130169,
116.950756961126));
#45546=CARTESIAN_POINT('Ctrl Pts',(-86.5075811499688,-33.6653500892044,
116.792808437933));
#45547=CARTESIAN_POINT('Ctrl Pts',(-84.8271048654275,-35.9405070116697,
116.634859914741));
#45548=CARTESIAN_POINT('Ctrl Pts',(-85.8135524913818,-38.5914050945837,
116.476911391548));
#45549=CARTESIAN_POINT('Ctrl Pts',(-88.5725419668272,-39.2145556695888,
116.318962868356));
#45550=CARTESIAN_POINT('Ctrl Pts',(-90.6025814452492,-37.244967062596,116.161014345163));
#45551=CARTESIAN_POINT('Ctrl Pts',(-90.0630958724223,-34.4684053612359,
116.003065821971));
#45552=CARTESIAN_POINT('Ctrl Pts',(-87.4432204095168,-33.4022946148249,
115.845117298778));
#45553=CARTESIAN_POINT('Ctrl Pts',(-85.1183164588386,-35.0132450128412,
115.687168775586));
#45554=CARTESIAN_POINT('Ctrl Pts',(-85.1963037237104,-37.8406568242449,
115.529220252393));
#45555=CARTESIAN_POINT('Ctrl Pts',(-87.6064735229483,-39.3210017514795,
115.371271729201));
#45556=CARTESIAN_POINT('Ctrl Pts',(-90.1635982015843,-38.1120960716771,
115.213323206008));
#45557=CARTESIAN_POINT('Ctrl Pts',(-90.5492105849305,-35.3100177975103,
115.055374682816));
#45558=CARTESIAN_POINT('Ctrl Pts',(-88.4136876528777,-33.4553260788078,
114.897426159623));
#45559=CARTESIAN_POINT('Ctrl Pts',(-85.6932430989239,-34.2296134890183,
114.739477636431));
#45560=CARTESIAN_POINT('Ctrl Pts',(-84.854421261558,-36.9308571821911,114.581529113239));
#45561=CARTESIAN_POINT('Ctrl Pts',(-86.6577563891068,-39.1099216563396,
114.423580590046));
#45562=CARTESIAN_POINT('Ctrl Pts',(-89.4682193673805,-38.7911154260036,
114.265632066854));
#45563=CARTESIAN_POINT('Ctrl Pts',(-90.7376488903457,-36.2634904041754,
114.107683543661));
#45564=CARTESIAN_POINT('Ctrl Pts',(-89.3150918174839,-33.8187673239068,
113.949735020469));
#45565=CARTESIAN_POINT('Ctrl Pts',(-86.490337381641,-33.6735022491857,113.791786497276));
#45566=CARTESIAN_POINT('Ctrl Pts',(-84.8245045187733,-35.9594026052244,
113.633837974084));
#45567=CARTESIAN_POINT('Ctrl Pts',(-85.8279532216264,-38.603912061719,113.475889450891));
#45568=CARTESIAN_POINT('Ctrl Pts',(-88.5908870698365,-39.2093343235855,
113.317940927699));
#45569=CARTESIAN_POINT('Ctrl Pts',(-90.6082379740656,-37.2267514390751,
113.159992404506));
#45570=CARTESIAN_POINT('Ctrl Pts',(-90.0509352244037,-34.4537110120408,
113.002043881314));
#45571=CARTESIAN_POINT('Ctrl Pts',(-87.4242682743722,-33.4044444594622,
112.844095358121));
#45572=CARTESIAN_POINT('Ctrl Pts',(-85.1097561611006,-35.030289852563,112.686146834929));
#45573=CARTESIAN_POINT('Ctrl Pts',(-85.2058966249883,-37.8571426212706,
112.528198311736));
#45574=CARTESIAN_POINT('Ctrl Pts',(-87.6255220314084,-39.3219813350391,
112.370249788544));
#45575=CARTESIAN_POINT('Ctrl Pts',(-90.1748316139398,-38.0966812831492,
112.212301265352));
#45576=CARTESIAN_POINT('Ctrl Pts',(-90.5424439078479,-35.2921847568347,
112.054352742159));
#45577=CARTESIAN_POINT('Ctrl Pts',(-88.3950560266678,-33.4512434615953,
111.896404218967));
#45578=CARTESIAN_POINT('Ctrl Pts',(-85.6796392524171,-34.2429828801331,
111.738455695774));
#45579=CARTESIAN_POINT('Ctrl Pts',(-84.8581793886376,-36.9495569613113,
111.580507172582));
#45580=CARTESIAN_POINT('Ctrl Pts',(-86.6754691102519,-39.116997302485,111.422558649389));
#45581=CARTESIAN_POINT('Ctrl Pts',(-89.483827097029,-38.780151665969,111.264610126197));
#45582=CARTESIAN_POINT('Ctrl Pts',(-90.7370005747289,-36.2444277458214,
111.106661603004));
#45583=CARTESIAN_POINT('Ctrl Pts',(-89.2987752646214,-33.8088892996237,
110.948713079812));
#45584=CARTESIAN_POINT('Ctrl Pts',(-86.473146313834,-33.6817649635238,110.790764556619));
#45585=CARTESIAN_POINT('Ctrl Pts',(-84.8220255542238,-35.9783145056534,
110.632816033427));
#45586=CARTESIAN_POINT('Ctrl Pts',(-85.8424339623762,-38.6163263048192,
110.474867510234));
#45587=CARTESIAN_POINT('Ctrl Pts',(-88.6091982680859,-39.2039952895745,
110.316918987042));
#45588=CARTESIAN_POINT('Ctrl Pts',(-90.613777424451,-37.2084998741394,110.158970463849));
#45589=CARTESIAN_POINT('Ctrl Pts',(-90.0386804733106,-34.439095041791,110.001021940657));
#45590=CARTESIAN_POINT('Ctrl Pts',(-87.4053303368919,-33.4067159667888,
109.843073417464));
#45591=CARTESIAN_POINT('Ctrl Pts',(-85.1013054789195,-35.0473892749383,
109.685124894272));
#45592=CARTESIAN_POINT('Ctrl Pts',(-85.215595195716,-37.8735665474884,109.52717637108));
#45593=CARTESIAN_POINT('Ctrl Pts',(-87.6445764125565,-39.3228384541829,
109.369227847887));
#45594=CARTESIAN_POINT('Ctrl Pts',(-90.1859658668476,-38.0811949578079,
109.211279324695));
#45595=CARTESIAN_POINT('Ctrl Pts',(-90.5355627605568,-35.2743949667504,
109.053330801502));
#45596=CARTESIAN_POINT('Ctrl Pts',(-88.3763987834983,-33.4472817259501,
108.89538227831));
#45597=CARTESIAN_POINT('Ctrl Pts',(-85.6661210922389,-34.2564369524755,
108.737433755117));
#45598=CARTESIAN_POINT('Ctrl Pts',(-84.8620584122606,-36.9682371464585,
108.579485231925));
#45599=CARTESIAN_POINT('Ctrl Pts',(-86.6932250423031,-39.1239489457093,
108.421536708732));
#45600=CARTESIAN_POINT('Ctrl Pts',(-89.4993679251268,-38.7691087355603,
108.26358818554));
#45601=CARTESIAN_POINT('Ctrl Pts',(-90.7362220179238,-36.225326822346,108.105639662347));
#45602=CARTESIAN_POINT('Ctrl Pts',(-89.2824117725574,-33.7992043149259,
107.947691139155));
#45603=CARTESIAN_POINT('Ctrl Pts',(-86.455975437068,-33.6899567687319,107.789742615962));
#45604=CARTESIAN_POINT('Ctrl Pts',(-84.8197363634497,-35.9976144787758,
107.63179409277));
#45605=CARTESIAN_POINT('Ctrl Pts',(-85.8568534149928,-38.627881180923,107.473845569577));
#45606=CARTESIAN_POINT('Ctrl Pts',(-88.6277564237406,-39.2001258219159,
107.315897046385));
#45607=CARTESIAN_POINT('Ctrl Pts',(-90.6185551090667,-37.1869579770143,
107.157948523193));
#45608=CARTESIAN_POINT('Ctrl Pts',(-90.2232169715586,-35.3519260775293,
107.052649507731));
#45609=CARTESIAN_POINT('Ctrl Pts',(-89.6820215852368,-34.718938871308,107.));
#45610=CARTESIAN_POINT('Ctrl Pts',(-90.2835504011883,-36.3531642868356,
121.112583302492));
#45611=CARTESIAN_POINT('Ctrl Pts',(-90.2854632662372,-36.0616114296406,
121.094195056371));
#45612=CARTESIAN_POINT('Ctrl Pts',(-90.2385919702165,-35.7706534224358,
121.07580681025));
#45613=CARTESIAN_POINT('Ctrl Pts',(-90.1402211051642,-35.4982975255724,
121.05741856413));
#45614=CARTESIAN_POINT('Ctrl Pts',(-89.8585641387499,-34.7184839531815,
121.004769056399));
#45615=CARTESIAN_POINT('Ctrl Pts',(-89.1547136083603,-34.0911705164269,
120.952119548668));
#45616=CARTESIAN_POINT('Ctrl Pts',(-88.3477629056644,-33.9007267159079,
120.899470040937));
#45617=CARTESIAN_POINT('Ctrl Pts',(-87.5408122029685,-33.7102829153889,
120.846820533206));
#45618=CARTESIAN_POINT('Ctrl Pts',(-86.6307613279662,-33.9567087511054,
120.794171025476));
#45619=CARTESIAN_POINT('Ctrl Pts',(-86.0301614626515,-34.5282973850589,
120.741521517745));
#45620=CARTESIAN_POINT('Ctrl Pts',(-85.4295615973368,-35.0998860190125,
120.688872010014));
#45621=CARTESIAN_POINT('Ctrl Pts',(-85.1384127417097,-35.9966374512031,
120.636222502283));
#45622=CARTESIAN_POINT('Ctrl Pts',(-85.2887059835297,-36.812019863374,120.583572994552));
#45623=CARTESIAN_POINT('Ctrl Pts',(-85.4389992253497,-37.6274022755449,
120.530923486821));
#45624=CARTESIAN_POINT('Ctrl Pts',(-86.0307345646168,-38.3614156676962,
120.478273979091));
#45625=CARTESIAN_POINT('Ctrl Pts',(-86.7956562367387,-38.6813077831314,
120.42562447136));
#45626=CARTESIAN_POINT('Ctrl Pts',(-87.5605779088606,-39.0011998985666,
120.372974963629));
#45627=CARTESIAN_POINT('Ctrl Pts',(-88.4986859138374,-38.9069707372859,
120.320325455898));
#45628=CARTESIAN_POINT('Ctrl Pts',(-89.1847040054158,-38.4413369016947,
120.267675948167));
#45629=CARTESIAN_POINT('Ctrl Pts',(-89.8583181592778,-37.9841222217589,
120.215978399609));
#45630=CARTESIAN_POINT('Ctrl Pts',(-90.288876093497,-37.1688122301997,120.16428085105));
#45631=CARTESIAN_POINT('Ctrl Pts',(-90.290141386937,-36.3546528235808,120.112583302492));
#45632=CARTESIAN_POINT('Ctrl Pts',(-88.5623548711056,-39.3241490284291,
122.));
#45633=CARTESIAN_POINT('Ctrl Pts',(-88.6554048794521,-39.2901109197242,
122.));
#45634=CARTESIAN_POINT('Ctrl Pts',(-88.7463897233141,-39.2513041051342,
122.));
#45635=CARTESIAN_POINT('Ctrl Pts',(-88.8351009182216,-39.2080569091679,
122.));
#45636=CARTESIAN_POINT('Ctrl Pts',(-88.9257790957573,-39.1638507983401,
122.));
#45637=CARTESIAN_POINT('Ctrl Pts',(-89.0140823477826,-39.1150045944796,
122.));
#45638=CARTESIAN_POINT('Ctrl Pts',(-89.0997590949921,-39.0618234076486,
122.));
#45639=CARTESIAN_POINT('Ctrl Pts',(-89.1821905332446,-39.010656645823,122.));
#45640=CARTESIAN_POINT('Ctrl Pts',(-89.2621909583464,-38.955476210875,122.));
#45641=CARTESIAN_POINT('Ctrl Pts',(-89.3395033436134,-38.8965237915301,
122.));
#45642=CARTESIAN_POINT('Ctrl Pts',(-89.4071516807222,-38.8449404246033,
122.));
#45643=CARTESIAN_POINT('Ctrl Pts',(-89.4727416970966,-38.7904684347609,
122.));
#45644=CARTESIAN_POINT('Ctrl Pts',(-89.5360765841124,-38.7332570353692,
122.));
#45645=CARTESIAN_POINT('Ctrl Pts',(-89.5502130714439,-38.7204873240644,
122.));
#45646=CARTESIAN_POINT('Ctrl Pts',(-89.564239852621,-38.7075784015462,122.));
#45647=CARTESIAN_POINT('Ctrl Pts',(-89.5781351542939,-38.6945504599679,
122.));
#45648=CARTESIAN_POINT('Ctrl Pts',(-89.6505652419802,-38.6266415384422,
122.));
#45649=CARTESIAN_POINT('Ctrl Pts',(-89.7195296422287,-38.5554106990788,
122.));
#45650=CARTESIAN_POINT('Ctrl Pts',(-89.7847884055803,-38.4811486670768,
122.));
#45651=CARTESIAN_POINT('Ctrl Pts',(-89.8496881543617,-38.4072951802285,
122.));
#45652=CARTESIAN_POINT('Ctrl Pts',(-89.9109234129235,-38.33044296365,122.));
#45653=CARTESIAN_POINT('Ctrl Pts',(-89.9682145606571,-38.2508512024992,
122.));
#45654=CARTESIAN_POINT('Ctrl Pts',(-90.0233774662291,-38.1742161030403,
122.));
#45655=CARTESIAN_POINT('Ctrl Pts',(-90.0748840116051,-38.0950404775979,
122.));
#45656=CARTESIAN_POINT('Ctrl Pts',(-90.1224397489187,-38.0135421014459,
122.));
#45657=CARTESIAN_POINT('Ctrl Pts',(-90.1423860806803,-37.9793591880777,
122.));
#45658=CARTESIAN_POINT('Ctrl Pts',(-90.1616368088772,-37.944767545073,122.));
#45659=CARTESIAN_POINT('Ctrl Pts',(-90.1801676233274,-37.9097829441458,
122.));
#45660=CARTESIAN_POINT('Ctrl Pts',(-90.1930501688088,-37.8854617944305,
122.));
#45661=CARTESIAN_POINT('Ctrl Pts',(-90.2055847495013,-37.8609507264995,
122.));
#45662=CARTESIAN_POINT('Ctrl Pts',(-90.2177627315331,-37.8362550336735,
122.));
#45663=CARTESIAN_POINT('Ctrl Pts',(-90.2256710650464,-37.8202177481283,
122.));
#45664=CARTESIAN_POINT('Ctrl Pts',(-90.2334301234711,-37.80409999056,122.));
#45665=CARTESIAN_POINT('Ctrl Pts',(-90.2410273664413,-37.787925400008,122.));
#45666=CARTESIAN_POINT('Ctrl Pts',(-90.283147662217,-37.6982509561637,122.));
#45667=CARTESIAN_POINT('Ctrl Pts',(-90.3203691262393,-37.6066929289713,
122.));
#45668=CARTESIAN_POINT('Ctrl Pts',(-90.3524004752756,-37.513523685623,122.));
#45669=CARTESIAN_POINT('Ctrl Pts',(-90.382280230974,-37.426612758871,122.));
#45670=CARTESIAN_POINT('Ctrl Pts',(-90.4076435357704,-37.3382990100201,
122.));
#45671=CARTESIAN_POINT('Ctrl Pts',(-90.4282034120715,-37.248794827624,122.));
#45672=CARTESIAN_POINT('Ctrl Pts',(-90.4296838958252,-37.2423497748434,
122.));
#45673=CARTESIAN_POINT('Ctrl Pts',(-90.4311394502785,-37.2358985482571,
122.));
#45674=CARTESIAN_POINT('Ctrl Pts',(-90.4325699576533,-37.229441226852,122.));
#45675=CARTESIAN_POINT('Ctrl Pts',(-90.4531761786108,-37.1364245853336,
122.));
#45676=CARTESIAN_POINT('Ctrl Pts',(-90.4685893763891,-37.0421422896564,
122.));
#45677=CARTESIAN_POINT('Ctrl Pts',(-90.4788864707506,-36.9470022043264,
122.));
#45678=CARTESIAN_POINT('Ctrl Pts',(-90.4846829926509,-36.8934451940809,
122.));
#45679=CARTESIAN_POINT('Ctrl Pts',(-90.4888573546745,-36.8396165495347,
122.));
#45680=CARTESIAN_POINT('Ctrl Pts',(-90.4914165163901,-36.7855916652876,
122.));
#45681=CARTESIAN_POINT('Ctrl Pts',(-90.4920773998915,-36.7716401613846,
122.));
#45682=CARTESIAN_POINT('Ctrl Pts',(-90.4926304468087,-36.7576761695281,
122.));
#45683=CARTESIAN_POINT('Ctrl Pts',(-90.4930755355952,-36.7437143575909,
122.));
#45684=CARTESIAN_POINT('Ctrl Pts',(-90.4960469521765,-36.6505051805635,
122.));
#45685=CARTESIAN_POINT('Ctrl Pts',(-90.4942192156142,-36.557237773971,122.));
#45686=CARTESIAN_POINT('Ctrl Pts',(-90.4877272199528,-36.4642872156905,
122.));
#45687=CARTESIAN_POINT('Ctrl Pts',(-90.4812244299425,-36.3711821069759,
122.));
#45688=CARTESIAN_POINT('Ctrl Pts',(-90.4700414792909,-36.2783939214527,
122.));
#45689=CARTESIAN_POINT('Ctrl Pts',(-90.4542630033313,-36.1863117068558,
122.));
#45690=CARTESIAN_POINT('Ctrl Pts',(-90.4387101222259,-36.0955460499439,
122.));
#45691=CARTESIAN_POINT('Ctrl Pts',(-90.4186917256712,-36.0054654767755,
122.));
#45692=CARTESIAN_POINT('Ctrl Pts',(-90.3942458454892,-35.9164677845401,
122.));
#45693=CARTESIAN_POINT('Ctrl Pts',(-90.3851470810519,-35.8833428149709,
122.));
#45694=CARTESIAN_POINT('Ctrl Pts',(-90.375434565641,-35.8503681770352,122.));
#45695=CARTESIAN_POINT('Ctrl Pts',(-90.3651088987993,-35.8175656480154,
122.));
#45696=CARTESIAN_POINT('Ctrl Pts',(-90.3581143447969,-35.7953453823259,
122.));
#45697=CARTESIAN_POINT('Ctrl Pts',(-90.3508384228978,-35.7732041064495,
122.));
#45698=CARTESIAN_POINT('Ctrl Pts',(-90.3432811403389,-35.7511488028356,
122.));
#45699=CARTESIAN_POINT('Ctrl Pts',(-90.338765074935,-35.7379690397597,122.));
#45700=CARTESIAN_POINT('Ctrl Pts',(-90.3341488817557,-35.724821150221,122.));
#45701=CARTESIAN_POINT('Ctrl Pts',(-90.3294360325543,-35.711715772054,122.));
#45702=CARTESIAN_POINT('Ctrl Pts',(-90.2978042850547,-35.6237549663183,
122.));
#45703=CARTESIAN_POINT('Ctrl Pts',(-90.261783323813,-35.5375919066344,122.));
#45704=CARTESIAN_POINT('Ctrl Pts',(-90.2214377122488,-35.4536408345172,
122.));
#45705=CARTESIAN_POINT('Ctrl Pts',(-90.1911785035756,-35.3906775304294,
122.));
#45706=CARTESIAN_POINT('Ctrl Pts',(-90.1584856317728,-35.3289589612895,
122.));
#45707=CARTESIAN_POINT('Ctrl Pts',(-90.1233703727677,-35.2686754163207,
122.));
#45708=CARTESIAN_POINT('Ctrl Pts',(-90.1099009754952,-35.2455520494658,
122.));
#45709=CARTESIAN_POINT('Ctrl Pts',(-90.0960750361369,-35.2226399806261,
122.));
#45710=CARTESIAN_POINT('Ctrl Pts',(-90.0818927106299,-35.1999505929771,
122.));
#45711=CARTESIAN_POINT('Ctrl Pts',(-90.0717686114082,-35.1837536997579,
122.));
#45712=CARTESIAN_POINT('Ctrl Pts',(-90.0614620660595,-35.1676692161304,
122.));
#45713=CARTESIAN_POINT('Ctrl Pts',(-90.0509832059227,-35.1517162866814,
122.));
#45714=CARTESIAN_POINT('Ctrl Pts',(-90.0037966280057,-35.0798798332293,
122.));
#45715=CARTESIAN_POINT('Ctrl Pts',(-89.9530751222339,-35.0106368288827,
122.));
#45716=CARTESIAN_POINT('Ctrl Pts',(-89.8988515797855,-34.9443392719291,
122.));
#45717=CARTESIAN_POINT('Ctrl Pts',(-89.850055152577,-34.8846772918016,122.));
#45718=CARTESIAN_POINT('Ctrl Pts',(-89.7984220271467,-34.8274007372017,
122.));
#45719=CARTESIAN_POINT('Ctrl Pts',(-89.7439556820556,-34.7727959467699,
122.));
#45720=CARTESIAN_POINT('Ctrl Pts',(-89.7248731118213,-34.7536648714829,
122.));
#45721=CARTESIAN_POINT('Ctrl Pts',(-89.7054425965606,-34.7348620441323,
122.));
#45722=CARTESIAN_POINT('Ctrl Pts',(-89.6856747112033,-34.7163919521557,
122.));
#45723=CARTESIAN_POINT('Origin',(-87.7685555885722,-36.3549260746835,114.));
#45724=CARTESIAN_POINT('Origin',(-36.3549260746835,-87.7685555885722,107.));
#45725=CARTESIAN_POINT('Ctrl Pts',(-38.2683920713481,-86.1325683851967,
107.));
#45726=CARTESIAN_POINT('Ctrl Pts',(-38.3305295883356,-86.1909623931506,
107.));
#45727=CARTESIAN_POINT('Ctrl Pts',(-38.3892917294532,-86.2526103113827,
107.));
#45728=CARTESIAN_POINT('Ctrl Pts',(-38.4446665159936,-86.3171356636189,
107.));
#45729=CARTESIAN_POINT('Ctrl Pts',(-38.5013963845958,-86.3832400223452,
107.));
#45730=CARTESIAN_POINT('Ctrl Pts',(-38.5545715537976,-86.4523648572664,
107.));
#45731=CARTESIAN_POINT('Ctrl Pts',(-38.6041502559258,-86.524151647146,107.));
#45732=CARTESIAN_POINT('Ctrl Pts',(-38.6170879438391,-86.5428845918156,
107.));
#45733=CARTESIAN_POINT('Ctrl Pts',(-38.6297805550942,-86.5617990222241,
107.));
#45734=CARTESIAN_POINT('Ctrl Pts',(-38.6422269720562,-86.5808890006484,
107.));
#45735=CARTESIAN_POINT('Ctrl Pts',(-38.6523970248712,-86.59648755318,107.));
#45736=CARTESIAN_POINT('Ctrl Pts',(-38.6624031432674,-86.6122042204815,
107.));
#45737=CARTESIAN_POINT('Ctrl Pts',(-38.6722358693769,-86.6280211675642,
107.));
#45738=CARTESIAN_POINT('Ctrl Pts',(-38.7196799641235,-86.7043398535153,
107.));
#45739=CARTESIAN_POINT('Ctrl Pts',(-38.7631404947387,-86.7830659002748,
107.));
#45740=CARTESIAN_POINT('Ctrl Pts',(-38.8025827758839,-86.863806756021,107.));
#45741=CARTESIAN_POINT('Ctrl Pts',(-38.8344112328972,-86.9289616299717,
107.));
#45742=CARTESIAN_POINT('Ctrl Pts',(-38.8636225491245,-86.9954296141671,
107.));
#45743=CARTESIAN_POINT('Ctrl Pts',(-38.8901813394751,-87.0630222348955,
107.));
#45744=CARTESIAN_POINT('Ctrl Pts',(-38.9007827444047,-87.0900030097402,
107.));
#45745=CARTESIAN_POINT('Ctrl Pts',(-38.9109613265359,-87.1171631300883,
107.));
#45746=CARTESIAN_POINT('Ctrl Pts',(-38.920714074785,-87.1444911545565,107.));
#45747=CARTESIAN_POINT('Ctrl Pts',(-38.9259550311851,-87.1591767571254,
107.));
#45748=CARTESIAN_POINT('Ctrl Pts',(-38.9310726354609,-87.1739100289027,
107.));
#45749=CARTESIAN_POINT('Ctrl Pts',(-38.9360624206009,-87.1886767156748,
107.));
#45750=CARTESIAN_POINT('Ctrl Pts',(-38.9656012135239,-87.2760933259059,
107.));
#45751=CARTESIAN_POINT('Ctrl Pts',(-38.9907045453902,-87.3647910403201,
107.));
#45752=CARTESIAN_POINT('Ctrl Pts',(-39.0113398488637,-87.4543720487631,
107.));
#45753=CARTESIAN_POINT('Ctrl Pts',(-39.0322966239254,-87.5453486145384,
107.));
#45754=CARTESIAN_POINT('Ctrl Pts',(-39.04864557461,-87.6372370153347,107.));
#45755=CARTESIAN_POINT('Ctrl Pts',(-39.0603107625964,-87.7296537434723,
107.));
#45756=CARTESIAN_POINT('Ctrl Pts',(-39.0718852370958,-87.8213517996373,
107.));
#45757=CARTESIAN_POINT('Ctrl Pts',(-39.0788488557146,-87.9135709280502,
107.));
#45758=CARTESIAN_POINT('Ctrl Pts',(-39.0810804934318,-88.0059557086637,
107.));
#45759=CARTESIAN_POINT('Ctrl Pts',(-39.0821911128068,-88.0519328520486,
107.));
#45760=CARTESIAN_POINT('Ctrl Pts',(-39.0821289726537,-88.0979512365569,
107.));
#45761=CARTESIAN_POINT('Ctrl Pts',(-39.0808743448802,-88.1439677515796,
107.));
#45762=CARTESIAN_POINT('Ctrl Pts',(-39.0805045717962,-88.1575300758302,
107.));
#45763=CARTESIAN_POINT('Ctrl Pts',(-39.0800311920668,-88.1710922383706,
107.));
#45764=CARTESIAN_POINT('Ctrl Pts',(-39.0794536442604,-88.1846531355265,
107.));
#45765=CARTESIAN_POINT('Ctrl Pts',(-39.0788331294174,-88.1992229042558,
107.));
#45766=CARTESIAN_POINT('Ctrl Pts',(-39.0780927731541,-88.2137814265114,
107.));
#45767=CARTESIAN_POINT('Ctrl Pts',(-39.0772325270316,-88.2283247728338,
107.));
#45768=CARTESIAN_POINT('Ctrl Pts',(-39.0715807131733,-88.3238745046424,
107.));
#45769=CARTESIAN_POINT('Ctrl Pts',(-39.0607562655325,-88.4188025145338,
107.));
#45770=CARTESIAN_POINT('Ctrl Pts',(-39.0446887301443,-88.5127131576963,
107.));
#45771=CARTESIAN_POINT('Ctrl Pts',(-39.0423083893799,-88.5266256418905,
107.));
#45772=CARTESIAN_POINT('Ctrl Pts',(-39.0398128903088,-88.5405158311432,
107.));
#45773=CARTESIAN_POINT('Ctrl Pts',(-39.0372019113363,-88.5543824697525,
107.));
#45774=CARTESIAN_POINT('Ctrl Pts',(-39.020256250766,-88.6443791160708,107.));
#45775=CARTESIAN_POINT('Ctrl Pts',(-38.9984507099304,-88.733383584132,107.));
#45776=CARTESIAN_POINT('Ctrl Pts',(-38.972087837954,-88.821163626335,107.));
#45777=CARTESIAN_POINT('Ctrl Pts',(-38.9451290233172,-88.9109279694868,
107.));
#45778=CARTESIAN_POINT('Ctrl Pts',(-38.9134042991795,-88.9994126041051,
107.));
#45779=CARTESIAN_POINT('Ctrl Pts',(-38.8771829581873,-89.0863654860054,
107.));
#45780=CARTESIAN_POINT('Ctrl Pts',(-38.864692810473,-89.1163493107169,107.));
#45781=CARTESIAN_POINT('Ctrl Pts',(-38.8516675352072,-89.1461509187054,
107.));
#45782=CARTESIAN_POINT('Ctrl Pts',(-38.8381168020892,-89.1757596360031,
107.));
#45783=CARTESIAN_POINT('Ctrl Pts',(-38.8314257154722,-89.1903798407058,
107.));
#45784=CARTESIAN_POINT('Ctrl Pts',(-38.824606501858,-89.2049530114955,107.));
#45785=CARTESIAN_POINT('Ctrl Pts',(-38.8176602661698,-89.2194778407777,
107.));
#45786=CARTESIAN_POINT('Ctrl Pts',(-38.8121664927493,-89.2309655190869,
107.));
#45787=CARTESIAN_POINT('Ctrl Pts',(-38.8065937046077,-89.2424219334059,
107.));
#45788=CARTESIAN_POINT('Ctrl Pts',(-38.8009470423584,-89.253837507682,107.));
#45789=CARTESIAN_POINT('Ctrl Pts',(-38.7582230887587,-89.3402103849944,
107.));
#45790=CARTESIAN_POINT('Ctrl Pts',(-38.7112082785351,-89.4243849391538,
107.));
#45791=CARTESIAN_POINT('Ctrl Pts',(-38.660245266337,-89.5061115333766,107.));
#45792=CARTESIAN_POINT('Ctrl Pts',(-38.6082715482375,-89.5894589413528,
107.));
#45793=CARTESIAN_POINT('Ctrl Pts',(-38.5521911589312,-89.670261101487,107.));
#45794=CARTESIAN_POINT('Ctrl Pts',(-38.4923125369602,-89.7482461987396,
107.));
#45795=CARTESIAN_POINT('Ctrl Pts',(-38.431947090932,-89.8268653289775,107.));
#45796=CARTESIAN_POINT('Ctrl Pts',(-38.3677209417352,-89.9026222404123,
107.));
#45797=CARTESIAN_POINT('Ctrl Pts',(-38.2999007811538,-89.9752191546411,
107.));
#45798=CARTESIAN_POINT('Ctrl Pts',(-38.2629001291875,-90.0148258605848,
107.));
#45799=CARTESIAN_POINT('Ctrl Pts',(-38.2248289148845,-90.0534915954115,
107.));
#45800=CARTESIAN_POINT('Ctrl Pts',(-38.1857250970592,-90.0911642251884,
107.));
#45801=CARTESIAN_POINT('Ctrl Pts',(-38.1737573203776,-90.1026939848193,
107.));
#45802=CARTESIAN_POINT('Ctrl Pts',(-38.1616927978678,-90.1141307004969,
107.));
#45803=CARTESIAN_POINT('Ctrl Pts',(-38.1495325546806,-90.1254728156509,
107.));
#45804=CARTESIAN_POINT('Ctrl Pts',(-38.1389867814773,-90.1353090806185,
107.));
#45805=CARTESIAN_POINT('Ctrl Pts',(-38.1283701312735,-90.1450730796272,
107.));
#45806=CARTESIAN_POINT('Ctrl Pts',(-38.1176923840407,-90.1547558196661,
107.));
#45807=CARTESIAN_POINT('Ctrl Pts',(-38.0421178908384,-90.2232878943906,
107.));
#45808=CARTESIAN_POINT('Ctrl Pts',(-37.9633666783311,-90.2878636215937,
107.));
#45809=CARTESIAN_POINT('Ctrl Pts',(-37.881766092165,-90.3482012299876,107.));
#45810=CARTESIAN_POINT('Ctrl Pts',(-37.8000613244985,-90.4086158729087,
107.));
#45811=CARTESIAN_POINT('Ctrl Pts',(-37.7154993294117,-90.4647824068464,
107.));
#45812=CARTESIAN_POINT('Ctrl Pts',(-37.6283634335479,-90.516392179797,107.));
#45813=CARTESIAN_POINT('Ctrl Pts',(-37.5429597747808,-90.5669759649802,
107.));
#45814=CARTESIAN_POINT('Ctrl Pts',(-37.4550828708226,-90.6131830404371,
107.));
#45815=CARTESIAN_POINT('Ctrl Pts',(-37.364965395232,-90.6546869942762,107.));
#45816=CARTESIAN_POINT('Ctrl Pts',(-37.3246165101986,-90.6732698301902,
107.));
#45817=CARTESIAN_POINT('Ctrl Pts',(-37.2838180606497,-90.6909092957975,
107.));
#45818=CARTESIAN_POINT('Ctrl Pts',(-37.242589176951,-90.7075731462259,107.));
#45819=CARTESIAN_POINT('Ctrl Pts',(-37.2121695381052,-90.7198681265004,
107.));
#45820=CARTESIAN_POINT('Ctrl Pts',(-37.1815155543152,-90.7316319541871,
107.));
#45821=CARTESIAN_POINT('Ctrl Pts',(-37.1506394945611,-90.7428673099699,
107.));
#45822=CARTESIAN_POINT('Ctrl Pts',(-35.5611267921512,-90.7377785423181,
107.));
#45823=CARTESIAN_POINT('Ctrl Pts',(-35.4662928857449,-90.7030878757344,
107.));
#45824=CARTESIAN_POINT('Ctrl Pts',(-35.3735021330788,-90.6634063262115,
107.));
#45825=CARTESIAN_POINT('Ctrl Pts',(-35.2829954573582,-90.6190542441227,
107.));
#45826=CARTESIAN_POINT('Ctrl Pts',(-35.1912159031789,-90.5740783979917,
107.));
#45827=CARTESIAN_POINT('Ctrl Pts',(-35.1017844554001,-90.5242990217277,
107.));
#45828=CARTESIAN_POINT('Ctrl Pts',(-35.014986370264,-90.4700094899543,107.));
#45829=CARTESIAN_POINT('Ctrl Pts',(-34.9904733516654,-90.4546773510023,
107.));
#45830=CARTESIAN_POINT('Ctrl Pts',(-34.9661706042967,-90.4389852821517,
107.));
#45831=CARTESIAN_POINT('Ctrl Pts',(-34.9420851497754,-90.42293943585,107.));
#45832=CARTESIAN_POINT('Ctrl Pts',(-34.9227556040072,-90.4100619989637,
107.));
#45833=CARTESIAN_POINT('Ctrl Pts',(-34.9035639060071,-90.39695507833,107.));
#45834=CARTESIAN_POINT('Ctrl Pts',(-34.8845329713075,-90.3836356190119,
107.));
#45835=CARTESIAN_POINT('Ctrl Pts',(-34.8018258702773,-90.325750187483,107.));
#45836=CARTESIAN_POINT('Ctrl Pts',(-34.7220736288122,-90.2638026101735,
107.));
#45837=CARTESIAN_POINT('Ctrl Pts',(-34.6455426085499,-90.1980902479038,
107.));
#45838=CARTESIAN_POINT('Ctrl Pts',(-34.5865494182568,-90.147436514572,107.));
#45839=CARTESIAN_POINT('Ctrl Pts',(-34.5294708955044,-90.094544854916,107.));
#45840=CARTESIAN_POINT('Ctrl Pts',(-34.4744466082576,-90.0395396993188,
107.));
#45841=CARTESIAN_POINT('Ctrl Pts',(-34.4451578629574,-90.0102611375584,
107.));
#45842=CARTESIAN_POINT('Ctrl Pts',(-34.4164514207639,-89.9803836100269,
107.));
#45843=CARTESIAN_POINT('Ctrl Pts',(-34.3883503519563,-89.949925051172,107.));
#45844=CARTESIAN_POINT('Ctrl Pts',(-34.3787143478639,-89.9394806513599,
107.));
#45845=CARTESIAN_POINT('Ctrl Pts',(-34.3691502594248,-89.9289686396398,
107.));
#45846=CARTESIAN_POINT('Ctrl Pts',(-34.3596656532768,-89.9183973517283,
107.));
#45847=CARTESIAN_POINT('Ctrl Pts',(-34.2938684614213,-89.8450615644514,
107.));
#45848=CARTESIAN_POINT('Ctrl Pts',(-34.2318034199732,-89.7687791536545,
107.));
#45849=CARTESIAN_POINT('Ctrl Pts',(-34.1737142975659,-89.6898286775609,
107.));
#45850=CARTESIAN_POINT('Ctrl Pts',(-34.1161516327794,-89.6115937240657,
107.));
#45851=CARTESIAN_POINT('Ctrl Pts',(-34.0624927127841,-89.5307380625027,
107.));
#45852=CARTESIAN_POINT('Ctrl Pts',(-34.0130204815364,-89.447510360224,107.));
#45853=CARTESIAN_POINT('Ctrl Pts',(-33.9649625424885,-89.366661937941,107.));
#45854=CARTESIAN_POINT('Ctrl Pts',(-33.9208551306922,-89.283574459218,107.));
#45855=CARTESIAN_POINT('Ctrl Pts',(-33.8810053974435,-89.1984655452966,
107.));
#45856=CARTESIAN_POINT('Ctrl Pts',(-33.8602009805094,-89.1540325921578,
107.));
#45857=CARTESIAN_POINT('Ctrl Pts',(-33.8405578495624,-89.1090485695462,
107.));
#45858=CARTESIAN_POINT('Ctrl Pts',(-33.8221254047308,-89.0635442081576,
107.));
#45859=CARTESIAN_POINT('Ctrl Pts',(-33.815067321247,-89.0461198466857,107.));
#45860=CARTESIAN_POINT('Ctrl Pts',(-33.8081867972032,-89.0286191918009,
107.));
#45861=CARTESIAN_POINT('Ctrl Pts',(-33.8014867681844,-89.0110439776197,
107.));
#45862=CARTESIAN_POINT('Ctrl Pts',(-33.7962450333404,-88.9972940949988,
107.));
#45863=CARTESIAN_POINT('Ctrl Pts',(-33.7911136745704,-88.9834980764818,
107.));
#45864=CARTESIAN_POINT('Ctrl Pts',(-33.7860992270484,-88.9696714653787,
107.));
#45865=CARTESIAN_POINT('Ctrl Pts',(-33.7544155410359,-88.8823083006666,
107.));
#45866=CARTESIAN_POINT('Ctrl Pts',(-33.7273406805785,-88.7935841918564,
107.));
#45867=CARTESIAN_POINT('Ctrl Pts',(-33.7051259018102,-88.7037226902072,
107.));
#45868=CARTESIAN_POINT('Ctrl Pts',(-33.7001419285477,-88.6835619077742,
107.));
#45869=CARTESIAN_POINT('Ctrl Pts',(-33.6954027892081,-88.6633438353985,
107.));
#45870=CARTESIAN_POINT('Ctrl Pts',(-33.6909116819337,-88.6430709420454,
107.));
#45871=CARTESIAN_POINT('Ctrl Pts',(-33.6705459299635,-88.5511397784083,
107.));
#45872=CARTESIAN_POINT('Ctrl Pts',(-33.6552763905805,-88.4580809934608,
107.));
#45873=CARTESIAN_POINT('Ctrl Pts',(-33.6449932387159,-88.3642861744627,
107.));
#45874=CARTESIAN_POINT('Ctrl Pts',(-33.6342593787364,-88.2663803507243,
107.));
#45875=CARTESIAN_POINT('Ctrl Pts',(-33.6289586023237,-88.1676713209843,
107.));
#45876=CARTESIAN_POINT('Ctrl Pts',(-33.6290234622339,-88.0686191026489,
107.));
#45877=CARTESIAN_POINT('Ctrl Pts',(-33.6290488323814,-88.0298745317877,
107.));
#45878=CARTESIAN_POINT('Ctrl Pts',(-33.6298957475537,-87.9910777096528,
107.));
#45879=CARTESIAN_POINT('Ctrl Pts',(-33.6315623951404,-87.9522573940279,
107.));
#45880=CARTESIAN_POINT('Ctrl Pts',(-33.6320954345873,-87.9398415961512,
107.));
#45881=CARTESIAN_POINT('Ctrl Pts',(-33.6327123205129,-87.9274247064713,
107.));
#45882=CARTESIAN_POINT('Ctrl Pts',(-33.6334122917911,-87.9150173343413,
107.));
#45883=CARTESIAN_POINT('Ctrl Pts',(-33.6386515097086,-87.8221493433258,
107.));
#45884=CARTESIAN_POINT('Ctrl Pts',(-33.6485471485414,-87.729664583953,107.));
#45885=CARTESIAN_POINT('Ctrl Pts',(-33.6629757491884,-87.6379346339504,
107.));
#45886=CARTESIAN_POINT('Ctrl Pts',(-33.6773703612078,-87.5464207669331,
107.));
#45887=CARTESIAN_POINT('Ctrl Pts',(-33.6962770140278,-87.4556572120266,
107.));
#45888=CARTESIAN_POINT('Ctrl Pts',(-33.7196217950054,-87.3660298796492,
107.));
#45889=CARTESIAN_POINT('Ctrl Pts',(-33.74257042567,-87.2779234823281,107.));
#45890=CARTESIAN_POINT('Ctrl Pts',(-33.7698083039621,-87.1909142870507,
107.));
#45891=CARTESIAN_POINT('Ctrl Pts',(-33.8013056575605,-87.1053979868551,
107.));
#45892=CARTESIAN_POINT('Ctrl Pts',(-33.8171471021691,-87.0623879692535,
107.));
#45893=CARTESIAN_POINT('Ctrl Pts',(-33.834066596719,-87.0197561200163,107.));
#45894=CARTESIAN_POINT('Ctrl Pts',(-33.8520637709505,-86.9775565705104,
107.));
#45895=CARTESIAN_POINT('Ctrl Pts',(-33.8576294774237,-86.9645061714404,
107.));
#45896=CARTESIAN_POINT('Ctrl Pts',(-33.8632982668804,-86.9514971375181,
107.));
#45897=CARTESIAN_POINT('Ctrl Pts',(-33.8690701692463,-86.9385311273666,
107.));
#45898=CARTESIAN_POINT('Ctrl Pts',(-33.8747496330137,-86.9257727714217,
107.));
#45899=CARTESIAN_POINT('Ctrl Pts',(-33.8805254520977,-86.9130639366889,
107.));
#45900=CARTESIAN_POINT('Ctrl Pts',(-33.8863958367835,-86.9004091087509,
107.));
#45901=CARTESIAN_POINT('Ctrl Pts',(-33.9238756397803,-86.8196136441493,
107.));
#45902=CARTESIAN_POINT('Ctrl Pts',(-33.9652255993582,-86.7409749585095,
107.));
#45903=CARTESIAN_POINT('Ctrl Pts',(-34.0103760392298,-86.6648406433426,
107.));
#45904=CARTESIAN_POINT('Ctrl Pts',(-34.0547690445968,-86.5899835418078,
107.));
#45905=CARTESIAN_POINT('Ctrl Pts',(-34.1028365417562,-86.5175468204594,
107.));
#45906=CARTESIAN_POINT('Ctrl Pts',(-34.1545485155578,-86.4478950466225,
107.));
#45907=CARTESIAN_POINT('Ctrl Pts',(-34.2046829695647,-86.3803680621503,
107.));
#45908=CARTESIAN_POINT('Ctrl Pts',(-34.2582433786248,-86.315458261135,107.));
#45909=CARTESIAN_POINT('Ctrl Pts',(-34.3152301022523,-86.2535381385478,
107.));
#45910=CARTESIAN_POINT('Ctrl Pts',(-34.3361976980218,-86.2307553565634,
107.));
#45911=CARTESIAN_POINT('Ctrl Pts',(-34.3576293877451,-86.2083777473769,
107.));
#45912=CARTESIAN_POINT('Ctrl Pts',(-34.3795260005218,-86.1864254754535,
107.));
#45913=CARTESIAN_POINT('Ctrl Pts',(-34.3986034365815,-86.1672995463313,
107.));
#45914=CARTESIAN_POINT('Ctrl Pts',(-34.4180338060146,-86.1484965041123,
107.));
#45915=CARTESIAN_POINT('Ctrl Pts',(-34.437806971968,-86.1300214773104,107.));
#45916=CARTESIAN_POINT('Origin',(-36.3549260746835,-87.7685555885722,124.208423447177));
#45917=CARTESIAN_POINT('Ctrl Pts',(-39.4317256223809,-87.7666280037969,
121.708423447177));
#45918=CARTESIAN_POINT('Ctrl Pts',(-39.4326483047755,-87.6433531015923,
121.702019850418));
#45919=CARTESIAN_POINT('Ctrl Pts',(-39.3701218467006,-86.5074462896477,
121.642966745928));
#45920=CARTESIAN_POINT('Ctrl Pts',(-37.9573948034252,-84.5150171095306,
121.531264133707));
#45921=CARTESIAN_POINT('Ctrl Pts',(-34.5067286900242,-84.648392448822,121.373315610515));
#45922=CARTESIAN_POINT('Ctrl Pts',(-32.7318386198642,-87.6103338151322,
121.215367087322));
#45923=CARTESIAN_POINT('Ctrl Pts',(-34.2418568983793,-90.7159201684501,
121.05741856413));
#45924=CARTESIAN_POINT('Ctrl Pts',(-37.6677476810076,-91.149128255265,120.899470040937));
#45925=CARTESIAN_POINT('Ctrl Pts',(-39.3142946536224,-89.2107570149594,
120.783138335286));
#45926=CARTESIAN_POINT('Ctrl Pts',(-39.4311722823457,-87.984115255456,120.719456137367));
#45927=CARTESIAN_POINT('Ctrl Pts',(-39.4292404520863,-87.7712393069318,
120.708423447177));
#45928=CARTESIAN_POINT('Ctrl Pts',(-39.4252046443693,-87.771569957437,121.791576552823));
#45929=CARTESIAN_POINT('Ctrl Pts',(-39.4202197512721,-87.0785516532724,
121.755752019753));
#45930=CARTESIAN_POINT('Ctrl Pts',(-38.847832523077,-85.3573626625651,121.667277978953));
#45931=CARTESIAN_POINT('Ctrl Pts',(-36.0033916957587,-84.1596937777799,
121.526154430423));
#45932=CARTESIAN_POINT('Ctrl Pts',(-33.1409988246472,-86.0888162082167,
121.36820590723));
#45933=CARTESIAN_POINT('Ctrl Pts',(-33.1913892046506,-89.5420981815712,
121.210257384038));
#45934=CARTESIAN_POINT('Ctrl Pts',(-36.1106392225623,-91.3867838745725,
121.052308860845));
#45935=CARTESIAN_POINT('Ctrl Pts',(-38.8854865669341,-90.1183415880482,
120.912748583774));
#45936=CARTESIAN_POINT('Ctrl Pts',(-39.4210163858766,-88.4296040393632,
120.825837814433));
#45937=CARTESIAN_POINT('Ctrl Pts',(-39.4253676065904,-87.7664047027925,
120.791576552823));
#45938=CARTESIAN_POINT('Ctrl Pts',(-34.4414600780185,-86.1325683851972,
122.));
#45939=CARTESIAN_POINT('Ctrl Pts',(-33.9002646916969,-86.7655555914187,
121.947350492269));
#45940=CARTESIAN_POINT('Ctrl Pts',(-33.5049263244719,-88.6005872421791,
121.842051476808));
#45941=CARTESIAN_POINT('Ctrl Pts',(-35.495725323147,-90.613755383703,121.684102953615));
#45942=CARTESIAN_POINT('Ctrl Pts',(-38.2666281885584,-90.0415106136082,
121.526154430423));
#45943=CARTESIAN_POINT('Ctrl Pts',(-39.3037452815429,-87.4112440285999,
121.36820590723));
#45944=CARTESIAN_POINT('Ctrl Pts',(-37.6675062030737,-85.1035862959133,
121.210257384038));
#45945=CARTESIAN_POINT('Ctrl Pts',(-34.8410699120416,-85.2128338692552,
121.052308860845));
#45946=CARTESIAN_POINT('Ctrl Pts',(-33.3872596788782,-87.6389563321429,
120.894360337653));
#45947=CARTESIAN_POINT('Ctrl Pts',(-34.6241137592953,-90.182738223953,120.73641181446));
#45948=CARTESIAN_POINT('Ctrl Pts',(-37.430256607926,-90.5375784252076,120.578463291268));
#45949=CARTESIAN_POINT('Ctrl Pts',(-39.2614232167573,-88.3818666539668,
120.420514768075));
#45950=CARTESIAN_POINT('Ctrl Pts',(-38.4573605460916,-85.6700664907204,
120.262566244883));
#45951=CARTESIAN_POINT('Ctrl Pts',(-35.7470828869712,-84.8609112744695,
120.10461772169));
#45952=CARTESIAN_POINT('Ctrl Pts',(-33.5879189354126,-86.6880244932926,
119.946669198498));
#45953=CARTESIAN_POINT('Ctrl Pts',(-33.9375158250034,-89.4948244513467,
119.788720675305));
#45954=CARTESIAN_POINT('Ctrl Pts',(-36.4789052492319,-90.7364679329367,
119.630772152113));
#45955=CARTESIAN_POINT('Ctrl Pts',(-38.9078864373474,-89.2871960434334,
119.472823628921));
#45956=CARTESIAN_POINT('Ctrl Pts',(-39.0221761527905,-86.4610188042813,
119.314875105728));
#45957=CARTESIAN_POINT('Ctrl Pts',(-36.7181513220674,-84.82034551555,119.156926582536));
#45958=CARTESIAN_POINT('Ctrl Pts',(-34.0848012167929,-85.8527245783361,
118.998978059343));
#45959=CARTESIAN_POINT('Ctrl Pts',(-33.5097042724549,-88.6221293779351,
118.841029536151));
#45960=CARTESIAN_POINT('Ctrl Pts',(-35.5142834051126,-90.6176247697674,
118.683081012958));
#45961=CARTESIAN_POINT('Ctrl Pts',(-38.2810476781003,-90.0299557919626,
118.525132489766));
#45962=CARTESIAN_POINT('Ctrl Pts',(-39.3014560741837,-87.3919440239953,
118.367183966573));
#45963=CARTESIAN_POINT('Ctrl Pts',(-37.6503353341005,-85.0953945090273,
118.209235443381));
#45964=CARTESIAN_POINT('Ctrl Pts',(-34.8247064167312,-85.2225188436243,
118.051286920188));
#45965=CARTESIAN_POINT('Ctrl Pts',(-33.3864811236342,-87.6580572610179,
117.893338396996));
#45966=CARTESIAN_POINT('Ctrl Pts',(-34.6396545865135,-90.1937811511754,
117.735389873803));
#45967=CARTESIAN_POINT('Ctrl Pts',(-37.4480125400769,-90.530626783707,117.577441350611));
#45968=CARTESIAN_POINT('Ctrl Pts',(-39.2653022401977,-88.3631864681666,
117.419492827418));
#45969=CARTESIAN_POINT('Ctrl Pts',(-38.443842386133,-85.6566124189988,117.261544304226));
#45970=CARTESIAN_POINT('Ctrl Pts',(-35.7284256439965,-84.8648730098256,
117.103595781034));
#45971=CARTESIAN_POINT('Ctrl Pts',(-33.5810377882138,-86.7058142832929,
116.945647257841));
#45972=CARTESIAN_POINT('Ctrl Pts',(-33.9486500777749,-89.5103107764393,
116.787698734649));
#45973=CARTESIAN_POINT('Ctrl Pts',(-36.4979596301566,-90.7356108138369,
116.629750211456));
#45974=CARTESIAN_POINT('Ctrl Pts',(-38.9175850079598,-89.2707721173922,
116.471801688264));
#45975=CARTESIAN_POINT('Ctrl Pts',(-39.0137254707097,-86.4439193821171,
116.313853165071));
#45976=CARTESIAN_POINT('Ctrl Pts',(-36.6992133848109,-84.8180740082457,
116.155904641879));
#45977=CARTESIAN_POINT('Ctrl Pts',(-34.0725464658448,-85.8673405484154,
115.997956118686));
#45978=CARTESIAN_POINT('Ctrl Pts',(-33.5152437227748,-88.6403809426538,
115.840007595494));
#45979=CARTESIAN_POINT('Ctrl Pts',(-35.5325946031457,-90.6229638037158,
115.682059072301));
#45980=CARTESIAN_POINT('Ctrl Pts',(-38.2955284186788,-90.0175415490088,
115.524110549109));
#45981=CARTESIAN_POINT('Ctrl Pts',(-39.2989771096636,-87.37303212379,115.366162025916));
#45982=CARTESIAN_POINT('Ctrl Pts',(-37.6331442664967,-85.0871317947868,
115.208213502724));
#45983=CARTESIAN_POINT('Ctrl Pts',(-34.8083898640617,-85.2323968677906,
115.050264979531));
#45984=CARTESIAN_POINT('Ctrl Pts',(-33.3858328080249,-87.6771199191464,
114.892316456339));
#45985=CARTESIAN_POINT('Ctrl Pts',(-34.6552623159776,-90.2047449110804,
114.734367933147));
#45986=CARTESIAN_POINT('Ctrl Pts',(-37.4657252610125,-90.5235511376453,
114.576419409954));
#45987=CARTESIAN_POINT('Ctrl Pts',(-39.269060367233,-88.3444866892675,114.418470886762));
#45988=CARTESIAN_POINT('Ctrl Pts',(-38.430238539787,-85.6432430280421,114.260522363569));
#45989=CARTESIAN_POINT('Ctrl Pts',(-35.7097940180071,-84.8689556269897,
114.102573840377));
#45990=CARTESIAN_POINT('Ctrl Pts',(-33.5742711112112,-86.7236473237577,
113.944625317184));
#45991=CARTESIAN_POINT('Ctrl Pts',(-33.9598834899978,-89.5257255647848,
113.786676793992));
#45992=CARTESIAN_POINT('Ctrl Pts',(-36.5170081383915,-90.734631230289,113.628728270799));
#45993=CARTESIAN_POINT('Ctrl Pts',(-38.9271779091243,-89.2542863205614,
113.470779747607));
#45994=CARTESIAN_POINT('Ctrl Pts',(-39.0051651730729,-86.4268745425969,
113.312831224414));
#45995=CARTESIAN_POINT('Ctrl Pts',(-36.6802612498903,-84.8159241636338,
113.154882701222));
#45996=CARTESIAN_POINT('Ctrl Pts',(-34.0603858179699,-85.8820348974369,
112.996934178029));
#45997=CARTESIAN_POINT('Ctrl Pts',(-33.5209002515244,-88.6585965659594,
112.838985654837));
#45998=CARTESIAN_POINT('Ctrl Pts',(-35.550939705938,-90.6281851496574,112.681037131644));
#45999=CARTESIAN_POINT('Ctrl Pts',(-38.3099291487532,-90.0050345820214,
112.523088608452));
#46000=CARTESIAN_POINT('Ctrl Pts',(-39.29637676304,-87.3541365304588,112.365140085259));
#46001=CARTESIAN_POINT('Ctrl Pts',(-37.6159004983729,-85.0789796349018,
112.207191562067));
#46002=CARTESIAN_POINT('Ctrl Pts',(-34.7921370745499,-85.2423794567828,
112.049243038875));
#46003=CARTESIAN_POINT('Ctrl Pts',(-33.3853069070695,-87.6961863471835,
111.891294515682));
#46004=CARTESIAN_POINT('Ctrl Pts',(-34.6709401219796,-90.2156082277396,
111.733345992489));
#46005=CARTESIAN_POINT('Ctrl Pts',(-37.4833921840904,-90.5163619041062,
111.575397469297));
#46006=CARTESIAN_POINT('Ctrl Pts',(-39.2726983455438,-88.325763164926,111.417448946105));
#46007=CARTESIAN_POINT('Ctrl Pts',(-38.4165491290474,-85.6299612629752,
111.259500422912));
#46008=CARTESIAN_POINT('Ctrl Pts',(-35.6911889905757,-84.8731577936227,
111.10155189972));
#46009=CARTESIAN_POINT('Ctrl Pts',(-33.5676190796432,-86.7415234454372,
110.943603376527));
#46010=CARTESIAN_POINT('Ctrl Pts',(-33.9712156489426,-89.5410679056005,
110.785654853335));
#46011=CARTESIAN_POINT('Ctrl Pts',(-36.5360499641112,-90.7335293565653,
110.627706330142));
#46012=CARTESIAN_POINT('Ctrl Pts',(-38.9366647571119,-89.2377392674329,
110.46975780695));
#46013=CARTESIAN_POINT('Ctrl Pts',(-38.9964956073178,-86.4098850204116,
110.311809283757));
#46014=CARTESIAN_POINT('Ctrl Pts',(-36.6612957008989,-84.8138960543492,
110.153860760565));
#46015=CARTESIAN_POINT('Ctrl Pts',(-34.0483197744451,-85.8968070283112,
109.995912237372));
#46016=CARTESIAN_POINT('Ctrl Pts',(-33.5266736235439,-88.6767754905713,
109.83796371418));
#46017=CARTESIAN_POINT('Ctrl Pts',(-35.5693179621701,-90.6332885994736,
109.680015190987));
#46018=CARTESIAN_POINT('Ctrl Pts',(-38.3242492637062,-89.9924353947184,
109.522066667795));
#46019=CARTESIAN_POINT('Ctrl Pts',(-39.2936551641482,-87.335258046265,109.364118144603));
#46020=CARTESIAN_POINT('Ctrl Pts',(-37.5986046940346,-85.0709383184164,
109.20616962141));
#46021=CARTESIAN_POINT('Ctrl Pts',(-34.7759488142895,-85.2524662955004,
109.048221098218));
#46022=CARTESIAN_POINT('Ctrl Pts',(-33.3849032449937,-87.7152555607639,
108.890272575025));
#46023=CARTESIAN_POINT('Ctrl Pts',(-34.686687764235,-90.2263710609368,108.732324051833));
#46024=CARTESIAN_POINT('Ctrl Pts',(-37.5010117457022,-90.5090585411099,
108.57437552864));
#46025=CARTESIAN_POINT('Ctrl Pts',(-39.2762177428359,-88.3070183913275,
108.416427005448));
#46026=CARTESIAN_POINT('Ctrl Pts',(-38.4027711856895,-85.6167641253612,
108.258478482255));
#46027=CARTESIAN_POINT('Ctrl Pts',(-35.672618594028,-84.8774866292816,108.100529959063));
#46028=CARTESIAN_POINT('Ctrl Pts',(-33.5610670260011,-86.7594269128483,
107.94258143587));
#46029=CARTESIAN_POINT('Ctrl Pts',(-33.9826768167633,-89.5563680122778,
107.784632912678));
#46030=CARTESIAN_POINT('Ctrl Pts',(-36.555021123935,-90.7322417998678,107.626684389485));
#46031=CARTESIAN_POINT('Ctrl Pts',(-38.9461751355661,-89.2212621070181,
107.468735866293));
#46032=CARTESIAN_POINT('Ctrl Pts',(-38.9874498238763,-86.392683146967,107.3107873431));
#46033=CARTESIAN_POINT('Ctrl Pts',(-36.6428674409066,-84.8125415007088,
107.152838819908));
#46034=CARTESIAN_POINT('Ctrl Pts',(-34.035217803829,-85.9105078648088,106.994890296715));
#46035=CARTESIAN_POINT('Ctrl Pts',(-33.534938467138,-88.6972348346522,106.836941773523));
#46036=CARTESIAN_POINT('Ctrl Pts',(-34.9001756782217,-89.9855519312418,
106.731642758061));
#46037=CARTESIAN_POINT('Ctrl Pts',(-35.7047260767089,-90.2006423906074,
106.678993250331));
#46038=CARTESIAN_POINT('Ctrl Pts',(-34.3005945243415,-86.0121302673453,
122.10700224989));
#46039=CARTESIAN_POINT('Ctrl Pts',(-33.7195574121284,-86.691716730324,122.054352742159));
#46040=CARTESIAN_POINT('Ctrl Pts',(-33.2951150221062,-88.6618397545135,
121.949053726697));
#46041=CARTESIAN_POINT('Ctrl Pts',(-35.4324726759634,-90.8232133229407,
121.791105203505));
#46042=CARTESIAN_POINT('Ctrl Pts',(-38.4073638886993,-90.2088410331937,
121.633156680312));
#46043=CARTESIAN_POINT('Ctrl Pts',(-39.5208314753878,-87.3849394635757,
121.47520815712));
#46044=CARTESIAN_POINT('Ctrl Pts',(-37.7641357365242,-84.9073965671192,
121.317259633927));
#46045=CARTESIAN_POINT('Ctrl Pts',(-34.7296228380358,-85.0246867291107,
121.159311110735));
#46046=CARTESIAN_POINT('Ctrl Pts',(-33.1687859925402,-87.6294154931395,
121.001362587543));
#46047=CARTESIAN_POINT('Ctrl Pts',(-34.4966948056566,-90.3604655387852,
120.84341406435));
#46048=CARTESIAN_POINT('Ctrl Pts',(-37.5094202989532,-90.7414283685601,
120.685465541158));
#46049=CARTESIAN_POINT('Ctrl Pts',(-39.4753937445287,-88.4270173924454,
120.527517017965));
#46050=CARTESIAN_POINT('Ctrl Pts',(-38.6121375823184,-85.5155799050329,
120.369568494773));
#46051=CARTESIAN_POINT('Ctrl Pts',(-35.7023346827516,-84.6468562941794,
120.21161997158));
#46052=CARTESIAN_POINT('Ctrl Pts',(-33.3842173836834,-86.6084779472515,
120.053671448388));
#46053=CARTESIAN_POINT('Ctrl Pts',(-33.759550899638,-89.6219089250578,119.895722925195));
#46054=CARTESIAN_POINT('Ctrl Pts',(-36.4880323490067,-90.9549597255175,
119.737774402003));
#46055=CARTESIAN_POINT('Ctrl Pts',(-39.0958302919176,-89.3989953274986,
119.57982587881));
#46056=CARTESIAN_POINT('Ctrl Pts',(-39.2185337884644,-86.3647605517735,
119.421877355618));
#46057=CARTESIAN_POINT('Ctrl Pts',(-36.7448912409745,-84.6033041649243,
119.263928832425));
#46058=CARTESIAN_POINT('Ctrl Pts',(-33.9176791484729,-85.7116849170728,
119.105980309233));
#46059=CARTESIAN_POINT('Ctrl Pts',(-33.3002447130985,-88.6849677793764,
118.94803178604));
#46060=CARTESIAN_POINT('Ctrl Pts',(-35.4523969669423,-90.8273675654965,
118.790083262848));
#46061=CARTESIAN_POINT('Ctrl Pts',(-38.4228449123274,-90.1964355686042,
118.632134739656));
#46062=CARTESIAN_POINT('Ctrl Pts',(-39.5183737411446,-87.3642186310916,
118.474186216463));
#46063=CARTESIAN_POINT('Ctrl Pts',(-37.7457007823939,-84.8986017172065,
118.316237693271));
#46064=CARTESIAN_POINT('Ctrl Pts',(-34.7120546948084,-85.0350846919935,
118.158289170078));
#46065=CARTESIAN_POINT('Ctrl Pts',(-33.1679501216105,-87.6499225943353,
118.000340646886));
#46066=CARTESIAN_POINT('Ctrl Pts',(-34.5133797176062,-90.3723214243045,
117.842392123693));
#46067=CARTESIAN_POINT('Ctrl Pts',(-37.5284833874464,-90.7339649610648,
117.684443600501));
#46068=CARTESIAN_POINT('Ctrl Pts',(-39.4795583339449,-88.4069620085909,
117.526495077308));
#46069=CARTESIAN_POINT('Ctrl Pts',(-38.5976242423615,-85.5011353713612,
117.368546554116));
#46070=CARTESIAN_POINT('Ctrl Pts',(-35.6823039307278,-84.6511096845977,
117.210598030923));
#46071=CARTESIAN_POINT('Ctrl Pts',(-33.3768296601401,-86.6275773861417,
117.052649507731));
#46072=CARTESIAN_POINT('Ctrl Pts',(-33.7715048339112,-89.6385353225436,
116.894700984538));
#46073=CARTESIAN_POINT('Ctrl Pts',(-36.508489475485,-90.9540395070176,116.736752461346));
#46074=CARTESIAN_POINT('Ctrl Pts',(-39.1062428519719,-89.3813623047506,
116.578803938153));
#46075=CARTESIAN_POINT('Ctrl Pts',(-39.2094609840087,-86.3464023042238,
116.420855414961));
#46076=CARTESIAN_POINT('Ctrl Pts',(-36.7245591305151,-84.6008654337788,
116.262906891769));
#46077=CARTESIAN_POINT('Ctrl Pts',(-33.9045222271802,-85.7273768857439,
116.104958368576));
#46078=CARTESIAN_POINT('Ctrl Pts',(-33.3061919667124,-88.7045629879195,
115.947009845384));
#46079=CARTESIAN_POINT('Ctrl Pts',(-35.4720561988855,-90.8330996484852,
115.789061322191));
#46080=CARTESIAN_POINT('Ctrl Pts',(-38.4383916961712,-90.1831074138222,
115.631112798999));
#46081=CARTESIAN_POINT('Ctrl Pts',(-39.5157122801964,-87.3439144744794,
115.473164275806));
#46082=CARTESIAN_POINT('Ctrl Pts',(-37.72724414265,-84.8897307184088,115.315215752614));
#46083=CARTESIAN_POINT('Ctrl Pts',(-34.6945369500458,-85.0456899166149,
115.157267229421));
#46084=CARTESIAN_POINT('Ctrl Pts',(-33.167254078298,-87.6703886073687,114.999318706229));
#46085=CARTESIAN_POINT('Ctrl Pts',(-34.5301364570117,-90.384092314366,114.841370183036));
#46086=CARTESIAN_POINT('Ctrl Pts',(-37.5475000836009,-90.7263684200397,
114.683421659844));
#46087=CARTESIAN_POINT('Ctrl Pts',(-39.4835931268037,-88.3868855892327,
114.525473136651));
#46088=CARTESIAN_POINT('Ctrl Pts',(-38.5830189079561,-85.4867817524837,
114.367524613459));
#46089=CARTESIAN_POINT('Ctrl Pts',(-35.6623006815607,-84.655492855902,114.209576090266));
#46090=CARTESIAN_POINT('Ctrl Pts',(-33.3695648338605,-86.6467232595093,
114.051627567074));
#46091=CARTESIAN_POINT('Ctrl Pts',(-33.7835652275568,-89.6550849168899,
113.893679043881));
#46092=CARTESIAN_POINT('Ctrl Pts',(-36.5289402969378,-90.9529878084809,
113.735730520689));
#46093=CARTESIAN_POINT('Ctrl Pts',(-39.1165419634042,-89.3636628564086,
113.577781997497));
#46094=CARTESIAN_POINT('Ctrl Pts',(-39.200270494318,-86.3281026575837,113.419833474304));
#46095=CARTESIAN_POINT('Ctrl Pts',(-36.7042117771879,-84.5985573218906,
113.261884951112));
#46096=CARTESIAN_POINT('Ctrl Pts',(-33.8914663366415,-85.7431530034586,
113.103936427919));
#46097=CARTESIAN_POINT('Ctrl Pts',(-33.3122649178366,-88.7241196091141,
112.945987904727));
#46098=CARTESIAN_POINT('Ctrl Pts',(-35.4917518315888,-90.8387053795102,
112.788039381534));
#46099=CARTESIAN_POINT('Ctrl Pts',(-38.453852579297,-90.169679708848,112.630090858342));
#46100=CARTESIAN_POINT('Ctrl Pts',(-39.5129205012362,-87.3236278252206,
112.472142335149));
#46101=CARTESIAN_POINT('Ctrl Pts',(-37.7087309226789,-84.8809784127581,
112.314193811957));
#46102=CARTESIAN_POINT('Ctrl Pts',(-34.6770876625573,-85.0564074039161,
112.156245288764));
#46103=CARTESIAN_POINT('Ctrl Pts',(-33.1666894615623,-87.690858667844,111.998296765572));
#46104=CARTESIAN_POINT('Ctrl Pts',(-34.5469684318501,-90.3957553667502,
111.840348242379));
#46105=CARTESIAN_POINT('Ctrl Pts',(-37.5664676103507,-90.7186499294537,
111.682399719187));
#46106=CARTESIAN_POINT('Ctrl Pts',(-39.4874989258283,-88.3667836763398,
111.524451195994));
#46107=CARTESIAN_POINT('Ctrl Pts',(-38.5683217100771,-85.4725222103394,
111.366502672802));
#46108=CARTESIAN_POINT('Ctrl Pts',(-35.6423259890843,-84.6600043776687,
111.20855414961));
#46109=CARTESIAN_POINT('Ctrl Pts',(-33.3624230929842,-86.6659153856447,
111.050605626417));
#46110=CARTESIAN_POINT('Ctrl Pts',(-33.7957316374614,-89.6715567302636,
110.892657103225));
#46111=CARTESIAN_POINT('Ctrl Pts',(-36.5493839439221,-90.9518048170095,
110.734708580032));
#46112=CARTESIAN_POINT('Ctrl Pts',(-39.1267272142361,-89.3458976422023,
110.57676005684));
#46113=CARTESIAN_POINT('Ctrl Pts',(-39.1909626924081,-86.3098624006304,
110.418811533647));
#46114=CARTESIAN_POINT('Ctrl Pts',(-36.6838500222728,-84.5963799072419,
110.260863010455));
#46115=CARTESIAN_POINT('Ctrl Pts',(-33.8785120150366,-85.7590126291711,
110.102914487262));
#46116=CARTESIAN_POINT('Ctrl Pts',(-33.3184633139996,-88.7436368299307,
109.94496596407));
#46117=CARTESIAN_POINT('Ctrl Pts',(-35.5114830584221,-90.8441845351322,
109.787017440877));
#46118=CARTESIAN_POINT('Ctrl Pts',(-38.469226912577,-90.1561529944824,109.629068917685));
#46119=CARTESIAN_POINT('Ctrl Pts',(-39.5099985436573,-87.30335954464,109.471120394492));
#46120=CARTESIAN_POINT('Ctrl Pts',(-37.6901618356908,-84.8723451105772,
109.3131718713));
#46121=CARTESIAN_POINT('Ctrl Pts',(-34.6597076548352,-85.0672368155999,
109.155223348107));
#46122=CARTESIAN_POINT('Ctrl Pts',(-33.1662560826888,-87.7113317189285,
108.997274824915));
#46123=CARTESIAN_POINT('Ctrl Pts',(-34.5638753841477,-90.40731053828,108.839326301722));
#46124=CARTESIAN_POINT('Ctrl Pts',(-37.5853842889775,-90.7108089074273,
108.68137777853));
#46125=CARTESIAN_POINT('Ctrl Pts',(-39.4912774141359,-88.3466589498619,
108.523429255338));
#46126=CARTESIAN_POINT('Ctrl Pts',(-38.5535294619846,-85.4583535257525,
108.365480732145));
#46127=CARTESIAN_POINT('Ctrl Pts',(-35.6223884769483,-84.6646518935827,
108.207532208953));
#46128=CARTESIAN_POINT('Ctrl Pts',(-33.3553886902093,-86.68513687065,108.04958368576));
#46129=CARTESIAN_POINT('Ctrl Pts',(-33.8080365536181,-89.6879832003056,
107.891635162568));
#46130=CARTESIAN_POINT('Ctrl Pts',(-36.5697517227279,-90.9504224729536,
107.733686639375));
#46131=CARTESIAN_POINT('Ctrl Pts',(-39.1369377278005,-89.328207466072,107.575738116183));
#46132=CARTESIAN_POINT('Ctrl Pts',(-39.1812509764153,-86.2913941595414,
107.41778959299));
#46133=CARTESIAN_POINT('Ctrl Pts',(-36.6640651105022,-84.5949256340617,
107.259841069798));
#46134=CARTESIAN_POINT('Ctrl Pts',(-33.8644455034523,-85.7737220939498,
107.101892546605));
#46135=CARTESIAN_POINT('Ctrl Pts',(-33.3273365989096,-88.7656023501531,
106.943944023413));
#46136=CARTESIAN_POINT('Ctrl Pts',(-34.793079852941,-90.1487627841414,106.838645007951));
#46137=CARTESIAN_POINT('Ctrl Pts',(-35.656859648523,-90.379687774511,106.78599550022));
#46138=CARTESIAN_POINT('Ctrl Pts',(-34.1597289706645,-85.8916921494934,
122.21400449978));
#46139=CARTESIAN_POINT('Ctrl Pts',(-33.53885013256,-86.6178778692294,122.161354992049));
#46140=CARTESIAN_POINT('Ctrl Pts',(-33.0853037197404,-88.7230922668478,
122.056055976587));
#46141=CARTESIAN_POINT('Ctrl Pts',(-35.3692200287798,-91.0326712621785,
121.898107453395));
#46142=CARTESIAN_POINT('Ctrl Pts',(-38.5480995888403,-90.3761714527792,
121.740158930202));
#46143=CARTESIAN_POINT('Ctrl Pts',(-39.7379176692327,-87.3586348985517,
121.58221040701));
#46144=CARTESIAN_POINT('Ctrl Pts',(-37.8607652699747,-84.7112068383249,
121.424261883817));
#46145=CARTESIAN_POINT('Ctrl Pts',(-34.61817576403,-84.8365395889664,121.266313360625));
#46146=CARTESIAN_POINT('Ctrl Pts',(-32.9503123062022,-87.6198746541358,
121.108364837432));
#46147=CARTESIAN_POINT('Ctrl Pts',(-34.369275852018,-90.5381928536177,120.95041631424));
#46148=CARTESIAN_POINT('Ctrl Pts',(-37.5885839899804,-90.9452783119125,
120.792467791047));
#46149=CARTESIAN_POINT('Ctrl Pts',(-39.6893642723,-88.472168130924,120.634519267855));
#46150=CARTESIAN_POINT('Ctrl Pts',(-38.7669146185452,-85.3610933193452,
120.476570744662));
#46151=CARTESIAN_POINT('Ctrl Pts',(-35.6575864785321,-84.4328013138893,
120.31862222147));
#46152=CARTESIAN_POINT('Ctrl Pts',(-33.1805158319542,-86.5289314012103,
120.160673698278));
#46153=CARTESIAN_POINT('Ctrl Pts',(-33.5815859742726,-89.7489933987689,
120.002725175085));
#46154=CARTESIAN_POINT('Ctrl Pts',(-36.4971594487814,-91.1734515180982,
119.844776651893));
#46155=CARTESIAN_POINT('Ctrl Pts',(-39.2837741464878,-89.510794611564,119.6868281287));
#46156=CARTESIAN_POINT('Ctrl Pts',(-39.4148914241384,-86.2685022992656,
119.528879605508));
#46157=CARTESIAN_POINT('Ctrl Pts',(-36.7716311598815,-84.3862628142986,
119.370931082315));
#46158=CARTESIAN_POINT('Ctrl Pts',(-33.7505570801529,-85.5706452558094,
119.212982559123));
#46159=CARTESIAN_POINT('Ctrl Pts',(-33.0907851537421,-88.7478061808178,
119.05503403593));
#46160=CARTESIAN_POINT('Ctrl Pts',(-35.390510528772,-91.0371103612257,118.897085512738));
#46161=CARTESIAN_POINT('Ctrl Pts',(-38.5646421465544,-90.3629153452456,
118.739136989545));
#46162=CARTESIAN_POINT('Ctrl Pts',(-39.7352914081054,-87.336493238188,118.581188466353));
#46163=CARTESIAN_POINT('Ctrl Pts',(-37.8410662306873,-84.7018089253856,
118.42323994316));
#46164=CARTESIAN_POINT('Ctrl Pts',(-34.5994029728857,-84.8476505403629,
118.265291419968));
#46165=CARTESIAN_POINT('Ctrl Pts',(-32.9494191195869,-87.6417879276527,
118.107342896776));
#46166=CARTESIAN_POINT('Ctrl Pts',(-34.3871048486989,-90.5508616974336,
117.949394373583));
#46167=CARTESIAN_POINT('Ctrl Pts',(-37.608954234816,-90.9373031384225,117.79144585039));
#46168=CARTESIAN_POINT('Ctrl Pts',(-39.6938144276922,-88.4507375490153,
117.633497327198));
#46169=CARTESIAN_POINT('Ctrl Pts',(-38.75140609859,-85.3456583237236,117.475548804006));
#46170=CARTESIAN_POINT('Ctrl Pts',(-35.6361822174592,-84.4373463593699,
117.317600280813));
#46171=CARTESIAN_POINT('Ctrl Pts',(-33.1726215320663,-86.5493404889904,
117.159651757621));
#46172=CARTESIAN_POINT('Ctrl Pts',(-33.5943595900474,-89.7667598686481,
117.001703234428));
#46173=CARTESIAN_POINT('Ctrl Pts',(-36.5190193208135,-91.1724682001983,
116.843754711236));
#46174=CARTESIAN_POINT('Ctrl Pts',(-39.2949006959841,-89.4919524921089,
116.685806188043));
#46175=CARTESIAN_POINT('Ctrl Pts',(-39.4051964973076,-86.2488852263305,
116.527857664851));
#46176=CARTESIAN_POINT('Ctrl Pts',(-36.7499048762192,-84.3836568593119,
116.369909141658));
#46177=CARTESIAN_POINT('Ctrl Pts',(-33.7364979885157,-85.5874132230723,
116.211960618466));
#46178=CARTESIAN_POINT('Ctrl Pts',(-33.09714021065,-88.7687450331853,116.054012095273));
#46179=CARTESIAN_POINT('Ctrl Pts',(-35.4115177946254,-91.0432354932543,
115.896063572081));
#46180=CARTESIAN_POINT('Ctrl Pts',(-38.5812549736636,-90.3486732786356,
115.738115048888));
#46181=CARTESIAN_POINT('Ctrl Pts',(-39.7324474507292,-87.3147968251685,
115.580166525696));
#46182=CARTESIAN_POINT('Ctrl Pts',(-37.8213440188034,-84.6923296420309,
115.422218002503));
#46183=CARTESIAN_POINT('Ctrl Pts',(-34.5806840360298,-84.8589829654392,
115.264269479311));
#46184=CARTESIAN_POINT('Ctrl Pts',(-32.9486753485711,-87.6636572955911,
115.106320956118));
#46185=CARTESIAN_POINT('Ctrl Pts',(-34.4050105980457,-90.5634397176517,
114.948372432926));
#46186=CARTESIAN_POINT('Ctrl Pts',(-37.6292749061893,-90.9291857024342,
114.790423909734));
#46187=CARTESIAN_POINT('Ctrl Pts',(-39.6981258863743,-88.4292844891979,
114.632475386541));
#46188=CARTESIAN_POINT('Ctrl Pts',(-38.7357992761253,-85.3303204769252,
114.474526863349));
#46189=CARTESIAN_POINT('Ctrl Pts',(-35.6148073451141,-84.4420300848144,
114.316578340156));
#46190=CARTESIAN_POINT('Ctrl Pts',(-33.1648585565099,-86.5697991952607,
114.158629816964));
#46191=CARTESIAN_POINT('Ctrl Pts',(-33.6072469651159,-89.7844442689952,
114.000681293771));
#46192=CARTESIAN_POINT('Ctrl Pts',(-36.5408724554843,-91.1713443866728,
113.842732770579));
#46193=CARTESIAN_POINT('Ctrl Pts',(-39.3059060176841,-89.4730393922558,
113.684784247386));
#46194=CARTESIAN_POINT('Ctrl Pts',(-39.3953758155633,-86.2293307725704,
113.526835724194));
#46195=CARTESIAN_POINT('Ctrl Pts',(-36.7281623044855,-84.3811904801474,
113.368887201001));
#46196=CARTESIAN_POINT('Ctrl Pts',(-33.7225468553131,-85.6042711094801,
113.210938677809));
#46197=CARTESIAN_POINT('Ctrl Pts',(-33.1036295841489,-88.7896426522691,
113.052990154616));
#46198=CARTESIAN_POINT('Ctrl Pts',(-35.4325639572396,-91.049225609363,112.895041631424));
#46199=CARTESIAN_POINT('Ctrl Pts',(-38.5977760098409,-90.3343248356746,
112.737093108231));
#46200=CARTESIAN_POINT('Ctrl Pts',(-39.7294642394323,-87.2931191199824,
112.579144585039));
#46201=CARTESIAN_POINT('Ctrl Pts',(-37.8015613469849,-84.6829771906143,
112.421196061847));
#46202=CARTESIAN_POINT('Ctrl Pts',(-34.5620382505646,-84.8704353510495,
112.263247538654));
#46203=CARTESIAN_POINT('Ctrl Pts',(-32.9480720160551,-87.6855309885044,
112.105299015462));
#46204=CARTESIAN_POINT('Ctrl Pts',(-34.4229967417206,-90.5759025057607,
111.947350492269));
#46205=CARTESIAN_POINT('Ctrl Pts',(-37.6495430366109,-90.9209379548012,
111.789401969077));
#46206=CARTESIAN_POINT('Ctrl Pts',(-39.7022995061128,-88.4078041877537,
111.631453445884));
#46207=CARTESIAN_POINT('Ctrl Pts',(-38.7200942911067,-85.3150831577036,
111.473504922692));
#46208=CARTESIAN_POINT('Ctrl Pts',(-35.5934629875929,-84.4468509617149,
111.315556399499));
#46209=CARTESIAN_POINT('Ctrl Pts',(-33.1572271063251,-86.590307325852,111.157607876307));
#46210=CARTESIAN_POINT('Ctrl Pts',(-33.6202476259802,-89.8020455549267,
110.999659353114));
#46211=CARTESIAN_POINT('Ctrl Pts',(-36.562717923733,-91.1700802774536,110.841710829922));
#46212=CARTESIAN_POINT('Ctrl Pts',(-39.3167896713602,-89.4540560169718,
110.683762306729));
#46213=CARTESIAN_POINT('Ctrl Pts',(-39.3854297774984,-86.2098397808493,
110.525813783537));
#46214=CARTESIAN_POINT('Ctrl Pts',(-36.7064043436466,-84.3788637601345,
110.367865260344));
#46215=CARTESIAN_POINT('Ctrl Pts',(-33.7087042556281,-85.6212182300311,
110.209916737152));
#46216=CARTESIAN_POINT('Ctrl Pts',(-33.1102530044553,-88.81049816929,110.05196821396));
#46217=CARTESIAN_POINT('Ctrl Pts',(-35.453648154674,-91.0550804707907,109.894019690767));
#46218=CARTESIAN_POINT('Ctrl Pts',(-38.6142045614478,-90.3198705942462,
109.736071167574));
#46219=CARTESIAN_POINT('Ctrl Pts',(-39.7263419231664,-87.2714610430151,
109.578122644382));
#46220=CARTESIAN_POINT('Ctrl Pts',(-37.7817189773471,-84.6737519027377,
109.42017412119));
#46221=CARTESIAN_POINT('Ctrl Pts',(-34.5434664953808,-84.8820073356995,
109.262225597997));
#46222=CARTESIAN_POINT('Ctrl Pts',(-32.9476089203839,-87.7074078770932,
109.104277074805));
#46223=CARTESIAN_POINT('Ctrl Pts',(-34.4410630040604,-90.5882500156232,
108.946328551612));
#46224=CARTESIAN_POINT('Ctrl Pts',(-37.6697568322527,-90.9125592737444,
108.78838002842));
#46225=CARTESIAN_POINT('Ctrl Pts',(-39.7063370854358,-88.3862995083966,
108.630431505227));
#46226=CARTESIAN_POINT('Ctrl Pts',(-38.7042877382798,-85.2999429261436,
108.472482982035));
#46227=CARTESIAN_POINT('Ctrl Pts',(-35.5721583598686,-84.451817157884,108.314534458842));
#46228=CARTESIAN_POINT('Ctrl Pts',(-33.1497103544175,-86.6108468284517,
108.15658593565));
#46229=CARTESIAN_POINT('Ctrl Pts',(-33.633396290473,-89.8195983883335,107.998637412457));
#46230=CARTESIAN_POINT('Ctrl Pts',(-36.5844823215209,-91.1686031460394,
107.840688889265));
#46231=CARTESIAN_POINT('Ctrl Pts',(-39.327700320035,-89.4351528251261,107.682740366072));
#46232=CARTESIAN_POINT('Ctrl Pts',(-39.3750521289544,-86.1901051721157,
107.52479184288));
#46233=CARTESIAN_POINT('Ctrl Pts',(-36.6852627800977,-84.3773097674146,
107.366843319688));
#46234=CARTESIAN_POINT('Ctrl Pts',(-33.6936732030756,-85.6369363230908,
107.208894796495));
#46235=CARTESIAN_POINT('Ctrl Pts',(-33.1197347306812,-88.833969865654,107.050946273303));
#46236=CARTESIAN_POINT('Ctrl Pts',(-34.6859840276602,-90.311973637041,106.945647257841));
#46237=CARTESIAN_POINT('Ctrl Pts',(-35.6089932203371,-90.5587331584145,
106.89299775011));
#46238=CARTESIAN_POINT('Ctrl Pts',(-34.0188634169875,-85.7712540316415,
122.321006749669));
#46239=CARTESIAN_POINT('Ctrl Pts',(-33.3581428529916,-86.5440390081347,
122.268357241939));
#46240=CARTESIAN_POINT('Ctrl Pts',(-32.8754924173746,-88.7843447791822,
122.163058226477));
#46241=CARTESIAN_POINT('Ctrl Pts',(-35.3059673815962,-91.2421292014162,
122.005109703285));
#46242=CARTESIAN_POINT('Ctrl Pts',(-38.6888352889812,-90.5435018723648,
121.847161180092));
#46243=CARTESIAN_POINT('Ctrl Pts',(-39.9550038630777,-87.3323303335276,
121.6892126569));
#46244=CARTESIAN_POINT('Ctrl Pts',(-37.9573948034252,-84.5150171095306,
121.531264133707));
#46245=CARTESIAN_POINT('Ctrl Pts',(-34.5067286900242,-84.648392448822,121.373315610515));
#46246=CARTESIAN_POINT('Ctrl Pts',(-32.7318386198642,-87.6103338151322,
121.215367087322));
#46247=CARTESIAN_POINT('Ctrl Pts',(-34.2418568983793,-90.7159201684501,
121.05741856413));
#46248=CARTESIAN_POINT('Ctrl Pts',(-37.6677476810076,-91.149128255265,120.899470040937));
#46249=CARTESIAN_POINT('Ctrl Pts',(-39.9033348000714,-88.5173188694026,
120.741521517745));
#46250=CARTESIAN_POINT('Ctrl Pts',(-38.921691654772,-85.2066067336577,120.583572994552));
#46251=CARTESIAN_POINT('Ctrl Pts',(-35.6128382743126,-84.2187463335991,
120.42562447136));
#46252=CARTESIAN_POINT('Ctrl Pts',(-32.976814280225,-86.4493848551693,120.267675948167));
#46253=CARTESIAN_POINT('Ctrl Pts',(-33.4036210489072,-89.8760778724798,
120.109727424975));
#46254=CARTESIAN_POINT('Ctrl Pts',(-36.5062865485562,-91.3919433106791,
119.951778901783));
#46255=CARTESIAN_POINT('Ctrl Pts',(-39.4717180010579,-89.6225938956291,
119.79383037859));
#46256=CARTESIAN_POINT('Ctrl Pts',(-39.6112490598123,-86.1722440467577,
119.635881855397));
#46257=CARTESIAN_POINT('Ctrl Pts',(-36.7983710787885,-84.169221463673,119.477933332205));
#46258=CARTESIAN_POINT('Ctrl Pts',(-33.5834350118328,-85.4296055945461,
119.319984809013));
#46259=CARTESIAN_POINT('Ctrl Pts',(-32.8813255943857,-88.8106445822591,
119.16203628582));
#46260=CARTESIAN_POINT('Ctrl Pts',(-35.3286240906017,-91.2468531569549,
119.004087762628));
#46261=CARTESIAN_POINT('Ctrl Pts',(-38.7064393807814,-90.5293951218872,
118.846139239435));
#46262=CARTESIAN_POINT('Ctrl Pts',(-39.9522090750663,-87.3087678452843,
118.688190716243));
#46263=CARTESIAN_POINT('Ctrl Pts',(-37.9364316789807,-84.5050161335647,
118.53024219305));
#46264=CARTESIAN_POINT('Ctrl Pts',(-34.4867512509629,-84.6602163887321,
118.372293669858));
#46265=CARTESIAN_POINT('Ctrl Pts',(-32.7308881175633,-87.6336532609701,
118.214345146665));
#46266=CARTESIAN_POINT('Ctrl Pts',(-34.2608299797916,-90.7294019705626,
118.056396623473));
#46267=CARTESIAN_POINT('Ctrl Pts',(-37.6894250821856,-91.1406413157804,
117.89844810028));
#46268=CARTESIAN_POINT('Ctrl Pts',(-39.9080705214394,-88.4945130894395,
117.740499577088));
#46269=CARTESIAN_POINT('Ctrl Pts',(-38.9051879548185,-85.190181276086,117.582551053895));
#46270=CARTESIAN_POINT('Ctrl Pts',(-35.5900605041904,-84.2235830341421,
117.424602530703));
#46271=CARTESIAN_POINT('Ctrl Pts',(-32.9684134039925,-86.4711035918391,
117.26665400751));
#46272=CARTESIAN_POINT('Ctrl Pts',(-33.4172143461837,-89.8949844147526,
117.108705484318));
#46273=CARTESIAN_POINT('Ctrl Pts',(-36.5295491661419,-91.390896893379,116.950756961125));
#46274=CARTESIAN_POINT('Ctrl Pts',(-39.4835585399962,-89.6025426794672,
116.792808437933));
#46275=CARTESIAN_POINT('Ctrl Pts',(-39.6009320106065,-86.1513681484373,
116.634859914741));
#46276=CARTESIAN_POINT('Ctrl Pts',(-36.7752506219235,-84.1664482848449,
116.476911391548));
#46277=CARTESIAN_POINT('Ctrl Pts',(-33.568473749851,-85.4474495604007,116.318962868356));
#46278=CARTESIAN_POINT('Ctrl Pts',(-32.8880884545876,-88.8329270784509,
116.161014345163));
#46279=CARTESIAN_POINT('Ctrl Pts',(-35.3509793903652,-91.2533713380237,
116.003065821971));
#46280=CARTESIAN_POINT('Ctrl Pts',(-38.724118251156,-90.5142391434489,115.845117298778));
#46281=CARTESIAN_POINT('Ctrl Pts',(-39.949182621262,-87.2856791758579,115.687168775586));
#46282=CARTESIAN_POINT('Ctrl Pts',(-37.9154438949567,-84.494928565653,115.529220252393));
#46283=CARTESIAN_POINT('Ctrl Pts',(-34.4668311220138,-84.6722760142634,
115.371271729201));
#46284=CARTESIAN_POINT('Ctrl Pts',(-32.7300966188443,-87.6569259838135,
115.213323206008));
#46285=CARTESIAN_POINT('Ctrl Pts',(-34.2798847390797,-90.7427871209372,
115.055374682816));
#46286=CARTESIAN_POINT('Ctrl Pts',(-37.7110497287778,-91.1320029848287,
114.897426159623));
#46287=CARTESIAN_POINT('Ctrl Pts',(-39.912658645945,-88.4716833891629,114.739477636431));
#46288=CARTESIAN_POINT('Ctrl Pts',(-38.8885796442944,-85.173859201367,114.581529113239));
#46289=CARTESIAN_POINT('Ctrl Pts',(-35.5673140086676,-84.2285673137265,
114.423580590046));
#46290=CARTESIAN_POINT('Ctrl Pts',(-32.9601522791593,-86.4928751310124,
114.265632066854));
#46291=CARTESIAN_POINT('Ctrl Pts',(-33.4309287026749,-89.9138036211001,
114.107683543661));
#46292=CARTESIAN_POINT('Ctrl Pts',(-36.5528046140307,-91.3897009648648,
113.949735020469));
#46293=CARTESIAN_POINT('Ctrl Pts',(-39.495270071964,-89.582415928103,113.791786497276));
#46294=CARTESIAN_POINT('Ctrl Pts',(-39.5904811368084,-86.1305588875572,
113.633837974084));
#46295=CARTESIAN_POINT('Ctrl Pts',(-36.7521128317831,-84.1638236384041,
113.475889450891));
#46296=CARTESIAN_POINT('Ctrl Pts',(-33.5536273739847,-85.4653892155019,
113.317940927699));
#46297=CARTESIAN_POINT('Ctrl Pts',(-32.8949942504612,-88.8551656954239,
113.159992404506));
#46298=CARTESIAN_POINT('Ctrl Pts',(-35.3733760828904,-91.2597458392159,
113.002043881314));
#46299=CARTESIAN_POINT('Ctrl Pts',(-38.7416994403848,-90.4989699625011,
112.844095358121));
#46300=CARTESIAN_POINT('Ctrl Pts',(-39.9460079776284,-87.2626104147444,
112.686146834929));
#46301=CARTESIAN_POINT('Ctrl Pts',(-37.8943917712909,-84.4849759684705,
112.528198311736));
#46302=CARTESIAN_POINT('Ctrl Pts',(-34.446988838572,-84.684463298183,112.370249788544));
#46303=CARTESIAN_POINT('Ctrl Pts',(-32.7294545705478,-87.6802033091648,
112.212301265352));
#46304=CARTESIAN_POINT('Ctrl Pts',(-34.299025051591,-90.7560496447713,112.054352742159));
#46305=CARTESIAN_POINT('Ctrl Pts',(-37.7326184628711,-91.1232259801486,
111.896404218966));
#46306=CARTESIAN_POINT('Ctrl Pts',(-39.9171000863972,-88.4488246991674,
111.738455695774));
#46307=CARTESIAN_POINT('Ctrl Pts',(-38.8718668721363,-85.1576441050679,
111.580507172582));
#46308=CARTESIAN_POINT('Ctrl Pts',(-35.5445999861014,-84.2336975457609,
111.422558649389));
#46309=CARTESIAN_POINT('Ctrl Pts',(-32.9520311196661,-86.5146992660596,
111.264610126197));
#46310=CARTESIAN_POINT('Ctrl Pts',(-33.444763614499,-89.9325343795896,111.106661603004));
#46311=CARTESIAN_POINT('Ctrl Pts',(-36.5760519035439,-91.3883557378978,
110.948713079812));
#46312=CARTESIAN_POINT('Ctrl Pts',(-39.5068521284844,-89.5622143917412,
110.790764556619));
#46313=CARTESIAN_POINT('Ctrl Pts',(-39.5798968625887,-86.1098171610682,
110.632816033427));
#46314=CARTESIAN_POINT('Ctrl Pts',(-36.7289586650204,-84.1613476130271,
110.474867510234));
#46315=CARTESIAN_POINT('Ctrl Pts',(-33.5388964962196,-85.4834238308911,
110.316918987042));
#46316=CARTESIAN_POINT('Ctrl Pts',(-32.9020426949109,-88.8773595086493,
110.158970463849));
#46317=CARTESIAN_POINT('Ctrl Pts',(-35.3958132509259,-91.2659764064493,
110.001021940657));
#46318=CARTESIAN_POINT('Ctrl Pts',(-38.7591822103186,-90.4835881940102,
109.843073417464));
#46319=CARTESIAN_POINT('Ctrl Pts',(-39.9426853026755,-87.23956254139,109.685124894272));
#46320=CARTESIAN_POINT('Ctrl Pts',(-37.8732761190034,-84.4751586948984,
109.52717637108));
#46321=CARTESIAN_POINT('Ctrl Pts',(-34.4272253359264,-84.6967778557991,
109.369227847887));
#46322=CARTESIAN_POINT('Ctrl Pts',(-32.728961758079,-87.7034840352579,109.211279324695));
#46323=CARTESIAN_POINT('Ctrl Pts',(-34.3182506239731,-90.7691894929664,
109.053330801502));
#46324=CARTESIAN_POINT('Ctrl Pts',(-37.754129375528,-91.1143096400617,108.89538227831));
#46325=CARTESIAN_POINT('Ctrl Pts',(-39.9213967567358,-88.425940066931,108.737433755117));
#46326=CARTESIAN_POINT('Ctrl Pts',(-38.8550460145749,-85.1415323265349,
108.579485231925));
#46327=CARTESIAN_POINT('Ctrl Pts',(-35.5219282427889,-84.238982422185,108.421536708732));
#46328=CARTESIAN_POINT('Ctrl Pts',(-32.9440320186257,-86.5365567862535,
108.26358818554));
#46329=CARTESIAN_POINT('Ctrl Pts',(-33.4587560273279,-89.9512135763613,
108.105639662347));
#46330=CARTESIAN_POINT('Ctrl Pts',(-36.5992129203138,-91.3867838191251,
107.947691139155));
#46331=CARTESIAN_POINT('Ctrl Pts',(-39.5184629122695,-89.5420981841802,
107.789742615962));
#46332=CARTESIAN_POINT('Ctrl Pts',(-39.5688532814934,-86.0888161846899,
107.63179409277));
#46333=CARTESIAN_POINT('Ctrl Pts',(-36.7064604496932,-84.1596939007676,
107.473845569577));
#46334=CARTESIAN_POINT('Ctrl Pts',(-33.5229009026989,-85.5001505522318,
107.315897046385));
#46335=CARTESIAN_POINT('Ctrl Pts',(-32.9121328624527,-88.9023373811549,
107.157948523192));
#46336=CARTESIAN_POINT('Ctrl Pts',(-34.5788882023795,-90.4751844899406,
107.052649507731));
#46337=CARTESIAN_POINT('Ctrl Pts',(-35.5611267921512,-90.7377785423181,
107.));
#46338=CARTESIAN_POINT('Ctrl Pts',(-34.4414600780185,-86.1325683851972,
122.));
#46339=CARTESIAN_POINT('Ctrl Pts',(-34.3798518775506,-86.1904649655976,
122.));
#46340=CARTESIAN_POINT('Ctrl Pts',(-34.3216128304826,-86.2515123055306,
122.));
#46341=CARTESIAN_POINT('Ctrl Pts',(-34.2667405503208,-86.3153255861301,
122.));
#46342=CARTESIAN_POINT('Ctrl Pts',(-34.2104153409142,-86.3808285392073,
122.));
#46343=CARTESIAN_POINT('Ctrl Pts',(-34.1576371151041,-86.4492462791581,
122.));
#46344=CARTESIAN_POINT('Ctrl Pts',(-34.1084287995683,-86.5202111532911,
122.));
#46345=CARTESIAN_POINT('Ctrl Pts',(-34.0578709059029,-86.5931222968921,
122.));
#46346=CARTESIAN_POINT('Ctrl Pts',(-34.0110808905349,-86.6687227614682,
122.));
#46347=CARTESIAN_POINT('Ctrl Pts',(-33.9681176865251,-86.7466567865213,
122.));
#46348=CARTESIAN_POINT('Ctrl Pts',(-33.9492077166618,-86.7809589317883,
122.));
#46349=CARTESIAN_POINT('Ctrl Pts',(-33.9310395849474,-86.8157136469207,
122.));
#46350=CARTESIAN_POINT('Ctrl Pts',(-33.9136207415204,-86.8508926744324,
122.));
#46351=CARTESIAN_POINT('Ctrl Pts',(-33.9036898968079,-86.8709489692613,
122.));
#46352=CARTESIAN_POINT('Ctrl Pts',(-33.8940026274005,-86.8911432023781,
122.));
#46353=CARTESIAN_POINT('Ctrl Pts',(-33.8845605482211,-86.9114702857301,
122.));
#46354=CARTESIAN_POINT('Ctrl Pts',(-33.8760549610638,-86.9297812716708,
122.));
#46355=CARTESIAN_POINT('Ctrl Pts',(-33.8677459643075,-86.9482057896219,
122.));
#46356=CARTESIAN_POINT('Ctrl Pts',(-33.8596483989529,-86.9667083655792,
122.));
#46357=CARTESIAN_POINT('Ctrl Pts',(-33.8230867710876,-87.0502500558377,
122.));
#46358=CARTESIAN_POINT('Ctrl Pts',(-33.7907853230142,-87.1354752893954,
122.));
#46359=CARTESIAN_POINT('Ctrl Pts',(-33.7627690901063,-87.2219852884617,
122.));
#46360=CARTESIAN_POINT('Ctrl Pts',(-33.7342897622732,-87.3099252564206,
122.));
#46361=CARTESIAN_POINT('Ctrl Pts',(-33.7102379922034,-87.399193569067,122.));
#46362=CARTESIAN_POINT('Ctrl Pts',(-33.6906791523764,-87.4894084695148,
122.));
#46363=CARTESIAN_POINT('Ctrl Pts',(-33.6717106761794,-87.5769003252127,
122.));
#46364=CARTESIAN_POINT('Ctrl Pts',(-33.6569678380238,-87.6652834048776,
122.));
#46365=CARTESIAN_POINT('Ctrl Pts',(-33.6465510103069,-87.754231352766,122.));
#46366=CARTESIAN_POINT('Ctrl Pts',(-33.6421821764996,-87.7915362609761,
122.));
#46367=CARTESIAN_POINT('Ctrl Pts',(-33.6385747935892,-87.8289407203117,
122.));
#46368=CARTESIAN_POINT('Ctrl Pts',(-33.6357386010791,-87.8664212731137,
122.));
#46369=CARTESIAN_POINT('Ctrl Pts',(-33.6339594736333,-87.8899326109151,
122.));
#46370=CARTESIAN_POINT('Ctrl Pts',(-33.632483836464,-87.9134738968258,122.));
#46371=CARTESIAN_POINT('Ctrl Pts',(-33.6313143896635,-87.937039373452,122.));
#46372=CARTESIAN_POINT('Ctrl Pts',(-33.6306300060648,-87.9508303605176,
122.));
#46373=CARTESIAN_POINT('Ctrl Pts',(-33.630050777169,-87.96462468597,122.));
#46374=CARTESIAN_POINT('Ctrl Pts',(-33.6295772037717,-87.9784133589186,
122.));
#46375=CARTESIAN_POINT('Ctrl Pts',(-33.6262498202146,-88.0752942308254,
122.));
#46376=CARTESIAN_POINT('Ctrl Pts',(-33.6281283514734,-88.1720100978643,
122.));
#46377=CARTESIAN_POINT('Ctrl Pts',(-33.6352771791366,-88.2681411935631,
122.));
#46378=CARTESIAN_POINT('Ctrl Pts',(-33.6424260067998,-88.3642722892619,
122.));
#46379=CARTESIAN_POINT('Ctrl Pts',(-33.6548447005543,-88.4598196576553,
122.));
#46380=CARTESIAN_POINT('Ctrl Pts',(-33.6726501049204,-88.5543823177475,
122.));
#46381=CARTESIAN_POINT('Ctrl Pts',(-33.6897081290363,-88.6449757186696,
122.));
#46382=CARTESIAN_POINT('Ctrl Pts',(-33.7117100089936,-88.7346663111608,
122.));
#46383=CARTESIAN_POINT('Ctrl Pts',(-33.7383811355958,-88.8232147557601,
122.));
#46384=CARTESIAN_POINT('Ctrl Pts',(-33.7472504814174,-88.8526610850746,
122.));
#46385=CARTESIAN_POINT('Ctrl Pts',(-33.7566366115083,-88.8819810727538,
122.));
#46386=CARTESIAN_POINT('Ctrl Pts',(-33.7665306757816,-88.9111657426682,
122.));
#46387=CARTESIAN_POINT('Ctrl Pts',(-33.7758509847573,-88.9386579979677,
122.));
#46388=CARTESIAN_POINT('Ctrl Pts',(-33.7856220321467,-88.9660301755988,
122.));
#46389=CARTESIAN_POINT('Ctrl Pts',(-33.795836894649,-88.9932746472985,122.));
#46390=CARTESIAN_POINT('Ctrl Pts',(-33.8009946724693,-89.0070311645134,
122.));
#46391=CARTESIAN_POINT('Ctrl Pts',(-33.8062625286193,-89.020746848332,122.));
#46392=CARTESIAN_POINT('Ctrl Pts',(-33.8116377932126,-89.0344173805264,
122.));
#46393=CARTESIAN_POINT('Ctrl Pts',(-33.8458891144019,-89.1215263555152,
122.));
#46394=CARTESIAN_POINT('Ctrl Pts',(-33.8845139350508,-89.2068465156693,
122.));
#46395=CARTESIAN_POINT('Ctrl Pts',(-33.9271822694107,-89.2901434462211,
122.));
#46396=CARTESIAN_POINT('Ctrl Pts',(-33.971412073536,-89.3764886710304,122.));
#46397=CARTESIAN_POINT('Ctrl Pts',(-34.0199868853076,-89.4606606049718,
122.));
#46398=CARTESIAN_POINT('Ctrl Pts',(-34.0725949938842,-89.5423946690003,
122.));
#46399=CARTESIAN_POINT('Ctrl Pts',(-34.125766055418,-89.6250033592851,122.));
#46400=CARTESIAN_POINT('Ctrl Pts',(-34.183057610295,-89.7051225474543,122.));
#46401=CARTESIAN_POINT('Ctrl Pts',(-34.2441993414934,-89.7824637049978,
122.));
#46402=CARTESIAN_POINT('Ctrl Pts',(-34.2668881997465,-89.8111639482889,
122.));
#46403=CARTESIAN_POINT('Ctrl Pts',(-34.2901077201578,-89.8394814287244,
122.));
#46404=CARTESIAN_POINT('Ctrl Pts',(-34.3138456838706,-89.8674005141729,
122.));
#46405=CARTESIAN_POINT('Ctrl Pts',(-34.3346009376308,-89.891811525591,122.));
#46406=CARTESIAN_POINT('Ctrl Pts',(-34.3557525477729,-89.91591796448,122.));
#46407=CARTESIAN_POINT('Ctrl Pts',(-34.3772928365918,-89.9397089990812,
122.));
#46408=CARTESIAN_POINT('Ctrl Pts',(-34.3890563049912,-89.9527016328417,
122.));
#46409=CARTESIAN_POINT('Ctrl Pts',(-34.4009310177164,-89.9655949494855,
122.));
#46410=CARTESIAN_POINT('Ctrl Pts',(-34.4129096494478,-89.9783813265245,
122.));
#46411=CARTESIAN_POINT('Ctrl Pts',(-34.4819204330028,-90.0520456579833,
122.));
#46412=CARTESIAN_POINT('Ctrl Pts',(-34.5544336142438,-90.1222254583658,
122.));
#46413=CARTESIAN_POINT('Ctrl Pts',(-34.6301406718656,-90.1886295132617,
122.));
#46414=CARTESIAN_POINT('Ctrl Pts',(-34.6923348072412,-90.243181135124,122.));
#46415=CARTESIAN_POINT('Ctrl Pts',(-34.7566855153176,-90.2951845232665,
122.));
#46416=CARTESIAN_POINT('Ctrl Pts',(-34.8230440286038,-90.344464887705,122.));
#46417=CARTESIAN_POINT('Ctrl Pts',(-34.847661598239,-90.3627468344084,122.));
#46418=CARTESIAN_POINT('Ctrl Pts',(-34.8725556727621,-90.3806538796401,
122.));
#46419=CARTESIAN_POINT('Ctrl Pts',(-34.8977192636688,-90.3981765345118,
122.));
#46420=CARTESIAN_POINT('Ctrl Pts',(-34.9145301473448,-90.4098827855725,
122.));
#46421=CARTESIAN_POINT('Ctrl Pts',(-34.9314624553121,-90.4214181097377,
122.));
#46422=CARTESIAN_POINT('Ctrl Pts',(-34.9484990431383,-90.4327698544389,
122.));
#46423=CARTESIAN_POINT('Ctrl Pts',(-35.0334095222549,-90.4893470335797,
122.));
#46424=CARTESIAN_POINT('Ctrl Pts',(-35.1209892792786,-90.5414249135277,
122.));
#46425=CARTESIAN_POINT('Ctrl Pts',(-35.2109479563236,-90.5886955781829,
122.));
#46426=CARTESIAN_POINT('Ctrl Pts',(-35.2944060034241,-90.6325503511392,
122.));
#46427=CARTESIAN_POINT('Ctrl Pts',(-35.3799123921453,-90.6722678394425,
122.));
#46428=CARTESIAN_POINT('Ctrl Pts',(-35.4672629815674,-90.7075731181594,
122.));
#46429=CARTESIAN_POINT('Ctrl Pts',(-35.4976931583414,-90.7198723582621,
122.));
#46430=CARTESIAN_POINT('Ctrl Pts',(-35.5283473555972,-90.7316358396728,
122.));
#46431=CARTESIAN_POINT('Ctrl Pts',(-35.5592126670537,-90.7428672848631,
122.));
#46432=CARTESIAN_POINT('Ctrl Pts',(-38.873093130194,-87.7707538189189,120.387416697508));
#46433=CARTESIAN_POINT('Ctrl Pts',(-38.8746754899396,-87.9451202416974,
120.398449387697));
#46434=CARTESIAN_POINT('Ctrl Pts',(-38.8580898958553,-88.1191876191089,
120.409482077886));
#46435=CARTESIAN_POINT('Ctrl Pts',(-38.8222183368412,-88.2891852552992,
120.420514768075));
#46436=CARTESIAN_POINT('Ctrl Pts',(-38.6510343471469,-89.1004372443804,
120.473164275806));
#46437=CARTESIAN_POINT('Ctrl Pts',(-38.0406454775365,-89.819007834794,120.525813783537));
#46438=CARTESIAN_POINT('Ctrl Pts',(-37.2677605679595,-90.1191530964584,
120.578463291268));
#46439=CARTESIAN_POINT('Ctrl Pts',(-36.4948756583824,-90.4192983581227,
120.631112798999));
#46440=CARTESIAN_POINT('Ctrl Pts',(-35.5594947088388,-90.3010182910378,
120.683762306729));
#46441=CARTESIAN_POINT('Ctrl Pts',(-34.8856618873309,-89.8179146088604,
120.73641181446));
#46442=CARTESIAN_POINT('Ctrl Pts',(-34.2118290658229,-89.3348109266829,
120.789061322191));
#46443=CARTESIAN_POINT('Ctrl Pts',(-33.7995443723506,-88.4868836294129,
120.841710829922));
#46444=CARTESIAN_POINT('Ctrl Pts',(-33.8357037311416,-87.6585662369633,
120.894360337653));
#46445=CARTESIAN_POINT('Ctrl Pts',(-33.8718630899327,-86.8302488445136,
120.947009845384));
#46446=CARTESIAN_POINT('Ctrl Pts',(-34.3564665009871,-86.0215413568844,
120.999659353114));
#46447=CARTESIAN_POINT('Ctrl Pts',(-35.0698409216864,-85.5989796841795,
121.052308860845));
#46448=CARTESIAN_POINT('Ctrl Pts',(-35.7832153423856,-85.1764180114746,
121.104958368576));
#46449=CARTESIAN_POINT('Ctrl Pts',(-36.7253607727297,-85.1400021536939,
121.157607876307));
#46450=CARTESIAN_POINT('Ctrl Pts',(-37.4691400009799,-85.506403846918,121.210257384038));
#46451=CARTESIAN_POINT('Ctrl Pts',(-38.2129192292301,-85.8728055401422,
121.262906891769));
#46452=CARTESIAN_POINT('Ctrl Pts',(-38.7583322553865,-86.642024784371,121.315556399499));
#46453=CARTESIAN_POINT('Ctrl Pts',(-38.8581859196339,-87.4650121706535,
121.36820590723));
#46454=CARTESIAN_POINT('Ctrl Pts',(-38.870330811929,-87.5651095806176,121.374609503989));
#46455=CARTESIAN_POINT('Ctrl Pts',(-38.8758844980629,-87.6660023883209,
121.381013100749));
#46456=CARTESIAN_POINT('Ctrl Pts',(-38.8751287300693,-87.7669767062971,
121.387416697508));
#46457=CARTESIAN_POINT('Ctrl Pts',(-37.1487253572165,-90.7377785423179,
122.));
#46458=CARTESIAN_POINT('Ctrl Pts',(-38.1309639469881,-90.4751844899402,
121.947350492269));
#46459=CARTESIAN_POINT('Ctrl Pts',(-39.7977192277978,-88.9023369720511,
121.842051476808));
#46460=CARTESIAN_POINT('Ctrl Pts',(-39.1869512976859,-85.5001506582564,
121.684102953615));
#46461=CARTESIAN_POINT('Ctrl Pts',(-36.0033916957587,-84.1596937777799,
121.526154430423));
#46462=CARTESIAN_POINT('Ctrl Pts',(-33.1409988246472,-86.0888162082167,
121.36820590723));
#46463=CARTESIAN_POINT('Ctrl Pts',(-33.1913892046506,-89.5420981815712,
121.210257384038));
#46464=CARTESIAN_POINT('Ctrl Pts',(-36.1106392225623,-91.3867838745725,
121.052308860845));
#46465=CARTESIAN_POINT('Ctrl Pts',(-39.2510961586208,-89.9512135954417,
120.894360337653));
#46466=CARTESIAN_POINT('Ctrl Pts',(-39.7658201696681,-86.5365567752375,
120.73641181446));
#46467=CARTESIAN_POINT('Ctrl Pts',(-37.1879239172525,-84.2389823785756,
120.578463291268));
#46468=CARTESIAN_POINT('Ctrl Pts',(-33.8548061047563,-85.1415322964398,
120.420514768075));
#46469=CARTESIAN_POINT('Ctrl Pts',(-32.7884553507106,-88.4259400742007,
120.262566244883));
#46470=CARTESIAN_POINT('Ctrl Pts',(-34.9557227571499,-91.1143096798933,
120.10461772169));
#46471=CARTESIAN_POINT('Ctrl Pts',(-38.3916015495585,-90.769189528319,119.946669198498));
#46472=CARTESIAN_POINT('Ctrl Pts',(-39.9808904341307,-87.7034840345569,
119.788720675305));
#46473=CARTESIAN_POINT('Ctrl Pts',(-38.2826268362602,-84.6967778194338,
119.630772152113));
#46474=CARTESIAN_POINT('Ctrl Pts',(-34.8365760123942,-84.4751586559665,
119.472823628921));
#46475=CARTESIAN_POINT('Ctrl Pts',(-32.7671668042656,-87.2395625351253,
119.314875105728));
#46476=CARTESIAN_POINT('Ctrl Pts',(-33.9506699106112,-90.4835882261257,
119.156926582536));
#46477=CARTESIAN_POINT('Ctrl Pts',(-37.3140389097867,-91.26597644781,118.998978059343));
#46478=CARTESIAN_POINT('Ctrl Pts',(-39.8078094952921,-88.8773595217634,
118.841029536151));
#46479=CARTESIAN_POINT('Ctrl Pts',(-39.170955686452,-85.483423803864,118.683081012958));
#46480=CARTESIAN_POINT('Ctrl Pts',(-35.980893479922,-84.1613475703659,118.525132489766));
#46481=CARTESIAN_POINT('Ctrl Pts',(-33.1299552486368,-86.109817141451,118.367183966573));
#46482=CARTESIAN_POINT('Ctrl Pts',(-33.2029999836058,-89.5622144129554,
118.209235443381));
#46483=CARTESIAN_POINT('Ctrl Pts',(-36.1338002432087,-91.3883557807084,
118.051286920188));
#46484=CARTESIAN_POINT('Ctrl Pts',(-39.2650885692864,-89.932534405182,117.893338396996));
#46485=CARTESIAN_POINT('Ctrl Pts',(-39.7578210699461,-86.5146992512298,
117.735389873803));
#46486=CARTESIAN_POINT('Ctrl Pts',(-37.1652521728484,-84.2336975039545,
117.577441350611));
#46487=CARTESIAN_POINT('Ctrl Pts',(-33.8379852474627,-85.1576440741897,
117.419492827418));
#46488=CARTESIAN_POINT('Ctrl Pts',(-32.7927520208408,-88.4488247072137,
117.261544304226));
#46489=CARTESIAN_POINT('Ctrl Pts',(-34.9772336702029,-91.123226019824,117.103595781034));
#46490=CARTESIAN_POINT('Ctrl Pts',(-38.4108271220914,-90.7560496801034,
116.945647257841));
#46491=CARTESIAN_POINT('Ctrl Pts',(-39.980397621697,-87.680203308119,116.787698734649));
#46492=CARTESIAN_POINT('Ctrl Pts',(-38.2628633333592,-84.6844632617075,
116.629750211456));
#46493=CARTESIAN_POINT('Ctrl Pts',(-34.8154603598683,-84.4849759296366,
116.471801688264));
#46494=CARTESIAN_POINT('Ctrl Pts',(-32.7638441292674,-87.2626104087614,
116.313853165071));
#46495=CARTESIAN_POINT('Ctrl Pts',(-33.9681526807548,-90.4989699947938,
116.155904641879));
#46496=CARTESIAN_POINT('Ctrl Pts',(-37.336476078086,-91.2597458805054,115.997956118686));
#46497=CARTESIAN_POINT('Ctrl Pts',(-39.8148579398261,-88.8551657082742,
115.840007595494));
#46498=CARTESIAN_POINT('Ctrl Pts',(-39.1562248085122,-85.4653891882622,
115.682059072301));
#46499=CARTESIAN_POINT('Ctrl Pts',(-35.9577393128856,-84.1638235957717,
115.524110549109));
#46500=CARTESIAN_POINT('Ctrl Pts',(-33.1193709742919,-86.1305588681857,
115.366162025916));
#46501=CARTESIAN_POINT('Ctrl Pts',(-33.2145820402631,-89.5824159495559,
115.208213502724));
#46502=CARTESIAN_POINT('Ctrl Pts',(-36.1570475329969,-91.3897010076914,
115.050264979531));
#46503=CARTESIAN_POINT('Ctrl Pts',(-39.2789234812742,-89.9138036464711,
114.892316456339));
#46504=CARTESIAN_POINT('Ctrl Pts',(-39.7496999103568,-86.4928751159242,
114.734367933147));
#46505=CARTESIAN_POINT('Ctrl Pts',(-37.1425381500136,-84.2285672718597,
114.576419409954));
#46506=CARTESIAN_POINT('Ctrl Pts',(-33.821272475107,-85.1738591706804,114.418470886761));
#46507=CARTESIAN_POINT('Ctrl Pts',(-32.7971934613455,-88.4716833974796,
114.260522363569));
#46508=CARTESIAN_POINT('Ctrl Pts',(-34.9988024045514,-91.1320030246078,
114.102573840377));
#46509=CARTESIAN_POINT('Ctrl Pts',(-38.4299674348291,-90.7427871561125,
113.944625317184));
#46510=CARTESIAN_POINT('Ctrl Pts',(-39.9797555733929,-87.6569259824923,
113.786676793992));
#46511=CARTESIAN_POINT('Ctrl Pts',(-38.2430210496827,-84.672275977644,113.628728270799));
#46512=CARTESIAN_POINT('Ctrl Pts',(-34.7944082359535,-84.4949285269366,
113.470779747607));
#46513=CARTESIAN_POINT('Ctrl Pts',(-32.7606694855963,-87.2856791701479,
113.312831224414));
#46514=CARTESIAN_POINT('Ctrl Pts',(-33.9857338701916,-90.514239175922,113.154882701222));
#46515=CARTESIAN_POINT('Ctrl Pts',(-37.3588727708761,-91.2533713792378,
112.996934178029));
#46516=CARTESIAN_POINT('Ctrl Pts',(-39.8217637357813,-88.8329270910382,
112.838985654837));
#46517=CARTESIAN_POINT('Ctrl Pts',(-39.1413784324703,-85.4474495329488,
112.681037131644));
#46518=CARTESIAN_POINT('Ctrl Pts',(-35.9346015224717,-84.1664482422435,
112.523088608452));
#46519=CARTESIAN_POINT('Ctrl Pts',(-33.1089201003701,-86.1513681293118,
112.365140085259));
#46520=CARTESIAN_POINT('Ctrl Pts',(-33.2262935723694,-89.6025427011582,
112.207191562067));
#46521=CARTESIAN_POINT('Ctrl Pts',(-36.1803029811607,-91.3908969362198,
112.049243038874));
#46522=CARTESIAN_POINT('Ctrl Pts',(-39.2926378379277,-89.8949844399009,
111.891294515682));
#46523=CARTESIAN_POINT('Ctrl Pts',(-39.7414387854258,-86.4711035764935,
111.733345992489));
#46524=CARTESIAN_POINT('Ctrl Pts',(-37.1197916542217,-84.2235829922162,
111.575397469297));
#46525=CARTESIAN_POINT('Ctrl Pts',(-33.8046641643864,-85.1901812455926,
111.417448946105));
#46526=CARTESIAN_POINT('Ctrl Pts',(-32.8017815859054,-88.494513098026,111.259500422912));
#46527=CARTESIAN_POINT('Ctrl Pts',(-35.0204270513993,-91.1406413556617,
111.10155189972));
#46528=CARTESIAN_POINT('Ctrl Pts',(-38.4490221943426,-90.7294020055796,
110.943603376527));
#46529=CARTESIAN_POINT('Ctrl Pts',(-39.9789640746645,-87.6336532593737,
110.785654853335));
#46530=CARTESIAN_POINT('Ctrl Pts',(-38.2231009204979,-84.66021635197,110.627706330142));
#46531=CARTESIAN_POINT('Ctrl Pts',(-34.7734204516813,-84.5050160949677,
110.46975780695));
#46532=CARTESIAN_POINT('Ctrl Pts',(-32.7576430317562,-87.3087678398475,
110.311809283757));
#46533=CARTESIAN_POINT('Ctrl Pts',(-34.0034127407753,-90.5293951545392,
110.153860760565));
#46534=CARTESIAN_POINT('Ctrl Pts',(-37.381228070904,-91.2468531980925,109.995912237372));
#46535=CARTESIAN_POINT('Ctrl Pts',(-39.8285265960631,-88.8106445945815,
109.83796371418));
#46536=CARTESIAN_POINT('Ctrl Pts',(-39.1264171703115,-85.429605566886,109.680015190987));
#46537=CARTESIAN_POINT('Ctrl Pts',(-35.9114810653333,-84.1692214210988,
109.522066667795));
#46538=CARTESIAN_POINT('Ctrl Pts',(-33.098603051042,-86.1722440278901,109.364118144602));
#46539=CARTESIAN_POINT('Ctrl Pts',(-33.2381341114487,-89.6225939175359,
109.20616962141));
#46540=CARTESIAN_POINT('Ctrl Pts',(-36.2035655990193,-91.3919433535738,
109.048221098218));
#46541=CARTESIAN_POINT('Ctrl Pts',(-39.3062311353703,-89.8760778973243,
108.890272575025));
#46542=CARTESIAN_POINT('Ctrl Pts',(-39.7330379090806,-86.4493848397213,
108.732324051833));
#46543=CARTESIAN_POINT('Ctrl Pts',(-37.0970138838616,-84.2187462913202,
108.57437552864));
#46544=CARTESIAN_POINT('Ctrl Pts',(-33.7881604641648,-85.2066067039222,
108.416427005448));
#46545=CARTESIAN_POINT('Ctrl Pts',(-32.8065173074963,-88.517318877192,108.258478482255));
#46546=CARTESIAN_POINT('Ctrl Pts',(-35.0421044524555,-91.1491282972506,
108.100529959063));
#46547=CARTESIAN_POINT('Ctrl Pts',(-38.4679952768287,-90.7159201995772,
107.94258143587));
#46548=CARTESIAN_POINT('Ctrl Pts',(-39.9780135704577,-87.6103338201277,
107.784632912678));
#46549=CARTESIAN_POINT('Ctrl Pts',(-38.2031234854001,-84.6483923994501,
107.626684389485));
#46550=CARTESIAN_POINT('Ctrl Pts',(-34.7524573177229,-84.5150170933021,
107.468735866293));
#46551=CARTESIAN_POINT('Ctrl Pts',(-32.7548482639927,-87.3323302896557,
107.3107873431));
#46552=CARTESIAN_POINT('Ctrl Pts',(-34.0210167874952,-90.5435019715025,
107.152838819908));
#46553=CARTESIAN_POINT('Ctrl Pts',(-37.403884869873,-91.2421291429392,106.994890296715));
#46554=CARTESIAN_POINT('Ctrl Pts',(-39.8343594515415,-88.7843450828379,
106.836941773523));
#46555=CARTESIAN_POINT('Ctrl Pts',(-39.3517092963752,-86.544039008134,106.731642758061));
#46556=CARTESIAN_POINT('Ctrl Pts',(-38.6909887323791,-85.7712540316409,
106.678993250331));
#46557=CARTESIAN_POINT('Ctrl Pts',(-37.1008589290305,-90.5587331584144,
122.10700224989));
#46558=CARTESIAN_POINT('Ctrl Pts',(-38.0238681217073,-90.3119736370407,
122.054352742159));
#46559=CARTESIAN_POINT('Ctrl Pts',(-39.5901173631341,-88.8339694812193,
121.949053726697));
#46560=CARTESIAN_POINT('Ctrl Pts',(-39.0161789942328,-85.6369364227221,
121.791105203505));
#46561=CARTESIAN_POINT('Ctrl Pts',(-36.0245893655903,-84.3773096518432,
121.633156680312));
#46562=CARTESIAN_POINT('Ctrl Pts',(-33.3347999797929,-86.1901051942237,
121.47520815712));
#46563=CARTESIAN_POINT('Ctrl Pts',(-33.3821517988416,-89.4351528226744,
121.317259633928));
#46564=CARTESIAN_POINT('Ctrl Pts',(-36.1253698217467,-91.1686031981433,
121.159311110735));
#46565=CARTESIAN_POINT('Ctrl Pts',(-39.0764558932698,-89.8195984062634,
121.001362587543));
#46566=CARTESIAN_POINT('Ctrl Pts',(-39.5601418315291,-86.6108468181,120.84341406435));
#46567=CARTESIAN_POINT('Ctrl Pts',(-37.1376937995291,-84.4518171169042,
120.685465541158));
#46568=CARTESIAN_POINT('Ctrl Pts',(-34.0055643828626,-85.2999428978633,
120.527517017965));
#46569=CARTESIAN_POINT('Ctrl Pts',(-33.0035150245384,-88.3862995152278,
120.369568494773));
#46570=CARTESIAN_POINT('Ctrl Pts',(-35.0400953014315,-90.9125593111742,
120.21161997158));
#46571=CARTESIAN_POINT('Ctrl Pts',(-38.2687891680141,-90.588250048844,120.053671448388));
#46572=CARTESIAN_POINT('Ctrl Pts',(-39.7622432692423,-87.7074078764345,
119.895722925195));
#46573=CARTESIAN_POINT('Ctrl Pts',(-38.1663856754298,-84.882007301527,119.737774402003));
#46574=CARTESIAN_POINT('Ctrl Pts',(-34.928133155134,-84.6737518661535,119.57982587881));
#46575=CARTESIAN_POINT('Ctrl Pts',(-32.983510186333,-87.271461037128,119.421877355618));
#46576=CARTESIAN_POINT('Ctrl Pts',(-34.0956475611968,-90.3198706244251,
119.263928832425));
#46577=CARTESIAN_POINT('Ctrl Pts',(-37.2562040053545,-91.0550805096574,
119.105980309233));
#46578=CARTESIAN_POINT('Ctrl Pts',(-39.5995991832854,-88.8104981816133,
118.94803178604));
#46579=CARTESIAN_POINT('Ctrl Pts',(-39.0011479250352,-85.6212182046338,
118.790083262848));
#46580=CARTESIAN_POINT('Ctrl Pts',(-36.0034478015626,-84.3788637200456,
118.632134739656));
#46581=CARTESIAN_POINT('Ctrl Pts',(-33.3244223360271,-86.2098397624152,
118.474186216463));
#46582=CARTESIAN_POINT('Ctrl Pts',(-33.3930624429777,-89.4540560369066,
118.316237693271));
#46583=CARTESIAN_POINT('Ctrl Pts',(-36.1471342231772,-91.1700803176829,
118.158289170078));
#46584=CARTESIAN_POINT('Ctrl Pts',(-39.0896045557298,-89.8020455789757,
118.000340646886));
#46585=CARTESIAN_POINT('Ctrl Pts',(-39.5526250808602,-86.5903073119166,
117.842392123693));
#46586=CARTESIAN_POINT('Ctrl Pts',(-37.1163891707791,-84.4468509224294,
117.684443600501));
#46587=CARTESIAN_POINT('Ctrl Pts',(-33.9897578302874,-85.3150831286874,
117.526495077308));
#46588=CARTESIAN_POINT('Ctrl Pts',(-33.0075526036656,-88.4078041953146,
117.368546554116));
#46589=CARTESIAN_POINT('Ctrl Pts',(-35.0603090974456,-90.920937992084,117.210598030923));
#46590=CARTESIAN_POINT('Ctrl Pts',(-38.2868554304956,-90.5759025389624,
117.052649507731));
#46591=CARTESIAN_POINT('Ctrl Pts',(-39.7617801736042,-87.6855309875216,
116.894700984538));
#46592=CARTESIAN_POINT('Ctrl Pts',(-38.1478139200059,-84.8704353167736,
116.736752461346));
#46593=CARTESIAN_POINT('Ctrl Pts',(-34.9082907852723,-84.6829771541221,
116.578803938153));
#46594=CARTESIAN_POINT('Ctrl Pts',(-32.9803878700246,-87.2931191143603,
116.420855414961));
#46595=CARTESIAN_POINT('Ctrl Pts',(-34.1120761130008,-90.33432486602,116.262906891769));
#46596=CARTESIAN_POINT('Ctrl Pts',(-37.2772882030368,-91.0492256481627,
116.104958368576));
#46597=CARTESIAN_POINT('Ctrl Pts',(-39.6062226036708,-88.7896426643444,
115.947009845384));
#46598=CARTESIAN_POINT('Ctrl Pts',(-38.9873053251861,-85.6042710838831,
115.789061322191));
#46599=CARTESIAN_POINT('Ctrl Pts',(-35.9816898404665,-84.3811904400857,
115.631112798999));
#46600=CARTESIAN_POINT('Ctrl Pts',(-33.3144762978446,-86.229330754367,115.473164275806));
#46601=CARTESIAN_POINT('Ctrl Pts',(-33.4039460967826,-89.4730394124151,
115.315215752614));
#46602=CARTESIAN_POINT('Ctrl Pts',(-36.1689796916844,-91.171344426917,115.157267229421));
#46603=CARTESIAN_POINT('Ctrl Pts',(-39.1026052167479,-89.784444292836,114.999318706229));
#46604=CARTESIAN_POINT('Ctrl Pts',(-39.5449936305852,-86.5697991810826,
114.841370183036));
#46605=CARTESIAN_POINT('Ctrl Pts',(-37.0950448130054,-84.4420300454719,
114.683421659844));
#46606=CARTESIAN_POINT('Ctrl Pts',(-33.974052845083,-85.3303204480892,114.525473136651));
#46607=CARTESIAN_POINT('Ctrl Pts',(-33.0117262234534,-88.4292844970128,
114.367524613459));
#46608=CARTESIAN_POINT('Ctrl Pts',(-35.0805772281069,-90.9291857398147,
114.209576090266));
#46609=CARTESIAN_POINT('Ctrl Pts',(-38.3048415743832,-90.5634397507058,
114.051627567074));
#46610=CARTESIAN_POINT('Ctrl Pts',(-39.761176841081,-87.6636572943497,113.893679043881));
#46611=CARTESIAN_POINT('Ctrl Pts',(-38.1291681343202,-84.8589829310279,
113.735730520689));
#46612=CARTESIAN_POINT('Ctrl Pts',(-34.8885081132199,-84.6923296056491,
113.577781997496));
#46613=CARTESIAN_POINT('Ctrl Pts',(-32.9774046586924,-87.314796819803,113.419833474304));
#46614=CARTESIAN_POINT('Ctrl Pts',(-34.1285971493736,-90.3486733091506,
113.261884951111));
#46615=CARTESIAN_POINT('Ctrl Pts',(-37.2983343658999,-91.0432355319833,
113.103936427919));
#46616=CARTESIAN_POINT('Ctrl Pts',(-39.6127119772464,-88.7687450450135,
112.945987904727));
#46617=CARTESIAN_POINT('Ctrl Pts',(-38.9733541918185,-85.5874131972758,
112.788039381534));
#46618=CARTESIAN_POINT('Ctrl Pts',(-35.9599472684757,-84.3836568192793,
112.630090858342));
#46619=CARTESIAN_POINT('Ctrl Pts',(-33.3046556159841,-86.2488852083584,
112.472142335149));
#46620=CARTESIAN_POINT('Ctrl Pts',(-33.4149514186127,-89.4919525124918,
112.314193811957));
#46621=CARTESIAN_POINT('Ctrl Pts',(-36.1908328266136,-91.1724682404558,
112.156245288764));
#46622=CARTESIAN_POINT('Ctrl Pts',(-39.1154925919688,-89.7667598922799,
111.998296765572));
#46623=CARTESIAN_POINT('Ctrl Pts',(-39.537230654937,-86.5493404745703,111.840348242379));
#46624=CARTESIAN_POINT('Ctrl Pts',(-37.0736699404075,-84.437346319972,111.682399719187));
#46625=CARTESIAN_POINT('Ctrl Pts',(-33.9584460224337,-85.345658295069,111.524451195995));
#46626=CARTESIAN_POINT('Ctrl Pts',(-33.0160376821866,-88.450737557084,111.366502672802));
#46627=CARTESIAN_POINT('Ctrl Pts',(-35.1008978997205,-90.937303175899,111.20855414961));
#46628=CARTESIAN_POINT('Ctrl Pts',(-38.3227473239418,-90.550861730339,111.050605626417));
#46629=CARTESIAN_POINT('Ctrl Pts',(-39.7604330700564,-87.6417879261526,
110.892657103225));
#46630=CARTESIAN_POINT('Ctrl Pts',(-38.1104491972429,-84.8476505058174,
110.734708580032));
#46631=CARTESIAN_POINT('Ctrl Pts',(-34.8687859011027,-84.701808889116,110.57676005684));
#46632=CARTESIAN_POINT('Ctrl Pts',(-32.9745607012825,-87.336493233079,110.418811533647));
#46633=CARTESIAN_POINT('Ctrl Pts',(-34.1452099766793,-90.3629153759288,
110.260863010455));
#46634=CARTESIAN_POINT('Ctrl Pts',(-37.3193416320017,-91.0371103998827,
110.102914487262));
#46635=CARTESIAN_POINT('Ctrl Pts',(-39.6190670342295,-88.7478061923971,
109.94496596407));
#46636=CARTESIAN_POINT('Ctrl Pts',(-38.959295100015,-85.5706452298173,109.787017440877));
#46637=CARTESIAN_POINT('Ctrl Pts',(-35.9382209845566,-84.3862627742917,
109.629068917685));
#46638=CARTESIAN_POINT('Ctrl Pts',(-33.2949606890383,-86.2685022815357,
109.471120394492));
#46639=CARTESIAN_POINT('Ctrl Pts',(-33.4260779682415,-89.5107946321496,
109.3131718713));
#46640=CARTESIAN_POINT('Ctrl Pts',(-36.2126926989021,-91.1734515584065,
109.155223348107));
#46641=CARTESIAN_POINT('Ctrl Pts',(-39.1282662078998,-89.748993422115,108.997274824915));
#46642=CARTESIAN_POINT('Ctrl Pts',(-39.5293363549431,-86.5289313866941,
108.839326301722));
#46643=CARTESIAN_POINT('Ctrl Pts',(-37.052265679111,-84.4328012741596,108.68137777853));
#46644=CARTESIAN_POINT('Ctrl Pts',(-33.9429375022266,-85.3610932914029,
108.523429255338));
#46645=CARTESIAN_POINT('Ctrl Pts',(-33.0204878377882,-88.4721681382437,
108.365480732145));
#46646=CARTESIAN_POINT('Ctrl Pts',(-35.1212681444417,-90.9452783513664,
108.207532208953));
#46647=CARTESIAN_POINT('Ctrl Pts',(-38.3405763216318,-90.5381928828679,
108.04958368576));
#46648=CARTESIAN_POINT('Ctrl Pts',(-39.7595398816501,-87.6198746588301,
107.891635162568));
#46649=CARTESIAN_POINT('Ctrl Pts',(-38.0916764098229,-84.8365395425716,
107.733686639375));
#46650=CARTESIAN_POINT('Ctrl Pts',(-34.849086852875,-84.711206823075,107.575738116183));
#46651=CARTESIAN_POINT('Ctrl Pts',(-32.9719344591821,-87.3586348573252,
107.41778959299));
#46652=CARTESIAN_POINT('Ctrl Pts',(-34.1617524920315,-90.376171545939,107.259841069798));
#46653=CARTESIAN_POINT('Ctrl Pts',(-37.3406322165325,-91.0326712072276,
107.101892546605));
#46654=CARTESIAN_POINT('Ctrl Pts',(-39.624548166087,-88.723092552193,106.943944023413));
#46655=CARTESIAN_POINT('Ctrl Pts',(-39.1710020168068,-86.6178778692287,
106.838645007951));
#46656=CARTESIAN_POINT('Ctrl Pts',(-38.5501231787021,-85.8916921494929,
106.78599550022));
#46657=CARTESIAN_POINT('Ctrl Pts',(-37.0529925008446,-90.3796877745108,
122.21400449978));
#46658=CARTESIAN_POINT('Ctrl Pts',(-37.9167722964266,-90.1487627841411,
122.161354992049));
#46659=CARTESIAN_POINT('Ctrl Pts',(-39.3825154984704,-88.7656019903875,
122.056055976587));
#46660=CARTESIAN_POINT('Ctrl Pts',(-38.8454066907797,-85.7737221871878,
121.898107453395));
#46661=CARTESIAN_POINT('Ctrl Pts',(-36.0457870354219,-84.5949255259064,
121.740158930202));
#46662=CARTESIAN_POINT('Ctrl Pts',(-33.5286011349385,-86.2913941802307,
121.58221040701));
#46663=CARTESIAN_POINT('Ctrl Pts',(-33.5729143930326,-89.3282074637777,
121.424261883817));
#46664=CARTESIAN_POINT('Ctrl Pts',(-36.140100420931,-90.950422521714,121.266313360625));
#46665=CARTESIAN_POINT('Ctrl Pts',(-38.9018156279188,-89.6879832170849,
121.108364837432));
#46666=CARTESIAN_POINT('Ctrl Pts',(-39.35446349339,-86.6851368609626,120.95041631424));
#46667=CARTESIAN_POINT('Ctrl Pts',(-37.0874636818057,-84.6646518552326,
120.792467791047));
#46668=CARTESIAN_POINT('Ctrl Pts',(-34.156322660969,-85.4583534992869,120.634519267855));
#46669=CARTESIAN_POINT('Ctrl Pts',(-33.2185746983661,-88.346658956255,120.476570744663));
#46670=CARTESIAN_POINT('Ctrl Pts',(-35.1244678457132,-90.7108089424551,
120.31862222147));
#46671=CARTESIAN_POINT('Ctrl Pts',(-38.1459767864696,-90.407310569369,120.160673698278));
#46672=CARTESIAN_POINT('Ctrl Pts',(-39.5435961043541,-87.7113317183121,
120.002725175085));
#46673=CARTESIAN_POINT('Ctrl Pts',(-38.0501445145994,-85.0672367836203,
119.844776651893));
#46674=CARTESIAN_POINT('Ctrl Pts',(-35.0196902978739,-84.8723450763404,
119.6868281287));
#46675=CARTESIAN_POINT('Ctrl Pts',(-33.1998535684004,-87.3033595391308,
119.528879605508));
#46676=CARTESIAN_POINT('Ctrl Pts',(-34.2406252117824,-90.1561530227245,
119.370931082315));
#46677=CARTESIAN_POINT('Ctrl Pts',(-37.1983691009222,-90.8441845715049,
119.212982559123));
#46678=CARTESIAN_POINT('Ctrl Pts',(-39.3913888712786,-88.7436368414631,
119.05503403593));
#46679=CARTESIAN_POINT('Ctrl Pts',(-38.8313401636184,-85.7590126054036,
118.897085512738));
#46680=CARTESIAN_POINT('Ctrl Pts',(-36.0260021232032,-84.5963798697255,
118.739136989545));
#46681=CARTESIAN_POINT('Ctrl Pts',(-33.5188894234174,-86.3098623833792,
118.581188466353));
#46682=CARTESIAN_POINT('Ctrl Pts',(-33.5831249023497,-89.345897660858,118.42323994316));
#46683=CARTESIAN_POINT('Ctrl Pts',(-36.1604682031458,-90.9518048546572,
118.265291419968));
#46684=CARTESIAN_POINT('Ctrl Pts',(-38.9141205421731,-89.6715567527695,
118.107342896775));
#46685=CARTESIAN_POINT('Ctrl Pts',(-39.3474290917744,-86.6659153726033,
117.949394373583));
#46686=CARTESIAN_POINT('Ctrl Pts',(-37.0675261687099,-84.6600043409043,
117.791445850391));
#46687=CARTESIAN_POINT('Ctrl Pts',(-34.141530413112,-85.4725221831851,117.633497327198));
#46688=CARTESIAN_POINT('Ctrl Pts',(-33.2223531864905,-88.3667836834157,
117.475548804005));
#46689=CARTESIAN_POINT('Ctrl Pts',(-35.1433845246883,-90.7186499643442,
117.317600280813));
#46690=CARTESIAN_POINT('Ctrl Pts',(-38.1628837388999,-90.3957553978212,
117.159651757621));
#46691=CARTESIAN_POINT('Ctrl Pts',(-39.5431627255114,-87.6908586669244,
117.001703234428));
#46692=CARTESIAN_POINT('Ctrl Pts',(-38.0327645066527,-85.0564073718396,
116.843754711236));
#46693=CARTESIAN_POINT('Ctrl Pts',(-35.0011212106762,-84.8809783786076,
116.685806188043));
#46694=CARTESIAN_POINT('Ctrl Pts',(-33.1969316107817,-87.3236278199592,
116.527857664851));
#46695=CARTESIAN_POINT('Ctrl Pts',(-34.2559995452469,-90.1696797372461,
116.369909141658));
#46696=CARTESIAN_POINT('Ctrl Pts',(-37.2181003279875,-90.8387054158202,
116.211960618466));
#46697=CARTESIAN_POINT('Ctrl Pts',(-39.3975872675156,-88.7241196204147,
116.054012095273));
#46698=CARTESIAN_POINT('Ctrl Pts',(-38.8183858418599,-85.743152979504,115.896063572081));
#46699=CARTESIAN_POINT('Ctrl Pts',(-36.0056403680474,-84.5985572843997,
115.738115048888));
#46700=CARTESIAN_POINT('Ctrl Pts',(-33.5095816213973,-86.3281026405484,
115.580166525696));
#46701=CARTESIAN_POINT('Ctrl Pts',(-33.593310153302,-89.3636628752742,115.422218002503));
#46702=CARTESIAN_POINT('Ctrl Pts',(-36.1809118503718,-90.9529878461426,
115.264269479311));
#46703=CARTESIAN_POINT('Ctrl Pts',(-38.9262869522217,-89.655084939201,115.106320956118));
#46704=CARTESIAN_POINT('Ctrl Pts',(-39.3402873508135,-86.6467232462409,
114.948372432926));
#46705=CARTESIAN_POINT('Ctrl Pts',(-37.0475514759973,-84.6554928190843,
114.790423909734));
#46706=CARTESIAN_POINT('Ctrl Pts',(-34.1268332150591,-85.486781725498,114.632475386541));
#46707=CARTESIAN_POINT('Ctrl Pts',(-33.2262589855613,-88.3868855965463,
114.474526863349));
#46708=CARTESIAN_POINT('Ctrl Pts',(-35.1623520516624,-90.7263684550214,
114.316578340156));
#46709=CARTESIAN_POINT('Ctrl Pts',(-38.1797157139374,-90.3840923452991,
114.158629816964));
#46710=CARTESIAN_POINT('Ctrl Pts',(-39.542598108769,-87.670388606207,114.000681293771));
#46711=CARTESIAN_POINT('Ctrl Pts',(-38.0153152189578,-85.0456898844117,
113.842732770579));
#46712=CARTESIAN_POINT('Ctrl Pts',(-34.9826079904861,-84.8897306843618,
113.684784247386));
#46713=CARTESIAN_POINT('Ctrl Pts',(-33.1941398317884,-87.3439144694579,
113.526835724194));
#46714=CARTESIAN_POINT('Ctrl Pts',(-34.2714604285556,-90.1831074423791,
113.368887201001));
#46715=CARTESIAN_POINT('Ctrl Pts',(-37.2377959609237,-90.8330996847288,
113.210938677809));
#46716=CARTESIAN_POINT('Ctrl Pts',(-39.4036602187116,-88.7045629989887,
113.052990154616));
#46717=CARTESIAN_POINT('Ctrl Pts',(-38.8053299511668,-85.7273768616027,
112.895041631424));
#46718=CARTESIAN_POINT('Ctrl Pts',(-35.9852930144797,-84.6008653963151,
112.737093108231));
#46719=CARTESIAN_POINT('Ctrl Pts',(-33.500391131598,-86.346402287405,112.579144585039));
#46720=CARTESIAN_POINT('Ctrl Pts',(-33.6036092648561,-89.3813623238255,
112.421196061847));
#46721=CARTESIAN_POINT('Ctrl Pts',(-36.2013626720665,-90.9540395446918,
112.263247538654));
#46722=CARTESIAN_POINT('Ctrl Pts',(-38.9383473460099,-89.638535344659,112.105299015462));
#46723=CARTESIAN_POINT('Ctrl Pts',(-39.3330225244481,-86.6275773726469,
111.947350492269));
#46724=CARTESIAN_POINT('Ctrl Pts',(-37.0275482265935,-84.6511096477281,
111.789401969077));
#46725=CARTESIAN_POINT('Ctrl Pts',(-34.112227880481,-85.5011353445453,111.631453445884));
#46726=CARTESIAN_POINT('Ctrl Pts',(-33.2302937784678,-88.4069620161419,
111.473504922692));
#46727=CARTESIAN_POINT('Ctrl Pts',(-35.1813687480418,-90.7339649961363,
111.315556399499));
#46728=CARTESIAN_POINT('Ctrl Pts',(-38.196472453541,-90.3723214550984,111.157607876307));
#46729=CARTESIAN_POINT('Ctrl Pts',(-39.5419020654483,-87.6499225929314,
110.999659353114));
#46730=CARTESIAN_POINT('Ctrl Pts',(-37.9977974739878,-85.0350846596649,
110.841710829922));
#46731=CARTESIAN_POINT('Ctrl Pts',(-34.964151350524,-84.8986016832643,110.68376230673));
#46732=CARTESIAN_POINT('Ctrl Pts',(-33.1914783708088,-87.3642186263104,
110.525813783537));
#46733=CARTESIAN_POINT('Ctrl Pts',(-34.2870072125833,-90.1964355973184,
110.367865260345));
#46734=CARTESIAN_POINT('Ctrl Pts',(-37.2574551930994,-90.827367601673,110.209916737152));
#46735=CARTESIAN_POINT('Ctrl Pts',(-39.4096074723959,-88.6849677902127,
110.05196821396));
#46736=CARTESIAN_POINT('Ctrl Pts',(-38.7921730297185,-85.7116848927485,
109.894019690767));
#46737=CARTESIAN_POINT('Ctrl Pts',(-35.9649609037799,-84.6033041274846,
109.736071167575));
#46738=CARTESIAN_POINT('Ctrl Pts',(-33.4913183270346,-86.3647605351813,
109.578122644382));
#46739=CARTESIAN_POINT('Ctrl Pts',(-33.6140218250344,-89.3989953467633,
109.42017412119));
#46740=CARTESIAN_POINT('Ctrl Pts',(-36.2218197987848,-90.954959763239,109.262225597997));
#46741=CARTESIAN_POINT('Ctrl Pts',(-38.9503012804293,-89.6219089469059,
109.104277074805));
#46742=CARTESIAN_POINT('Ctrl Pts',(-39.3256348008056,-86.6084779336666,
108.946328551612));
#46743=CARTESIAN_POINT('Ctrl Pts',(-37.0075174743604,-84.6468562569993,
108.78838002842));
#46744=CARTESIAN_POINT('Ctrl Pts',(-34.0977145402883,-85.5155798788835,
108.630431505227));
#46745=CARTESIAN_POINT('Ctrl Pts',(-33.2344583680801,-88.4270173992954,
108.472482982035));
#46746=CARTESIAN_POINT('Ctrl Pts',(-35.2004318364279,-90.7414284054822,
108.314534458842));
#46747=CARTESIAN_POINT('Ctrl Pts',(-38.213157366435,-90.3604655661585,108.15658593565));
#46748=CARTESIAN_POINT('Ctrl Pts',(-39.5410661928425,-87.6294154975324,
107.998637412457));
#46749=CARTESIAN_POINT('Ctrl Pts',(-37.9802293342459,-85.0246866856932,
107.840688889265));
#46750=CARTESIAN_POINT('Ctrl Pts',(-34.9457163880272,-84.9073965528478,
107.682740366073));
#46751=CARTESIAN_POINT('Ctrl Pts',(-33.1890206543715,-87.3849394249949,
107.52479184288));
#46752=CARTESIAN_POINT('Ctrl Pts',(-34.3024881965678,-90.2088411203753,
107.366843319688));
#46753=CARTESIAN_POINT('Ctrl Pts',(-37.2773795631922,-90.8232132715162,
107.208894796495));
#46754=CARTESIAN_POINT('Ctrl Pts',(-39.4147368806325,-88.661840021548,107.050946273303));
#46755=CARTESIAN_POINT('Ctrl Pts',(-38.9902947372383,-86.6917167303234,
106.945647257841));
#46756=CARTESIAN_POINT('Ctrl Pts',(-38.4092576250251,-86.0121302673448,
106.89299775011));
#46757=CARTESIAN_POINT('Ctrl Pts',(-37.0051260726587,-90.2006423906073,
122.321006749669));
#46758=CARTESIAN_POINT('Ctrl Pts',(-37.8096764711458,-89.9855519312415,
122.268357241939));
#46759=CARTESIAN_POINT('Ctrl Pts',(-39.1749136338067,-88.6972344995558,
122.163058226477));
#46760=CARTESIAN_POINT('Ctrl Pts',(-38.6746343873266,-85.9105079516534,
122.005109703285));
#46761=CARTESIAN_POINT('Ctrl Pts',(-36.0669847052535,-84.8125413999697,
121.847161180092));
#46762=CARTESIAN_POINT('Ctrl Pts',(-33.7224022900841,-86.3926831662377,
121.6892126569));
#46763=CARTESIAN_POINT('Ctrl Pts',(-33.7636769872236,-89.221262104881,121.531264133707));
#46764=CARTESIAN_POINT('Ctrl Pts',(-36.1548310201154,-90.7322418452847,
121.373315610515));
#46765=CARTESIAN_POINT('Ctrl Pts',(-38.7271753625677,-89.5563680279066,
121.215367087322));
#46766=CARTESIAN_POINT('Ctrl Pts',(-39.1487851552509,-86.7594269038251,
121.05741856413));
#46767=CARTESIAN_POINT('Ctrl Pts',(-37.0372335640824,-84.8774865935611,
120.899470040937));
#46768=CARTESIAN_POINT('Ctrl Pts',(-34.3070809390753,-85.6167641007104,
120.741521517745));
#46769=CARTESIAN_POINT('Ctrl Pts',(-33.4336343721939,-88.3070183972821,
120.583572994552));
#46770=CARTESIAN_POINT('Ctrl Pts',(-35.2088403899947,-90.5090585737361,
120.42562447136));
#46771=CARTESIAN_POINT('Ctrl Pts',(-38.0231644049252,-90.226371089894,120.267675948167));
#46772=CARTESIAN_POINT('Ctrl Pts',(-39.3249489394657,-87.7152555601897,
120.109727424975));
#46773=CARTESIAN_POINT('Ctrl Pts',(-37.933903353769,-85.2524662657136,119.951778901782));
#46774=CARTESIAN_POINT('Ctrl Pts',(-35.1112474406138,-85.0709382865273,
119.79383037859));
#46775=CARTESIAN_POINT('Ctrl Pts',(-33.4161969504678,-87.3352580411336,
119.635881855397));
#46776=CARTESIAN_POINT('Ctrl Pts',(-34.3856028623679,-89.9924354210241,
119.477933332205));
#46777=CARTESIAN_POINT('Ctrl Pts',(-37.14053419649,-90.6332886333521,119.319984809013));
#46778=CARTESIAN_POINT('Ctrl Pts',(-39.1831785592718,-88.676775501313,119.16203628582));
#46779=CARTESIAN_POINT('Ctrl Pts',(-38.6615324022017,-85.8968070061733,
119.004087762628));
#46780=CARTESIAN_POINT('Ctrl Pts',(-36.0485564448438,-84.8138960194053,
118.846139239435));
#46781=CARTESIAN_POINT('Ctrl Pts',(-33.7133565108077,-86.4098850043433,
118.688190716243));
#46782=CARTESIAN_POINT('Ctrl Pts',(-33.7731873617217,-89.2377392848093,
118.53024219305));
#46783=CARTESIAN_POINT('Ctrl Pts',(-36.1738021831143,-90.7335293916316,
118.372293669858));
#46784=CARTESIAN_POINT('Ctrl Pts',(-38.7386365286165,-89.5410679265632,
118.214345146665));
#46785=CARTESIAN_POINT('Ctrl Pts',(-39.1422331026885,-86.7415234332901,
118.056396623473));
#46786=CARTESIAN_POINT('Ctrl Pts',(-37.0186631666406,-84.8731577593791,
117.89844810028));
#46787=CARTESIAN_POINT('Ctrl Pts',(-34.2933029959367,-85.629961237683,117.740499577088));
#46788=CARTESIAN_POINT('Ctrl Pts',(-33.4371537693153,-88.3257631715166,
117.582551053895));
#46789=CARTESIAN_POINT('Ctrl Pts',(-35.226459951931,-90.5163619366043,117.424602530703));
#46790=CARTESIAN_POINT('Ctrl Pts',(-38.0389120473041,-90.2156082566802,
117.26665400751));
#46791=CARTESIAN_POINT('Ctrl Pts',(-39.3245452774186,-87.696186346327,117.108705484318));
#46792=CARTESIAN_POINT('Ctrl Pts',(-37.9177150932994,-85.2423794269058,
116.950756961126));
#46793=CARTESIAN_POINT('Ctrl Pts',(-35.0939516360802,-85.0789796030929,
116.792808437933));
#46794=CARTESIAN_POINT('Ctrl Pts',(-33.4134753515389,-87.3541365255583,
116.634859914741));
#46795=CARTESIAN_POINT('Ctrl Pts',(-34.3999229774928,-90.0050346084722,
116.476911391548));
#46796=CARTESIAN_POINT('Ctrl Pts',(-37.1589124529382,-90.6281851834776,
116.318962868356));
#46797=CARTESIAN_POINT('Ctrl Pts',(-39.1889519313604,-88.658596576485,116.161014345163));
#46798=CARTESIAN_POINT('Ctrl Pts',(-38.6494663585338,-85.8820348751248,
116.003065821971));
#46799=CARTESIAN_POINT('Ctrl Pts',(-36.0295908956283,-84.8159241287137,
115.845117298778));
#46800=CARTESIAN_POINT('Ctrl Pts',(-33.70468694495,-86.4268745267296,115.687168775586));
#46801=CARTESIAN_POINT('Ctrl Pts',(-33.7826742098215,-89.2542863381334,
115.529220252393));
#46802=CARTESIAN_POINT('Ctrl Pts',(-36.1928440090593,-90.7346312653682,
115.371271729201));
#46803=CARTESIAN_POINT('Ctrl Pts',(-38.7499686876954,-89.525725585566,115.213323206008));
#46804=CARTESIAN_POINT('Ctrl Pts',(-39.1355810710419,-86.7236473113992,
115.055374682816));
#46805=CARTESIAN_POINT('Ctrl Pts',(-37.0000581389892,-84.8689555926966,
114.897426159623));
#46806=CARTESIAN_POINT('Ctrl Pts',(-34.2796135850352,-85.6432430029069,
114.739477636431));
#46807=CARTESIAN_POINT('Ctrl Pts',(-33.4407917476692,-88.3444866960797,
114.581529113239));
#46808=CARTESIAN_POINT('Ctrl Pts',(-35.2441268752179,-90.5235511702282,
114.423580590046));
#46809=CARTESIAN_POINT('Ctrl Pts',(-38.0545898534915,-90.2047449398924,
114.265632066854));
#46810=CARTESIAN_POINT('Ctrl Pts',(-39.324019376457,-87.6771199180644,114.107683543661));
#46811=CARTESIAN_POINT('Ctrl Pts',(-37.9014623035953,-85.2323968377956,
113.949735020469));
#46812=CARTESIAN_POINT('Ctrl Pts',(-35.0767078677524,-85.0871317630744,
113.791786497276));
#46813=CARTESIAN_POINT('Ctrl Pts',(-33.4108750048845,-87.3730321191129,
113.633837974084));
#46814=CARTESIAN_POINT('Ctrl Pts',(-34.4143237077375,-90.0175415756076,
113.475889450891));
#46815=CARTESIAN_POINT('Ctrl Pts',(-37.1772575559475,-90.6229638374742,
113.317940927699));
#46816=CARTESIAN_POINT('Ctrl Pts',(-39.1946084601768,-88.6403809529641,
113.159992404506));
#46817=CARTESIAN_POINT('Ctrl Pts',(-38.6373057105151,-85.8673405259296,
113.002043881314));
#46818=CARTESIAN_POINT('Ctrl Pts',(-36.0106387604836,-84.8180739733509,
112.844095358121));
#46819=CARTESIAN_POINT('Ctrl Pts',(-33.6961266472119,-86.4439193664515,
112.686146834929));
#46820=CARTESIAN_POINT('Ctrl Pts',(-33.7922671110994,-89.2707721351592,
112.528198311736));
#46821=CARTESIAN_POINT('Ctrl Pts',(-36.2118925175195,-90.7356108489278,
112.370249788544));
#46822=CARTESIAN_POINT('Ctrl Pts',(-38.7612021000511,-89.5103107970381,
112.212301265351));
#46823=CARTESIAN_POINT('Ctrl Pts',(-39.1288143939592,-86.7058142707235,
112.054352742159));
#46824=CARTESIAN_POINT('Ctrl Pts',(-36.9814265127793,-84.8648729754841,
111.896404218966));
#46825=CARTESIAN_POINT('Ctrl Pts',(-34.2660097385283,-85.6566123940217,
111.738455695774));
#46826=CARTESIAN_POINT('Ctrl Pts',(-33.444549874749,-88.3631864751999,111.580507172581));
#46827=CARTESIAN_POINT('Ctrl Pts',(-35.261839596363,-90.5306268163736,111.422558649389));
#46828=CARTESIAN_POINT('Ctrl Pts',(-38.0701975831402,-90.1937811798578,
111.264610126197));
#46829=CARTESIAN_POINT('Ctrl Pts',(-39.3233710608401,-87.6580572597103,
111.106661603004));
#46830=CARTESIAN_POINT('Ctrl Pts',(-37.8851457507329,-85.2225188135125,
110.948713079812));
#46831=CARTESIAN_POINT('Ctrl Pts',(-35.0595167999453,-85.0953944774125,
110.790764556619));
#46832=CARTESIAN_POINT('Ctrl Pts',(-33.4083960403351,-87.391944019542,110.632816033427));
#46833=CARTESIAN_POINT('Ctrl Pts',(-34.4288044484873,-90.0299558187079,
110.474867510234));
#46834=CARTESIAN_POINT('Ctrl Pts',(-37.1955687541971,-90.6176248034632,
110.316918987042));
#46835=CARTESIAN_POINT('Ctrl Pts',(-39.2001479105622,-88.6221293880284,
110.158970463849));
#46836=CARTESIAN_POINT('Ctrl Pts',(-38.625050959422,-85.8527245556798,110.001021940657));
#46837=CARTESIAN_POINT('Ctrl Pts',(-35.9917008230032,-84.8203454806775,
109.843073417464));
#46838=CARTESIAN_POINT('Ctrl Pts',(-33.6876759650309,-86.4610187888269,
109.685124894272));
#46839=CARTESIAN_POINT('Ctrl Pts',(-33.8019656818272,-89.287196061377,109.527176371079));
#46840=CARTESIAN_POINT('Ctrl Pts',(-36.2309468986677,-90.7364679680718,
109.369227847887));
#46841=CARTESIAN_POINT('Ctrl Pts',(-38.7723363529588,-89.4948244716966,
109.211279324695));
#46842=CARTESIAN_POINT('Ctrl Pts',(-39.1219332466681,-86.6880244806394,
109.053330801502));
#46843=CARTESIAN_POINT('Ctrl Pts',(-36.9627692696098,-84.8609112398387,
108.89538227831));
#46844=CARTESIAN_POINT('Ctrl Pts',(-34.2524915783501,-85.6700664663643,
108.737433755117));
#46845=CARTESIAN_POINT('Ctrl Pts',(-33.4484288983719,-88.381866660347,108.579485231925));
#46846=CARTESIAN_POINT('Ctrl Pts',(-35.2795955284141,-90.5375784595981,
108.421536708732));
#46847=CARTESIAN_POINT('Ctrl Pts',(-38.0857384112381,-90.1827382494491,
108.26358818554));
#46848=CARTESIAN_POINT('Ctrl Pts',(-39.3225925040349,-87.6389563362348,
108.105639662347));
#46849=CARTESIAN_POINT('Ctrl Pts',(-37.8687822586688,-85.2128338288146,
107.947691139155));
#46850=CARTESIAN_POINT('Ctrl Pts',(-35.0423459231792,-85.1035862826206,
107.789742615962));
#46851=CARTESIAN_POINT('Ctrl Pts',(-33.406106849561,-87.4112439926645,107.63179409277));
#46852=CARTESIAN_POINT('Ctrl Pts',(-34.443223901104,-90.0415106948117,107.473845569577));
#46853=CARTESIAN_POINT('Ctrl Pts',(-37.2141269098517,-90.6137553358046,
107.315897046385));
#46854=CARTESIAN_POINT('Ctrl Pts',(-39.204925595178,-88.6005874909031,107.157948523193));
#46855=CARTESIAN_POINT('Ctrl Pts',(-38.8095874576699,-86.7655555914181,
107.052649507731));
#46856=CARTESIAN_POINT('Ctrl Pts',(-38.2683920713481,-86.1325683851967,
107.));
#46857=CARTESIAN_POINT('Ctrl Pts',(-38.8699208872996,-87.7667938007243,
121.112583302492));
#46858=CARTESIAN_POINT('Ctrl Pts',(-38.8718337523485,-87.4752409435295,
121.094195056371));
#46859=CARTESIAN_POINT('Ctrl Pts',(-38.8249624563278,-87.1842829363247,
121.07580681025));
#46860=CARTESIAN_POINT('Ctrl Pts',(-38.7265915912756,-86.9119270394614,
121.05741856413));
#46861=CARTESIAN_POINT('Ctrl Pts',(-38.4449346248614,-86.1321134670705,
121.004769056399));
#46862=CARTESIAN_POINT('Ctrl Pts',(-37.7410840944719,-85.5048000303158,
120.952119548668));
#46863=CARTESIAN_POINT('Ctrl Pts',(-36.934133391776,-85.3143562297967,120.899470040937));
#46864=CARTESIAN_POINT('Ctrl Pts',(-36.12718268908,-85.1239124292776,120.846820533206));
#46865=CARTESIAN_POINT('Ctrl Pts',(-35.2171318140777,-85.370338264994,120.794171025476));
#46866=CARTESIAN_POINT('Ctrl Pts',(-34.6165319487629,-85.9419268989475,
120.741521517745));
#46867=CARTESIAN_POINT('Ctrl Pts',(-34.0159320834482,-86.513515532901,120.688872010014));
#46868=CARTESIAN_POINT('Ctrl Pts',(-33.724783227821,-87.4102669650915,120.636222502283));
#46869=CARTESIAN_POINT('Ctrl Pts',(-33.8750764696409,-88.2256493772624,
120.583572994552));
#46870=CARTESIAN_POINT('Ctrl Pts',(-34.0253697114608,-89.0410317894334,
120.530923486821));
#46871=CARTESIAN_POINT('Ctrl Pts',(-34.6171050507278,-89.7750451815847,
120.478273979091));
#46872=CARTESIAN_POINT('Ctrl Pts',(-35.3820267228497,-90.09493729702,120.42562447136));
#46873=CARTESIAN_POINT('Ctrl Pts',(-36.1469483949716,-90.4148294124554,
120.372974963629));
#46874=CARTESIAN_POINT('Ctrl Pts',(-37.0850563999484,-90.3206002511747,
120.320325455898));
#46875=CARTESIAN_POINT('Ctrl Pts',(-37.7710744915269,-89.8549664155836,
120.267675948167));
#46876=CARTESIAN_POINT('Ctrl Pts',(-38.4446886453889,-89.3977517356478,
120.215978399609));
#46877=CARTESIAN_POINT('Ctrl Pts',(-38.8752465796083,-88.5824417440886,
120.16428085105));
#46878=CARTESIAN_POINT('Ctrl Pts',(-38.8765118730483,-87.7682823374696,
120.112583302492));
#46879=CARTESIAN_POINT('Ctrl Pts',(-37.1487253572165,-90.7377785423179,
122.));
#46880=CARTESIAN_POINT('Ctrl Pts',(-37.2417753655626,-90.7037404336132,
122.));
#46881=CARTESIAN_POINT('Ctrl Pts',(-37.3327602094243,-90.6649336190233,
122.));
#46882=CARTESIAN_POINT('Ctrl Pts',(-37.4214714043315,-90.6216864230573,
122.));
#46883=CARTESIAN_POINT('Ctrl Pts',(-37.5121495818684,-90.577480312229,122.));
#46884=CARTESIAN_POINT('Ctrl Pts',(-37.6004528338949,-90.5286341083678,
122.));
#46885=CARTESIAN_POINT('Ctrl Pts',(-37.6861295811054,-90.475452921536,122.));
#46886=CARTESIAN_POINT('Ctrl Pts',(-37.7685610193578,-90.4242861597104,
122.));
#46887=CARTESIAN_POINT('Ctrl Pts',(-37.8485614444594,-90.3691057247624,
122.));
#46888=CARTESIAN_POINT('Ctrl Pts',(-37.9258738297264,-90.3101533054175,
122.));
#46889=CARTESIAN_POINT('Ctrl Pts',(-37.993522166835,-90.2585699384908,122.));
#46890=CARTESIAN_POINT('Ctrl Pts',(-38.0591121832093,-90.2040979486484,
122.));
#46891=CARTESIAN_POINT('Ctrl Pts',(-38.122447070225,-90.1468865492567,122.));
#46892=CARTESIAN_POINT('Ctrl Pts',(-38.1365835575632,-90.1341168379459,
122.));
#46893=CARTESIAN_POINT('Ctrl Pts',(-38.1506103387469,-90.1212079154214,
122.));
#46894=CARTESIAN_POINT('Ctrl Pts',(-38.1645056404263,-90.1081799738368,
122.));
#46895=CARTESIAN_POINT('Ctrl Pts',(-38.2369357281125,-90.0402710523098,
122.));
#46896=CARTESIAN_POINT('Ctrl Pts',(-38.3059001283609,-89.9690402129453,
122.));
#46897=CARTESIAN_POINT('Ctrl Pts',(-38.3711588917122,-89.894778180942,122.));
#46898=CARTESIAN_POINT('Ctrl Pts',(-38.4360586404937,-89.8209246940919,
122.));
#46899=CARTESIAN_POINT('Ctrl Pts',(-38.4972938990556,-89.7440724775117,
122.));
#46900=CARTESIAN_POINT('Ctrl Pts',(-38.554585046789,-89.6644807163591,122.));
#46901=CARTESIAN_POINT('Ctrl Pts',(-38.6097479523584,-89.587845616902,122.));
#46902=CARTESIAN_POINT('Ctrl Pts',(-38.6612544977319,-89.5086699914616,
122.));
#46903=CARTESIAN_POINT('Ctrl Pts',(-38.7088102350433,-89.4271716153117,
122.));
#46904=CARTESIAN_POINT('Ctrl Pts',(-38.7287565668071,-89.3929887019389,
122.));
#46905=CARTESIAN_POINT('Ctrl Pts',(-38.7480072950061,-89.3583970589295,
122.));
#46906=CARTESIAN_POINT('Ctrl Pts',(-38.7665381094582,-89.3234124579976,
122.));
#46907=CARTESIAN_POINT('Ctrl Pts',(-38.7794206549516,-89.2990913082588,
122.));
#46908=CARTESIAN_POINT('Ctrl Pts',(-38.7919552356554,-89.2745802403039,
122.));
#46909=CARTESIAN_POINT('Ctrl Pts',(-38.8041332176979,-89.2498845474537,
122.));
#46910=CARTESIAN_POINT('Ctrl Pts',(-38.8120415511817,-89.2338472619665,
122.));
#46911=CARTESIAN_POINT('Ctrl Pts',(-38.819800609578,-89.2177295044568,122.));
#46912=CARTESIAN_POINT('Ctrl Pts',(-38.827397852521,-89.2015549139639,122.));
#46913=CARTESIAN_POINT('Ctrl Pts',(-38.8695181483044,-89.1118804701093,
122.));
#46914=CARTESIAN_POINT('Ctrl Pts',(-38.9067396123332,-89.0203224429062,
122.));
#46915=CARTESIAN_POINT('Ctrl Pts',(-38.9387709613748,-88.9271531995467,
122.));
#46916=CARTESIAN_POINT('Ctrl Pts',(-38.9686507170741,-88.840242272796,122.));
#46917=CARTESIAN_POINT('Ctrl Pts',(-38.9940140218715,-88.7519285239463,
122.));
#46918=CARTESIAN_POINT('Ctrl Pts',(-39.0145738981738,-88.6624243415515,
122.));
#46919=CARTESIAN_POINT('Ctrl Pts',(-39.0160543819306,-88.6559792887581,
122.));
#46920=CARTESIAN_POINT('Ctrl Pts',(-39.0175099363868,-88.649528062159,122.));
#46921=CARTESIAN_POINT('Ctrl Pts',(-39.0189404437644,-88.6430707407411,
122.));
#46922=CARTESIAN_POINT('Ctrl Pts',(-39.0395466647231,-88.5500540992174,
122.));
#46923=CARTESIAN_POINT('Ctrl Pts',(-39.0549598625021,-88.4557718035346,
122.));
#46924=CARTESIAN_POINT('Ctrl Pts',(-39.0652569568635,-88.3606317181991,
122.));
#46925=CARTESIAN_POINT('Ctrl Pts',(-39.0710534787644,-88.3070747079457,
122.));
#46926=CARTESIAN_POINT('Ctrl Pts',(-39.075227840788,-88.2532460633916,122.));
#46927=CARTESIAN_POINT('Ctrl Pts',(-39.0777870025032,-88.1992211791364,
122.));
#46928=CARTESIAN_POINT('Ctrl Pts',(-39.0784478860045,-88.1852696752318,
122.));
#46929=CARTESIAN_POINT('Ctrl Pts',(-39.0790009329215,-88.1713056833736,
122.));
#46930=CARTESIAN_POINT('Ctrl Pts',(-39.0794460217079,-88.1573438714348,
122.));
#46931=CARTESIAN_POINT('Ctrl Pts',(-39.0824174382877,-88.0641346944071,
122.));
#46932=CARTESIAN_POINT('Ctrl Pts',(-39.0805897017238,-87.9708672878142,
122.));
#46933=CARTESIAN_POINT('Ctrl Pts',(-39.0740977060608,-87.8779167295335,
122.));
#46934=CARTESIAN_POINT('Ctrl Pts',(-39.067594916049,-87.7848116208187,122.));
#46935=CARTESIAN_POINT('Ctrl Pts',(-39.0564119653958,-87.6920234352952,
122.));
#46936=CARTESIAN_POINT('Ctrl Pts',(-39.0406334894346,-87.5999412206982,
122.));
#46937=CARTESIAN_POINT('Ctrl Pts',(-39.0250806083283,-87.5091755637904,
122.));
#46938=CARTESIAN_POINT('Ctrl Pts',(-39.0050622117732,-87.4190949906259,
122.));
#46939=CARTESIAN_POINT('Ctrl Pts',(-38.980616331591,-87.3300972983945,122.));
#46940=CARTESIAN_POINT('Ctrl Pts',(-38.97151756715,-87.2969723288138,122.));
#46941=CARTESIAN_POINT('Ctrl Pts',(-38.9618050517351,-87.2639976908667,
122.));
#46942=CARTESIAN_POINT('Ctrl Pts',(-38.951479384889,-87.2311951618355,122.));
#46943=CARTESIAN_POINT('Ctrl Pts',(-38.9444848308163,-87.2089748959248,
122.));
#46944=CARTESIAN_POINT('Ctrl Pts',(-38.9372089088412,-87.1868336198287,
122.));
#46945=CARTESIAN_POINT('Ctrl Pts',(-38.9296516262008,-87.1647783159968,
122.));
#46946=CARTESIAN_POINT('Ctrl Pts',(-38.9251355607667,-87.1515985528445,
122.));
#46947=CARTESIAN_POINT('Ctrl Pts',(-38.920519367556,-87.1384506632302,122.));
#46948=CARTESIAN_POINT('Ctrl Pts',(-38.9158065183222,-87.125345284988,122.));
#46949=CARTESIAN_POINT('Ctrl Pts',(-38.8841747708194,-87.0373844793449,
122.));
#46950=CARTESIAN_POINT('Ctrl Pts',(-38.8481538095828,-86.9512214197519,
122.));
#46951=CARTESIAN_POINT('Ctrl Pts',(-38.8078081980317,-86.8672703477228,
122.));
#46952=CARTESIAN_POINT('Ctrl Pts',(-38.7775489893683,-86.8043070437009,
122.));
#46953=CARTESIAN_POINT('Ctrl Pts',(-38.7448561175797,-86.7425884746254,
122.));
#46954=CARTESIAN_POINT('Ctrl Pts',(-38.7097408585933,-86.6823049297191,
122.));
#46955=CARTESIAN_POINT('Ctrl Pts',(-38.696271461237,-86.659181562732,122.));
#46956=CARTESIAN_POINT('Ctrl Pts',(-38.6824455217908,-86.6362694937627,
122.));
#46957=CARTESIAN_POINT('Ctrl Pts',(-38.6682631961917,-86.6135801059869,
122.));
#46958=CARTESIAN_POINT('Ctrl Pts',(-38.6581390971867,-86.5973832131288,
122.));
#46959=CARTESIAN_POINT('Ctrl Pts',(-38.6478325520626,-86.5812987298577,
122.));
#46960=CARTESIAN_POINT('Ctrl Pts',(-38.6373536921582,-86.5653458007593,
122.));
#46961=CARTESIAN_POINT('Ctrl Pts',(-38.5901671142441,-86.4935093472977,
122.));
#46962=CARTESIAN_POINT('Ctrl Pts',(-38.5394456084747,-86.4242663429416,
122.));
#46963=CARTESIAN_POINT('Ctrl Pts',(-38.4852220660282,-86.3579687859785,
122.));
#46964=CARTESIAN_POINT('Ctrl Pts',(-38.4364256387811,-86.2983068057933,
122.));
#46965=CARTESIAN_POINT('Ctrl Pts',(-38.384792513307,-86.2410302511397,122.));
#46966=CARTESIAN_POINT('Ctrl Pts',(-38.3303261681671,-86.1864254606589,
122.));
#46967=CARTESIAN_POINT('Ctrl Pts',(-38.3112435979327,-86.1672943853717,
122.));
#46968=CARTESIAN_POINT('Ctrl Pts',(-38.2918130826719,-86.1484915580211,
122.));
#46969=CARTESIAN_POINT('Ctrl Pts',(-38.2720451973146,-86.1300214660444,
122.));
#46970=CARTESIAN_POINT('Origin',(-36.3549260746835,-87.7685555885722,114.));
#46971=CARTESIAN_POINT('Origin',(87.7685555885722,36.3549260746835,107.));
#46972=CARTESIAN_POINT('Ctrl Pts',(85.8550895919077,37.990913278059,107.));
#46973=CARTESIAN_POINT('Ctrl Pts',(85.7929520311059,37.9325192289305,107.));
#46974=CARTESIAN_POINT('Ctrl Pts',(85.7341898434987,37.870871272988,107.));
#46975=CARTESIAN_POINT('Ctrl Pts',(85.6788150093107,37.8063458857252,107.));
#46976=CARTESIAN_POINT('Ctrl Pts',(85.6220850990849,37.7402414994929,107.));
#46977=CARTESIAN_POINT('Ctrl Pts',(85.5689098861403,37.6711166406476,107.));
#46978=CARTESIAN_POINT('Ctrl Pts',(85.5193311397496,37.5993298294372,107.));
#46979=CARTESIAN_POINT('Ctrl Pts',(85.5063933542064,37.5805967545636,107.));
#46980=CARTESIAN_POINT('Ctrl Pts',(85.4937006485471,37.5616821917131,107.));
#46981=CARTESIAN_POINT('Ctrl Pts',(85.4812541404578,37.5425920787089,107.));
#46982=CARTESIAN_POINT('Ctrl Pts',(85.4710842317646,37.5269937514671,107.));
#46983=CARTESIAN_POINT('Ctrl Pts',(85.4610782527306,37.5112773132593,107.));
#46984=CARTESIAN_POINT('Ctrl Pts',(85.451245660872,37.4954605983594,107.));
#46985=CARTESIAN_POINT('Ctrl Pts',(85.4038015149672,37.4191419084113,107.));
#46986=CARTESIAN_POINT('Ctrl Pts',(85.3603409327412,37.3404158601138,107.));
#46987=CARTESIAN_POINT('Ctrl Pts',(85.3208986011901,37.2596750041506,107.));
#46988=CARTESIAN_POINT('Ctrl Pts',(85.289070121347,37.1945201665567,107.));
#46989=CARTESIAN_POINT('Ctrl Pts',(85.2598587801396,37.1280522210504,107.));
#46990=CARTESIAN_POINT('Ctrl Pts',(85.2332999634681,37.0604596404359,107.));
#46991=CARTESIAN_POINT('Ctrl Pts',(85.222698407226,37.03347852325,107.));
#46992=CARTESIAN_POINT('Ctrl Pts',(85.2125196847992,37.0063180560248,107.));
#46993=CARTESIAN_POINT('Ctrl Pts',(85.202766807445,36.9789896805406,107.));
#46994=CARTESIAN_POINT('Ctrl Pts',(85.1975258836901,36.9643041752218,107.));
#46995=CARTESIAN_POINT('Ctrl Pts',(85.1924083106982,36.9495710019478,107.));
#46996=CARTESIAN_POINT('Ctrl Pts',(85.1874185552013,36.9348044141012,107.));
#46997=CARTESIAN_POINT('Ctrl Pts',(85.1578797376145,36.8473877971847,107.));
#46998=CARTESIAN_POINT('Ctrl Pts',(85.1327763850984,36.7586900770684,107.));
#46999=CARTESIAN_POINT('Ctrl Pts',(85.1121410667902,36.6691090626677,107.));
#47000=CARTESIAN_POINT('Ctrl Pts',(85.0911842873704,36.5781325373261,107.));
#47001=CARTESIAN_POINT('Ctrl Pts',(85.0748353336161,36.4862441776303,107.));
#47002=CARTESIAN_POINT('Ctrl Pts',(85.063170145668,36.3938274894209,107.));
#47003=CARTESIAN_POINT('Ctrl Pts',(85.0515956741347,36.302129496071,107.));
#47004=CARTESIAN_POINT('Ctrl Pts',(85.044632059208,36.2099104295858,107.));
#47005=CARTESIAN_POINT('Ctrl Pts',(85.0424004276122,36.1175257080037,107.));
#47006=CARTESIAN_POINT('Ctrl Pts',(85.0412898130999,36.0715486691903,107.));
#47007=CARTESIAN_POINT('Ctrl Pts',(85.0413519548824,36.0255303886718,107.));
#47008=CARTESIAN_POINT('Ctrl Pts',(85.0426065811632,35.9795139766001,107.));
#47009=CARTESIAN_POINT('Ctrl Pts',(85.0429763592658,35.9659514824889,107.));
#47010=CARTESIAN_POINT('Ctrl Pts',(85.0434497468013,35.9523891500023,107.));
#47011=CARTESIAN_POINT('Ctrl Pts',(85.0440273052287,35.9388280828518,107.));
#47012=CARTESIAN_POINT('Ctrl Pts',(85.0446478097844,35.9242586409637,107.));
#47013=CARTESIAN_POINT('Ctrl Pts',(85.0453881505517,35.9097004462176,107.));
#47014=CARTESIAN_POINT('Ctrl Pts',(85.0462483760475,35.8951574260082,107.));
#47015=CARTESIAN_POINT('Ctrl Pts',(85.0519001792078,35.7996077265604,107.));
#47016=CARTESIAN_POINT('Ctrl Pts',(85.062724622194,35.704679743261,107.));
#47017=CARTESIAN_POINT('Ctrl Pts',(85.0787921606883,35.6107691191273,107.));
#47018=CARTESIAN_POINT('Ctrl Pts',(85.0811724830822,35.5968567478123,107.));
#47019=CARTESIAN_POINT('Ctrl Pts',(85.0836679621313,35.58296667092,107.));
#47020=CARTESIAN_POINT('Ctrl Pts',(85.0862789194279,35.5691001441169,107.));
#47021=CARTESIAN_POINT('Ctrl Pts',(85.1032245667356,35.4791035467392,107.));
#47022=CARTESIAN_POINT('Ctrl Pts',(85.1250300977973,35.3900991191957,107.));
#47023=CARTESIAN_POINT('Ctrl Pts',(85.1513929626019,35.3023191100351,107.));
#47024=CARTESIAN_POINT('Ctrl Pts',(85.1783517741502,35.2125547865366,107.));
#47025=CARTESIAN_POINT('Ctrl Pts',(85.2100764994212,35.124070164157,107.));
#47026=CARTESIAN_POINT('Ctrl Pts',(85.2462978446929,35.0371172881203,107.));
#47027=CARTESIAN_POINT('Ctrl Pts',(85.2587879482913,35.0071335748779,107.));
#47028=CARTESIAN_POINT('Ctrl Pts',(85.271813175909,34.9773320762697,107.));
#47029=CARTESIAN_POINT('Ctrl Pts',(85.285363857908,34.9477234661865,107.));
#47030=CARTESIAN_POINT('Ctrl Pts',(85.2920548932063,34.9331033714035,107.));
#47031=CARTESIAN_POINT('Ctrl Pts',(85.2988740536566,34.9185303096388,107.));
#47032=CARTESIAN_POINT('Ctrl Pts',(85.3058202343552,34.9040055884619,107.));
#47033=CARTESIAN_POINT('Ctrl Pts',(85.311314009465,34.8925179011785,107.));
#47034=CARTESIAN_POINT('Ctrl Pts',(85.3168867996743,34.8810614773674,107.));
#47035=CARTESIAN_POINT('Ctrl Pts',(85.3225334641222,34.8696458936071,107.));
#47036=CARTESIAN_POINT('Ctrl Pts',(85.3652573996406,34.7832730147196,107.));
#47037=CARTESIAN_POINT('Ctrl Pts',(85.4122721941406,34.6990984517528,107.));
#47038=CARTESIAN_POINT('Ctrl Pts',(85.4632351918275,34.617371842537,107.));
#47039=CARTESIAN_POINT('Ctrl Pts',(85.5152089048678,34.5340244036513,107.));
#47040=CARTESIAN_POINT('Ctrl Pts',(85.5712892919147,34.4532222071275,107.));
#47041=CARTESIAN_POINT('Ctrl Pts',(85.6311679130609,34.375237069139,107.));
#47042=CARTESIAN_POINT('Ctrl Pts',(85.6915333690277,34.2966178838074,107.));
#47043=CARTESIAN_POINT('Ctrl Pts',(85.7557595309992,34.2208609138809,107.));
#47044=CARTESIAN_POINT('Ctrl Pts',(85.8235797056875,34.148263938979,107.));
#47045=CARTESIAN_POINT('Ctrl Pts',(85.8605803979252,34.1086571650643,107.));
#47046=CARTESIAN_POINT('Ctrl Pts',(85.8986516547817,34.0699913632724,107.));
#47047=CARTESIAN_POINT('Ctrl Pts',(85.9377555171043,34.0323186678644,107.));
#47048=CARTESIAN_POINT('Ctrl Pts',(85.9497228887807,34.0207892914493,107.));
#47049=CARTESIAN_POINT('Ctrl Pts',(85.9617869996997,34.0093529526037,107.));
#47050=CARTESIAN_POINT('Ctrl Pts',(85.9739468248078,33.9980112077434,107.));
#47051=CARTESIAN_POINT('Ctrl Pts',(85.9844926071238,33.988174917228,107.));
#47052=CARTESIAN_POINT('Ctrl Pts',(85.9951092677648,33.9784108917292,107.));
#47053=CARTESIAN_POINT('Ctrl Pts',(86.0057870254269,33.9687281255323,107.));
#47054=CARTESIAN_POINT('Ctrl Pts',(86.0813614985429,33.9001959508192,107.));
#47055=CARTESIAN_POINT('Ctrl Pts',(86.1601126924122,33.835620120822,107.));
#47056=CARTESIAN_POINT('Ctrl Pts',(86.2417132596611,33.7752824079571,107.));
#47057=CARTESIAN_POINT('Ctrl Pts',(86.3234180225243,33.7148676499775,107.));
#47058=CARTESIAN_POINT('Ctrl Pts',(86.407980013518,33.6587010007676,107.));
#47059=CARTESIAN_POINT('Ctrl Pts',(86.4951159042006,33.6070911134787,107.));
#47060=CARTESIAN_POINT('Ctrl Pts',(86.5805195599158,33.55650721503,107.));
#47061=CARTESIAN_POINT('Ctrl Pts',(86.6683964598967,33.5103000274096,107.));
#47062=CARTESIAN_POINT('Ctrl Pts',(86.7585139289399,33.4687959635278,107.));
#47063=CARTESIAN_POINT('Ctrl Pts',(86.7988635962662,33.4502127167045,107.));
#47064=CARTESIAN_POINT('Ctrl Pts',(86.8396628450883,33.4325728773236,107.));
#47065=CARTESIAN_POINT('Ctrl Pts',(86.8808925437874,33.4159086922478,107.));
#47066=CARTESIAN_POINT('Ctrl Pts',(86.9113121896724,33.4036137052611,107.));
#47067=CARTESIAN_POINT('Ctrl Pts',(86.9419661799092,33.3918498714135,107.));
#47068=CARTESIAN_POINT('Ctrl Pts',(86.9728422455434,33.3806145099939,107.));
#47069=CARTESIAN_POINT('Ctrl Pts',(88.5623548711045,33.3857031209377,107.));
#47070=CARTESIAN_POINT('Ctrl Pts',(88.6571887453956,33.4203937757735,107.));
#47071=CARTESIAN_POINT('Ctrl Pts',(88.7499794657697,33.4600753209604,107.));
#47072=CARTESIAN_POINT('Ctrl Pts',(88.8404861096065,33.5044274043379,107.));
#47073=CARTESIAN_POINT('Ctrl Pts',(88.9322656542038,33.5494032629243,107.));
#47074=CARTESIAN_POINT('Ctrl Pts',(89.0216970916563,33.5991826598102,107.));
#47075=CARTESIAN_POINT('Ctrl Pts',(89.1084951661564,33.6534722183007,107.));
#47076=CARTESIAN_POINT('Ctrl Pts',(89.1330081756223,33.6688043609645,107.));
#47077=CARTESIAN_POINT('Ctrl Pts',(89.1573109139389,33.6844964338333,107.));
#47078=CARTESIAN_POINT('Ctrl Pts',(89.181396359504,33.7005422844173,107.));
#47079=CARTESIAN_POINT('Ctrl Pts',(89.2007259405543,33.7134197530341,107.));
#47080=CARTESIAN_POINT('Ctrl Pts',(89.2199176733195,33.7265267065963,107.));
#47081=CARTESIAN_POINT('Ctrl Pts',(89.2389486421628,33.7398461999266,107.));
#47082=CARTESIAN_POINT('Ctrl Pts',(89.3216557387194,33.7977316722863,107.));
#47083=CARTESIAN_POINT('Ctrl Pts',(89.4014079749861,33.859679295932,107.));
#47084=CARTESIAN_POINT('Ctrl Pts',(89.4779389896606,33.9253917079193,107.));
#47085=CARTESIAN_POINT('Ctrl Pts',(89.5369321760609,33.9760454799314,107.));
#47086=CARTESIAN_POINT('Ctrl Pts',(89.5940106946619,34.02893718031,107.));
#47087=CARTESIAN_POINT('Ctrl Pts',(89.6490349776499,34.0839423776965,107.));
#47088=CARTESIAN_POINT('Ctrl Pts',(89.67832371242,34.1132209534407,107.));
#47089=CARTESIAN_POINT('Ctrl Pts',(89.7070301443814,34.14309849492,107.));
#47090=CARTESIAN_POINT('Ctrl Pts',(89.7351312032978,34.1735570675531,107.));
#47091=CARTESIAN_POINT('Ctrl Pts',(89.7447672055864,34.184001473811,107.));
#47092=CARTESIAN_POINT('Ctrl Pts',(89.754331292257,34.1945134919992,107.));
#47093=CARTESIAN_POINT('Ctrl Pts',(89.7638158966534,34.2050847863686,107.));
#47094=CARTESIAN_POINT('Ctrl Pts',(89.8296130855822,34.2784206287274,107.));
#47095=CARTESIAN_POINT('Ctrl Pts',(89.8916781239792,34.3547030951306,107.));
#47096=CARTESIAN_POINT('Ctrl Pts',(89.9497672435115,34.4336536253152,107.));
#47097=CARTESIAN_POINT('Ctrl Pts',(90.007329905769,34.5118886328459,107.));
#47098=CARTESIAN_POINT('Ctrl Pts',(90.0609888233644,34.5927443469894,107.));
#47099=CARTESIAN_POINT('Ctrl Pts',(90.1104610526296,34.6759720983802,107.));
#47100=CARTESIAN_POINT('Ctrl Pts',(90.158518993482,34.7568205746472,107.));
#47101=CARTESIAN_POINT('Ctrl Pts',(90.2026264068637,34.8399081044317,107.));
#47102=CARTESIAN_POINT('Ctrl Pts',(90.2424761416749,34.9250170645243,107.));
#47103=CARTESIAN_POINT('Ctrl Pts',(90.2632805570366,34.969450036667,107.));
#47104=CARTESIAN_POINT('Ctrl Pts',(90.2829236866711,35.0144340768218,107.));
#47105=CARTESIAN_POINT('Ctrl Pts',(90.3013561304951,35.059938454011,107.));
#47106=CARTESIAN_POINT('Ctrl Pts',(90.3084142100976,35.077362812904,107.));
#47107=CARTESIAN_POINT('Ctrl Pts',(90.3152947304807,35.0948634648789,107.));
#47108=CARTESIAN_POINT('Ctrl Pts',(90.3219947560663,35.1124386758054,107.));
#47109=CARTESIAN_POINT('Ctrl Pts',(90.3272364930471,35.1261885685308,107.));
#47110=CARTESIAN_POINT('Ctrl Pts',(90.3323678538939,35.1399845970363,107.));
#47111=CARTESIAN_POINT('Ctrl Pts',(90.3373823034241,35.1538112179767,107.));
#47112=CARTESIAN_POINT('Ctrl Pts',(90.3690659930617,35.2411744198563,107.));
#47113=CARTESIAN_POINT('Ctrl Pts',(90.3961408570781,35.3298985591593,107.));
#47114=CARTESIAN_POINT('Ctrl Pts',(90.4183556395185,35.4197600827214,107.));
#47115=CARTESIAN_POINT('Ctrl Pts',(90.4233396105618,35.4399208577615,107.));
#47116=CARTESIAN_POINT('Ctrl Pts',(90.428078747987,35.4601389222423,107.));
#47117=CARTESIAN_POINT('Ctrl Pts',(90.4325698536593,35.4804118071808,107.));
#47118=CARTESIAN_POINT('Ctrl Pts',(90.4529356080426,35.5723429763467,107.));
#47119=CARTESIAN_POINT('Ctrl Pts',(90.4682051514147,35.6654017572121,107.));
#47120=CARTESIAN_POINT('Ctrl Pts',(90.4784883085329,35.7591965641434,107.));
#47121=CARTESIAN_POINT('Ctrl Pts',(90.4892221738777,35.8571023742028,107.));
#47122=CARTESIAN_POINT('Ctrl Pts',(90.4945229571543,35.9558113815426,107.));
#47123=CARTESIAN_POINT('Ctrl Pts',(90.4944581052541,36.0548635705765,107.));
#47124=CARTESIAN_POINT('Ctrl Pts',(90.4944327382416,36.0936081272758,107.));
#47125=CARTESIAN_POINT('Ctrl Pts',(90.4935858264941,36.1324049341854,107.));
#47126=CARTESIAN_POINT('Ctrl Pts',(90.4919191826006,36.1712252336368,107.));
#47127=CARTESIAN_POINT('Ctrl Pts',(90.4913861442009,36.1836410294607,107.));
#47128=CARTESIAN_POINT('Ctrl Pts',(90.4907692593077,36.196057916994,107.));
#47129=CARTESIAN_POINT('Ctrl Pts',(90.4900692890457,36.2084652868845,107.));
#47130=CARTESIAN_POINT('Ctrl Pts',(90.4848300798159,36.3013332419655,107.));
#47131=CARTESIAN_POINT('Ctrl Pts',(90.4749344507016,36.3938179603827,107.));
#47132=CARTESIAN_POINT('Ctrl Pts',(90.460505860486,36.4855478660498,107.));
#47133=CARTESIAN_POINT('Ctrl Pts',(90.4461112583523,36.5770616921485,107.));
#47134=CARTESIAN_POINT('Ctrl Pts',(90.4272046158018,36.6678252027151,107.));
#47135=CARTESIAN_POINT('Ctrl Pts',(90.4038598451766,36.757452488896,107.));
#47136=CARTESIAN_POINT('Ctrl Pts',(90.3809112220297,36.845558851013,107.));
#47137=CARTESIAN_POINT('Ctrl Pts',(90.3536733503429,36.9325680090356,107.));
#47138=CARTESIAN_POINT('Ctrl Pts',(90.3221760021516,37.0180842712926,107.));
#47139=CARTESIAN_POINT('Ctrl Pts',(90.3063345627045,37.0610942631835,107.));
#47140=CARTESIAN_POINT('Ctrl Pts',(90.2894150733447,37.1037260866538,107.));
#47141=CARTESIAN_POINT('Ctrl Pts',(90.271417904293,37.1459256105394,107.));
#47142=CARTESIAN_POINT('Ctrl Pts',(90.2658521901144,37.1589760235097,107.));
#47143=CARTESIAN_POINT('Ctrl Pts',(90.2601833926065,37.1719850712082,107.));
#47144=CARTESIAN_POINT('Ctrl Pts',(90.2544114818424,37.1849510950093,107.));
#47145=CARTESIAN_POINT('Ctrl Pts',(90.2487320287865,37.1977094217589,107.));
#47146=CARTESIAN_POINT('Ctrl Pts',(90.2429562207695,37.2104182274025,107.));
#47147=CARTESIAN_POINT('Ctrl Pts',(90.2370858474454,37.223073026501,107.));
#47148=CARTESIAN_POINT('Ctrl Pts',(90.1996060503623,37.3038684505993,107.));
#47149=CARTESIAN_POINT('Ctrl Pts',(90.1582560956766,37.3825070965564,107.));
#47150=CARTESIAN_POINT('Ctrl Pts',(90.1131056594066,37.4586413742266,107.));
#47151=CARTESIAN_POINT('Ctrl Pts',(90.0687126527172,37.5334984470951,107.));
#47152=CARTESIAN_POINT('Ctrl Pts',(90.0206451521835,37.6059351413586,107.));
#47153=CARTESIAN_POINT('Ctrl Pts',(89.9689331726878,37.6755868908959,107.));
#47154=CARTESIAN_POINT('Ctrl Pts',(89.9187987056358,37.7431138619449,107.));
#47155=CARTESIAN_POINT('Ctrl Pts',(89.8652382803223,37.8080236513692,107.));
#47156=CARTESIAN_POINT('Ctrl Pts',(89.8082515369522,37.8699437651603,107.));
#47157=CARTESIAN_POINT('Ctrl Pts',(89.7872839822743,37.8927264913663,107.));
#47158=CARTESIAN_POINT('Ctrl Pts',(89.7658523353103,37.9151040470214,107.));
#47159=CARTESIAN_POINT('Ctrl Pts',(89.7439557669509,37.9370562678499,107.));
#47160=CARTESIAN_POINT('Ctrl Pts',(89.7248783320863,37.9561821900545,107.));
#47161=CARTESIAN_POINT('Ctrl Pts',(89.7054479637193,37.9749852259363,107.));
#47162=CARTESIAN_POINT('Ctrl Pts',(89.6856747987074,37.9934602469551,107.));
#47163=CARTESIAN_POINT('Origin',(87.7685555885722,36.3549260746835,124.208423447177));
#47164=CARTESIAN_POINT('Ctrl Pts',(84.6917558532639,36.3568536987801,121.708423447177));
#47165=CARTESIAN_POINT('Ctrl Pts',(84.6908331767989,36.4801286173767,121.702019850418));
#47166=CARTESIAN_POINT('Ctrl Pts',(84.7533596868374,37.6160355665901,121.642966745928));
#47167=CARTESIAN_POINT('Ctrl Pts',(86.1660867076132,39.608464641385,121.531264133707));
#47168=CARTESIAN_POINT('Ctrl Pts',(89.6167531138159,39.4750894807855,121.373315610515));
#47169=CARTESIAN_POINT('Ctrl Pts',(91.3916432643928,36.5131478211936,121.215367087322));
#47170=CARTESIAN_POINT('Ctrl Pts',(89.8816249043036,33.4075613268254,121.05741856413));
#47171=CARTESIAN_POINT('Ctrl Pts',(86.4557338964297,32.9743531814506,120.899470040937));
#47172=CARTESIAN_POINT('Ctrl Pts',(84.8091868209017,34.9127245576495,120.783138335287));
#47173=CARTESIAN_POINT('Ctrl Pts',(84.6923091848726,36.1393663959276,120.719456137367));
#47174=CARTESIAN_POINT('Ctrl Pts',(84.6942410152602,36.3522423579965,120.708423447177));
#47175=CARTESIAN_POINT('Ctrl Pts',(84.6982769289315,36.3519105223041,121.791576552823));
#47176=CARTESIAN_POINT('Ctrl Pts',(84.7032619010314,37.0449291327262,121.755752019753));
#47177=CARTESIAN_POINT('Ctrl Pts',(85.2756494227156,38.7661195118029,121.667277978953));
#47178=CARTESIAN_POINT('Ctrl Pts',(88.1200899430042,39.9637871161453,121.526154430423));
#47179=CARTESIAN_POINT('Ctrl Pts',(90.9824825683396,38.0346656023702,121.36820590723));
#47180=CARTESIAN_POINT('Ctrl Pts',(90.9320922557558,34.5813834652293,121.210257384038));
#47181=CARTESIAN_POINT('Ctrl Pts',(88.0128424000897,32.736698135431,121.052308860845));
#47182=CARTESIAN_POINT('Ctrl Pts',(85.2379952936913,34.0051402209467,120.912748583773));
#47183=CARTESIAN_POINT('Ctrl Pts',(84.702465507281,35.6938776623451,120.825837814433));
#47184=CARTESIAN_POINT('Ctrl Pts',(84.6981142843292,36.357076956871,120.791576552823));
#47185=CARTESIAN_POINT('Ctrl Pts',(89.6820215852375,37.9909132780583,122.));
#47186=CARTESIAN_POINT('Ctrl Pts',(90.223216971559,37.3579260718367,121.947350492269));
#47187=CARTESIAN_POINT('Ctrl Pts',(90.6185540996391,35.5228930793523,121.842051476808));
#47188=CARTESIAN_POINT('Ctrl Pts',(88.6277567910025,33.5097265376366,121.684102953615));
#47189=CARTESIAN_POINT('Ctrl Pts',(85.856853152671,34.0819706116619,121.526154430423));
#47190=CARTESIAN_POINT('Ctrl Pts',(84.8197362830911,36.7122378284436,121.36820590723));
#47191=CARTESIAN_POINT('Ctrl Pts',(86.455975335501,39.0198954391445,121.210257384038));
#47192=CARTESIAN_POINT('Ctrl Pts',(89.2824118663666,38.910648012169,121.052308860845));
#47193=CARTESIAN_POINT('Ctrl Pts',(90.7362221653994,36.4845253090545,120.894360337653));
#47194=CARTESIAN_POINT('Ctrl Pts',(89.4993680181651,33.9407433017105,120.73641181446));
#47195=CARTESIAN_POINT('Ctrl Pts',(86.693224985036,33.5859030524893,120.578463291268));
#47196=CARTESIAN_POINT('Ctrl Pts',(84.8620582617521,35.7416149748606,120.420514768075));
#47197=CARTESIAN_POINT('Ctrl Pts',(85.6661209826721,38.4534153039653,120.262566244883));
#47198=CARTESIAN_POINT('Ctrl Pts',(88.3763988152143,39.2625705756491,120.10461772169));
#47199=CARTESIAN_POINT('Ctrl Pts',(90.5355629043657,37.4354572382365,119.946669198498));
#47200=CARTESIAN_POINT('Ctrl Pts',(90.1859659925477,34.6286571020984,119.788720675305));
#47201=CARTESIAN_POINT('Ctrl Pts',(87.6445764061016,33.3870135407333,119.630772152113));
#47202=CARTESIAN_POINT('Ctrl Pts',(85.2155950629905,34.8362855230027,119.472823628921));
#47203=CARTESIAN_POINT('Ctrl Pts',(85.1013053402489,37.6624629423688,119.314875105728));
#47204=CARTESIAN_POINT('Ctrl Pts',(87.4053303180094,39.3031363358758,119.156926582536));
#47205=CARTESIAN_POINT('Ctrl Pts',(90.0386805913348,38.2707572071686,118.998978059343));
#47206=CARTESIAN_POINT('Ctrl Pts',(90.6137775723734,35.5013522308546,118.841029536151));
#47207=CARTESIAN_POINT('Ctrl Pts',(88.6091983117898,33.5058567116668,118.683081012958));
#47208=CARTESIAN_POINT('Ctrl Pts',(85.8424338622364,34.09352572698,118.525132489766));
#47209=CARTESIAN_POINT('Ctrl Pts',(84.8220254010344,36.7315376632941,118.367183966573));
#47210=CARTESIAN_POINT('Ctrl Pts',(86.4731462464867,39.0280873248214,118.209235443381));
#47211=CARTESIAN_POINT('Ctrl Pts',(89.2987753441784,38.9009629821107,118.051286920188));
#47212=CARTESIAN_POINT('Ctrl Pts',(90.737000729058,36.4654244092894,117.893338396996));
#47213=CARTESIAN_POINT('Ctrl Pts',(89.4838271862048,33.9297003573102,117.735389873803));
#47214=CARTESIAN_POINT('Ctrl Pts',(86.6754690534216,33.5928547032827,117.577441350611));
#47215=CARTESIAN_POINT('Ctrl Pts',(84.8581792373272,35.7602951571421,117.419492827418));
#47216=CARTESIAN_POINT('Ctrl Pts',(85.6796391438154,38.4668693790345,117.261544304226));
#47217=CARTESIAN_POINT('Ctrl Pts',(88.3950560592406,39.2586088387336,117.103595781033));
#47218=CARTESIAN_POINT('Ctrl Pts',(90.5424440520624,37.4176674477831,116.945647257841));
#47219=CARTESIAN_POINT('Ctrl Pts',(90.1748317390413,34.6131707756633,116.787698734649));
#47220=CARTESIAN_POINT('Ctrl Pts',(87.6255220239709,33.3878706600712,116.629750211456));
#47221=CARTESIAN_POINT('Ctrl Pts',(85.2058964917554,34.8527094499973,116.471801688264));
#47222=CARTESIAN_POINT('Ctrl Pts',(85.1097560228704,37.6795623656728,116.313853165071));
#47223=CARTESIAN_POINT('Ctrl Pts',(87.4242682564739,39.3054078433001,116.155904641879));
#47224=CARTESIAN_POINT('Ctrl Pts',(90.050935343065,38.2561412361693,115.997956118686));
#47225=CARTESIAN_POINT('Ctrl Pts',(90.6082381217001,35.4831006649647,115.840007595494));
#47226=CARTESIAN_POINT('Ctrl Pts',(88.5908871125881,33.5005176773809,115.682059072301));
#47227=CARTESIAN_POINT('Ctrl Pts',(85.827953120734,34.1059399707242,115.524110549109));
#47228=CARTESIAN_POINT('Ctrl Pts',(84.8245043657124,36.750449564707,115.366162025916));
#47229=CARTESIAN_POINT('Ctrl Pts',(86.4903373151876,39.0363500395887,115.208213502724));
#47230=CARTESIAN_POINT('Ctrl Pts',(89.3150918978891,38.8910849573142,115.050264979531));
#47231=CARTESIAN_POINT('Ctrl Pts',(90.7376490447086,36.4463617499443,114.892316456339));
#47232=CARTESIAN_POINT('Ctrl Pts',(89.4682194557448,33.9187365967057,114.734367933146));
#47233=CARTESIAN_POINT('Ctrl Pts',(86.6577563313556,33.599930349796,114.576419409954));
#47234=CARTESIAN_POINT('Ctrl Pts',(84.8544211100522,35.7789949372344,114.418470886761));
#47235=CARTESIAN_POINT('Ctrl Pts',(85.6932429910294,38.4802387708443,114.260522363569));
#47236=CARTESIAN_POINT('Ctrl Pts',(88.4136876864191,39.2545262213089,114.102573840377));
#47237=CARTESIAN_POINT('Ctrl Pts',(90.5492107294969,37.3998344061804,113.944625317184));
#47238=CARTESIAN_POINT('Ctrl Pts',(90.1635983261015,34.597755986334,113.786676793992));
#47239=CARTESIAN_POINT('Ctrl Pts',(87.6064735145206,33.3888502436817,113.628728270799));
#47240=CARTESIAN_POINT('Ctrl Pts',(85.1963035899787,34.8691952478801,113.470779747607));
#47241=CARTESIAN_POINT('Ctrl Pts',(85.1183163210536,37.6966072062807,113.312831224414));
#47242=CARTESIAN_POINT('Ctrl Pts',(87.4432203926037,39.3075576880492,113.154882701222));
#47243=CARTESIAN_POINT('Ctrl Pts',(90.0630959917161,38.2414468862103,112.996934178029));
#47244=CARTESIAN_POINT('Ctrl Pts',(90.6025815925894,35.4648850404968,112.838985654837));
#47245=CARTESIAN_POINT('Ctrl Pts',(88.5725420086254,33.4952963311062,112.681037131644));
#47246=CARTESIAN_POINT('Ctrl Pts',(85.8135523897406,34.1184469385098,112.523088608452));
#47247=CARTESIAN_POINT('Ctrl Pts',(84.8271047125021,36.769345159244,112.365140085259));
#47248=CARTESIAN_POINT('Ctrl Pts',(86.5075810844117,39.0445021999939,112.207191562067));
#47249=CARTESIAN_POINT('Ctrl Pts',(89.3313446884382,38.8811023676852,112.049243038875));
#47250=CARTESIAN_POINT('Ctrl Pts',(90.7381749456975,36.4272953206904,111.891294515682));
#47251=CARTESIAN_POINT('Ctrl Pts',(89.4525416487424,33.9078732793532,111.73334599249));
#47252=CARTESIAN_POINT('Ctrl Pts',(86.6400894071501,33.6071195837937,111.575397469297));
#47253=CARTESIAN_POINT('Ctrl Pts',(84.8507831315093,35.7977184627708,111.417448946105));
#47254=CARTESIAN_POINT('Ctrl Pts',(85.7069324026425,38.4935205367586,111.259500422912));
#47255=CARTESIAN_POINT('Ctrl Pts',(88.4322927150377,39.2503240544078,111.10155189972));
#47256=CARTESIAN_POINT('Ctrl Pts',(90.5558627614894,37.3819582833603,110.943603376527));
#47257=CARTESIAN_POINT('Ctrl Pts',(90.1522661664334,34.5824136445391,110.785654853335));
#47258=CARTESIAN_POINT('Ctrl Pts',(87.5874316875858,33.3899521174758,110.627706330142));
#47259=CARTESIAN_POINT('Ctrl Pts',(85.1868167413855,34.8857423020643,110.46975780695));
#47260=CARTESIAN_POINT('Ctrl Pts',(85.1269858873624,37.7135967295509,110.311809283757));
#47261=CARTESIAN_POINT('Ctrl Pts',(87.4621859428045,39.3095857974618,110.153860760565));
#47262=CARTESIAN_POINT('Ctrl Pts',(90.0751620360126,38.226674754396,109.995912237372));
#47263=CARTESIAN_POINT('Ctrl Pts',(90.5968082201978,35.4467061147194,109.83796371418));
#47264=CARTESIAN_POINT('Ctrl Pts',(88.5541637512274,33.4901928809749,109.680015190988));
#47265=CARTESIAN_POINT('Ctrl Pts',(85.7992322738601,34.131046126596,109.522066667795));
#47266=CARTESIAN_POINT('Ctrl Pts',(84.829826311594,36.7882236446833,109.364118144603));
#47267=CARTESIAN_POINT('Ctrl Pts',(86.5248768898034,39.0525435169123,109.20616962141));
#47268=CARTESIAN_POINT('Ctrl Pts',(89.3475329498274,38.8710155284806,109.048221098218));
#47269=CARTESIAN_POINT('Ctrl Pts',(90.7385786076185,36.4082261055872,108.890272575025));
#47270=CARTESIAN_POINT('Ctrl Pts',(89.4367940058201,33.8971104460649,108.732324051833));
#47271=CARTESIAN_POINT('Ctrl Pts',(86.6224698437883,33.6144229461006,108.57437552864));
#47272=CARTESIAN_POINT('Ctrl Pts',(84.8472637351372,35.8164632397989,108.416427005448));
#47273=CARTESIAN_POINT('Ctrl Pts',(85.7207103448185,38.5067176709154,108.258478482255));
#47274=CARTESIAN_POINT('Ctrl Pts',(88.4508631164072,39.2459952267107,108.100529959063));
#47275=CARTESIAN_POINT('Ctrl Pts',(90.5624148093091,37.3640547991069,107.94258143587));
#47276=CARTESIAN_POINT('Ctrl Pts',(90.1408050081674,34.5671135666176,107.784632912678));
#47277=CARTESIAN_POINT('Ctrl Pts',(87.568460510638,33.391239618368,107.626684389485));
#47278=CARTESIAN_POINT('Ctrl Pts',(85.1773063842678,34.9022195676905,107.468735866293));
#47279=CARTESIAN_POINT('Ctrl Pts',(85.1360316483359,37.7307984124518,107.3107873431));
#47280=CARTESIAN_POINT('Ctrl Pts',(87.4806142050603,39.310940705901,107.152838819908));
#47281=CARTESIAN_POINT('Ctrl Pts',(90.08826408482,38.2129733303543,106.994890296716));
#47282=CARTESIAN_POINT('Ctrl Pts',(90.5885429349443,35.4262486362238,106.836941773523));
#47283=CARTESIAN_POINT('Ctrl Pts',(89.223305985034,34.1379297320139,106.731642758061));
#47284=CARTESIAN_POINT('Ctrl Pts',(88.4187555865468,33.9228392726483,106.678993250331));
#47285=CARTESIAN_POINT('Ctrl Pts',(89.8228871389145,38.1113513959102,122.10700224989));
#47286=CARTESIAN_POINT('Ctrl Pts',(90.4039242511275,37.4317649329314,122.054352742159));
#47287=CARTESIAN_POINT('Ctrl Pts',(90.8283653107815,35.4616404682428,121.949053726697));
#47288=CARTESIAN_POINT('Ctrl Pts',(88.6910094713799,33.3002686173985,121.791105203505));
#47289=CARTESIAN_POINT('Ctrl Pts',(85.716117428823,33.9146401598327,121.633156680312));
#47290=CARTESIAN_POINT('Ctrl Pts',(84.6026500819859,36.7385424077339,121.47520815712));
#47291=CARTESIAN_POINT('Ctrl Pts',(86.3593457928718,39.2160851732247,121.317259633928));
#47292=CARTESIAN_POINT('Ctrl Pts',(89.3938589488496,39.0987951683745,121.159311110735));
#47293=CARTESIAN_POINT('Ctrl Pts',(90.9546958650639,36.4940661464342,121.001362587542));
#47294=CARTESIAN_POINT('Ctrl Pts',(89.6267869802113,33.7630159767488,120.84341406435));
#47295=CARTESIAN_POINT('Ctrl Pts',(86.6140612888339,33.3820530954764,120.685465541158));
#47296=CARTESIAN_POINT('Ctrl Pts',(84.6480877203801,35.6964642338475,120.527517017965));
#47297=CARTESIAN_POINT('Ctrl Pts',(85.5113439365442,38.6079018993285,120.369568494773));
#47298=CARTESIAN_POINT('Ctrl Pts',(88.4211470222998,39.4766255696957,120.21161997158));
#47299=CARTESIAN_POINT('Ctrl Pts',(90.7392644690901,37.5150037893038,120.053671448388));
#47300=CARTESIAN_POINT('Ctrl Pts',(90.363930929272,34.5015726203033,119.895722925195));
#47301=CARTESIAN_POINT('Ctrl Pts',(87.6354493057437,33.1685217341956,119.737774402003));
#47302=CARTESIAN_POINT('Ctrl Pts',(85.0276511964266,34.7244862318098,119.57982587881));
#47303=CARTESIAN_POINT('Ctrl Pts',(84.904947692044,37.758721201016,119.421877355618));
#47304=CARTESIAN_POINT('Ctrl Pts',(87.3785903973958,39.5201777003541,119.263928832425));
#47305=CARTESIAN_POINT('Ctrl Pts',(90.2058026703201,38.4117968774317,119.105980309233));
#47306=CARTESIAN_POINT('Ctrl Pts',(90.8232371450967,35.4385138254036,118.94803178604));
#47307=CARTESIAN_POINT('Ctrl Pts',(88.6710847539095,33.2961139025523,118.790083262848));
#47308=CARTESIAN_POINT('Ctrl Pts',(85.7006366189604,33.9270459397144,118.632134739656));
#47309=CARTESIAN_POINT('Ctrl Pts',(84.6051077202304,36.759263057967,118.474186216463));
#47310=CARTESIAN_POINT('Ctrl Pts',(86.3777807921075,39.224880129201,118.316237693271));
#47311=CARTESIAN_POINT('Ctrl Pts',(89.4114270732902,39.0883971457029,118.158289170078));
#47312=CARTESIAN_POINT('Ctrl Pts',(90.9555317450275,36.4735590764911,118.000340646886));
#47313=CARTESIAN_POINT('Ctrl Pts',(89.6101020631707,33.7511600727872,117.842392123693));
#47314=CARTESIAN_POINT('Ctrl Pts',(86.5949982009164,33.3895165129485,117.684443600501));
#47315=CARTESIAN_POINT('Ctrl Pts',(84.6439231299071,35.7165196139242,117.526495077308));
#47316=CARTESIAN_POINT('Ctrl Pts',(85.5258572777729,38.6223464365941,117.368546554116));
#47317=CARTESIAN_POINT('Ctrl Pts',(88.4411777754528,39.4723721776031,117.210598030923));
#47318=CARTESIAN_POINT('Ctrl Pts',(90.746652193168,37.4959043499272,117.052649507731));
#47319=CARTESIAN_POINT('Ctrl Pts',(90.3519769942099,34.4849462213759,116.894700984538));
#47320=CARTESIAN_POINT('Ctrl Pts',(87.6149921779705,33.1694419529511,116.736752461346));
#47321=CARTESIAN_POINT('Ctrl Pts',(85.0172386357038,34.7421192555815,116.578803938153));
#47322=CARTESIAN_POINT('Ctrl Pts',(84.9140204970802,37.7770794497893,116.420855414961));
#47323=CARTESIAN_POINT('Ctrl Pts',(87.3989225091523,39.5226164316286,116.262906891769));
#47324=CARTESIAN_POINT('Ctrl Pts',(90.2189595924524,38.3961049077729,116.104958368576));
#47325=CARTESIAN_POINT('Ctrl Pts',(90.8172898911033,35.4189186156031,115.947009845384));
#47326=CARTESIAN_POINT('Ctrl Pts',(88.6514255207118,33.2903818192015,115.789061322191));
#47327=CARTESIAN_POINT('Ctrl Pts',(85.6850898341244,33.9403740953451,115.631112798999));
#47328=CARTESIAN_POINT('Ctrl Pts',(84.6077691813485,36.7795672158759,115.473164275806));
#47329=CARTESIAN_POINT('Ctrl Pts',(86.3962374330291,39.2337511285642,115.315215752614));
#47330=CARTESIAN_POINT('Ctrl Pts',(89.4289448191708,39.077791920405,115.157267229421));
#47331=CARTESIAN_POINT('Ctrl Pts',(90.9562277883844,36.4530930621514,114.999318706229));
#47332=CARTESIAN_POINT('Ctrl Pts',(89.5933453226959,33.7393891819747,114.841370183036));
#47333=CARTESIAN_POINT('Ctrl Pts',(86.5759815035485,33.3971130544583,114.683421659844));
#47334=CARTESIAN_POINT('Ctrl Pts',(84.6398883367908,35.7365960345636,114.525473136651));
#47335=CARTESIAN_POINT('Ctrl Pts',(85.5404626131103,38.6367000563875,114.367524613459));
#47336=CARTESIAN_POINT('Ctrl Pts',(88.4611810258964,39.4679890060191,114.209576090266));
#47337=CARTESIAN_POINT('Ctrl Pts',(90.7539170199113,37.4767584753379,114.051627567074));
#47338=CARTESIAN_POINT('Ctrl Pts',(90.3399165997945,34.4683966259736,113.893679043881));
#47339=CARTESIAN_POINT('Ctrl Pts',(87.5945413552127,33.170493651555,113.735730520689));
#47340=CARTESIAN_POINT('Ctrl Pts',(85.0069395236142,34.7598187050529,113.577781997496));
#47341=CARTESIAN_POINT('Ctrl Pts',(84.9232109873573,37.7953790975972,113.419833474304));
#47342=CARTESIAN_POINT('Ctrl Pts',(87.4192698637778,39.5249245436641,113.261884951112));
#47343=CARTESIAN_POINT('Ctrl Pts',(90.2320154838242,38.3803287890515,113.103936427919));
#47344=CARTESIAN_POINT('Ctrl Pts',(90.8112169395917,35.3993619931605,112.945987904727));
#47345=CARTESIAN_POINT('Ctrl Pts',(88.6317298867517,33.2847760878186,112.788039381534));
#47346=CARTESIAN_POINT('Ctrl Pts',(85.669628950012,33.9538018011761,112.630090858342));
#47347=CARTESIAN_POINT('Ctrl Pts',(84.6105609604868,36.7998538664292,112.472142335149));
#47348=CARTESIAN_POINT('Ctrl Pts',(86.4147506541817,39.2425034347734,112.314193811957));
#47349=CARTESIAN_POINT('Ctrl Pts',(89.4463941077727,39.0670744324199,112.156245288764));
#47350=CARTESIAN_POINT('Ctrl Pts',(90.9567924051563,36.43262300037,111.998296765572));
#47351=CARTESIAN_POINT('Ctrl Pts',(89.5765133467833,33.7277261288462,111.840348242379));
#47352=CARTESIAN_POINT('Ctrl Pts',(86.5570139755884,33.4048315455369,111.682399719187));
#47353=CARTESIAN_POINT('Ctrl Pts',(84.6359825375168,35.7566979487393,111.524451195994));
#47354=CARTESIAN_POINT('Ctrl Pts',(85.5551598119273,38.6509595994417,111.366502672802));
#47355=CARTESIAN_POINT('Ctrl Pts',(88.4811557196474,39.4634774839645,111.208554149609));
#47356=CARTESIAN_POINT('Ctrl Pts',(90.7610587612434,37.4575663479778,111.050605626417));
#47357=CARTESIAN_POINT('Ctrl Pts',(90.3277501891135,34.4519248115488,110.892657103225));
#47358=CARTESIAN_POINT('Ctrl Pts',(87.574097706924,33.171676643102,110.734708580032));
#47359=CARTESIAN_POINT('Ctrl Pts',(84.9967542721322,34.7775839203925,110.57676005684));
#47360=CARTESIAN_POINT('Ctrl Pts',(84.9325187898617,37.8136193557152,110.418811533647));
#47361=CARTESIAN_POINT('Ctrl Pts',(87.4396316199912,39.5271019584502,110.260863010455));
#47362=CARTESIAN_POINT('Ctrl Pts',(90.244969806258,38.3644691623298,110.102914487262));
#47363=CARTESIAN_POINT('Ctrl Pts',(90.8050185430291,35.3798447710928,109.94496596407));
#47364=CARTESIAN_POINT('Ctrl Pts',(88.6119986586669,33.2792969318584,109.787017440877));
#47365=CARTESIAN_POINT('Ctrl Pts',(85.6542546157362,33.9673285163827,109.629068917685));
#47366=CARTESIAN_POINT('Ctrl Pts',(84.6134829182805,36.820122148347,109.471120394492));
#47367=CARTESIAN_POINT('Ctrl Pts',(86.4333197423005,39.2511367374193,109.3131718713));
#47368=CARTESIAN_POINT('Ctrl Pts',(89.4637741167068,39.0562450202134,109.155223348107));
#47369=CARTESIAN_POINT('Ctrl Pts',(90.9572257838634,36.4121499476504,108.997274824915));
#47370=CARTESIAN_POINT('Ctrl Pts',(89.5596063937697,33.7161709572185,108.839326301722));
#47371=CARTESIAN_POINT('Ctrl Pts',(86.5380972950825,33.4126725668232,108.68137777853));
#47372=CARTESIAN_POINT('Ctrl Pts',(84.6322040501972,35.7768226788991,108.523429255338));
#47373=CARTESIAN_POINT('Ctrl Pts',(85.5699520587506,38.6651282803169,108.365480732145));
#47374=CARTESIAN_POINT('Ctrl Pts',(88.5010932369602,39.4588299765984,108.207532208953));
#47375=CARTESIAN_POINT('Ctrl Pts',(90.7680931577672,37.4383448448904,108.04958368576));
#47376=CARTESIAN_POINT('Ctrl Pts',(90.3154452832148,34.4354983723793,107.891635162568));
#47377=CARTESIAN_POINT('Ctrl Pts',(87.5537299097335,33.1730589272443,107.733686639375));
#47378=CARTESIAN_POINT('Ctrl Pts',(84.986543781475,34.7952742094795,107.575738116183));
#47379=CARTESIAN_POINT('Ctrl Pts',(84.9422304817326,37.8320873922332,107.41778959299));
#47380=CARTESIAN_POINT('Ctrl Pts',(87.4594165341921,39.5285566125487,107.259841069798));
#47381=CARTESIAN_POINT('Ctrl Pts',(90.2590364017897,38.3497590667532,107.101892546605));
#47382=CARTESIAN_POINT('Ctrl Pts',(90.7961447839457,35.3578812537963,106.943944023413));
#47383=CARTESIAN_POINT('Ctrl Pts',(89.3304018103147,33.9747188791143,106.838645007951));
#47384=CARTESIAN_POINT('Ctrl Pts',(88.4666220147327,33.7437938887448,106.78599550022));
#47385=CARTESIAN_POINT('Ctrl Pts',(89.9637526925915,38.2317895137621,122.21400449978));
#47386=CARTESIAN_POINT('Ctrl Pts',(90.5846315306959,37.505603794026,122.161354992049));
#47387=CARTESIAN_POINT('Ctrl Pts',(91.0381765219239,35.4003878571334,122.056055976587));
#47388=CARTESIAN_POINT('Ctrl Pts',(88.7542621517574,33.0908106971605,121.898107453395));
#47389=CARTESIAN_POINT('Ctrl Pts',(85.5753817049752,33.7473097080035,121.740158930202));
#47390=CARTESIAN_POINT('Ctrl Pts',(84.3855638808806,36.7648469870243,121.58221040701));
#47391=CARTESIAN_POINT('Ctrl Pts',(86.2627162502425,39.4122749073048,121.424261883817));
#47392=CARTESIAN_POINT('Ctrl Pts',(89.5053060313328,39.28694232458,121.266313360625));
#47393=CARTESIAN_POINT('Ctrl Pts',(91.1731695647284,36.5036069838139,121.108364837432));
#47394=CARTESIAN_POINT('Ctrl Pts',(89.7542059422574,33.5852886517871,120.95041631424));
#47395=CARTESIAN_POINT('Ctrl Pts',(86.5348975926318,33.1782031384635,120.792467791047));
#47396=CARTESIAN_POINT('Ctrl Pts',(84.434117179008,35.6513134928344,120.634519267855));
#47397=CARTESIAN_POINT('Ctrl Pts',(85.3565668904165,38.7623884946917,120.476570744662));
#47398=CARTESIAN_POINT('Ctrl Pts',(88.4658952293851,39.6906805637423,120.31862222147));
#47399=CARTESIAN_POINT('Ctrl Pts',(90.9429660338145,37.5945503403711,120.160673698278));
#47400=CARTESIAN_POINT('Ctrl Pts',(90.5418958659962,34.3744881385083,120.002725175085));
#47401=CARTESIAN_POINT('Ctrl Pts',(87.6263222053857,32.9500299276578,119.844776651893));
#47402=CARTESIAN_POINT('Ctrl Pts',(84.8397073298627,34.6126869406169,119.6868281287));
#47403=CARTESIAN_POINT('Ctrl Pts',(84.7085900438391,37.8549794596632,119.528879605508));
#47404=CARTESIAN_POINT('Ctrl Pts',(87.3518504767824,39.7372190648325,119.370931082315));
#47405=CARTESIAN_POINT('Ctrl Pts',(90.3729247493053,38.5528365476947,119.212982559123));
#47406=CARTESIAN_POINT('Ctrl Pts',(91.0326967178202,35.3756754199526,119.05503403593));
#47407=CARTESIAN_POINT('Ctrl Pts',(88.7329711960293,33.0863710934378,118.897085512738));
#47408=CARTESIAN_POINT('Ctrl Pts',(85.5588393756842,33.7605661524489,118.739136989545));
#47409=CARTESIAN_POINT('Ctrl Pts',(84.3881900394267,36.78698845264,118.581188466353));
#47410=CARTESIAN_POINT('Ctrl Pts',(86.2824153377281,39.4216729335805,118.42323994316));
#47411=CARTESIAN_POINT('Ctrl Pts',(89.5240788024021,39.275831309295,118.265291419968));
#47412=CARTESIAN_POINT('Ctrl Pts',(91.1740627609971,36.4816937436928,118.107342896775));
#47413=CARTESIAN_POINT('Ctrl Pts',(89.7363769401363,33.5726197882643,117.949394373583));
#47414=CARTESIAN_POINT('Ctrl Pts',(86.5145273484115,33.1861783226143,117.791445850391));
#47415=CARTESIAN_POINT('Ctrl Pts',(84.4296670224867,35.6727440707063,117.633497327198));
#47416=CARTESIAN_POINT('Ctrl Pts',(85.3720754117306,38.7778234941537,117.475548804006));
#47417=CARTESIAN_POINT('Ctrl Pts',(88.4872994916648,39.6861355164726,117.317600280813));
#47418=CARTESIAN_POINT('Ctrl Pts',(90.9508603342737,37.5741412520713,117.159651757621));
#47419=CARTESIAN_POINT('Ctrl Pts',(90.5291222493784,34.3567216670886,117.001703234428));
#47420=CARTESIAN_POINT('Ctrl Pts',(87.6044623319701,32.951013245831,116.843754711236));
#47421=CARTESIAN_POINT('Ctrl Pts',(84.8285807796521,34.6315290611657,116.685806188043));
#47422=CARTESIAN_POINT('Ctrl Pts',(84.7182849712901,37.8745965339058,116.527857664851));
#47423=CARTESIAN_POINT('Ctrl Pts',(87.3735767618306,39.7398250199571,116.369909141658));
#47424=CARTESIAN_POINT('Ctrl Pts',(90.3869838418398,38.5360685793765,116.211960618466));
#47425=CARTESIAN_POINT('Ctrl Pts',(91.0263416605067,35.3547365662415,116.054012095273));
#47426=CARTESIAN_POINT('Ctrl Pts',(88.7119639288353,33.080245961022,115.896063572081));
#47427=CARTESIAN_POINT('Ctrl Pts',(85.5422265475149,33.7748082199658,115.738115048889));
#47428=CARTESIAN_POINT('Ctrl Pts',(84.3910339969842,36.8086848670448,115.580166525696));
#47429=CARTESIAN_POINT('Ctrl Pts',(86.3021375508707,39.4311522175397,115.422218002504));
#47430=CARTESIAN_POINT('Ctrl Pts',(89.5427977404525,39.2644988834957,115.264269479311));
#47431=CARTESIAN_POINT('Ctrl Pts',(91.1748065320602,36.4598243743587,115.106320956119));
#47432=CARTESIAN_POINT('Ctrl Pts',(89.7184711896471,33.5600417672437,114.948372432926));
#47433=CARTESIAN_POINT('Ctrl Pts',(86.4942066757414,33.1942957591207,114.790423909734));
#47434=CARTESIAN_POINT('Ctrl Pts',(84.4253555635294,35.6941971318927,114.632475386541));
#47435=CARTESIAN_POINT('Ctrl Pts',(85.3876822351913,38.7931613419308,114.474526863349));
#47436=CARTESIAN_POINT('Ctrl Pts',(88.5086743653739,39.6814517907293,114.316578340156));
#47437=CARTESIAN_POINT('Ctrl Pts',(90.9586233103255,37.5536825444954,114.158629816964));
#47438=CARTESIAN_POINT('Ctrl Pts',(90.5162348734876,34.3390372656131,114.000681293771));
#47439=CARTESIAN_POINT('Ctrl Pts',(87.5826091959047,32.9521370594283,113.842732770579));
#47440=CARTESIAN_POINT('Ctrl Pts',(84.8175754572497,34.6504421622257,113.684784247386));
#47441=CARTESIAN_POINT('Ctrl Pts',(84.7281056536611,37.8941509889138,113.526835724194));
#47442=CARTESIAN_POINT('Ctrl Pts',(87.3953193349517,39.7422913992789,113.368887201001));
#47443=CARTESIAN_POINT('Ctrl Pts',(90.4009349759326,38.5192106918928,113.210938677809));
#47444=CARTESIAN_POINT('Ctrl Pts',(91.0198522865937,35.3338389458242,113.052990154616));
#47445=CARTESIAN_POINT('Ctrl Pts',(88.6909177648781,33.0742558445311,112.895041631424));
#47446=CARTESIAN_POINT('Ctrl Pts',(85.5257055102833,33.7891566638425,112.737093108231));
#47447=CARTESIAN_POINT('Ctrl Pts',(84.3940172084717,36.8303625736143,112.579144585039));
#47448=CARTESIAN_POINT('Ctrl Pts',(86.3219202239515,39.440504669553,112.421196061847));
#47449=CARTESIAN_POINT('Ctrl Pts',(89.5614435271075,39.2530464971546,112.263247538654));
#47450=CARTESIAN_POINT('Ctrl Pts',(91.1754098646149,36.4379506800496,112.105299015462));
#47451=CARTESIAN_POINT('Ctrl Pts',(89.7004850448244,33.5475789783393,111.947350492269));
#47452=CARTESIAN_POINT('Ctrl Pts',(86.4739385440265,33.2025435072801,111.789401969077));
#47453=CARTESIAN_POINT('Ctrl Pts',(84.4211819435246,35.7156774347077,111.631453445884));
#47454=CARTESIAN_POINT('Ctrl Pts',(85.403387221212,38.8083986621247,111.473504922692));
#47455=CARTESIAN_POINT('Ctrl Pts',(88.5300187242571,39.6766309135212,111.315556399499));
#47456=CARTESIAN_POINT('Ctrl Pts',(90.9662547609973,37.5331744125954,111.157607876307));
#47457=CARTESIAN_POINT('Ctrl Pts',(90.5032342117935,34.3214359785583,110.999659353114));
#47458=CARTESIAN_POINT('Ctrl Pts',(87.5607637262621,32.9534011687283,110.841710829922));
#47459=CARTESIAN_POINT('Ctrl Pts',(84.8066918028788,34.6694255387206,110.683762306729));
#47460=CARTESIAN_POINT('Ctrl Pts',(84.7380516923612,37.9136419818796,110.525813783537));
#47461=CARTESIAN_POINT('Ctrl Pts',(87.417077297178,39.7446181194386,110.367865260344));
#47462=CARTESIAN_POINT('Ctrl Pts',(90.4147775765031,38.5022635702636,110.209916737152));
#47463=CARTESIAN_POINT('Ctrl Pts',(91.0132288658605,35.3129834274662,110.051968213959));
#47464=CARTESIAN_POINT('Ctrl Pts',(88.6698335661064,33.0684009827419,109.894019690767));
#47465=CARTESIAN_POINT('Ctrl Pts',(85.5092769576124,33.8036109061693,109.736071167575));
#47466=CARTESIAN_POINT('Ctrl Pts',(84.3971395249671,36.8520206520106,109.578122644382));
#47467=CARTESIAN_POINT('Ctrl Pts',(86.3417625947976,39.4497299579264,109.42017412119));
#47468=CARTESIAN_POINT('Ctrl Pts',(89.5800152835865,39.241474511946,109.262225597997));
#47469=CARTESIAN_POINT('Ctrl Pts',(91.1758729601082,36.4160737897136,109.104277074805));
#47470=CARTESIAN_POINT('Ctrl Pts',(89.6824187817193,33.5352314683722,108.946328551612));
#47471=CARTESIAN_POINT('Ctrl Pts',(86.4537247463768,33.2109221875459,108.78838002842));
#47472=CARTESIAN_POINT('Ctrl Pts',(84.4171443652571,35.7371821179993,108.630431505227));
#47473=CARTESIAN_POINT('Ctrl Pts',(85.4191937726829,38.8235388897184,108.472482982035));
#47474=CARTESIAN_POINT('Ctrl Pts',(88.5513233575131,39.6716647264861,108.314534458842));
#47475=CARTESIAN_POINT('Ctrl Pts',(90.9737715062253,37.5126348906738,108.15658593565));
#47476=CARTESIAN_POINT('Ctrl Pts',(90.4900855582621,34.303883178141,107.998637412457));
#47477=CARTESIAN_POINT('Ctrl Pts',(87.538999308829,32.9548782361206,107.840688889265));
#47478=CARTESIAN_POINT('Ctrl Pts',(84.7957811786821,34.6883288512686,107.682740366072));
#47479=CARTESIAN_POINT('Ctrl Pts',(84.7484293151293,37.9333763720146,107.52479184288));
#47480=CARTESIAN_POINT('Ctrl Pts',(87.4382188633238,39.7461725191965,107.366843319687));
#47481=CARTESIAN_POINT('Ctrl Pts',(90.4298087187594,38.4865448031522,107.208894796495));
#47482=CARTESIAN_POINT('Ctrl Pts',(91.0037466329471,35.2895138713688,107.050946273303));
#47483=CARTESIAN_POINT('Ctrl Pts',(89.4374976355954,33.8115080262147,106.945647257841));
#47484=CARTESIAN_POINT('Ctrl Pts',(88.5144884429186,33.5647485048412,106.89299775011));
#47485=CARTESIAN_POINT('Ctrl Pts',(90.1046182462686,38.352227631614,122.321006749669));
#47486=CARTESIAN_POINT('Ctrl Pts',(90.7653388102644,37.5794426551206,122.268357241939));
#47487=CARTESIAN_POINT('Ctrl Pts',(91.2479877330663,35.3391352460239,122.163058226477));
#47488=CARTESIAN_POINT('Ctrl Pts',(88.8175148321351,32.8813527769224,122.005109703284));
#47489=CARTESIAN_POINT('Ctrl Pts',(85.4346459811273,33.5799792561743,121.847161180092));
#47490=CARTESIAN_POINT('Ctrl Pts',(84.1684776797754,36.7911515663147,121.6892126569));
#47491=CARTESIAN_POINT('Ctrl Pts',(86.1660867076132,39.608464641385,121.531264133707));
#47492=CARTESIAN_POINT('Ctrl Pts',(89.6167531138159,39.4750894807855,121.373315610515));
#47493=CARTESIAN_POINT('Ctrl Pts',(91.3916432643928,36.5131478211936,121.215367087322));
#47494=CARTESIAN_POINT('Ctrl Pts',(89.8816249043036,33.4075613268254,121.05741856413));
#47495=CARTESIAN_POINT('Ctrl Pts',(86.4557338964297,32.9743531814506,120.899470040937));
#47496=CARTESIAN_POINT('Ctrl Pts',(84.220146637636,35.6061627518213,120.741521517745));
#47497=CARTESIAN_POINT('Ctrl Pts',(85.2017898442886,38.9168750900549,120.583572994552));
#47498=CARTESIAN_POINT('Ctrl Pts',(88.5106434364707,39.9047355577889,120.42562447136));
#47499=CARTESIAN_POINT('Ctrl Pts',(91.146667598539,37.6740968914383,120.267675948167));
#47500=CARTESIAN_POINT('Ctrl Pts',(90.7198608027206,34.2474036567132,120.109727424975));
#47501=CARTESIAN_POINT('Ctrl Pts',(87.6171951050278,32.7315381211201,119.951778901782));
#47502=CARTESIAN_POINT('Ctrl Pts',(84.6517634632988,34.5008876494239,119.79383037859));
#47503=CARTESIAN_POINT('Ctrl Pts',(84.5122323956342,37.9512377183104,119.635881855397));
#47504=CARTESIAN_POINT('Ctrl Pts',(87.325110556169,39.9542604293109,119.477933332205));
#47505=CARTESIAN_POINT('Ctrl Pts',(90.5400468282905,38.6938762179578,119.319984809012));
#47506=CARTESIAN_POINT('Ctrl Pts',(91.2421562905436,35.3128370145015,119.16203628582));
#47507=CARTESIAN_POINT('Ctrl Pts',(88.7948576381488,32.8766282843233,119.004087762628));
#47508=CARTESIAN_POINT('Ctrl Pts',(85.4170421324083,33.5940863651833,118.846139239435));
#47509=CARTESIAN_POINT('Ctrl Pts',(84.1712723586227,36.814713847313,118.688190716243));
#47510=CARTESIAN_POINT('Ctrl Pts',(86.1870498833489,39.6184657379601,118.53024219305));
#47511=CARTESIAN_POINT('Ctrl Pts',(89.6367305315139,39.4632654728871,118.372293669858));
#47512=CARTESIAN_POINT('Ctrl Pts',(91.3925937769666,36.4898284108945,118.214345146665));
#47513=CARTESIAN_POINT('Ctrl Pts',(89.8626518171021,33.3940795037413,118.056396623473));
#47514=CARTESIAN_POINT('Ctrl Pts',(86.4340564959065,32.9828401322801,117.89844810028));
#47515=CARTESIAN_POINT('Ctrl Pts',(84.2154109150663,35.6289685274884,117.740499577088));
#47516=CARTESIAN_POINT('Ctrl Pts',(85.2182935456883,38.9333005517133,117.582551053896));
#47517=CARTESIAN_POINT('Ctrl Pts',(88.5334212078769,39.8998988553421,117.424602530703));
#47518=CARTESIAN_POINT('Ctrl Pts',(91.1550684753794,37.6523781542154,117.266654007511));
#47519=CARTESIAN_POINT('Ctrl Pts',(90.7062675045469,34.2284971128012,117.108705484318));
#47520=CARTESIAN_POINT('Ctrl Pts',(87.5939324859696,32.7325845387109,116.950756961126));
#47521=CARTESIAN_POINT('Ctrl Pts',(84.6399229236004,34.5209388667498,116.792808437933));
#47522=CARTESIAN_POINT('Ctrl Pts',(84.5225494454999,37.9721136180223,116.634859914741));
#47523=CARTESIAN_POINT('Ctrl Pts',(87.3482310145089,39.9570336082856,116.476911391548));
#47524=CARTESIAN_POINT('Ctrl Pts',(90.5550080912271,38.6760322509801,116.318962868356));
#47525=CARTESIAN_POINT('Ctrl Pts',(91.2353934299102,35.2905545168799,116.161014345163));
#47526=CARTESIAN_POINT('Ctrl Pts',(88.7725023369588,32.8701101028426,116.003065821971));
#47527=CARTESIAN_POINT('Ctrl Pts',(85.3993632609055,33.6092423445867,115.845117298778));
#47528=CARTESIAN_POINT('Ctrl Pts',(84.1742988126201,36.8378025182137,115.687168775586));
#47529=CARTESIAN_POINT('Ctrl Pts',(86.2080376687123,39.6285533065152,115.529220252393));
#47530=CARTESIAN_POINT('Ctrl Pts',(89.6566506617342,39.4512058465864,115.371271729201));
#47531=CARTESIAN_POINT('Ctrl Pts',(91.3933852757362,36.4665556865659,115.213323206008));
#47532=CARTESIAN_POINT('Ctrl Pts',(89.843597056598,33.3806943525127,115.055374682816));
#47533=CARTESIAN_POINT('Ctrl Pts',(86.4124318479345,32.9914784637831,114.897426159623));
#47534=CARTESIAN_POINT('Ctrl Pts',(84.2108227902679,35.6517982292218,114.739477636431));
#47535=CARTESIAN_POINT('Ctrl Pts',(85.2349018572721,38.949622627474,114.581529113238));
#47536=CARTESIAN_POINT('Ctrl Pts',(88.5561677048511,39.8949145754395,114.423580590046));
#47537=CARTESIAN_POINT('Ctrl Pts',(91.1633296007399,37.630606613653,114.265632066854));
#47538=CARTESIAN_POINT('Ctrl Pts',(90.6925531471805,34.2096779052527,114.107683543661));
#47539=CARTESIAN_POINT('Ctrl Pts',(87.5706770365969,32.7337804673015,113.949735020469));
#47540=CARTESIAN_POINT('Ctrl Pts',(84.6282113908853,34.5410656193985,113.791786497276));
#47541=CARTESIAN_POINT('Ctrl Pts',(84.5330003199649,37.9929228802303,113.633837974084));
#47542=CARTESIAN_POINT('Ctrl Pts',(87.3713688061258,39.9596582548938,113.475889450891));
#47543=CARTESIAN_POINT('Ctrl Pts',(90.5698544680408,38.6580925947341,113.317940927699));
#47544=CARTESIAN_POINT('Ctrl Pts',(91.2284876335959,35.2683158984878,113.159992404506));
#47545=CARTESIAN_POINT('Ctrl Pts',(88.7501056430045,32.8637356012436,113.002043881314));
#47546=CARTESIAN_POINT('Ctrl Pts',(85.3817820705547,33.6245115265088,112.844095358121));
#47547=CARTESIAN_POINT('Ctrl Pts',(84.1774734564564,36.8608712807994,112.686146834929));
#47548=CARTESIAN_POINT('Ctrl Pts',(86.2290897937213,39.6385059043325,112.528198311736));
#47549=CARTESIAN_POINT('Ctrl Pts',(89.6764929464422,39.4390185618894,112.370249788544));
#47550=CARTESIAN_POINT('Ctrl Pts',(91.3940273240736,36.4432783597291,112.212301265351));
#47551=CARTESIAN_POINT('Ctrl Pts',(89.8244567428654,33.3674318278324,112.054352742159));
#47552=CARTESIAN_POINT('Ctrl Pts',(86.3908631124647,33.0002554690232,111.896404218966));
#47553=CARTESIAN_POINT('Ctrl Pts',(84.2063813495323,35.6746569206761,111.738455695774));
#47554=CARTESIAN_POINT('Ctrl Pts',(85.2516146304968,38.9658377248078,111.580507172581));
#47555=CARTESIAN_POINT('Ctrl Pts',(88.5788817288668,39.8897843430778,111.422558649389));
#47556=CARTESIAN_POINT('Ctrl Pts',(91.1714507607514,37.608782477213,111.264610126197));
#47557=CARTESIAN_POINT('Ctrl Pts',(90.6787182344735,34.1909471455679,111.106661603004));
#47558=CARTESIAN_POINT('Ctrl Pts',(87.5474297456003,32.7351256943546,110.948713079812));
#47559=CARTESIAN_POINT('Ctrl Pts',(84.6166293336255,34.5612671570488,110.790764556619));
#47560=CARTESIAN_POINT('Ctrl Pts',(84.5435845948607,38.0136646080439,110.632816033427));
#47561=CARTESIAN_POINT('Ctrl Pts',(87.3945229743647,39.962134280427,110.474867510234));
#47562=CARTESIAN_POINT('Ctrl Pts',(90.5845853467483,38.6400579781975,110.316918987042));
#47563=CARTESIAN_POINT('Ctrl Pts',(91.2214391886919,35.2461220838395,110.158970463849));
#47564=CARTESIAN_POINT('Ctrl Pts',(88.7276684735458,32.8575050336255,110.001021940657));
#47565=CARTESIAN_POINT('Ctrl Pts',(85.3642992994886,33.6398932959559,109.843073417464));
#47566=CARTESIAN_POINT('Ctrl Pts',(84.1807961316536,36.8839191556743,109.685124894272));
#47567=CARTESIAN_POINT('Ctrl Pts',(86.2502054472947,39.6483231784334,109.527176371079));
#47568=CARTESIAN_POINT('Ctrl Pts',(89.696256450466,39.4267040036787,109.369227847887));
#47569=CARTESIAN_POINT('Ctrl Pts',(91.3945201363532,36.4199976317768,109.211279324695));
#47570=CARTESIAN_POINT('Ctrl Pts',(89.805231169669,33.3542919795258,109.053330801502));
#47571=CARTESIAN_POINT('Ctrl Pts',(86.3693521976711,33.0091718082685,108.89538227831));
#47572=CARTESIAN_POINT('Ctrl Pts',(84.202084680317,35.6975415570995,108.737433755117));
#47573=CARTESIAN_POINT('Ctrl Pts',(85.268435486615,38.9819494991199,108.579485231925));
#47574=CARTESIAN_POINT('Ctrl Pts',(88.6015534780661,39.8844994763739,108.421536708732));
#47575=CARTESIAN_POINT('Ctrl Pts',(91.1794498546833,37.5869249364573,108.26358818554));
#47576=CARTESIAN_POINT('Ctrl Pts',(90.6647258333095,34.1722679839027,108.105639662347));
#47577=CARTESIAN_POINT('Ctrl Pts',(87.5242687079243,32.736697544997,107.947691139155));
#47578=CARTESIAN_POINT('Ctrl Pts',(84.6050185758893,34.5813834930577,107.789742615962));
#47579=CARTESIAN_POINT('Ctrl Pts',(84.5546281485259,38.034665351796,107.63179409277));
#47580=CARTESIAN_POINT('Ctrl Pts',(87.4170211924556,39.9637884258442,107.473845569577));
#47581=CARTESIAN_POINT('Ctrl Pts',(90.6005810357291,38.6233305395511,107.315897046385));
#47582=CARTESIAN_POINT('Ctrl Pts',(91.2113484819485,35.2211464889414,107.157948523192));
#47583=CARTESIAN_POINT('Ctrl Pts',(89.5445934608762,33.6482971733151,107.052649507731));
#47584=CARTESIAN_POINT('Ctrl Pts',(88.5623548711045,33.3857031209377,107.));
#47585=CARTESIAN_POINT('Ctrl Pts',(89.6820215852375,37.9909132780583,122.));
#47586=CARTESIAN_POINT('Ctrl Pts',(89.7436297460741,37.9330167349015,122.));
#47587=CARTESIAN_POINT('Ctrl Pts',(89.8018687515423,37.8719694294382,122.));
#47588=CARTESIAN_POINT('Ctrl Pts',(89.8567409894119,37.8081561811477,122.));
#47589=CARTESIAN_POINT('Ctrl Pts',(89.9130661596494,37.7426532563005,122.));
#47590=CARTESIAN_POINT('Ctrl Pts',(89.9658443450239,37.6742355418645,122.));
#47591=CARTESIAN_POINT('Ctrl Pts',(90.0150526202045,37.603270691292,122.));
#47592=CARTESIAN_POINT('Ctrl Pts',(90.0656105084705,37.5303595198906,122.));
#47593=CARTESIAN_POINT('Ctrl Pts',(90.11240051315,37.4547590216188,122.));
#47594=CARTESIAN_POINT('Ctrl Pts',(90.1553637025152,37.3768249585536,122.));
#47595=CARTESIAN_POINT('Ctrl Pts',(90.1742736966932,37.3425227407573,122.));
#47596=CARTESIAN_POINT('Ctrl Pts',(90.1924418495419,37.307767950786,122.));
#47597=CARTESIAN_POINT('Ctrl Pts',(90.2098607109953,37.2725888463926,122.));
#47598=CARTESIAN_POINT('Ctrl Pts',(90.2197915565536,37.2525325267792,122.));
#47599=CARTESIAN_POINT('Ctrl Pts',(90.2294788262591,37.2323382684758,122.));
#47600=CARTESIAN_POINT('Ctrl Pts',(90.2389209052051,37.2120111595686,122.));
#47601=CARTESIAN_POINT('Ctrl Pts',(90.2474264863267,37.1937001631485,122.));
#47602=CARTESIAN_POINT('Ctrl Pts',(90.2557354768874,37.1752756345613,122.));
#47603=CARTESIAN_POINT('Ctrl Pts',(90.26383303591,37.1567730478507,122.));
#47604=CARTESIAN_POINT('Ctrl Pts',(90.3003946147543,37.0732313557234,122.));
#47605=CARTESIAN_POINT('Ctrl Pts',(90.3326960157527,36.9880061197598,122.));
#47606=CARTESIAN_POINT('Ctrl Pts',(90.3607122049495,36.9014961187041,122.));
#47607=CARTESIAN_POINT('Ctrl Pts',(90.3891914944112,36.8135561300035,122.));
#47608=CARTESIAN_POINT('Ctrl Pts',(90.4132432276989,36.7242877964807,122.));
#47609=CARTESIAN_POINT('Ctrl Pts',(90.4328020337916,36.6340728762632,122.));
#47610=CARTESIAN_POINT('Ctrl Pts',(90.4517704842742,36.5465809690975,122.));
#47611=CARTESIAN_POINT('Ctrl Pts',(90.4665132964625,36.4581978383469,122.));
#47612=CARTESIAN_POINT('Ctrl Pts',(90.4769300991962,36.369249841242,122.));
#47613=CARTESIAN_POINT('Ctrl Pts',(90.4812989257395,36.3319448849463,122.));
#47614=CARTESIAN_POINT('Ctrl Pts',(90.4849063004385,36.2945403777073,122.));
#47615=CARTESIAN_POINT('Ctrl Pts',(90.4877424838587,36.2570597773456,122.));
#47616=CARTESIAN_POINT('Ctrl Pts',(90.489521604424,36.2335484252839,122.));
#47617=CARTESIAN_POINT('Ctrl Pts',(90.4909972347691,36.210007125288,122.));
#47618=CARTESIAN_POINT('Ctrl Pts',(90.4921666748232,36.1864416347799,122.));
#47619=CARTESIAN_POINT('Ctrl Pts',(90.4928510541084,36.1726506469527,122.));
#47620=CARTESIAN_POINT('Ctrl Pts',(90.4934302788315,36.1588563208053,122.));
#47621=CARTESIAN_POINT('Ctrl Pts',(90.4939038482032,36.1450676472443,122.));
#47622=CARTESIAN_POINT('Ctrl Pts',(90.497231204613,36.0481867379194,122.));
#47623=CARTESIAN_POINT('Ctrl Pts',(90.4953526498791,35.9514708375007,122.));
#47624=CARTESIAN_POINT('Ctrl Pts',(90.4882038039179,35.8553397140996,122.));
#47625=CARTESIAN_POINT('Ctrl Pts',(90.4810549579567,35.7592085906985,122.));
#47626=CARTESIAN_POINT('Ctrl Pts',(90.4686362510781,35.6636612002769,122.));
#47627=CARTESIAN_POINT('Ctrl Pts',(90.4508308402664,35.5690985254714,122.));
#47628=CARTESIAN_POINT('Ctrl Pts',(90.4337728060187,35.4785050894403,122.));
#47629=CARTESIAN_POINT('Ctrl Pts',(90.4117709197647,35.388814468969,122.));
#47630=CARTESIAN_POINT('Ctrl Pts',(90.3850997898583,35.3002660026689,122.));
#47631=CARTESIAN_POINT('Ctrl Pts',(90.3762304376694,35.2708196486464,122.));
#47632=CARTESIAN_POINT('Ctrl Pts',(90.3668443009283,35.2414996371044,122.));
#47633=CARTESIAN_POINT('Ctrl Pts',(90.3569502297067,35.2123149441589,122.));
#47634=CARTESIAN_POINT('Ctrl Pts',(90.3476298672125,35.184822528606,122.));
#47635=CARTESIAN_POINT('Ctrl Pts',(90.3378587614969,35.1574501926698,122.));
#47636=CARTESIAN_POINT('Ctrl Pts',(90.3276438359507,35.1302055647186,122.));
#47637=CARTESIAN_POINT('Ctrl Pts',(90.3224861204142,35.1164492196299,122.));
#47638=CARTESIAN_POINT('Ctrl Pts',(90.3172183296157,35.1027337076298,122.));
#47639=CARTESIAN_POINT('Ctrl Pts',(90.3118431330481,35.0890633460052,122.));
#47640=CARTESIAN_POINT('Ctrl Pts',(90.2775918092556,35.0019543488783,122.));
#47641=CARTESIAN_POINT('Ctrl Pts',(90.2389669873983,34.9166341728923,122.));
#47642=CARTESIAN_POINT('Ctrl Pts',(90.1962986524644,34.8333372319883,122.));
#47643=CARTESIAN_POINT('Ctrl Pts',(90.1520688572906,34.7469920150849,122.));
#47644=CARTESIAN_POINT('Ctrl Pts',(90.103494057027,34.6628200939995,122.));
#47645=CARTESIAN_POINT('Ctrl Pts',(90.0508859614636,34.581086046773,122.));
#47646=CARTESIAN_POINT('Ctrl Pts',(89.9977149201083,34.498477384386,122.));
#47647=CARTESIAN_POINT('Ctrl Pts',(89.940423388037,34.4183582274894,122.));
#47648=CARTESIAN_POINT('Ctrl Pts',(89.8792816811015,34.3410171035127,122.));
#47649=CARTESIAN_POINT('Ctrl Pts',(89.8565927777255,34.3123168042104,122.));
#47650=CARTESIAN_POINT('Ctrl Pts',(89.8333732098606,34.2839992699063,122.));
#47651=CARTESIAN_POINT('Ctrl Pts',(89.8096351963912,34.2560801327903,122.));
#47652=CARTESIAN_POINT('Ctrl Pts',(89.7888795976702,34.2316687216432,122.));
#47653=CARTESIAN_POINT('Ctrl Pts',(89.7677276292938,34.2075618935548,122.));
#47654=CARTESIAN_POINT('Ctrl Pts',(89.7461869693122,34.1837704808018,122.));
#47655=CARTESIAN_POINT('Ctrl Pts',(89.734423948481,34.1707783587378,122.));
#47656=CARTESIAN_POINT('Ctrl Pts',(89.7225496929772,34.1578855474185,122.));
#47657=CARTESIAN_POINT('Ctrl Pts',(89.7105715260522,34.1450996670866,122.));
#47658=CARTESIAN_POINT('Ctrl Pts',(89.6415607698904,34.0714353680812,122.));
#47659=CARTESIAN_POINT('Ctrl Pts',(89.5690476160887,34.0012556015445,122.));
#47660=CARTESIAN_POINT('Ctrl Pts',(89.4933405847835,33.9348515807767,122.));
#47661=CARTESIAN_POINT('Ctrl Pts',(89.4311464894629,33.8803000031212,122.));
#47662=CARTESIAN_POINT('Ctrl Pts',(89.3667958219628,33.8282966578679,122.));
#47663=CARTESIAN_POINT('Ctrl Pts',(89.3004373490015,33.7790163342467,122.));
#47664=CARTESIAN_POINT('Ctrl Pts',(89.275819727738,33.7607343532348,122.));
#47665=CARTESIAN_POINT('Ctrl Pts',(89.2509256000565,33.7428272754375,122.));
#47666=CARTESIAN_POINT('Ctrl Pts',(89.2257619544786,33.7253045897815,122.));
#47667=CARTESIAN_POINT('Ctrl Pts',(89.2089511913507,33.7135984275319,122.));
#47668=CARTESIAN_POINT('Ctrl Pts',(89.1920190055838,33.7020631898191,122.));
#47669=CARTESIAN_POINT('Ctrl Pts',(89.174982541295,33.6907115289679,122.));
#47670=CARTESIAN_POINT('Ctrl Pts',(89.0900720965275,33.634134380366,122.));
#47671=CARTESIAN_POINT('Ctrl Pts',(89.0024923712921,33.5820565285997,122.));
#47672=CARTESIAN_POINT('Ctrl Pts',(88.9125337222617,33.5347858885666,122.));
#47673=CARTESIAN_POINT('Ctrl Pts',(88.8290756905137,33.4909311328633,122.));
#47674=CARTESIAN_POINT('Ctrl Pts',(88.7435693133768,33.4512136598047,122.));
#47675=CARTESIAN_POINT('Ctrl Pts',(88.6562187308696,33.4159083934617,122.));
#47676=CARTESIAN_POINT('Ctrl Pts',(88.6257885601688,33.4036091591507,122.));
#47677=CARTESIAN_POINT('Ctrl Pts',(88.5951343684732,33.3918456830543,122.));
#47678=CARTESIAN_POINT('Ctrl Pts',(88.5642690620869,33.3806142427251,122.));
#47679=CARTESIAN_POINT('Ctrl Pts',(85.2503883725927,36.3527278457068,120.387416697508));
#47680=CARTESIAN_POINT('Ctrl Pts',(85.2488060127422,36.178361411834,120.398449387697));
#47681=CARTESIAN_POINT('Ctrl Pts',(85.2653916078632,36.0042940232439,120.409482077886));
#47682=CARTESIAN_POINT('Ctrl Pts',(85.3012631691194,35.8342963759829,120.420514768075));
#47683=CARTESIAN_POINT('Ctrl Pts',(85.4724471695134,35.0230443340702,120.473164275806));
#47684=CARTESIAN_POINT('Ctrl Pts',(86.0828360772747,34.3044736932798,120.525813783537));
#47685=CARTESIAN_POINT('Ctrl Pts',(86.8557210366768,34.0043284144214,120.578463291268));
#47686=CARTESIAN_POINT('Ctrl Pts',(87.628605996079,33.704183135563,120.631112798999));
#47687=CARTESIAN_POINT('Ctrl Pts',(88.563987007122,33.8224632186368,120.683762306729));
#47688=CARTESIAN_POINT('Ctrl Pts',(89.2378198705159,34.3055669280643,120.73641181446));
#47689=CARTESIAN_POINT('Ctrl Pts',(89.9116527339098,34.7886706374918,120.789061322191));
#47690=CARTESIAN_POINT('Ctrl Pts',(90.3239374496546,35.6365979732731,120.841710829922));
#47691=CARTESIAN_POINT('Ctrl Pts',(90.2877780910216,36.4649154250162,120.894360337653));
#47692=CARTESIAN_POINT('Ctrl Pts',(90.2516187323885,37.2932328767593,120.947009845383));
#47693=CARTESIAN_POINT('Ctrl Pts',(89.7670152993775,38.1019404444642,120.999659353114));
#47694=CARTESIAN_POINT('Ctrl Pts',(89.0536408277278,38.5245021328125,121.052308860845));
#47695=CARTESIAN_POINT('Ctrl Pts',(88.3402663560781,38.9470638211609,121.104958368576));
#47696=CARTESIAN_POINT('Ctrl Pts',(87.3981208457895,38.9834796301527,121.157607876307));
#47697=CARTESIAN_POINT('Ctrl Pts',(86.6543415819103,38.6170779328651,121.210257384038));
#47698=CARTESIAN_POINT('Ctrl Pts',(85.9105623180311,38.2506762355775,121.262906891768));
#47699=CARTESIAN_POINT('Ctrl Pts',(85.3651493005611,37.4814570320105,121.315556399499));
#47700=CARTESIAN_POINT('Ctrl Pts',(85.2652956034228,36.6584695607634,121.36820590723));
#47701=CARTESIAN_POINT('Ctrl Pts',(85.2531507071272,36.5583721404652,121.374609503989));
#47702=CARTESIAN_POINT('Ctrl Pts',(85.2475970163779,36.4574793205693,121.381013100749));
#47703=CARTESIAN_POINT('Ctrl Pts',(85.2483527795145,36.3565049891663,121.387416697508));
#47704=CARTESIAN_POINT('Ctrl Pts',(86.9747563060389,33.385703120938,122.));
#47705=CARTESIAN_POINT('Ctrl Pts',(85.9925177162673,33.6482971733158,121.947350492269));
#47706=CARTESIAN_POINT('Ctrl Pts',(84.3257620656596,35.2211421325034,121.842051476808));
#47707=CARTESIAN_POINT('Ctrl Pts',(84.9365306847115,38.623331668768,121.684102953615));
#47708=CARTESIAN_POINT('Ctrl Pts',(88.1200899430042,39.9637871161453,121.526154430423));
#47709=CARTESIAN_POINT('Ctrl Pts',(90.9824825683396,38.0346656023702,121.36820590723));
#47710=CARTESIAN_POINT('Ctrl Pts',(90.9320922557558,34.5813834652293,121.210257384038));
#47711=CARTESIAN_POINT('Ctrl Pts',(88.0128424000897,32.736698135431,121.052308860845));
#47712=CARTESIAN_POINT('Ctrl Pts',(84.8723857333594,34.1722681870687,120.894360337653));
#47713=CARTESIAN_POINT('Ctrl Pts',(84.3576617369607,37.5869248191736,120.73641181446));
#47714=CARTESIAN_POINT('Ctrl Pts',(86.9355578127517,39.8844990120122,120.578463291268));
#47715=CARTESIAN_POINT('Ctrl Pts',(90.2686753707106,38.9819491786592,120.420514768075));
#47716=CARTESIAN_POINT('Ctrl Pts',(91.3350260504491,35.6975416344974,120.262566244883));
#47717=CARTESIAN_POINT('Ctrl Pts',(89.1677588017562,33.0091722323982,120.10461772169));
#47718=CARTESIAN_POINT('Ctrl Pts',(85.7318802647753,33.3542923559705,119.946669198498));
#47719=CARTESIAN_POINT('Ctrl Pts',(84.1425914969864,36.4199976243217,119.788720675305));
#47720=CARTESIAN_POINT('Ctrl Pts',(85.8408549696731,39.426703616461,119.630772152113));
#47721=CARTESIAN_POINT('Ctrl Pts',(89.286905538518,39.6483227638767,119.472823628921));
#47722=CARTESIAN_POINT('Ctrl Pts',(91.3563145937352,36.8839190889564,119.314875105728));
#47723=CARTESIAN_POINT('Ctrl Pts',(90.1728115748451,33.639893637919,119.156926582536));
#47724=CARTESIAN_POINT('Ctrl Pts',(86.8094428243991,32.8575054740432,118.998978059343));
#47725=CARTESIAN_POINT('Ctrl Pts',(84.3156724232774,35.2461222234895,118.841029536151));
#47726=CARTESIAN_POINT('Ctrl Pts',(84.9525261850344,38.6400576904171,118.683081012958));
#47727=CARTESIAN_POINT('Ctrl Pts',(88.1425881556754,39.9621338261614,118.525132489766));
#47728=CARTESIAN_POINT('Ctrl Pts',(90.9935261761534,38.0136643991501,118.367183966573));
#47729=CARTESIAN_POINT('Ctrl Pts',(90.9204814465843,34.5612673829304,118.209235443381));
#47730=CARTESIAN_POINT('Ctrl Pts',(87.989681403696,32.7351261502086,118.051286920188));
#47731=CARTESIAN_POINT('Ctrl Pts',(84.8583933091573,34.1909474180868,117.893338396996));
#47732=CARTESIAN_POINT('Ctrl Pts',(84.3656608449326,37.6087823193115,117.735389873803));
#47733=CARTESIAN_POINT('Ctrl Pts',(86.9582295503262,39.8897838979207,117.577441350611));
#47734=CARTESIAN_POINT('Ctrl Pts',(90.2854962296813,38.9658373960053,117.419492827418));
#47735=CARTESIAN_POINT('Ctrl Pts',(91.3307293790144,35.6746570063435,117.261544304226));
#47736=CARTESIAN_POINT('Ctrl Pts',(89.1462478911809,33.0002558914885,117.103595781033));
#47737=CARTESIAN_POINT('Ctrl Pts',(85.712654693185,33.367432204059,116.945647257841));
#47738=CARTESIAN_POINT('Ctrl Pts',(84.1430843096398,36.443278348604,116.787698734649));
#47739=CARTESIAN_POINT('Ctrl Pts',(85.8606184709768,39.4390181734991,116.629750211456));
#47740=CARTESIAN_POINT('Ctrl Pts',(89.3080211895539,39.6385054908189,116.471801688264));
#47741=CARTESIAN_POINT('Ctrl Pts',(91.3596372684504,36.8608712170826,116.313853165071));
#47742=CARTESIAN_POINT('Ctrl Pts',(90.1553288060137,33.6245118703589,116.155904641879));
#47743=CARTESIAN_POINT('Ctrl Pts',(86.7870056577489,32.8637360409022,115.997956118686));
#47744=CARTESIAN_POINT('Ctrl Pts',(84.30862397927,35.2683160353299,115.840007595494));
#47745=CARTESIAN_POINT('Ctrl Pts',(84.9672570618822,38.6580923046891,115.682059072301));
#47746=CARTESIAN_POINT('Ctrl Pts',(88.1657423210009,39.9596578009367,115.524110549109));
#47747=CARTESIAN_POINT('Ctrl Pts',(91.0041104497151,37.9929226739502,115.366162025916));
#47748=CARTESIAN_POINT('Ctrl Pts',(90.9088993907837,34.5410658478232,115.208213502724));
#47749=CARTESIAN_POINT('Ctrl Pts',(87.9664341156267,32.7337809233254,115.050264979531));
#47750=CARTESIAN_POINT('Ctrl Pts',(84.8445583981927,34.2096781754126,114.892316456339));
#47751=CARTESIAN_POINT('Ctrl Pts',(84.3737820039213,37.6306064530032,114.734367933146));
#47752=CARTESIAN_POINT('Ctrl Pts',(86.9809435714815,39.8949141296362,114.576419409954));
#47753=CARTESIAN_POINT('Ctrl Pts',(90.3022090008012,38.9496223007136,114.418470886762));
#47754=CARTESIAN_POINT('Ctrl Pts',(91.3262879388381,35.6517983177679,114.260522363569));
#47755=CARTESIAN_POINT('Ctrl Pts',(89.1246791584273,32.9914788873536,114.102573840377));
#47756=CARTESIAN_POINT('Ctrl Pts',(85.6935143818628,33.3806947270693,113.944625317184));
#47757=CARTESIAN_POINT('Ctrl Pts',(84.1437263578963,36.4665556725093,113.786676793992));
#47758=CARTESIAN_POINT('Ctrl Pts',(85.880460753186,39.4512054566615,113.628728270799));
#47759=CARTESIAN_POINT('Ctrl Pts',(89.3290733119119,39.6285528942548,113.470779747607));
#47760=CARTESIAN_POINT('Ctrl Pts',(91.3628119118867,36.837802457402,113.312831224414));
#47761=CARTESIAN_POINT('Ctrl Pts',(90.1377476178771,33.6092426903596,113.154882701222));
#47762=CARTESIAN_POINT('Ctrl Pts',(86.7646089666149,32.8701105416984,112.996934178029));
#47763=CARTESIAN_POINT('Ctrl Pts',(84.3017181838254,35.2905546509213,112.838985654837));
#47764=CARTESIAN_POINT('Ctrl Pts',(84.9821034368262,38.6760319586759,112.681037131644));
#47765=CARTESIAN_POINT('Ctrl Pts',(88.188880109704,39.957033154659,112.523088608452));
#47766=CARTESIAN_POINT('Ctrl Pts',(91.0145613228638,37.9721134143629,112.365140085259));
#47767=CARTESIAN_POINT('Ctrl Pts',(90.8971878595435,34.5209390977093,112.207191562067));
#47768=CARTESIAN_POINT('Ctrl Pts',(87.9431786691826,32.7325849948854,112.049243038874));
#47769=CARTESIAN_POINT('Ctrl Pts',(84.8308440425533,34.2284973805913,111.891294515682));
#47770=CARTESIAN_POINT('Ctrl Pts',(84.3820431282414,37.6523779908239,111.73334599249));
#47771=CARTESIAN_POINT('Ctrl Pts',(87.0036900655912,39.8998984089112,111.575397469297));
#47772=CARTESIAN_POINT('Ctrl Pts',(90.3188173102936,38.9333002270083,111.417448946105));
#47773=CARTESIAN_POINT('Ctrl Pts',(91.3216998146175,35.6289686189096,111.259500422912));
#47774=CARTESIAN_POINT('Ctrl Pts',(89.1030545131784,32.9828405569386,111.10155189972));
#47775=CARTESIAN_POINT('Ctrl Pts',(85.6744596237584,33.3940798766124,110.943603376527));
#47776=CARTESIAN_POINT('Ctrl Pts',(84.1445178565661,36.4898283939069,110.785654853335));
#47777=CARTESIAN_POINT('Ctrl Pts',(85.9003808808979,39.463265081444,110.627706330142));
#47778=CARTESIAN_POINT('Ctrl Pts',(89.3500610946321,39.6184653269691,110.46975780695));
#47779=CARTESIAN_POINT('Ctrl Pts',(91.365838365503,36.8147137894109,110.311809283757));
#47780=CARTESIAN_POINT('Ctrl Pts',(90.1200687486007,33.5940867128609,110.153860760565));
#47781=CARTESIAN_POINT('Ctrl Pts',(86.7422536682402,32.8766287223663,109.995912237372));
#47782=CARTESIAN_POINT('Ctrl Pts',(84.2949553240436,35.3128371457212,109.83796371418));
#47783=CARTESIAN_POINT('Ctrl Pts',(84.9970646978785,38.6938759234372,109.680015190987));
#47784=CARTESIAN_POINT('Ctrl Pts',(88.2120005651333,39.9542599759734,109.522066667795));
#47785=CARTESIAN_POINT('Ctrl Pts',(91.0248783714271,37.9512375173972,109.364118144602));
#47786=CARTESIAN_POINT('Ctrl Pts',(90.8853473213453,34.5008878826802,109.20616962141));
#47787=CARTESIAN_POINT('Ctrl Pts',(87.9199160530301,32.731538577869,109.048221098218));
#47788=CARTESIAN_POINT('Ctrl Pts',(84.8172507461507,34.247403921267,108.890272575025));
#47789=CARTESIAN_POINT('Ctrl Pts',(84.3904440038818,37.6740967269575,108.732324051833));
#47790=CARTESIAN_POINT('Ctrl Pts',(87.0264678344641,39.9047351075969,108.57437552864));
#47791=CARTESIAN_POINT('Ctrl Pts',(90.3353210088379,38.9168747734219,108.416427005448));
#47792=CARTESIAN_POINT('Ctrl Pts',(91.3169640944224,35.6061628347523,108.258478482255));
#47793=CARTESIAN_POINT('Ctrl Pts',(89.0813771113567,32.9743536285202,108.100529959063));
#47794=CARTESIAN_POINT('Ctrl Pts',(85.6554865479944,33.4075616582705,107.94258143587));
#47795=CARTESIAN_POINT('Ctrl Pts',(84.1454683488411,36.5131478744096,107.784632912678));
#47796=CARTESIAN_POINT('Ctrl Pts',(85.920358340807,39.4750889550508,107.626684389485));
#47797=CARTESIAN_POINT('Ctrl Pts',(89.3710241690437,39.6084644686119,107.468735866293));
#47798=CARTESIAN_POINT('Ctrl Pts',(91.3686332599885,36.7911510990924,107.3107873431));
#47799=CARTESIAN_POINT('Ctrl Pts',(90.1024644197946,33.5799803118859,107.152838819908));
#47800=CARTESIAN_POINT('Ctrl Pts',(86.7195974323738,32.8813521540788,106.994890296716));
#47801=CARTESIAN_POINT('Ctrl Pts',(84.2891204576078,35.33913847958,106.836941773523));
#47802=CARTESIAN_POINT('Ctrl Pts',(84.7717723668806,37.5794426551218,106.731642758061));
#47803=CARTESIAN_POINT('Ctrl Pts',(85.4324929308767,38.3522276316149,106.678993250331));
#47804=CARTESIAN_POINT('Ctrl Pts',(87.0226227342249,33.5647485048415,122.10700224989));
#47805=CARTESIAN_POINT('Ctrl Pts',(86.0996135415481,33.8115080262153,122.054352742159));
#47806=CARTESIAN_POINT('Ctrl Pts',(84.5333639526222,35.2895097776259,121.949053726697));
#47807=CARTESIAN_POINT('Ctrl Pts',(85.1073029689203,38.4865458642768,121.791105203505));
#47808=CARTESIAN_POINT('Ctrl Pts',(88.0988922746495,39.746171288473,121.633156680312));
#47809=CARTESIAN_POINT('Ctrl Pts',(90.7886814294914,37.933376607479,121.47520815712));
#47810=CARTESIAN_POINT('Ctrl Pts',(90.7413296737966,34.6883288251183,121.317259633928));
#47811=CARTESIAN_POINT('Ctrl Pts',(87.9981118033538,32.9548787909513,121.159311110735));
#47812=CARTESIAN_POINT('Ctrl Pts',(85.0470259849183,34.3038833690559,121.001362587543));
#47813=CARTESIAN_POINT('Ctrl Pts',(84.5633400604243,37.5126347804625,120.84341406435));
#47814=CARTESIAN_POINT('Ctrl Pts',(86.9857879264501,39.6716642901257,120.685465541158));
#47815=CARTESIAN_POINT('Ctrl Pts',(90.117917103928,38.8235385885816,120.527517017965));
#47816=CARTESIAN_POINT('Ctrl Pts',(91.1199663924258,35.7371821907302,120.369568494773));
#47817=CARTESIAN_POINT('Ctrl Pts',(89.0833862637669,33.2109225861004,120.21161997158));
#47818=CARTESIAN_POINT('Ctrl Pts',(85.8546926372097,33.5352318221171,120.053671448388));
#47819=CARTESIAN_POINT('Ctrl Pts',(84.3612386457225,36.4160737827081,119.895722925195));
#47820=CARTESIAN_POINT('Ctrl Pts',(85.9570961219,39.2414741480778,119.737774402003));
#47821=CARTESIAN_POINT('Ctrl Pts',(89.1953484025524,39.4497295683677,119.57982587881));
#47822=CARTESIAN_POINT('Ctrl Pts',(91.1399712276629,36.8520205893159,119.421877355618));
#47823=CARTESIAN_POINT('Ctrl Pts',(90.0278339349809,33.8036112275119,119.263928832425));
#47824=CARTESIAN_POINT('Ctrl Pts',(86.8672777245543,33.0684013966023,119.105980309233));
#47825=CARTESIAN_POINT('Ctrl Pts',(84.5238827198886,35.3129835586951,118.948031786041));
#47826=CARTESIAN_POINT('Ctrl Pts',(85.1223339338948,38.5022632998365,118.790083262848));
#47827=CARTESIAN_POINT('Ctrl Pts',(88.1200338357027,39.7446176925654,118.632134739656));
#47828=CARTESIAN_POINT('Ctrl Pts',(90.7990591031426,37.9136417855822,118.474186216463));
#47829=CARTESIAN_POINT('Ctrl Pts',(90.7304190012663,34.6694257509815,118.316237693271));
#47830=CARTESIAN_POINT('Ctrl Pts',(87.9763474247134,32.9534015970941,118.158289170078));
#47831=CARTESIAN_POINT('Ctrl Pts',(85.033877309738,34.3214362346443,118.000340646886));
#47832=CARTESIAN_POINT('Ctrl Pts',(84.5708568188455,37.5331742642154,117.842392123693));
#47833=CARTESIAN_POINT('Ctrl Pts',(87.0070925487824,39.6766304952072,117.684443600501));
#47834=CARTESIAN_POINT('Ctrl Pts',(90.1337236580792,38.8083983531492,117.526495077308));
#47835=CARTESIAN_POINT('Ctrl Pts',(91.1159288120728,35.7156775152093,117.368546554116));
#47836=CARTESIAN_POINT('Ctrl Pts',(89.063172470081,33.2025439042705,117.210598030923));
#47837=CARTESIAN_POINT('Ctrl Pts',(85.836626375614,33.5475793318793,117.052649507731));
#47838=CARTESIAN_POINT('Ctrl Pts',(84.3617017415672,36.4379506695953,116.894700984538));
#47839=CARTESIAN_POINT('Ctrl Pts',(85.9756678758229,39.2530461321845,116.736752461346));
#47840=CARTESIAN_POINT('Ctrl Pts',(89.2151907710141,39.4405042809744,116.578803938153));
#47841=CARTESIAN_POINT('Ctrl Pts',(91.1430935437054,36.8303625137396,116.420855414961));
#47842=CARTESIAN_POINT('Ctrl Pts',(90.0114053844099,33.7891569869583,116.262906891768));
#47843=CARTESIAN_POINT('Ctrl Pts',(86.8461935284216,33.0742562576781,116.104958368576));
#47844=CARTESIAN_POINT('Ctrl Pts',(84.5172592999978,35.3338390744146,115.947009845384));
#47845=CARTESIAN_POINT('Ctrl Pts',(85.1361765327179,38.5192104193376,115.789061322191));
#47846=CARTESIAN_POINT('Ctrl Pts',(88.141791795191,39.7422909726956,115.631112798999));
#47847=CARTESIAN_POINT('Ctrl Pts',(90.8090051405891,37.8941507950725,115.473164275806));
#47848=CARTESIAN_POINT('Ctrl Pts',(90.7195353482665,34.6504423768763,115.315215752614));
#47849=CARTESIAN_POINT('Ctrl Pts',(87.9545019578215,32.9521374879537,115.157267229421));
#47850=CARTESIAN_POINT('Ctrl Pts',(85.0208766496814,34.3390375194823,114.999318706229));
#47851=CARTESIAN_POINT('Ctrl Pts',(84.5784882685562,37.5536823935329,114.841370183036));
#47852=CARTESIAN_POINT('Ctrl Pts',(87.0284369049777,39.6814513718082,114.683421659844));
#47853=CARTESIAN_POINT('Ctrl Pts',(90.1494286421223,38.7931610348741,114.525473136651));
#47854=CARTESIAN_POINT('Ctrl Pts',(91.1117551925935,35.6941972150994,114.367524613459));
#47855=CARTESIAN_POINT('Ctrl Pts',(89.0429043409186,33.1942961571498,114.209576090266));
#47856=CARTESIAN_POINT('Ctrl Pts',(85.8186402330563,33.5600421192143,114.051627567074));
#47857=CARTESIAN_POINT('Ctrl Pts',(84.3623050740457,36.4598243611497,113.893679043881));
#47858=CARTESIAN_POINT('Ctrl Pts',(85.9943136601298,39.2644985170834,113.735730520689));
#47859=CARTESIAN_POINT('Ctrl Pts',(89.2349734416037,39.4311518301388,113.577781997497));
#47860=CARTESIAN_POINT('Ctrl Pts',(91.1460767548168,36.8086848099001,113.419833474304));
#47861=CARTESIAN_POINT('Ctrl Pts',(89.994884349259,33.7748085448886,113.261884951112));
#47862=CARTESIAN_POINT('Ctrl Pts',(86.8251473671147,33.0802463734147,113.103936427919));
#47863=CARTESIAN_POINT('Ctrl Pts',(84.5107699269021,35.3547366922002,112.945987904727));
#47864=CARTESIAN_POINT('Ctrl Pts',(85.1501276650537,38.5360683046983,112.788039381534));
#47865=CARTESIAN_POINT('Ctrl Pts',(88.1635343655741,39.7398245936844,112.630090858342));
#47866=CARTESIAN_POINT('Ctrl Pts',(90.8188258217234,37.8745963425271,112.472142335149));
#47867=CARTESIAN_POINT('Ctrl Pts',(90.7085300272501,34.6315292781982,112.314193811957));
#47868=CARTESIAN_POINT('Ctrl Pts',(87.9326488245083,32.9510136744979,112.156245288764));
#47869=CARTESIAN_POINT('Ctrl Pts',(85.0079892754134,34.3567219187308,111.998296765572));
#47870=CARTESIAN_POINT('Ctrl Pts',(84.5862512436303,37.5741410985324,111.840348242379));
#47871=CARTESIAN_POINT('Ctrl Pts',(87.049811775995,39.6861350969617,111.682399719187));
#47872=CARTESIAN_POINT('Ctrl Pts',(90.1650354636175,38.7778231890285,111.524451195994));
#47873=CARTESIAN_POINT('Ctrl Pts',(91.1074437341793,35.6727441566147,111.366502672802));
#47874=CARTESIAN_POINT('Ctrl Pts',(89.0225836708075,33.1861787216656,111.20855414961));
#47875=CARTESIAN_POINT('Ctrl Pts',(85.8007344848218,33.5726201386511,111.050605626417));
#47876=CARTESIAN_POINT('Ctrl Pts',(84.3630488450153,36.4816937277295,110.892657103225));
#47877=CARTESIAN_POINT('Ctrl Pts',(86.0130325958229,39.275830941456,110.734708580032));
#47878=CARTESIAN_POINT('Ctrl Pts',(89.2546956522624,39.4216725473725,110.57676005684));
#47879=CARTESIAN_POINT('Ctrl Pts',(91.1489207120165,36.7869883982294,110.418811533647));
#47880=CARTESIAN_POINT('Ctrl Pts',(89.9782715231816,33.7605664791613,110.260863010455));
#47881=CARTESIAN_POINT('Ctrl Pts',(86.8041401025664,33.0863715050666,110.102914487262));
#47882=CARTESIAN_POINT('Ctrl Pts',(84.504414870389,35.3756755432596,109.94496596407));
#47883=CARTESIAN_POINT('Ctrl Pts',(85.1641867558175,38.5528362709339,109.787017440877));
#47884=CARTESIAN_POINT('Ctrl Pts',(88.1852606478871,39.7372186388315,109.629068917685));
#47885=CARTESIAN_POINT('Ctrl Pts',(90.8285207479504,37.8549792708652,109.471120394492));
#47886=CARTESIAN_POINT('Ctrl Pts',(90.6974034784492,34.6126871598077,109.3131718713));
#47887=CARTESIAN_POINT('Ctrl Pts',(87.9107889538232,32.9500303568646,109.155223348107));
#47888=CARTESIAN_POINT('Ctrl Pts',(84.9952156604596,34.3744883871094,108.997274824915));
#47889=CARTESIAN_POINT('Ctrl Pts',(84.5941455429619,37.5945501858085,108.839326301722));
#47890=CARTESIAN_POINT('Ctrl Pts',(87.071216035894,39.6906801406971,108.68137777853));
#47891=CARTESIAN_POINT('Ctrl Pts',(90.1805439822485,38.7623881971518,108.523429255338));
#47892=CARTESIAN_POINT('Ctrl Pts',(91.1029935798892,35.6513135707646,108.365480732145));
#47893=CARTESIAN_POINT('Ctrl Pts',(89.002213425367,33.1782035585746,108.207532208953));
#47894=CARTESIAN_POINT('Ctrl Pts',(85.7829054934487,33.5852889632459,108.04958368576));
#47895=CARTESIAN_POINT('Ctrl Pts',(84.3639420222092,36.503607033821,107.891635162568));
#47896=CARTESIAN_POINT('Ctrl Pts',(86.031805406558,39.2869418305473,107.733686639375));
#47897=CARTESIAN_POINT('Ctrl Pts',(89.2743946445339,39.4122747449501,107.575738116183));
#47898=CARTESIAN_POINT('Ctrl Pts',(91.1515470731975,36.7648465479756,107.41778959299));
#47899=CARTESIAN_POINT('Ctrl Pts',(89.9617287427533,33.7473107000553,107.259841069798));
#47900=CARTESIAN_POINT('Ctrl Pts',(86.7828500471828,33.0908101118746,107.101892546605));
#47901=CARTESIAN_POINT('Ctrl Pts',(84.4989318488357,35.4003908957046,106.943944023413));
#47902=CARTESIAN_POINT('Ctrl Pts',(84.952479646449,37.5056037940271,106.838645007951));
#47903=CARTESIAN_POINT('Ctrl Pts',(85.5733584845537,38.2317895137629,106.78599550022));
#47904=CARTESIAN_POINT('Ctrl Pts',(87.0704891624108,33.743793888745,122.21400449978));
#47905=CARTESIAN_POINT('Ctrl Pts',(86.2067093668289,33.9747188791149,122.161354992049));
#47906=CARTESIAN_POINT('Ctrl Pts',(84.7409658395849,35.3578774227484,122.056055976587));
#47907=CARTESIAN_POINT('Ctrl Pts',(85.2780752531291,38.3497600597857,121.898107453395));
#47908=CARTESIAN_POINT('Ctrl Pts',(88.0776946062948,39.5285554608006,121.740158930202));
#47909=CARTESIAN_POINT('Ctrl Pts',(90.5948802906431,37.8320876125879,121.58221040701));
#47910=CARTESIAN_POINT('Ctrl Pts',(90.5505670918375,34.7952741850072,121.424261883817));
#47911=CARTESIAN_POINT('Ctrl Pts',(87.9833812066179,33.1730594464715,121.266313360625));
#47912=CARTESIAN_POINT('Ctrl Pts',(85.221666236477,34.4354985510432,121.108364837432));
#47913=CARTESIAN_POINT('Ctrl Pts',(84.7690183838881,37.4383447417513,120.95041631424));
#47914=CARTESIAN_POINT('Ctrl Pts',(87.0360180401483,39.4588295682391,120.792467791047));
#47915=CARTESIAN_POINT('Ctrl Pts',(89.9671588371456,38.665127998504,120.634519267855));
#47916=CARTESIAN_POINT('Ctrl Pts',(90.9049067344024,35.7768227469628,120.476570744662));
#47917=CARTESIAN_POINT('Ctrl Pts',(88.9990137257777,33.4126729398025,120.31862222147));
#47918=CARTESIAN_POINT('Ctrl Pts',(85.977505009644,33.7161712882636,120.160673698278));
#47919=CARTESIAN_POINT('Ctrl Pts',(84.5798857944587,36.4121499410944,120.002725175085));
#47920=CARTESIAN_POINT('Ctrl Pts',(86.0733372741268,39.0562446796945,119.844776651893));
#47921=CARTESIAN_POINT('Ctrl Pts',(89.103791266587,39.2511363728585,119.6868281287));
#47922=CARTESIAN_POINT('Ctrl Pts',(90.9236278615904,36.8201220896753,119.528879605508));
#47923=CARTESIAN_POINT('Ctrl Pts',(89.8828562951167,33.9673288171048,119.370931082315));
#47924=CARTESIAN_POINT('Ctrl Pts',(86.9251126247094,33.2792973191614,119.212982559123));
#47925=CARTESIAN_POINT('Ctrl Pts',(84.7320930164998,35.3798448939008,119.05503403593));
#47926=CARTESIAN_POINT('Ctrl Pts',(85.2921416827553,38.364468909256,118.897085512738));
#47927=CARTESIAN_POINT('Ctrl Pts',(88.0974795157296,39.5271015589694,118.739136989545));
#47928=CARTESIAN_POINT('Ctrl Pts',(90.6045920301321,37.8136191720142,118.581188466353));
#47929=CARTESIAN_POINT('Ctrl Pts',(90.5403565559482,34.7775841190325,118.42323994316));
#47930=CARTESIAN_POINT('Ctrl Pts',(87.963013445731,33.1716770439797,118.265291419968));
#47931=CARTESIAN_POINT('Ctrl Pts',(85.2093613103188,34.4519250512017,118.107342896775));
#47932=CARTESIAN_POINT('Ctrl Pts',(84.7760527927585,37.4575662091194,117.949394373583));
#47933=CARTESIAN_POINT('Ctrl Pts',(87.0559555472384,39.4634770924937,117.79144585039));
#47934=CARTESIAN_POINT('Ctrl Pts',(89.9819510864773,38.6509593102931,117.633497327198));
#47935=CARTESIAN_POINT('Ctrl Pts',(90.901128245131,35.7566980240751,117.475548804005));
#47936=CARTESIAN_POINT('Ctrl Pts',(88.9800970489813,33.4048319170525,117.317600280813));
#47937=CARTESIAN_POINT('Ctrl Pts',(85.9605980580428,33.7277264596997,117.159651757621));
#47938=CARTESIAN_POINT('Ctrl Pts',(84.5803191734944,36.4326229905866,117.001703234428));
#47939=CARTESIAN_POINT('Ctrl Pts',(86.0907172806691,39.0670740908699,116.843754711236));
#47940=CARTESIAN_POINT('Ctrl Pts',(89.1223603524743,39.2425030711299,116.685806188043));
#47941=CARTESIAN_POINT('Ctrl Pts',(90.9265498189602,36.7998538103966,116.527857664851));
#47942=CARTESIAN_POINT('Ctrl Pts',(89.8674819628062,33.9538021035576,116.369909141658));
#47943=CARTESIAN_POINT('Ctrl Pts',(86.9053813990943,33.284776474454,116.211960618466));
#47944=CARTESIAN_POINT('Ctrl Pts',(84.7258946207258,35.3993621134993,116.054012095273));
#47945=CARTESIAN_POINT('Ctrl Pts',(85.3050960035535,38.3803285339862,115.896063572081));
#47946=CARTESIAN_POINT('Ctrl Pts',(88.1178412693811,39.5249241444546,115.738115048888));
#47947=CARTESIAN_POINT('Ctrl Pts',(90.6138998314632,37.7953789161947,115.580166525696));
#47948=CARTESIAN_POINT('Ctrl Pts',(90.5301713057494,34.7598189059295,115.422218002503));
#47949=CARTESIAN_POINT('Ctrl Pts',(87.9425698000164,33.170494052582,115.264269479311));
#47950=CARTESIAN_POINT('Ctrl Pts',(85.19719490117,34.468396863552,115.106320956119));
#47951=CARTESIAN_POINT('Ctrl Pts',(84.7831945331911,37.4767583340626,114.948372432926));
#47952=CARTESIAN_POINT('Ctrl Pts',(87.0759302384741,39.4679886139801,114.790423909734));
#47953=CARTESIAN_POINT('Ctrl Pts',(89.9966482834433,38.6366997690347,114.632475386541));
#47954=CARTESIAN_POINT('Ctrl Pts',(90.897222446349,35.7365961124309,114.474526863349));
#47955=CARTESIAN_POINT('Ctrl Pts',(88.9611295234098,33.397113426946,114.316578340156));
#47956=CARTESIAN_POINT('Ctrl Pts',(85.9437660842499,33.7393895113594,114.158629816964));
#47957=CARTESIAN_POINT('Ctrl Pts',(84.5808837901952,36.4530930497901,114.000681293771));
#47958=CARTESIAN_POINT('Ctrl Pts',(86.1081665670736,39.0777915775053,113.842732770579));
#47959=CARTESIAN_POINT('Ctrl Pts',(89.1408735712955,39.2337507660228,113.684784247386));
#47960=CARTESIAN_POINT('Ctrl Pts',(90.929341597747,36.7795671623981,113.526835724194));
#47961=CARTESIAN_POINT('Ctrl Pts',(89.8520210806407,33.9403743994175,113.368887201002));
#47962=CARTESIAN_POINT('Ctrl Pts',(86.8856857676146,33.2903822051309,113.210938677809));
#47963=CARTESIAN_POINT('Ctrl Pts',(84.7198216699789,35.4189187334791,113.052990154617));
#47964=CARTESIAN_POINT('Ctrl Pts',(85.3181518932811,38.3961046507208,112.895041631424));
#47965=CARTESIAN_POINT('Ctrl Pts',(88.1381886214443,39.5226160327098,112.737093108232));
#47966=CARTESIAN_POINT('Ctrl Pts',(90.6230903205828,37.7770792706913,112.579144585039));
#47967=CARTESIAN_POINT('Ctrl Pts',(90.519872194957,34.742119458687,112.421196061847));
#47968=CARTESIAN_POINT('Ctrl Pts',(87.9221189798339,33.1694423541105,112.263247538654));
#47969=CARTESIAN_POINT('Ctrl Pts',(85.1851345082736,34.4849464568703,112.105299015462));
#47970=CARTESIAN_POINT('Ctrl Pts',(84.7904593590192,37.4959042062408,111.947350492269));
#47971=CARTESIAN_POINT('Ctrl Pts',(87.0959334863987,39.4723717850122,111.789401969077));
#47972=CARTESIAN_POINT('Ctrl Pts',(90.0112536169413,38.6223461510488,111.631453445884));
#47973=CARTESIAN_POINT('Ctrl Pts',(90.8931876537409,35.7165196943199,111.473504922692));
#47974=CARTESIAN_POINT('Ctrl Pts',(88.9421128284366,33.3895168863927,111.315556399499));
#47975=CARTESIAN_POINT('Ctrl Pts',(85.9270093458854,33.7511604006897,111.157607876307));
#47976=CARTESIAN_POINT('Ctrl Pts',(84.5815798334644,36.4735590615522,110.999659353114));
#47977=CARTESIAN_POINT('Ctrl Pts',(86.125684310748,39.0883968014681,110.841710829922));
#47978=CARTESIAN_POINT('Ctrl Pts',(89.1593302098928,39.2248797677758,110.683762306729));
#47979=CARTESIAN_POINT('Ctrl Pts',(90.9320030585298,36.759263007048,110.525813783537));
#47980=CARTESIAN_POINT('Ctrl Pts',(89.8364742977627,33.9270462454618,110.367865260344));
#47981=CARTESIAN_POINT('Ctrl Pts',(86.8660265368926,33.2961142877669,110.209916737152));
#47982=CARTESIAN_POINT('Ctrl Pts',(84.7138744167345,35.4385139407981,110.05196821396));
#47983=CARTESIAN_POINT('Ctrl Pts',(85.3313088137564,38.4117966184305,109.894019690767));
#47984=CARTESIAN_POINT('Ctrl Pts',(88.158520730641,39.5201773016895,109.736071167575));
#47985=CARTESIAN_POINT('Ctrl Pts',(90.6321631244736,37.7587210243331,109.578122644382));
#47986=CARTESIAN_POINT('Ctrl Pts',(90.5094596355534,34.7244864369352,109.42017412119));
#47987=CARTESIAN_POINT('Ctrl Pts',(87.901661854616,33.1685221358602,109.262225597997));
#47988=CARTESIAN_POINT('Ctrl Pts',(85.1731805747687,34.5015728529517,109.104277074805));
#47989=CARTESIAN_POINT('Ctrl Pts',(84.7978470820419,37.5150036446594,108.946328551612));
#47990=CARTESIAN_POINT('Ctrl Pts',(87.1159642373238,39.4766251737973,108.78838002842));
#47991=CARTESIAN_POINT('Ctrl Pts',(90.0257669556591,38.6079016208817,108.630431505227));
#47992=CARTESIAN_POINT('Ctrl Pts',(90.8890230653562,35.696464306777,108.472482982035));
#47993=CARTESIAN_POINT('Ctrl Pts',(88.9230497393773,33.382053488629,108.314534458842));
#47994=CARTESIAN_POINT('Ctrl Pts',(85.9103244389029,33.7630162682213,108.15658593565));
#47995=CARTESIAN_POINT('Ctrl Pts',(84.5824156955773,36.4940661932323,107.998637412457));
#47996=CARTESIAN_POINT('Ctrl Pts',(86.143252472309,39.0987947060438,107.840688889265));
#47997=CARTESIAN_POINT('Ctrl Pts',(89.1777651200243,39.2160850212882,107.682740366073));
#47998=CARTESIAN_POINT('Ctrl Pts',(90.9344608864062,36.738541996859,107.52479184288));
#47999=CARTESIAN_POINT('Ctrl Pts',(89.8209930657121,33.9146410882247,107.366843319688));
#48000=CARTESIAN_POINT('Ctrl Pts',(86.8461026619917,33.3002680696704,107.208894796495));
#48001=CARTESIAN_POINT('Ctrl Pts',(84.7087432400635,35.4616433118293,107.050946273303));
#48002=CARTESIAN_POINT('Ctrl Pts',(85.1331869260174,37.4317649329324,106.945647257841));
#48003=CARTESIAN_POINT('Ctrl Pts',(85.7142240382307,38.111351395911,106.89299775011));
#48004=CARTESIAN_POINT('Ctrl Pts',(87.1183555905968,33.9228392726486,122.321006749669));
#48005=CARTESIAN_POINT('Ctrl Pts',(86.3138051921097,34.1379297320145,122.268357241939));
#48006=CARTESIAN_POINT('Ctrl Pts',(84.9485677265476,35.4262450678709,122.163058226477));
#48007=CARTESIAN_POINT('Ctrl Pts',(85.4488475373378,38.2129742552945,122.005109703284));
#48008=CARTESIAN_POINT('Ctrl Pts',(88.0564969379401,39.3109396331282,121.847161180092));
#48009=CARTESIAN_POINT('Ctrl Pts',(90.4010791517949,37.7307986176968,121.6892126569));
#48010=CARTESIAN_POINT('Ctrl Pts',(90.3598045098783,34.9022195448962,121.531264133707));
#48011=CARTESIAN_POINT('Ctrl Pts',(87.968650609882,33.3912401019918,121.373315610515));
#48012=CARTESIAN_POINT('Ctrl Pts',(85.3963064880358,34.5671137330305,121.215367087322));
#48013=CARTESIAN_POINT('Ctrl Pts',(84.9746967073516,37.3640547030401,121.05741856413));
#48014=CARTESIAN_POINT('Ctrl Pts',(87.0862481538468,39.2459948463526,120.899470040937));
#48015=CARTESIAN_POINT('Ctrl Pts',(89.816400570363,38.5067174084264,120.741521517745));
#48016=CARTESIAN_POINT('Ctrl Pts',(90.6898470763792,35.8164633031955,120.583572994552));
#48017=CARTESIAN_POINT('Ctrl Pts',(88.9146411877884,33.6144232935047,120.42562447136));
#48018=CARTESIAN_POINT('Ctrl Pts',(86.1003173820783,33.8971107544102,120.267675948167));
#48019=CARTESIAN_POINT('Ctrl Pts',(84.7985329431949,36.4082260994807,120.109727424975));
#48020=CARTESIAN_POINT('Ctrl Pts',(86.1895784263537,38.8710152113111,119.951778901782));
#48021=CARTESIAN_POINT('Ctrl Pts',(89.0122341306214,39.0525431773495,119.79383037859));
#48022=CARTESIAN_POINT('Ctrl Pts',(90.7072844955181,36.7882235900348,119.635881855397));
#48023=CARTESIAN_POINT('Ctrl Pts',(89.7378786552524,34.1310464066976,119.477933332205));
#48024=CARTESIAN_POINT('Ctrl Pts',(86.9829475248645,33.4901932417205,119.319984809013));
#48025=CARTESIAN_POINT('Ctrl Pts',(84.9403033131111,35.4467062291065,119.16203628582));
#48026=CARTESIAN_POINT('Ctrl Pts',(85.4619494316156,38.2266745186755,119.004087762628));
#48027=CARTESIAN_POINT('Ctrl Pts',(88.074925195757,39.3095854253735,118.846139239435));
#48028=CARTESIAN_POINT('Ctrl Pts',(90.4101249571212,37.7135965584462,118.688190716243));
#48029=CARTESIAN_POINT('Ctrl Pts',(90.3502941106303,34.8857424870836,118.53024219305));
#48030=CARTESIAN_POINT('Ctrl Pts',(87.9496794667482,33.3899524908652,118.372293669858));
#48031=CARTESIAN_POINT('Ctrl Pts',(85.3848453108996,34.5824138677591,118.214345146665));
#48032=CARTESIAN_POINT('Ctrl Pts',(84.9812487666711,37.3819581540233,118.056396623473));
#48033=CARTESIAN_POINT('Ctrl Pts',(87.1048185456946,39.2503236897802,117.89844810028));
#48034=CARTESIAN_POINT('Ctrl Pts',(89.8301785148752,38.4935202674369,117.740499577088));
#48035=CARTESIAN_POINT('Ctrl Pts',(90.6863276781894,35.7977185329409,117.582551053895));
#48036=CARTESIAN_POINT('Ctrl Pts',(88.8970216278814,33.6071199298345,117.424602530703));
#48037=CARTESIAN_POINT('Ctrl Pts',(86.0845697404717,33.90787358752,117.266654007511));
#48038=CARTESIAN_POINT('Ctrl Pts',(84.7989366054219,36.4272953115779,117.108705484318));
#48039=CARTESIAN_POINT('Ctrl Pts',(86.205766685515,38.8811020495552,116.950756961125));
#48040=CARTESIAN_POINT('Ctrl Pts',(89.0295299339346,39.0445018612854,116.792808437933));
#48041=CARTESIAN_POINT('Ctrl Pts',(90.710006094215,36.7693451070536,116.634859914741));
#48042=CARTESIAN_POINT('Ctrl Pts',(89.7235585412025,34.118447220157,116.476911391548));
#48043=CARTESIAN_POINT('Ctrl Pts',(86.9645692697669,33.4952966912299,116.318962868356));
#48044=CARTESIAN_POINT('Ctrl Pts',(84.9345299414539,35.464885152584,116.161014345163));
#48045=CARTESIAN_POINT('Ctrl Pts',(85.474015474389,38.2414466486347,116.003065821971));
#48046=CARTESIAN_POINT('Ctrl Pts',(88.0938907435712,39.3075573162135,115.845117298778));
#48047=CARTESIAN_POINT('Ctrl Pts',(90.4187945223373,37.696607037317,115.687168775586));
#48048=CARTESIAN_POINT('Ctrl Pts',(90.3408072632322,34.8691954349826,115.529220252393));
#48049=CARTESIAN_POINT('Ctrl Pts',(87.9306376422113,33.3888506172103,115.371271729201));
#48050=CARTESIAN_POINT('Ctrl Pts',(85.3735131526587,34.5977562076217,115.213323206008));
#48051=CARTESIAN_POINT('Ctrl Pts',(84.9879007978259,37.3998342745923,115.055374682816));
#48052=CARTESIAN_POINT('Ctrl Pts',(87.1234235719704,39.254525856152,114.897426159623));
#48053=CARTESIAN_POINT('Ctrl Pts',(89.8438679247643,38.4802385031952,114.739477636431));
#48054=CARTESIAN_POINT('Ctrl Pts',(90.6826897001046,35.7789950097624,114.581529113238));
#48055=CARTESIAN_POINT('Ctrl Pts',(88.879354705901,33.5999306967421,114.423580590046));
#48056=CARTESIAN_POINT('Ctrl Pts',(86.0688919354435,33.9187369035045,114.265632066854));
#48057=CARTESIAN_POINT('Ctrl Pts',(84.7994625063446,36.4463617384305,114.107683543661));
#48058=CARTESIAN_POINT('Ctrl Pts',(86.2220194740172,38.8910846379272,113.949735020469));
#48059=CARTESIAN_POINT('Ctrl Pts',(89.0467737009874,39.0363497019068,113.791786497276));
#48060=CARTESIAN_POINT('Ctrl Pts',(90.712606440677,36.7504495148962,113.633837974084));
#48061=CARTESIAN_POINT('Ctrl Pts',(89.7091578120227,34.1059402539464,113.475889450891));
#48062=CARTESIAN_POINT('Ctrl Pts',(86.9462241681142,33.5005180368472,113.317940927699));
#48063=CARTESIAN_POINT('Ctrl Pts',(84.9288734130558,35.4831007747579,113.159992404506));
#48064=CARTESIAN_POINT('Ctrl Pts',(85.4861761215085,38.2561409967433,113.002043881314));
#48065=CARTESIAN_POINT('Ctrl Pts',(88.1128428773144,39.3054074717351,112.844095358121));
#48066=CARTESIAN_POINT('Ctrl Pts',(90.4273548194423,37.6795621988556,112.686146834929));
#48067=CARTESIAN_POINT('Ctrl Pts',(90.3312143626637,34.8527096391759,112.528198311737));
#48068=CARTESIAN_POINT('Ctrl Pts',(87.9115891351597,33.3878710337231,112.370249788544));
#48069=CARTESIAN_POINT('Ctrl Pts',(85.3622797411336,34.6131709950098,112.212301265351));
#48070=CARTESIAN_POINT('Ctrl Pts',(84.9946674744083,37.4176673139493,112.054352742159));
#48071=CARTESIAN_POINT('Ctrl Pts',(87.1420551968024,39.2586084730626,111.896404218967));
#48072=CARTESIAN_POINT('Ctrl Pts',(89.8574717702652,38.466869113069,111.738455695774));
#48073=CARTESIAN_POINT('Ctrl Pts',(90.6789315733027,35.760295232025,111.580507172582));
#48074=CARTESIAN_POINT('Ctrl Pts',(88.8616419860657,33.5928550511199,111.422558649389));
#48075=CARTESIAN_POINT('Ctrl Pts',(86.0532842069489,33.9297006627284,111.264610126197));
#48076=CARTESIAN_POINT('Ctrl Pts',(84.8001108219136,36.4654243953749,111.106661603004));
#48077=CARTESIAN_POINT('Ctrl Pts',(86.2383360256732,38.9009626614801,110.948713079812));
#48078=CARTESIAN_POINT('Ctrl Pts',(89.0639647675231,39.0280869881792,110.790764556619));
#48079=CARTESIAN_POINT('Ctrl Pts',(90.7150854050432,36.7315376158666,110.632816033427));
#48080=CARTESIAN_POINT('Ctrl Pts',(89.6946770723436,34.0935260117623,110.474867510234));
#48081=CARTESIAN_POINT('Ctrl Pts',(86.9279129712189,33.5058570704672,110.316918987042));
#48082=CARTESIAN_POINT('Ctrl Pts',(84.9233339630798,35.5013523383365,110.158970463849));
#48083=CARTESIAN_POINT('Ctrl Pts',(85.4984308716953,38.2707569659272,110.001021940657));
#48084=CARTESIAN_POINT('Ctrl Pts',(88.1317808133949,39.3031359645476,109.843073417464));
#48085=CARTESIAN_POINT('Ctrl Pts',(90.4358055009968,37.662462777801,109.685124894272));
#48086=CARTESIAN_POINT('Ctrl Pts',(90.3215157926575,34.8362857140626,109.52717637108));
#48087=CARTESIAN_POINT('Ctrl Pts',(87.892534755409,33.3870139148558,109.369227847887));
#48088=CARTESIAN_POINT('Ctrl Pts',(85.3511454890778,34.6286573187941,109.211279324695));
#48089=CARTESIAN_POINT('Ctrl Pts',(85.001548621122,37.4354571035105,109.053330801502));
#48090=CARTESIAN_POINT('Ctrl Pts',(87.1607124387537,39.2625702068974,108.89538227831));
#48091=CARTESIAN_POINT('Ctrl Pts',(89.8709899290696,38.4534150446116,108.737433755117));
#48092=CARTESIAN_POINT('Ctrl Pts',(90.6750525508231,35.7416150427893,108.579485231925));
#48093=CARTESIAN_POINT('Ctrl Pts',(88.8438860533876,33.5859034186835,108.421536708732));
#48094=CARTESIAN_POINT('Ctrl Pts',(86.0377433843573,33.9407435731967,108.26358818554));
#48095=CARTESIAN_POINT('Ctrl Pts',(84.8008893689454,36.4845253526437,108.105639662347));
#48096=CARTESIAN_POINT('Ctrl Pts',(86.25469953806,38.9106475815404,107.947691139155));
#48097=CARTESIAN_POINT('Ctrl Pts',(89.0811355955146,39.0198952976263,107.789742615962));
#48098=CARTESIAN_POINT('Ctrl Pts',(90.717374699615,36.7122374457423,107.63179409277));
#48099=CARTESIAN_POINT('Ctrl Pts',(89.6802573886707,34.081971476394,107.473845569577));
#48100=CARTESIAN_POINT('Ctrl Pts',(86.9093552768007,33.5097260274662,107.315897046385));
#48101=CARTESIAN_POINT('Ctrl Pts',(84.9185546312914,35.522895727954,107.157948523192));
#48102=CARTESIAN_POINT('Ctrl Pts',(85.3138942055859,37.3579260718377,107.052649507731));
#48103=CARTESIAN_POINT('Ctrl Pts',(85.8550895919077,37.990913278059,107.));
#48104=CARTESIAN_POINT('Ctrl Pts',(85.2535609624353,36.356687859589,121.112583302492));
#48105=CARTESIAN_POINT('Ctrl Pts',(85.2516480964026,36.6482406983004,121.094195056371));
#48106=CARTESIAN_POINT('Ctrl Pts',(85.2985193878855,36.9391986870805,121.07580681025));
#48107=CARTESIAN_POINT('Ctrl Pts',(85.3968902452148,37.2115545652573,121.05741856413));
#48108=CARTESIAN_POINT('Ctrl Pts',(85.6785471895167,37.9913680841443,121.004769056399));
#48109=CARTESIAN_POINT('Ctrl Pts',(86.3823976716817,38.6186814652484,120.952119548668));
#48110=CARTESIAN_POINT('Ctrl Pts',(87.189348315517,38.8091252494795,120.899470040937));
#48111=CARTESIAN_POINT('Ctrl Pts',(87.9962989593522,38.9995690337106,120.846820533206));
#48112=CARTESIAN_POINT('Ctrl Pts',(88.9063497648576,38.7531432210685,120.794171025476));
#48113=CARTESIAN_POINT('Ctrl Pts',(89.5069495852796,38.1815546305423,120.741521517745));
#48114=CARTESIAN_POINT('Ctrl Pts',(90.1075494057017,37.6099660400161,120.688872010014));
#48115=CARTESIAN_POINT('Ctrl Pts',(90.3986982410404,36.7132146716058,120.636222502283));
#48116=CARTESIAN_POINT('Ctrl Pts',(90.2484050106114,35.8978323191188,120.583572994552));
#48117=CARTESIAN_POINT('Ctrl Pts',(90.0981117801823,35.0824499666319,120.530923486821));
#48118=CARTESIAN_POINT('Ctrl Pts',(89.5063764839853,34.3484366300683,120.478273979091));
#48119=CARTESIAN_POINT('Ctrl Pts',(88.7414548682685,34.0285445386041,120.42562447136));
#48120=CARTESIAN_POINT('Ctrl Pts',(87.9765332525517,33.7086524471399,120.372974963629));
#48121=CARTESIAN_POINT('Ctrl Pts',(87.038425317315,33.802881600775,120.320325455898));
#48122=CARTESIAN_POINT('Ctrl Pts',(86.3524072765494,34.268515401771,120.267675948167));
#48123=CARTESIAN_POINT('Ctrl Pts',(85.6787931725816,34.7257300477372,120.215978399609));
#48124=CARTESIAN_POINT('Ctrl Pts',(85.2482352700075,35.5410399793431,120.16428085105));
#48125=CARTESIAN_POINT('Ctrl Pts',(85.2469699766098,36.3551993258525,120.112583302492));
#48126=CARTESIAN_POINT('Ctrl Pts',(86.9747563060389,33.385703120938,122.));
#48127=CARTESIAN_POINT('Ctrl Pts',(86.8817062479769,33.419741247829,122.));
#48128=CARTESIAN_POINT('Ctrl Pts',(86.7907213548637,33.4585480736554,122.));
#48129=CARTESIAN_POINT('Ctrl Pts',(86.7020101118859,33.5017952757603,122.));
#48130=CARTESIAN_POINT('Ctrl Pts',(86.611331909906,33.5460013808254,122.));
#48131=CARTESIAN_POINT('Ctrl Pts',(86.5230286333761,33.5948475710693,122.));
#48132=CARTESIAN_POINT('Ctrl Pts',(86.4373518622086,33.6480287386438,122.));
#48133=CARTESIAN_POINT('Ctrl Pts',(86.3549204309049,33.6991954633212,122.));
#48134=CARTESIAN_POINT('Ctrl Pts',(86.2749200114897,33.7543758529771,122.));
#48135=CARTESIAN_POINT('Ctrl Pts',(86.1976076309381,33.8133282211128,122.));
#48136=CARTESIAN_POINT('Ctrl Pts',(86.1299592979554,33.8649115432316,122.));
#48137=CARTESIAN_POINT('Ctrl Pts',(86.0643692849632,33.9193834837333,122.));
#48138=CARTESIAN_POINT('Ctrl Pts',(86.0010344007775,33.9765948307505,122.));
#48139=CARTESIAN_POINT('Ctrl Pts',(85.9868979548522,33.989364493533,122.));
#48140=CARTESIAN_POINT('Ctrl Pts',(85.9728712144497,34.0022733665456,122.));
#48141=CARTESIAN_POINT('Ctrl Pts',(85.9589759527776,34.015301257801,122.));
#48142=CARTESIAN_POINT('Ctrl Pts',(85.8865458564609,34.0832101205986,122.));
#48143=CARTESIAN_POINT('Ctrl Pts',(85.8175814474561,34.1544408988363,122.));
#48144=CARTESIAN_POINT('Ctrl Pts',(85.7523226756092,34.2287028696647,122.));
#48145=CARTESIAN_POINT('Ctrl Pts',(85.6874229281471,34.3025562845606,122.));
#48146=CARTESIAN_POINT('Ctrl Pts',(85.6261876700599,34.3794084282326,122.));
#48147=CARTESIAN_POINT('Ctrl Pts',(85.5688965222133,34.4590001179627,122.));
#48148=CARTESIAN_POINT('Ctrl Pts',(85.5137336076299,34.5356351610219,122.));
#48149=CARTESIAN_POINT('Ctrl Pts',(85.4622270538762,34.6148107322579,122.));
#48150=CARTESIAN_POINT('Ctrl Pts',(85.4146713091807,34.6963090585297,122.));
#48151=CARTESIAN_POINT('Ctrl Pts',(85.3947249791741,34.7304919426631,122.));
#48152=CARTESIAN_POINT('Ctrl Pts',(85.3754742525693,34.7650835569962,122.));
#48153=CARTESIAN_POINT('Ctrl Pts',(85.3569434395582,34.8000681299898,122.));
#48154=CARTESIAN_POINT('Ctrl Pts',(85.344060903815,34.8243892437899,122.));
#48155=CARTESIAN_POINT('Ctrl Pts',(85.3315263323148,34.8489002759048,122.));
#48156=CARTESIAN_POINT('Ctrl Pts',(85.3193483589149,34.8735959330844,122.));
#48157=CARTESIAN_POINT('Ctrl Pts',(85.3114400096724,34.8896332387456,122.));
#48158=CARTESIAN_POINT('Ctrl Pts',(85.3036809360749,34.9057510169598,122.));
#48159=CARTESIAN_POINT('Ctrl Pts',(85.2960836785505,34.9219256286096,122.));
#48160=CARTESIAN_POINT('Ctrl Pts',(85.2539633762117,35.0116000316037,122.));
#48161=CARTESIAN_POINT('Ctrl Pts',(85.2167419072931,35.1031580252053,122.));
#48162=CARTESIAN_POINT('Ctrl Pts',(85.1847105554573,35.1963272446824,122.));
#48163=CARTESIAN_POINT('Ctrl Pts',(85.1548308024479,35.2832381337491,122.));
#48164=CARTESIAN_POINT('Ctrl Pts',(85.1294675005642,35.3715518528724,122.));
#48165=CARTESIAN_POINT('Ctrl Pts',(85.1089076276163,35.4610560157098,122.));
#48166=CARTESIAN_POINT('Ctrl Pts',(85.1074271401942,35.4675010841028,122.));
#48167=CARTESIAN_POINT('Ctrl Pts',(85.1059715822065,35.4739523263869,122.));
#48168=CARTESIAN_POINT('Ctrl Pts',(85.1045410714323,35.4804096635754,122.));
#48169=CARTESIAN_POINT('Ctrl Pts',(85.0839348524742,35.5734263023821,122.));
#48170=CARTESIAN_POINT('Ctrl Pts',(85.06852165899,35.6677086068536,122.));
#48171=CARTESIAN_POINT('Ctrl Pts',(85.0582245708442,35.7628487105457,122.));
#48172=CARTESIAN_POINT('Ctrl Pts',(85.0524280535226,35.8164057211517,122.));
#48173=CARTESIAN_POINT('Ctrl Pts',(85.0482536960829,35.8702343689899,122.));
#48174=CARTESIAN_POINT('Ctrl Pts',(85.0456945388939,35.9242592591601,122.));
#48175=CARTESIAN_POINT('Ctrl Pts',(85.0450336564343,35.9382107672774,122.));
#48176=CARTESIAN_POINT('Ctrl Pts',(85.0444806105962,35.9521747635378,122.));
#48177=CARTESIAN_POINT('Ctrl Pts',(85.0440355229243,35.9661365800473,122.));
#48178=CARTESIAN_POINT('Ctrl Pts',(85.0410641138316,36.0593457861118,122.));
#48179=CARTESIAN_POINT('Ctrl Pts',(85.0428918593198,36.1526132293267,122.));
#48180=CARTESIAN_POINT('Ctrl Pts',(85.0493838649713,36.2455638298956,122.));
#48181=CARTESIAN_POINT('Ctrl Pts',(85.055886664939,36.3386689802641,122.));
#48182=CARTESIAN_POINT('Ctrl Pts',(85.0670696265457,36.4314572131348,122.));
#48183=CARTESIAN_POINT('Ctrl Pts',(85.0828481140956,36.5235394789013,122.));
#48184=CARTESIAN_POINT('Ctrl Pts',(85.0984010048097,36.6143051756542,122.));
#48185=CARTESIAN_POINT('Ctrl Pts',(85.1184194105491,36.7043857925402,122.));
#48186=CARTESIAN_POINT('Ctrl Pts',(85.142865299154,36.7933835307099,122.));
#48187=CARTESIAN_POINT('Ctrl Pts',(85.1519640629711,36.8265085037045,122.));
#48188=CARTESIAN_POINT('Ctrl Pts',(85.1616765771494,36.8594831454966,122.));
#48189=CARTESIAN_POINT('Ctrl Pts',(85.1720022421283,36.8922856787441,122.));
#48190=CARTESIAN_POINT('Ctrl Pts',(85.1789967228274,36.9145057184361,122.));
#48191=CARTESIAN_POINT('Ctrl Pts',(85.1862725653383,36.9366467701123,122.));
#48192=CARTESIAN_POINT('Ctrl Pts',(85.1938297624176,36.9587018515215,122.));
#48193=CARTESIAN_POINT('Ctrl Pts',(85.1983458216605,36.9718816129072,122.));
#48194=CARTESIAN_POINT('Ctrl Pts',(85.202962008638,36.9850295012457,122.));
#48195=CARTESIAN_POINT('Ctrl Pts',(85.2076748514515,36.9981348782542,122.));
#48196=CARTESIAN_POINT('Ctrl Pts',(85.2393066085118,37.0860958220241,122.));
#48197=CARTESIAN_POINT('Ctrl Pts',(85.2753275863277,37.1722590184577,122.));
#48198=CARTESIAN_POINT('Ctrl Pts',(85.3156732208267,37.2562102232251,122.));
#48199=CARTESIAN_POINT('Ctrl Pts',(85.3459324467009,37.3191736268007,122.));
#48200=CARTESIAN_POINT('Ctrl Pts',(85.3786253392863,37.3808922931221,122.));
#48201=CARTESIAN_POINT('Ctrl Pts',(85.4137406224306,37.4411759317203,122.));
#48202=CARTESIAN_POINT('Ctrl Pts',(85.4272099477612,37.4642991950884,122.));
#48203=CARTESIAN_POINT('Ctrl Pts',(85.4410358113732,37.4872111624651,122.));
#48204=CARTESIAN_POINT('Ctrl Pts',(85.4552180573203,37.5099004508088,122.));
#48205=CARTESIAN_POINT('Ctrl Pts',(85.4653423426853,37.526097661799,122.));
#48206=CARTESIAN_POINT('Ctrl Pts',(85.475649081078,37.5421824590417,122.));
#48207=CARTESIAN_POINT('Ctrl Pts',(85.4861281406993,37.5581356970078,122.));
#48208=CARTESIAN_POINT('Ctrl Pts',(85.5333147178236,37.629972170974,122.));
#48209=CARTESIAN_POINT('Ctrl Pts',(85.5840362197561,37.699215193506,122.));
#48210=CARTESIAN_POINT('Ctrl Pts',(85.6382597550527,37.7655127650129,122.));
#48211=CARTESIAN_POINT('Ctrl Pts',(85.6870561730674,37.8251747548651,122.));
#48212=CARTESIAN_POINT('Ctrl Pts',(85.7386892863001,37.8824513165183,122.));
#48213=CARTESIAN_POINT('Ctrl Pts',(85.7931556159572,37.9370561104042,122.));
#48214=CARTESIAN_POINT('Ctrl Pts',(85.8122381875779,37.9561871937123,122.));
#48215=CARTESIAN_POINT('Ctrl Pts',(85.831668704075,37.9749900284081,122.));
#48216=CARTESIAN_POINT('Ctrl Pts',(85.8514365905237,37.9934601270859,122.));
#48217=CARTESIAN_POINT('Origin',(87.7685555885722,36.3549260746835,114.));
#48218=CARTESIAN_POINT('Origin',(36.3549260746835,87.7685555885722,107.));
#48219=CARTESIAN_POINT('Ctrl Pts',(34.441460078019,89.4045427919478,107.));
#48220=CARTESIAN_POINT('Ctrl Pts',(34.3793225172007,89.3461487428037,107.));
#48221=CARTESIAN_POINT('Ctrl Pts',(34.3205603295786,89.2845007868439,107.));
#48222=CARTESIAN_POINT('Ctrl Pts',(34.2651854953777,89.2199753995623,107.));
#48223=CARTESIAN_POINT('Ctrl Pts',(34.2084555851626,89.1538710133388,107.));
#48224=CARTESIAN_POINT('Ctrl Pts',(34.1552803722276,89.0847461545033,107.));
#48225=CARTESIAN_POINT('Ctrl Pts',(34.1057016258454,89.0129593433036,107.));
#48226=CARTESIAN_POINT('Ctrl Pts',(34.0927638402984,88.9942262684241,107.));
#48227=CARTESIAN_POINT('Ctrl Pts',(34.0800711346354,88.9753117055674,107.));
#48228=CARTESIAN_POINT('Ctrl Pts',(34.0676246265426,88.9562215925571,107.));
#48229=CARTESIAN_POINT('Ctrl Pts',(34.0574547177416,88.9406232651493,107.));
#48230=CARTESIAN_POINT('Ctrl Pts',(34.0474487386034,88.924906826773,107.));
#48231=CARTESIAN_POINT('Ctrl Pts',(34.0376161466441,88.9090901117026,107.));
#48232=CARTESIAN_POINT('Ctrl Pts',(33.9901720007546,88.832771421737,107.));
#48233=CARTESIAN_POINT('Ctrl Pts',(33.9467114185444,88.7540453734224,107.));
#48234=CARTESIAN_POINT('Ctrl Pts',(33.90726908701,88.6733045174429,107.));
#48235=CARTESIAN_POINT('Ctrl Pts',(33.875440607195,88.6081496798658,107.));
#48236=CARTESIAN_POINT('Ctrl Pts',(33.8462292660138,88.5416817343779,107.));
#48237=CARTESIAN_POINT('Ctrl Pts',(33.8196704493666,88.4740891537832,107.));
#48238=CARTESIAN_POINT('Ctrl Pts',(33.8090688925697,88.4471080351685,107.));
#48239=CARTESIAN_POINT('Ctrl Pts',(33.7988901696328,88.4199475664955,107.));
#48240=CARTESIAN_POINT('Ctrl Pts',(33.7891372918137,88.3926191895465,107.));
#48241=CARTESIAN_POINT('Ctrl Pts',(33.7838963682359,88.377933684637,107.));
#48242=CARTESIAN_POINT('Ctrl Pts',(33.778778795415,88.3632005117775,107.));
#48243=CARTESIAN_POINT('Ctrl Pts',(33.7737890400817,88.3484339243473,107.));
#48244=CARTESIAN_POINT('Ctrl Pts',(33.7442502226087,88.261017307367,107.));
#48245=CARTESIAN_POINT('Ctrl Pts',(33.7191468702095,88.1723195871917,107.));
#48246=CARTESIAN_POINT('Ctrl Pts',(33.6985115520217,88.0827385727371,107.));
#48247=CARTESIAN_POINT('Ctrl Pts',(33.6775547727315,87.9917620473723,107.));
#48248=CARTESIAN_POINT('Ctrl Pts',(33.6612058191073,87.899873687659,107.));
#48249=CARTESIAN_POINT('Ctrl Pts',(33.6495406312905,87.8074569994372,107.));
#48250=CARTESIAN_POINT('Ctrl Pts',(33.6379661598897,87.7157590060932,107.));
#48251=CARTESIAN_POINT('Ctrl Pts',(33.6310025450947,87.623539939619,107.));
#48252=CARTESIAN_POINT('Ctrl Pts',(33.6287709136307,87.5311552180529,107.));
#48253=CARTESIAN_POINT('Ctrl Pts',(33.6276602991915,87.4851781795572,107.));
#48254=CARTESIAN_POINT('Ctrl Pts',(33.6277224410312,87.4391598993582,107.));
#48255=CARTESIAN_POINT('Ctrl Pts',(33.628977067353,87.3931434876068,107.));
#48256=CARTESIAN_POINT('Ctrl Pts',(33.6293468454931,87.3795809926617,107.));
#48257=CARTESIAN_POINT('Ctrl Pts',(33.6298202330787,87.3660186593414,107.));
#48258=CARTESIAN_POINT('Ctrl Pts',(33.6303977915693,87.3524575913575,107.));
#48259=CARTESIAN_POINT('Ctrl Pts',(33.6310182960977,87.337888150802,107.));
#48260=CARTESIAN_POINT('Ctrl Pts',(33.6317586368159,87.323329957392,107.));
#48261=CARTESIAN_POINT('Ctrl Pts',(33.6326188622406,87.3087869385134,107.));
#48262=CARTESIAN_POINT('Ctrl Pts',(33.6382706654492,87.2132372391001,107.));
#48263=CARTESIAN_POINT('Ctrl Pts',(33.6490951084808,87.1183092558368,107.));
#48264=CARTESIAN_POINT('Ctrl Pts',(33.6651626470178,87.0243986317404,107.));
#48265=CARTESIAN_POINT('Ctrl Pts',(33.667542969346,87.0104862608519,107.));
#48266=CARTESIAN_POINT('Ctrl Pts',(33.6700384483224,86.996596184385,107.));
#48267=CARTESIAN_POINT('Ctrl Pts',(33.6726494055391,86.9827296580056,107.));
#48268=CARTESIAN_POINT('Ctrl Pts',(33.6895950528478,86.8927330606227,107.));
#48269=CARTESIAN_POINT('Ctrl Pts',(33.7114005839111,86.8037286330741,107.));
#48270=CARTESIAN_POINT('Ctrl Pts',(33.7377634487177,86.7159486239087,107.));
#48271=CARTESIAN_POINT('Ctrl Pts',(33.7647222602648,86.6261843004161,107.));
#48272=CARTESIAN_POINT('Ctrl Pts',(33.796446985534,86.5376996780423,107.));
#48273=CARTESIAN_POINT('Ctrl Pts',(33.8326683308032,86.4507468020112,107.));
#48274=CARTESIAN_POINT('Ctrl Pts',(33.8451584343998,86.4207630887731,107.));
#48275=CARTESIAN_POINT('Ctrl Pts',(33.8581836620157,86.390961590169,107.));
#48276=CARTESIAN_POINT('Ctrl Pts',(33.8717343440126,86.3613529800899,107.));
#48277=CARTESIAN_POINT('Ctrl Pts',(33.8784253792389,86.3467328854639,107.));
#48278=CARTESIAN_POINT('Ctrl Pts',(33.8852445396145,86.3321598238552,107.));
#48279=CARTESIAN_POINT('Ctrl Pts',(33.8921907202356,86.3176351028333,107.));
#48280=CARTESIAN_POINT('Ctrl Pts',(33.8976844953031,86.306147415633,107.));
#48281=CARTESIAN_POINT('Ctrl Pts',(33.903257285469,86.2946909919042,107.));
#48282=CARTESIAN_POINT('Ctrl Pts',(33.9089039498725,86.2832754082256,107.));
#48283=CARTESIAN_POINT('Ctrl Pts',(33.951627885367,86.1969025293251,107.));
#48284=CARTESIAN_POINT('Ctrl Pts',(33.9986426798443,86.1127279663445,107.));
#48285=CARTESIAN_POINT('Ctrl Pts',(34.0496056775094,86.0310013571143,107.));
#48286=CARTESIAN_POINT('Ctrl Pts',(34.1015793905264,85.9476539182156,107.));
#48287=CARTESIAN_POINT('Ctrl Pts',(34.1576597775509,85.8668517216779,107.));
#48288=CARTESIAN_POINT('Ctrl Pts',(34.2175383986755,85.7888665836747,107.));
#48289=CARTESIAN_POINT('Ctrl Pts',(34.2779038546066,85.7102473983462,107.));
#48290=CARTESIAN_POINT('Ctrl Pts',(34.3421300165413,85.6344904284207,107.));
#48291=CARTESIAN_POINT('Ctrl Pts',(34.4099501911919,85.5618934535173,107.));
#48292=CARTESIAN_POINT('Ctrl Pts',(34.4469508834432,85.5222866795653,107.));
#48293=CARTESIAN_POINT('Ctrl Pts',(34.485022140315,85.483620877737,107.));
#48294=CARTESIAN_POINT('Ctrl Pts',(34.5241260026544,85.4459481822937,107.));
#48295=CARTESIAN_POINT('Ctrl Pts',(34.5360933740782,85.4344188061162,107.));
#48296=CARTESIAN_POINT('Ctrl Pts',(34.5481574847406,85.4229824675042,107.));
#48297=CARTESIAN_POINT('Ctrl Pts',(34.5603173095881,85.4116407228736,107.));
#48298=CARTESIAN_POINT('Ctrl Pts',(34.5708630920203,85.4018044322382,107.));
#48299=CARTESIAN_POINT('Ctrl Pts',(34.5814797527798,85.3920404066204,107.));
#48300=CARTESIAN_POINT('Ctrl Pts',(34.5921575105618,85.3823576403064,107.));
#48301=CARTESIAN_POINT('Ctrl Pts',(34.6677319836388,85.3138254655697,107.));
#48302=CARTESIAN_POINT('Ctrl Pts',(34.7464831774698,85.2492496355464,107.));
#48303=CARTESIAN_POINT('Ctrl Pts',(34.8280837446808,85.1889119226529,107.));
#48304=CARTESIAN_POINT('Ctrl Pts',(34.9097885075176,85.1284971646361,107.));
#48305=CARTESIAN_POINT('Ctrl Pts',(34.9943504984862,85.0723305153877,107.));
#48306=CARTESIAN_POINT('Ctrl Pts',(35.0814863891448,85.0207206280586,107.));
#48307=CARTESIAN_POINT('Ctrl Pts',(35.1668900448395,84.9701367295688,107.));
#48308=CARTESIAN_POINT('Ctrl Pts',(35.2547669448013,84.923929541906,107.));
#48309=CARTESIAN_POINT('Ctrl Pts',(35.3448844138265,84.8824254779805,107.));
#48310=CARTESIAN_POINT('Ctrl Pts',(35.3852340815519,84.8638422309501,107.));
#48311=CARTESIAN_POINT('Ctrl Pts',(35.4260333307823,84.8462023913809,107.));
#48312=CARTESIAN_POINT('Ctrl Pts',(35.4672630298986,84.8295382061365,107.));
#48313=CARTESIAN_POINT('Ctrl Pts',(35.4976826757836,84.8172432191498,107.));
#48314=CARTESIAN_POINT('Ctrl Pts',(35.5283366660204,84.8054793853022,107.));
#48315=CARTESIAN_POINT('Ctrl Pts',(35.5592127316546,84.7942440238826,107.));
#48316=CARTESIAN_POINT('Ctrl Pts',(37.1487253572157,84.7993326348264,107.));
#48317=CARTESIAN_POINT('Ctrl Pts',(37.2435592315062,84.834023289662,107.));
#48318=CARTESIAN_POINT('Ctrl Pts',(37.3363499518797,84.8737048348486,107.));
#48319=CARTESIAN_POINT('Ctrl Pts',(37.426856595716,84.9180569182258,107.));
#48320=CARTESIAN_POINT('Ctrl Pts',(37.5186361403217,84.9630327768162,107.));
#48321=CARTESIAN_POINT('Ctrl Pts',(37.6080675777822,85.012812173707,107.));
#48322=CARTESIAN_POINT('Ctrl Pts',(37.6948656522897,85.0671017322032,107.));
#48323=CARTESIAN_POINT('Ctrl Pts',(37.7193786617565,85.0824338748678,107.));
#48324=CARTESIAN_POINT('Ctrl Pts',(37.7436814000741,85.0981259477375,107.));
#48325=CARTESIAN_POINT('Ctrl Pts',(37.7677668456399,85.1141717983225,107.));
#48326=CARTESIAN_POINT('Ctrl Pts',(37.7870964269421,85.1270492671074,107.));
#48327=CARTESIAN_POINT('Ctrl Pts',(37.8062881599554,85.1401562208434,107.));
#48328=CARTESIAN_POINT('Ctrl Pts',(37.8253191290425,85.1534757143532,107.));
#48329=CARTESIAN_POINT('Ctrl Pts',(37.9080262255787,85.2113611867365,107.));
#48330=CARTESIAN_POINT('Ctrl Pts',(37.9877784618244,85.2733088104048,107.));
#48331=CARTESIAN_POINT('Ctrl Pts',(38.0643094764772,85.3390212224136,107.));
#48332=CARTESIAN_POINT('Ctrl Pts',(38.1233026628328,85.3896749944183,107.));
#48333=CARTESIAN_POINT('Ctrl Pts',(38.1803811813906,85.4425666947868,107.));
#48334=CARTESIAN_POINT('Ctrl Pts',(38.2354054643368,85.4975718921607,107.));
#48335=CARTESIAN_POINT('Ctrl Pts',(38.2646941992609,85.5268504680742,107.));
#48336=CARTESIAN_POINT('Ctrl Pts',(38.2934006313696,85.5567280097293,107.));
#48337=CARTESIAN_POINT('Ctrl Pts',(38.3215016904264,85.5871865825445,107.));
#48338=CARTESIAN_POINT('Ctrl Pts',(38.3311376927784,85.5976309888813,107.));
#48339=CARTESIAN_POINT('Ctrl Pts',(38.3407017795108,85.6081430071488,107.));
#48340=CARTESIAN_POINT('Ctrl Pts',(38.350186383968,85.6187143015985,107.));
#48341=CARTESIAN_POINT('Ctrl Pts',(38.4159835728468,85.6920501439884,107.));
#48342=CARTESIAN_POINT('Ctrl Pts',(38.4780486111932,85.7683326104205,107.));
#48343=CARTESIAN_POINT('Ctrl Pts',(38.5361377306736,85.847283140632,107.));
#48344=CARTESIAN_POINT('Ctrl Pts',(38.5937003927959,85.9255181480756,107.));
#48345=CARTESIAN_POINT('Ctrl Pts',(38.6473593102664,86.0063738621224,107.));
#48346=CARTESIAN_POINT('Ctrl Pts',(38.6968315394181,86.0896016134082,107.));
#48347=CARTESIAN_POINT('Ctrl Pts',(38.7448894802278,86.1704500896869,107.));
#48348=CARTESIAN_POINT('Ctrl Pts',(38.7889968935663,86.2535376194815,107.));
#48349=CARTESIAN_POINT('Ctrl Pts',(38.8288466283339,86.3386465795827,107.));
#48350=CARTESIAN_POINT('Ctrl Pts',(38.8496510436295,86.3830795516376,107.));
#48351=CARTESIAN_POINT('Ctrl Pts',(38.8692941732027,86.4280635917019,107.));
#48352=CARTESIAN_POINT('Ctrl Pts',(38.8877266169703,86.4735679687981,107.));
#48353=CARTESIAN_POINT('Ctrl Pts',(38.8947846967753,86.4909923282087,107.));
#48354=CARTESIAN_POINT('Ctrl Pts',(38.9016652173504,86.5084929807057,107.));
#48355=CARTESIAN_POINT('Ctrl Pts',(38.9083652431171,86.5260681921585,107.));
#48356=CARTESIAN_POINT('Ctrl Pts',(38.913606979836,86.5398180842369,107.));
#48357=CARTESIAN_POINT('Ctrl Pts',(38.9187383404309,86.5536141120902,107.));
#48358=CARTESIAN_POINT('Ctrl Pts',(38.9237527897203,86.5674407323754,107.));
#48359=CARTESIAN_POINT('Ctrl Pts',(38.9554364793356,86.6548039342482,107.));
#48360=CARTESIAN_POINT('Ctrl Pts',(38.9825113433306,86.7435280735438,107.));
#48361=CARTESIAN_POINT('Ctrl Pts',(39.0047261257503,86.8333895970977,107.));
#48362=CARTESIAN_POINT('Ctrl Pts',(39.0097100967495,86.8535503719762,107.));
#48363=CARTESIAN_POINT('Ctrl Pts',(39.0144492341345,86.8737684362943,107.));
#48364=CARTESIAN_POINT('Ctrl Pts',(39.0189403397705,86.8940413210693,107.));
#48365=CARTESIAN_POINT('Ctrl Pts',(39.0393060941569,86.9859724902492,107.));
#48366=CARTESIAN_POINT('Ctrl Pts',(39.0545756375306,87.0790312711289,107.));
#48367=CARTESIAN_POINT('Ctrl Pts',(39.0648587946489,87.1728260780746,107.));
#48368=CARTESIAN_POINT('Ctrl Pts',(39.0755926599919,87.2707318881325,107.));
#48369=CARTESIAN_POINT('Ctrl Pts',(39.0808934432669,87.3694408954707,107.));
#48370=CARTESIAN_POINT('Ctrl Pts',(39.0808285913654,87.4684930845029,107.));
#48371=CARTESIAN_POINT('Ctrl Pts',(39.0808032243523,87.5072376411785,107.));
#48372=CARTESIAN_POINT('Ctrl Pts',(39.0799563126054,87.5460344480642,107.));
#48373=CARTESIAN_POINT('Ctrl Pts',(39.0782896687133,87.5848547474918,107.));
#48374=CARTESIAN_POINT('Ctrl Pts',(39.0777566303355,87.5972705428099,107.));
#48375=CARTESIAN_POINT('Ctrl Pts',(39.077139745471,87.6096874298378,107.));
#48376=CARTESIAN_POINT('Ctrl Pts',(39.0764397752444,87.6220947992235,107.));
#48377=CARTESIAN_POINT('Ctrl Pts',(39.0712005660668,87.714962754302,107.));
#48378=CARTESIAN_POINT('Ctrl Pts',(39.0613049370046,87.8074474727188,107.));
#48379=CARTESIAN_POINT('Ctrl Pts',(39.0468763468412,87.8991773783878,107.));
#48380=CARTESIAN_POINT('Ctrl Pts',(39.032481744757,87.9906912045047,107.));
#48381=CARTESIAN_POINT('Ctrl Pts',(39.0135751022545,88.0814547150913,107.));
#48382=CARTESIAN_POINT('Ctrl Pts',(38.9902303316761,88.1710820012943,107.));
#48383=CARTESIAN_POINT('Ctrl Pts',(38.9672817085728,88.2591883634421,107.));
#48384=CARTESIAN_POINT('Ctrl Pts',(38.9400438369275,88.3461975214973,107.));
#48385=CARTESIAN_POINT('Ctrl Pts',(38.908546488776,88.4317137837883,107.));
#48386=CARTESIAN_POINT('Ctrl Pts',(38.8927050493307,88.4747237757455,107.));
#48387=CARTESIAN_POINT('Ctrl Pts',(38.87578555997,88.5173555992814,107.));
#48388=CARTESIAN_POINT('Ctrl Pts',(38.8577883909143,88.5595551232321,107.));
#48389=CARTESIAN_POINT('Ctrl Pts',(38.8522226770006,88.5726055355986,107.));
#48390=CARTESIAN_POINT('Ctrl Pts',(38.8465538797673,88.5856145826971,107.));
#48391=CARTESIAN_POINT('Ctrl Pts',(38.8407819692872,88.5985806059024,107.));
#48392=CARTESIAN_POINT('Ctrl Pts',(38.8351025158747,88.6113389334947,107.));
#48393=CARTESIAN_POINT('Ctrl Pts',(38.8293267074872,88.6240477399775,107.));
#48394=CARTESIAN_POINT('Ctrl Pts',(38.8234563337807,88.6367025399068,107.));
#48395=CARTESIAN_POINT('Ctrl Pts',(38.7859765367107,88.7174979640187,107.));
#48396=CARTESIAN_POINT('Ctrl Pts',(38.7446265820373,88.79613660999,107.));
#48397=CARTESIAN_POINT('Ctrl Pts',(38.6994761457792,88.8722708876746,107.));
#48398=CARTESIAN_POINT('Ctrl Pts',(38.6550831391013,88.9471279605575,107.));
#48399=CARTESIAN_POINT('Ctrl Pts',(38.6070156385787,89.0195646548357,107.));
#48400=CARTESIAN_POINT('Ctrl Pts',(38.5553036590933,89.0892164043883,107.));
#48401=CARTESIAN_POINT('Ctrl Pts',(38.5051691920445,89.1567433754613,107.));
#48402=CARTESIAN_POINT('Ctrl Pts',(38.4516087667327,89.2216531649094,107.));
#48403=CARTESIAN_POINT('Ctrl Pts',(38.3946220233629,89.2835732787236,107.));
#48404=CARTESIAN_POINT('Ctrl Pts',(38.3736544685896,89.306356005042,107.));
#48405=CARTESIAN_POINT('Ctrl Pts',(38.3522228215257,89.3287335608056,107.));
#48406=CARTESIAN_POINT('Ctrl Pts',(38.3303262530622,89.3506857817386,107.));
#48407=CARTESIAN_POINT('Ctrl Pts',(38.3112488181976,89.3698117039432,107.));
#48408=CARTESIAN_POINT('Ctrl Pts',(38.2918184498306,89.388614739825,107.));
#48409=CARTESIAN_POINT('Ctrl Pts',(38.2720452848187,89.4070897608438,107.));
#48410=CARTESIAN_POINT('Origin',(36.3549260746835,87.7685555885722,124.208423447177));
#48411=CARTESIAN_POINT('Ctrl Pts',(33.2781263393751,87.7704832126688,121.708423447178));
#48412=CARTESIAN_POINT('Ctrl Pts',(33.2772036629102,87.8937581312653,121.702019850418));
#48413=CARTESIAN_POINT('Ctrl Pts',(33.3397301729486,89.0296650804786,121.642966745928));
#48414=CARTESIAN_POINT('Ctrl Pts',(34.7524571937242,91.0220941552736,121.531264133707));
#48415=CARTESIAN_POINT('Ctrl Pts',(38.2031235999269,90.8887189946743,121.373315610515));
#48416=CARTESIAN_POINT('Ctrl Pts',(39.9780137505041,87.9267773350827,121.215367087322));
#48417=CARTESIAN_POINT('Ctrl Pts',(38.4679953904151,84.8211908407143,121.05741856413));
#48418=CARTESIAN_POINT('Ctrl Pts',(35.0421043825414,84.3879826953392,120.899470040937));
#48419=CARTESIAN_POINT('Ctrl Pts',(33.395557307013,86.3263540715381,120.783138335286));
#48420=CARTESIAN_POINT('Ctrl Pts',(33.2786796709839,87.5529959098163,120.719456137367));
#48421=CARTESIAN_POINT('Ctrl Pts',(33.2806115013714,87.7658718718852,120.708423447177));
#48422=CARTESIAN_POINT('Ctrl Pts',(33.2846474150427,87.7655400361928,121.791576552823));
#48423=CARTESIAN_POINT('Ctrl Pts',(33.2896323871427,88.4585586466148,121.755752019753));
#48424=CARTESIAN_POINT('Ctrl Pts',(33.8620199088269,90.1797490256915,121.667277978953));
#48425=CARTESIAN_POINT('Ctrl Pts',(36.7064604291151,91.377416630034,121.526154430423));
#48426=CARTESIAN_POINT('Ctrl Pts',(39.5688530544509,89.4482951162593,121.36820590723));
#48427=CARTESIAN_POINT('Ctrl Pts',(39.5184627418672,85.9950129791182,121.210257384038));
#48428=CARTESIAN_POINT('Ctrl Pts',(36.5992128862014,84.1503276493198,121.052308860845));
#48429=CARTESIAN_POINT('Ctrl Pts',(33.8243657798026,85.4187697348352,120.912748583773));
#48430=CARTESIAN_POINT('Ctrl Pts',(33.2888359933922,87.1075071762337,120.825837814433));
#48431=CARTESIAN_POINT('Ctrl Pts',(33.2844847704405,87.7707064707598,120.791576552823));
#48432=CARTESIAN_POINT('Ctrl Pts',(38.2683920713486,89.4045427919472,122.));
#48433=CARTESIAN_POINT('Ctrl Pts',(38.8095874576702,88.7715555857257,121.947350492269));
#48434=CARTESIAN_POINT('Ctrl Pts',(39.2049245857504,86.9365225932413,121.842051476808));
#48435=CARTESIAN_POINT('Ctrl Pts',(37.214127277114,84.9233560515254,121.684102953615));
#48436=CARTESIAN_POINT('Ctrl Pts',(34.4432236387825,85.4956001255505,121.526154430423));
#48437=CARTESIAN_POINT('Ctrl Pts',(33.4061067692024,88.125867342332,121.36820590723));
#48438=CARTESIAN_POINT('Ctrl Pts',(35.0423458216121,90.4335249530331,121.210257384038));
#48439=CARTESIAN_POINT('Ctrl Pts',(37.8687823524776,90.3242775260579,121.052308860845));
#48440=CARTESIAN_POINT('Ctrl Pts',(39.3225926515107,87.8981548229434,120.894360337653));
#48441=CARTESIAN_POINT('Ctrl Pts',(38.0857385042766,85.3543728155993,120.73641181446));
#48442=CARTESIAN_POINT('Ctrl Pts',(35.2795954711475,84.999532566378,120.578463291268));
#48443=CARTESIAN_POINT('Ctrl Pts',(33.4484287478634,87.1552444887491,120.420514768075));
#48444=CARTESIAN_POINT('Ctrl Pts',(34.2524914687833,89.8670448178538,120.262566244883));
#48445=CARTESIAN_POINT('Ctrl Pts',(36.9627693013253,90.6762000895379,120.10461772169));
#48446=CARTESIAN_POINT('Ctrl Pts',(39.1219333904769,88.8490867521255,119.946669198498));
#48447=CARTESIAN_POINT('Ctrl Pts',(38.7723364786591,86.0422866159873,119.788720675305));
#48448=CARTESIAN_POINT('Ctrl Pts',(36.2309468922132,84.800643054622,119.630772152113));
#48449=CARTESIAN_POINT('Ctrl Pts',(33.8019655491018,86.2499150368912,119.472823628921));
#48450=CARTESIAN_POINT('Ctrl Pts',(33.6876758263602,89.0760924562573,119.314875105728));
#48451=CARTESIAN_POINT('Ctrl Pts',(35.9917008041203,90.7167658497645,119.156926582536));
#48452=CARTESIAN_POINT('Ctrl Pts',(38.625051077446,89.6843867210575,118.998978059343));
#48453=CARTESIAN_POINT('Ctrl Pts',(39.2001480584847,86.9149817447435,118.841029536151));
#48454=CARTESIAN_POINT('Ctrl Pts',(37.1955687979013,84.9194862255556,118.683081012958));
#48455=CARTESIAN_POINT('Ctrl Pts',(34.4288043483479,85.5071552408685,118.525132489766));
#48456=CARTESIAN_POINT('Ctrl Pts',(33.4083958871456,88.1451671771827,118.367183966573));
#48457=CARTESIAN_POINT('Ctrl Pts',(35.0595167325978,90.44171683871,118.209235443381));
#48458=CARTESIAN_POINT('Ctrl Pts',(37.8851458302896,90.3145924959996,118.051286920188));
#48459=CARTESIAN_POINT('Ctrl Pts',(39.3233712151692,87.8790539231783,117.893338396996));
#48460=CARTESIAN_POINT('Ctrl Pts',(38.0701976723164,85.343329871199,117.735389873803));
#48461=CARTESIAN_POINT('Ctrl Pts',(35.2618395395329,85.0064842171713,117.577441350611));
#48462=CARTESIAN_POINT('Ctrl Pts',(33.4445497234387,87.1739246710306,117.419492827418));
#48463=CARTESIAN_POINT('Ctrl Pts',(34.2660096299264,89.8804988929231,117.261544304226));
#48464=CARTESIAN_POINT('Ctrl Pts',(36.9814265453518,90.6722383526224,117.103595781034));
#48465=CARTESIAN_POINT('Ctrl Pts',(39.1288145381736,88.831296961672,116.945647257841));
#48466=CARTESIAN_POINT('Ctrl Pts',(38.7612022251526,86.0268002895521,116.787698734649));
#48467=CARTESIAN_POINT('Ctrl Pts',(36.2118925100824,84.8015001739599,116.629750211456));
#48468=CARTESIAN_POINT('Ctrl Pts',(33.7922669778667,86.2663389638858,116.471801688264));
#48469=CARTESIAN_POINT('Ctrl Pts',(33.6961265089816,89.0931918795614,116.313853165071));
#48470=CARTESIAN_POINT('Ctrl Pts',(36.010638742585,90.7190373571888,116.155904641879));
#48471=CARTESIAN_POINT('Ctrl Pts',(38.6373058291762,89.6697707500582,115.997956118686));
#48472=CARTESIAN_POINT('Ctrl Pts',(39.1946086078113,86.8967301788536,115.840007595494));
#48473=CARTESIAN_POINT('Ctrl Pts',(37.1772575986997,84.9141471912696,115.682059072301));
#48474=CARTESIAN_POINT('Ctrl Pts',(34.4143236068453,85.5195694846129,115.524110549109));
#48475=CARTESIAN_POINT('Ctrl Pts',(33.4108748518238,88.1640790785956,115.366162025916));
#48476=CARTESIAN_POINT('Ctrl Pts',(35.0767078012988,90.4499795534774,115.208213502724));
#48477=CARTESIAN_POINT('Ctrl Pts',(37.9014623840002,90.3047144712031,115.050264979531));
#48478=CARTESIAN_POINT('Ctrl Pts',(39.3240195308199,87.8599912638331,114.892316456339));
#48479=CARTESIAN_POINT('Ctrl Pts',(38.0545899418562,85.3323661105944,114.734367933147));
#48480=CARTESIAN_POINT('Ctrl Pts',(35.2441268174668,85.0135598636845,114.576419409954));
#48481=CARTESIAN_POINT('Ctrl Pts',(33.4407915961636,87.192624451123,114.418470886762));
#48482=CARTESIAN_POINT('Ctrl Pts',(34.2796134771405,89.8938682847329,114.260522363569));
#48483=CARTESIAN_POINT('Ctrl Pts',(37.0000581725303,90.6681557351977,114.102573840377));
#48484=CARTESIAN_POINT('Ctrl Pts',(39.1355812156081,88.8134639200691,113.944625317184));
#48485=CARTESIAN_POINT('Ctrl Pts',(38.7499688122129,86.0113855002229,113.786676793992));
#48486=CARTESIAN_POINT('Ctrl Pts',(36.1928440006319,84.8024797575703,113.628728270799));
#48487=CARTESIAN_POINT('Ctrl Pts',(33.78267407609,86.2828247617688,113.470779747607));
#48488=CARTESIAN_POINT('Ctrl Pts',(33.7046868071648,89.1102367201694,113.312831224414));
#48489=CARTESIAN_POINT('Ctrl Pts',(36.0295908787149,90.7211872019379,113.154882701222));
#48490=CARTESIAN_POINT('Ctrl Pts',(38.6494664778272,89.6550764000991,112.996934178029));
#48491=CARTESIAN_POINT('Ctrl Pts',(39.1889520787008,86.8785145543856,112.838985654837));
#48492=CARTESIAN_POINT('Ctrl Pts',(37.1589124947367,84.9089258449949,112.681037131644));
#48493=CARTESIAN_POINT('Ctrl Pts',(34.3999228758519,85.5320764523986,112.523088608452));
#48494=CARTESIAN_POINT('Ctrl Pts',(33.4134751986133,88.1829746731326,112.365140085259));
#48495=CARTESIAN_POINT('Ctrl Pts',(35.093951570523,90.4581317138827,112.207191562067));
#48496=CARTESIAN_POINT('Ctrl Pts',(37.9177151745493,90.2947318815738,112.049243038874));
#48497=CARTESIAN_POINT('Ctrl Pts',(39.3245454318088,87.8409248345793,111.891294515682));
#48498=CARTESIAN_POINT('Ctrl Pts',(38.0389121348537,85.3215027932418,111.73334599249));
#48499=CARTESIAN_POINT('Ctrl Pts',(35.2264598932615,85.0207490976825,111.575397469297));
#48500=CARTESIAN_POINT('Ctrl Pts',(33.4371536176206,87.2113479766595,111.417448946105));
#48501=CARTESIAN_POINT('Ctrl Pts',(34.2933028887537,89.9071500506473,111.259500422912));
#48502=CARTESIAN_POINT('Ctrl Pts',(37.018663201149,90.6639535682966,111.10155189972));
#48503=CARTESIAN_POINT('Ctrl Pts',(39.1422332476006,88.795587797249,110.943603376527));
#48504=CARTESIAN_POINT('Ctrl Pts',(38.7386366525448,85.9960431584279,110.785654853335));
#48505=CARTESIAN_POINT('Ctrl Pts',(36.1738021736971,84.8035816313644,110.627706330142));
#48506=CARTESIAN_POINT('Ctrl Pts',(33.7731872274968,86.299371815953,110.46975780695));
#48507=CARTESIAN_POINT('Ctrl Pts',(33.7133563734736,89.1272262434396,110.311809283757));
#48508=CARTESIAN_POINT('Ctrl Pts',(36.0485564289157,90.7232153113506,110.153860760565));
#48509=CARTESIAN_POINT('Ctrl Pts',(38.6615325221239,89.6403042682848,109.995912237372));
#48510=CARTESIAN_POINT('Ctrl Pts',(39.1831787063092,86.8603356286082,109.83796371418));
#48511=CARTESIAN_POINT('Ctrl Pts',(37.1405342373388,84.9038223948635,109.680015190987));
#48512=CARTESIAN_POINT('Ctrl Pts',(34.3856027599713,85.5446756404848,109.522066667795));
#48513=CARTESIAN_POINT('Ctrl Pts',(33.4161967977053,88.2018531585721,109.364118144603));
#48514=CARTESIAN_POINT('Ctrl Pts',(35.1112473759147,90.466173030801,109.20616962141));
#48515=CARTESIAN_POINT('Ctrl Pts',(37.9339034359386,90.2846450423694,109.048221098218));
#48516=CARTESIAN_POINT('Ctrl Pts',(39.3249490937297,87.8218556194758,108.890272575025));
#48517=CARTESIAN_POINT('Ctrl Pts',(38.0231644919314,85.3107399599536,108.732324051833));
#48518=CARTESIAN_POINT('Ctrl Pts',(35.2088403298994,85.0280524599893,108.57437552864));
#48519=CARTESIAN_POINT('Ctrl Pts',(33.4336342212486,87.2300927536877,108.416427005448));
#48520=CARTESIAN_POINT('Ctrl Pts',(34.3070808309297,89.9203471848041,108.258478482255));
#48521=CARTESIAN_POINT('Ctrl Pts',(37.0372336025185,90.6596247405995,108.100529959063));
#48522=CARTESIAN_POINT('Ctrl Pts',(39.1487852954204,88.7776843129956,107.94258143587));
#48523=CARTESIAN_POINT('Ctrl Pts',(38.7271754942787,85.9807430805063,107.784632912678));
#48524=CARTESIAN_POINT('Ctrl Pts',(36.1548309967493,84.8048691322566,107.626684389485));
#48525=CARTESIAN_POINT('Ctrl Pts',(33.7636768703791,86.3158490815793,107.468735866293));
#48526=CARTESIAN_POINT('Ctrl Pts',(33.7224021344473,89.1444279263405,107.310787343101));
#48527=CARTESIAN_POINT('Ctrl Pts',(36.0669846911716,90.7245702197898,107.152838819908));
#48528=CARTESIAN_POINT('Ctrl Pts',(38.6746345709313,89.6266028442429,106.994890296716));
#48529=CARTESIAN_POINT('Ctrl Pts',(39.1749134210556,86.8398781501125,106.836941773523));
#48530=CARTESIAN_POINT('Ctrl Pts',(37.8096764711452,85.5515592459026,106.731642758061));
#48531=CARTESIAN_POINT('Ctrl Pts',(37.0051260726581,85.336468786537,106.678993250331));
#48532=CARTESIAN_POINT('Ctrl Pts',(38.4092576250256,89.5249809097991,122.10700224989));
#48533=CARTESIAN_POINT('Ctrl Pts',(38.9902947372387,88.8453944468204,122.054352742159));
#48534=CARTESIAN_POINT('Ctrl Pts',(39.4147357968929,86.8752699821318,121.949053726697));
#48535=CARTESIAN_POINT('Ctrl Pts',(37.2773799574915,84.7138981312874,121.791105203505));
#48536=CARTESIAN_POINT('Ctrl Pts',(34.3024879149346,85.3282696737212,121.633156680312));
#48537=CARTESIAN_POINT('Ctrl Pts',(33.1890205680971,88.1521719216224,121.47520815712));
#48538=CARTESIAN_POINT('Ctrl Pts',(34.9457162789828,90.6297146871132,121.317259633927));
#48539=CARTESIAN_POINT('Ctrl Pts',(37.9802294349607,90.5124246822634,121.159311110735));
#48540=CARTESIAN_POINT('Ctrl Pts',(39.5410663511752,87.9076956603232,121.001362587542));
#48541=CARTESIAN_POINT('Ctrl Pts',(38.2131574663228,85.1766454906377,120.84341406435));
#48542=CARTESIAN_POINT('Ctrl Pts',(35.2004317749455,84.7956826093651,120.685465541158));
#48543=CARTESIAN_POINT('Ctrl Pts',(33.2344582064914,87.1100937477359,120.527517017965));
#48544=CARTESIAN_POINT('Ctrl Pts',(34.0977144226554,90.0215314132171,120.369568494773));
#48545=CARTESIAN_POINT('Ctrl Pts',(37.0075175084107,90.8902550835844,120.21161997158));
#48546=CARTESIAN_POINT('Ctrl Pts',(39.3256349552013,88.9286333031928,120.053671448388));
#48547=CARTESIAN_POINT('Ctrl Pts',(38.9503014153834,85.9152021341922,119.895722925195));
#48548=CARTESIAN_POINT('Ctrl Pts',(36.2218197918553,84.5821512480842,119.737774402003));
#48549=CARTESIAN_POINT('Ctrl Pts',(33.614021682538,86.1381157456983,119.57982587881));
#48550=CARTESIAN_POINT('Ctrl Pts',(33.4913181781552,89.1723507149046,119.421877355618));
#48551=CARTESIAN_POINT('Ctrl Pts',(35.9649608835069,90.9338072142428,119.263928832425));
#48552=CARTESIAN_POINT('Ctrl Pts',(38.7921731564312,89.8254263913206,119.105980309233));
#48553=CARTESIAN_POINT('Ctrl Pts',(39.4096076312081,86.8521433392924,118.94803178604));
#48554=CARTESIAN_POINT('Ctrl Pts',(37.2574552400211,84.7097434164411,118.790083262848));
#48555=CARTESIAN_POINT('Ctrl Pts',(34.2870071050718,85.3406754536029,118.632134739656));
#48556=CARTESIAN_POINT('Ctrl Pts',(33.1914782063417,88.1728925718556,118.474186216463));
#48557=CARTESIAN_POINT('Ctrl Pts',(34.9641512782186,90.6385096430895,118.316237693271));
#48558=CARTESIAN_POINT('Ctrl Pts',(37.9977975594013,90.5020266595918,118.158289170078));
#48559=CARTESIAN_POINT('Ctrl Pts',(39.5419022311388,87.8871885903799,118.000340646886));
#48560=CARTESIAN_POINT('Ctrl Pts',(38.1964725492822,85.1647895866762,117.842392123693));
#48561=CARTESIAN_POINT('Ctrl Pts',(35.1813686870279,84.803146026837,117.684443600501));
#48562=CARTESIAN_POINT('Ctrl Pts',(33.2302936160184,87.1301491278129,117.526495077308));
#48563=CARTESIAN_POINT('Ctrl Pts',(34.112227763884,90.0359759504825,117.368546554116));
#48564=CARTESIAN_POINT('Ctrl Pts',(37.0275482615639,90.8860016914921,117.210598030923));
#48565=CARTESIAN_POINT('Ctrl Pts',(39.3330226792793,88.909533863816,117.052649507731));
#48566=CARTESIAN_POINT('Ctrl Pts',(38.9383474803212,85.8985757352649,116.894700984538));
#48567=CARTESIAN_POINT('Ctrl Pts',(36.201362664082,84.5830714668398,116.736752461346));
#48568=CARTESIAN_POINT('Ctrl Pts',(33.6036091218151,86.15574876947,116.578803938153));
#48569=CARTESIAN_POINT('Ctrl Pts',(33.5003909831914,89.1907089636779,116.420855414961));
#48570=CARTESIAN_POINT('Ctrl Pts',(35.9852929952633,90.9362459455173,116.262906891768));
#48571=CARTESIAN_POINT('Ctrl Pts',(38.8053300785636,89.8097344216618,116.104958368576));
#48572=CARTESIAN_POINT('Ctrl Pts',(39.4036603772148,86.8325481294921,115.947009845384));
#48573=CARTESIAN_POINT('Ctrl Pts',(37.2377960068232,84.7040113330902,115.789061322191));
#48574=CARTESIAN_POINT('Ctrl Pts',(34.2714603202359,85.3540036092337,115.631112798999));
#48575=CARTESIAN_POINT('Ctrl Pts',(33.1941396674596,88.1931967297645,115.473164275806));
#48576=CARTESIAN_POINT('Ctrl Pts',(34.9826079191403,90.6473806424528,115.315215752614));
#48577=CARTESIAN_POINT('Ctrl Pts',(38.0153153052819,90.4914214342938,115.157267229421));
#48578=CARTESIAN_POINT('Ctrl Pts',(39.5425982744958,87.8667225760403,114.999318706229));
#48579=CARTESIAN_POINT('Ctrl Pts',(38.1797158088073,85.1530186958635,114.841370183036));
#48580=CARTESIAN_POINT('Ctrl Pts',(35.1623519896598,84.810742568347,114.683421659844));
#48581=CARTESIAN_POINT('Ctrl Pts',(33.2262588229021,87.1502255484521,114.525473136651));
#48582=CARTESIAN_POINT('Ctrl Pts',(34.1268330992215,90.0503295702762,114.367524613459));
#48583=CARTESIAN_POINT('Ctrl Pts',(37.0475515120076,90.8816185199078,114.209576090267));
#48584=CARTESIAN_POINT('Ctrl Pts',(39.3402875060225,88.8903879892268,114.051627567074));
#48585=CARTESIAN_POINT('Ctrl Pts',(38.9262870859059,85.8820261398624,113.893679043881));
#48586=CARTESIAN_POINT('Ctrl Pts',(36.1809118413241,84.5841231654436,113.735730520689));
#48587=CARTESIAN_POINT('Ctrl Pts',(33.5933100097256,86.1734482189416,113.577781997497));
#48588=CARTESIAN_POINT('Ctrl Pts',(33.5095814734685,89.2090086114858,113.419833474304));
#48589=CARTESIAN_POINT('Ctrl Pts',(36.005640349889,90.9385540575528,113.261884951112));
#48590=CARTESIAN_POINT('Ctrl Pts',(38.8183859699355,89.7939583029403,113.103936427919));
#48591=CARTESIAN_POINT('Ctrl Pts',(39.397587425703,86.8129915070493,112.945987904727));
#48592=CARTESIAN_POINT('Ctrl Pts',(37.218100372863,84.6984056017074,112.788039381534));
#48593=CARTESIAN_POINT('Ctrl Pts',(34.2559994361233,85.3674313150648,112.630090858342));
#48594=CARTESIAN_POINT('Ctrl Pts',(33.1969314465981,88.2134833803179,112.472142335149));
#48595=CARTESIAN_POINT('Ctrl Pts',(35.0011211402929,90.656132948662,112.314193811957));
#48596=CARTESIAN_POINT('Ctrl Pts',(38.032764593884,90.4807039463087,112.156245288764));
#48597=CARTESIAN_POINT('Ctrl Pts',(39.5431628912675,87.8462525142588,111.998296765572));
#48598=CARTESIAN_POINT('Ctrl Pts',(38.1628838328947,85.141355642735,111.840348242379));
#48599=CARTESIAN_POINT('Ctrl Pts',(35.1433844616997,84.8184610594256,111.682399719187));
#48600=CARTESIAN_POINT('Ctrl Pts',(33.2223530236282,87.1703274626279,111.524451195995));
#48601=CARTESIAN_POINT('Ctrl Pts',(34.1415302980385,90.0645891133304,111.366502672802));
#48602=CARTESIAN_POINT('Ctrl Pts',(37.0675262057587,90.8771069978532,111.20855414961));
#48603=CARTESIAN_POINT('Ctrl Pts',(39.3474292473546,88.8711958618666,111.050605626417));
#48604=CARTESIAN_POINT('Ctrl Pts',(38.9141206752248,85.8655543254375,110.892657103225));
#48605=CARTESIAN_POINT('Ctrl Pts',(36.1604681930353,84.5853061569907,110.734708580032));
#48606=CARTESIAN_POINT('Ctrl Pts',(33.5831247582434,86.1912134342811,110.57676005684));
#48607=CARTESIAN_POINT('Ctrl Pts',(33.5188892759731,89.2272488696041,110.418811533647));
#48608=CARTESIAN_POINT('Ctrl Pts',(36.0260021061025,90.9407314723389,110.260863010455));
#48609=CARTESIAN_POINT('Ctrl Pts',(38.8313402923692,89.7780986762186,110.102914487262));
#48610=CARTESIAN_POINT('Ctrl Pts',(39.3913890291405,86.7934742849815,109.94496596407));
#48611=CARTESIAN_POINT('Ctrl Pts',(37.1983691447782,84.6929264457471,109.787017440877));
#48612=CARTESIAN_POINT('Ctrl Pts',(34.2406251018475,85.3809580302714,109.629068917685));
#48613=CARTESIAN_POINT('Ctrl Pts',(33.1998534043918,88.2337516622358,109.471120394492));
#48614=CARTESIAN_POINT('Ctrl Pts',(35.0196902284118,90.664766251308,109.3131718713));
#48615=CARTESIAN_POINT('Ctrl Pts',(38.0501446028181,90.469874534102,109.155223348107));
#48616=CARTESIAN_POINT('Ctrl Pts',(39.5435962699747,87.8257794615391,108.997274824915));
#48617=CARTESIAN_POINT('Ctrl Pts',(38.145976879881,85.1298004711073,108.839326301723));
#48618=CARTESIAN_POINT('Ctrl Pts',(35.1244677811938,84.826302080712,108.68137777853));
#48619=CARTESIAN_POINT('Ctrl Pts',(33.2185745363085,87.1904521927878,108.523429255338));
#48620=CARTESIAN_POINT('Ctrl Pts',(34.1563225448619,90.0787577942057,108.365480732145));
#48621=CARTESIAN_POINT('Ctrl Pts',(37.0874637230715,90.8724594904871,108.207532208953));
#48622=CARTESIAN_POINT('Ctrl Pts',(39.3544636438785,88.8519743587791,108.04958368576));
#48623=CARTESIAN_POINT('Ctrl Pts',(38.901815769326,85.849127886268,107.891635162568));
#48624=CARTESIAN_POINT('Ctrl Pts',(36.1401003958448,84.5866884411331,107.733686639375));
#48625=CARTESIAN_POINT('Ctrl Pts',(33.5729142675862,86.2089037233683,107.575738116183));
#48626=CARTESIAN_POINT('Ctrl Pts',(33.5286009678439,89.245716906122,107.41778959299));
#48627=CARTESIAN_POINT('Ctrl Pts',(36.0457870203034,90.9421861264375,107.259841069798));
#48628=CARTESIAN_POINT('Ctrl Pts',(38.845406887901,89.7633885806419,107.101892546605));
#48629=CARTESIAN_POINT('Ctrl Pts',(39.382515270057,86.771510767685,106.943944023413));
#48630=CARTESIAN_POINT('Ctrl Pts',(37.916772296426,85.388348393003,106.838645007951));
#48631=CARTESIAN_POINT('Ctrl Pts',(37.052992500844,85.1574234026335,106.78599550022));
#48632=CARTESIAN_POINT('Ctrl Pts',(38.5501231787026,89.645419027651,122.21400449978));
#48633=CARTESIAN_POINT('Ctrl Pts',(39.1710020168071,88.919233307915,122.161354992049));
#48634=CARTESIAN_POINT('Ctrl Pts',(39.6245470080353,86.8140173710224,122.056055976587));
#48635=CARTESIAN_POINT('Ctrl Pts',(37.3406326378691,84.5044402110492,121.898107453395));
#48636=CARTESIAN_POINT('Ctrl Pts',(34.1617521910867,85.160939221892,121.740158930202));
#48637=CARTESIAN_POINT('Ctrl Pts',(32.9719343669918,88.1784765009128,121.58221040701));
#48638=CARTESIAN_POINT('Ctrl Pts',(34.8490867363534,90.8259044211933,121.424261883817));
#48639=CARTESIAN_POINT('Ctrl Pts',(38.0916765174438,90.700571838469,121.266313360625));
#48640=CARTESIAN_POINT('Ctrl Pts',(39.7595400508396,87.9172364977028,121.108364837432));
#48641=CARTESIAN_POINT('Ctrl Pts',(38.3405764283689,84.9989181656761,120.95041631424));
#48642=CARTESIAN_POINT('Ctrl Pts',(35.1212680787434,84.5918326523521,120.792467791047));
#48643=CARTESIAN_POINT('Ctrl Pts',(33.0204876651193,87.0649430067228,120.634519267855));
#48644=CARTESIAN_POINT('Ctrl Pts',(33.9429373765276,90.1760180085803,120.476570744662));
#48645=CARTESIAN_POINT('Ctrl Pts',(37.0522657154962,91.104310077631,120.31862222147));
#48646=CARTESIAN_POINT('Ctrl Pts',(39.5293365199257,89.0081798542601,120.160673698278));
#48647=CARTESIAN_POINT('Ctrl Pts',(39.1282663521078,85.7881176523972,120.002725175085));
#48648=CARTESIAN_POINT('Ctrl Pts',(36.2126926914973,84.3636594415466,119.844776651893));
#48649=CARTESIAN_POINT('Ctrl Pts',(33.4260778159742,86.0263164545053,119.6868281287));
#48650=CARTESIAN_POINT('Ctrl Pts',(33.2949605299503,89.2686089735517,119.528879605508));
#48651=CARTESIAN_POINT('Ctrl Pts',(35.9382209628934,91.1508485787212,119.370931082315));
#48652=CARTESIAN_POINT('Ctrl Pts',(38.9592952354164,89.9664660615837,119.212982559123));
#48653=CARTESIAN_POINT('Ctrl Pts',(39.6190672039315,86.7893049338414,119.05503403593));
#48654=CARTESIAN_POINT('Ctrl Pts',(37.3193416821408,84.5000006073266,118.897085512738));
#48655=CARTESIAN_POINT('Ctrl Pts',(34.1452098617957,85.1741956663374,118.739136989545));
#48656=CARTESIAN_POINT('Ctrl Pts',(32.9745605255379,88.2006179665285,118.581188466353));
#48657=CARTESIAN_POINT('Ctrl Pts',(34.8687858238393,90.8353024474691,118.42323994316));
#48658=CARTESIAN_POINT('Ctrl Pts',(38.1104492885132,90.6894608231839,118.265291419968));
#48659=CARTESIAN_POINT('Ctrl Pts',(39.7604332471084,87.8953232575818,118.107342896775));
#48660=CARTESIAN_POINT('Ctrl Pts',(38.3227474262479,84.9862493021531,117.949394373583));
#48661=CARTESIAN_POINT('Ctrl Pts',(35.1008978345229,84.5998078365029,117.79144585039));
#48662=CARTESIAN_POINT('Ctrl Pts',(33.016037508598,87.0863735845948,117.633497327198));
#48663=CARTESIAN_POINT('Ctrl Pts',(33.9584458978417,90.1914530080422,117.475548804005));
#48664=CARTESIAN_POINT('Ctrl Pts',(37.0736699777759,91.0997650303614,117.317600280813));
#48665=CARTESIAN_POINT('Ctrl Pts',(39.537230820385,88.9877707659602,117.159651757621));
#48666=CARTESIAN_POINT('Ctrl Pts',(39.1154927354898,85.7703511809776,117.001703234428));
#48667=CARTESIAN_POINT('Ctrl Pts',(36.1908328180816,84.3646427597196,116.843754711236));
#48668=CARTESIAN_POINT('Ctrl Pts',(33.4149512657634,86.0451585750542,116.685806188043));
#48669=CARTESIAN_POINT('Ctrl Pts',(33.3046554574013,89.2882260477943,116.527857664851));
#48670=CARTESIAN_POINT('Ctrl Pts',(35.9599472479417,91.1534545338459,116.369909141658));
#48671=CARTESIAN_POINT('Ctrl Pts',(38.9733543279509,89.9496980932653,116.211960618466));
#48672=CARTESIAN_POINT('Ctrl Pts',(39.6127121466181,86.7683660801305,116.054012095273));
#48673=CARTESIAN_POINT('Ctrl Pts',(37.2983344149467,84.4938754749107,115.896063572081));
#48674=CARTESIAN_POINT('Ctrl Pts',(34.1285970336264,85.1884377338545,115.738115048889));
#48675=CARTESIAN_POINT('Ctrl Pts',(32.9774044830955,88.2223143809333,115.580166525696));
#48676=CARTESIAN_POINT('Ctrl Pts',(34.8885080369818,90.8447817314284,115.422218002503));
#48677=CARTESIAN_POINT('Ctrl Pts',(38.1291682265636,90.6781283973845,115.264269479311));
#48678=CARTESIAN_POINT('Ctrl Pts',(39.7611770181716,87.8734538882476,115.106320956119));
#48679=CARTESIAN_POINT('Ctrl Pts',(38.3048416757584,84.9736712811325,114.948372432926));
#48680=CARTESIAN_POINT('Ctrl Pts',(35.0805771618529,84.6079252730093,114.790423909734));
#48681=CARTESIAN_POINT('Ctrl Pts',(33.0117260496407,87.1078266457813,114.632475386541));
#48682=CARTESIAN_POINT('Ctrl Pts',(33.9740527213024,90.2067908558194,114.474526863349));
#48683=CARTESIAN_POINT('Ctrl Pts',(37.095044851485,91.0950813046181,114.316578340156));
#48684=CARTESIAN_POINT('Ctrl Pts',(39.5449937964367,88.9673120583842,114.158629816964));
#48685=CARTESIAN_POINT('Ctrl Pts',(39.1026053595989,85.752666779502,114.000681293771));
#48686=CARTESIAN_POINT('Ctrl Pts',(36.1689796820162,84.365766573317,113.842732770579));
#48687=CARTESIAN_POINT('Ctrl Pts',(33.403945943361,86.0640716761142,113.684784247386));
#48688=CARTESIAN_POINT('Ctrl Pts',(33.3144761397724,89.3077805028025,113.526835724194));
#48689=CARTESIAN_POINT('Ctrl Pts',(35.9816898210629,91.1559209131676,113.368887201001));
#48690=CARTESIAN_POINT('Ctrl Pts',(38.9873054620438,89.9328402057817,113.210938677809));
#48691=CARTESIAN_POINT('Ctrl Pts',(39.6062227727051,86.7474684597129,113.052990154616));
#48692=CARTESIAN_POINT('Ctrl Pts',(37.2772882509894,84.4878853584198,112.895041631424));
#48693=CARTESIAN_POINT('Ctrl Pts',(34.1120759963947,85.2027861777312,112.737093108232));
#48694=CARTESIAN_POINT('Ctrl Pts',(32.9803876945829,88.2439920875028,112.579144585039));
#48695=CARTESIAN_POINT('Ctrl Pts',(34.9082907100627,90.8541341834417,112.421196061847));
#48696=CARTESIAN_POINT('Ctrl Pts',(38.1478140132187,90.6666760110434,112.263247538654));
#48697=CARTESIAN_POINT('Ctrl Pts',(39.7617803507262,87.8515801939384,112.105299015462));
#48698=CARTESIAN_POINT('Ctrl Pts',(38.2868555309357,84.961208492228,111.947350492269));
#48699=CARTESIAN_POINT('Ctrl Pts',(35.0603090301378,84.6161730211687,111.789401969077));
#48700=CARTESIAN_POINT('Ctrl Pts',(33.0075524296359,87.1293069485963,111.631453445884));
#48701=CARTESIAN_POINT('Ctrl Pts',(33.9897577073232,90.2220281760135,111.473504922692));
#48702=CARTESIAN_POINT('Ctrl Pts',(37.1163892103684,91.0902604274099,111.315556399499));
#48703=CARTESIAN_POINT('Ctrl Pts',(39.5526252471086,88.9468039264842,111.157607876307));
#48704=CARTESIAN_POINT('Ctrl Pts',(39.0896046979049,85.735065492447,110.999659353114));
#48705=CARTESIAN_POINT('Ctrl Pts',(36.1471342123734,84.3670306826171,110.841710829922));
#48706=CARTESIAN_POINT('Ctrl Pts',(33.3930622889901,86.0830550526093,110.683762306729));
#48707=CARTESIAN_POINT('Ctrl Pts',(33.3244221784725,89.3272714957683,110.525813783537));
#48708=CARTESIAN_POINT('Ctrl Pts',(36.0034477832893,91.1582476333273,110.367865260344));
#48709=CARTESIAN_POINT('Ctrl Pts',(39.0011480626143,89.9158930841524,110.209916737152));
#48710=CARTESIAN_POINT('Ctrl Pts',(39.5995993519719,86.7266129413549,110.05196821396));
#48711=CARTESIAN_POINT('Ctrl Pts',(37.2562040522177,84.4820304966307,109.894019690767));
#48712=CARTESIAN_POINT('Ctrl Pts',(34.0956474437237,85.217240420058,109.736071167575));
#48713=CARTESIAN_POINT('Ctrl Pts',(32.9835100110784,88.2656501658994,109.578122644382));
#48714=CARTESIAN_POINT('Ctrl Pts',(34.9281330809089,90.863359471815,109.42017412119));
#48715=CARTESIAN_POINT('Ctrl Pts',(38.1663857696977,90.6551040258348,109.262225597997));
#48716=CARTESIAN_POINT('Ctrl Pts',(39.7622434462196,87.8297033036023,109.104277074805));
#48717=CARTESIAN_POINT('Ctrl Pts',(38.2687892678307,84.9488609822609,108.946328551612));
#48718=CARTESIAN_POINT('Ctrl Pts',(35.0400952324881,84.6245517014347,108.78838002842));
#48719=CARTESIAN_POINT('Ctrl Pts',(33.0035148513684,87.1508116318879,108.630431505227));
#48720=CARTESIAN_POINT('Ctrl Pts',(34.0055642587942,90.2371684036073,108.472482982035));
#48721=CARTESIAN_POINT('Ctrl Pts',(37.1376938436244,91.0852942403748,108.314534458842));
#48722=CARTESIAN_POINT('Ctrl Pts',(39.5601419923366,88.9262644045625,108.15658593565));
#48723=CARTESIAN_POINT('Ctrl Pts',(39.0764560443734,85.7175126920297,107.998637412457));
#48724=CARTESIAN_POINT('Ctrl Pts',(36.1253697949403,84.3685077500094,107.840688889265));
#48725=CARTESIAN_POINT('Ctrl Pts',(33.3821516647933,86.1019583651574,107.682740366072));
#48726=CARTESIAN_POINT('Ctrl Pts',(33.3347998012407,89.3470058859034,107.52479184288));
#48727=CARTESIAN_POINT('Ctrl Pts',(36.0245893494351,91.1598020330852,107.366843319687));
#48728=CARTESIAN_POINT('Ctrl Pts',(39.0161792048708,89.9001743170408,107.208894796495));
#48729=CARTESIAN_POINT('Ctrl Pts',(39.5901171190583,86.7031433852574,107.050946273303));
#48730=CARTESIAN_POINT('Ctrl Pts',(38.0238681217067,85.2251375401034,106.945647257841));
#48731=CARTESIAN_POINT('Ctrl Pts',(37.1008589290298,84.9783780187299,106.89299775011));
#48732=CARTESIAN_POINT('Ctrl Pts',(38.6909887323797,89.7658571455029,122.321006749669));
#48733=CARTESIAN_POINT('Ctrl Pts',(39.3517092963755,88.9930721690097,122.268357241939));
#48734=CARTESIAN_POINT('Ctrl Pts',(39.8343582191777,86.7527647599131,122.163058226477));
#48735=CARTESIAN_POINT('Ctrl Pts',(37.4038853182466,84.2949822908111,122.005109703285));
#48736=CARTESIAN_POINT('Ctrl Pts',(34.0210164672389,84.9936087700628,121.847161180092));
#48737=CARTESIAN_POINT('Ctrl Pts',(32.7548481658866,88.204781080203,121.6892126569));
#48738=CARTESIAN_POINT('Ctrl Pts',(34.7524571937242,91.0220941552736,121.531264133707));
#48739=CARTESIAN_POINT('Ctrl Pts',(38.2031235999269,90.8887189946743,121.373315610515));
#48740=CARTESIAN_POINT('Ctrl Pts',(39.9780137505041,87.9267773350827,121.215367087322));
#48741=CARTESIAN_POINT('Ctrl Pts',(38.4679953904151,84.8211908407143,121.05741856413));
#48742=CARTESIAN_POINT('Ctrl Pts',(35.0421043825414,84.3879826953392,120.899470040937));
#48743=CARTESIAN_POINT('Ctrl Pts',(32.8065171237473,87.0197922657097,120.741521517745));
#48744=CARTESIAN_POINT('Ctrl Pts',(33.7881603303997,90.3305046039434,120.583572994552));
#48745=CARTESIAN_POINT('Ctrl Pts',(37.0970139225816,91.3183650716777,120.42562447136));
#48746=CARTESIAN_POINT('Ctrl Pts',(39.7330380846501,89.0877264053273,120.267675948167));
#48747=CARTESIAN_POINT('Ctrl Pts',(39.3062312888321,85.6610331706022,120.109727424975));
#48748=CARTESIAN_POINT('Ctrl Pts',(36.2035655911394,84.1451676350087,119.951778901782));
#48749=CARTESIAN_POINT('Ctrl Pts',(33.2381339494103,85.9145171633124,119.79383037859));
#48750=CARTESIAN_POINT('Ctrl Pts',(33.0986028817453,89.3648672321989,119.635881855398));
#48751=CARTESIAN_POINT('Ctrl Pts',(35.91148104228,91.3678899431996,119.477933332205));
#48752=CARTESIAN_POINT('Ctrl Pts',(39.1264173144016,90.1075057318468,119.319984809013));
#48753=CARTESIAN_POINT('Ctrl Pts',(39.8285267766549,86.7264665283904,119.16203628582));
#48754=CARTESIAN_POINT('Ctrl Pts',(37.3812281242605,84.2902577982121,119.004087762628));
#48755=CARTESIAN_POINT('Ctrl Pts',(34.0034126185196,85.0077158790718,118.846139239435));
#48756=CARTESIAN_POINT('Ctrl Pts',(32.757642844734,88.2283433612014,118.688190716243));
#48757=CARTESIAN_POINT('Ctrl Pts',(34.7734203694599,91.0320952518487,118.53024219305));
#48758=CARTESIAN_POINT('Ctrl Pts',(38.223101017625,90.876894986776,118.372293669858));
#48759=CARTESIAN_POINT('Ctrl Pts',(39.9789642630779,87.9034579247835,118.214345146665));
#48760=CARTESIAN_POINT('Ctrl Pts',(38.4490223032137,84.8077090176302,118.056396623473));
#48761=CARTESIAN_POINT('Ctrl Pts',(35.020426982018,84.3964696461687,117.89844810028));
#48762=CARTESIAN_POINT('Ctrl Pts',(32.8017814011777,87.042598041377,117.740499577088));
#48763=CARTESIAN_POINT('Ctrl Pts',(33.8046640317993,90.3469300656019,117.582551053895));
#48764=CARTESIAN_POINT('Ctrl Pts',(37.1197916939879,91.3135283692309,117.424602530703));
#48765=CARTESIAN_POINT('Ctrl Pts',(39.7414389614906,89.0660076681044,117.26665400751));
#48766=CARTESIAN_POINT('Ctrl Pts',(39.2926379906584,85.6421266266902,117.108705484318));
#48767=CARTESIAN_POINT('Ctrl Pts',(36.1803029720811,84.1462140525996,116.950756961126));
#48768=CARTESIAN_POINT('Ctrl Pts',(33.2262934097118,85.9345683806384,116.792808437933));
#48769=CARTESIAN_POINT('Ctrl Pts',(33.1089199316111,89.3857431319108,116.634859914741));
#48770=CARTESIAN_POINT('Ctrl Pts',(35.93460150062,91.3706631221744,116.476911391548));
#48771=CARTESIAN_POINT('Ctrl Pts',(39.1413785773383,90.0896617648689,116.318962868356));
#48772=CARTESIAN_POINT('Ctrl Pts',(39.8217639160215,86.7041840307689,116.161014345163));
#48773=CARTESIAN_POINT('Ctrl Pts',(37.3588728230703,84.2837396167312,116.003065821971));
#48774=CARTESIAN_POINT('Ctrl Pts',(33.9857337470169,85.0228718584753,115.845117298778));
#48775=CARTESIAN_POINT('Ctrl Pts',(32.7606692987314,88.2514320321021,115.687168775586));
#48776=CARTESIAN_POINT('Ctrl Pts',(34.7944081548233,91.0421828204038,115.529220252393));
#48777=CARTESIAN_POINT('Ctrl Pts',(38.2430211478453,90.8648353604754,115.371271729201));
#48778=CARTESIAN_POINT('Ctrl Pts',(39.9797557618474,87.8801852004548,115.213323206008));
#48779=CARTESIAN_POINT('Ctrl Pts',(38.4299675427095,84.7943238664015,115.055374682816));
#48780=CARTESIAN_POINT('Ctrl Pts',(34.9988023340458,84.4051079776717,114.897426159623));
#48781=CARTESIAN_POINT('Ctrl Pts',(32.7971932763793,87.0654277431103,114.739477636431));
#48782=CARTESIAN_POINT('Ctrl Pts',(33.8212723433833,90.3632521413627,114.581529113238));
#48783=CARTESIAN_POINT('Ctrl Pts',(37.1425381909624,91.3085440893281,114.423580590046));
#48784=CARTESIAN_POINT('Ctrl Pts',(39.749700086851,89.0442361275419,114.265632066853));
#48785=CARTESIAN_POINT('Ctrl Pts',(39.2789236332919,85.6233074191414,114.107683543661));
#48786=CARTESIAN_POINT('Ctrl Pts',(36.1570475227083,84.1474099811903,113.949735020469));
#48787=CARTESIAN_POINT('Ctrl Pts',(33.2145818769966,85.954695133287,113.791786497276));
#48788=CARTESIAN_POINT('Ctrl Pts',(33.1193708060762,89.4065523941189,113.633837974084));
#48789=CARTESIAN_POINT('Ctrl Pts',(35.9577392922369,91.3732877687825,113.475889450891));
#48790=CARTESIAN_POINT('Ctrl Pts',(39.1562249541521,90.071722108623,113.317940927699));
#48791=CARTESIAN_POINT('Ctrl Pts',(39.8148581197072,86.6819454123766,113.159992404506));
#48792=CARTESIAN_POINT('Ctrl Pts',(37.3364761291159,84.2773651151324,113.002043881314));
#48793=CARTESIAN_POINT('Ctrl Pts',(33.9681525566661,85.0381410403975,112.844095358121));
#48794=CARTESIAN_POINT('Ctrl Pts',(32.7638439425676,88.2745007946881,112.686146834929));
#48795=CARTESIAN_POINT('Ctrl Pts',(34.8154602798326,91.0521354182212,112.528198311736));
#48796=CARTESIAN_POINT('Ctrl Pts',(38.2628634325534,90.8526480757781,112.370249788544));
#48797=CARTESIAN_POINT('Ctrl Pts',(39.9803978101849,87.856907873618,112.212301265351));
#48798=CARTESIAN_POINT('Ctrl Pts',(38.4108272289767,84.7810613417211,112.054352742159));
#48799=CARTESIAN_POINT('Ctrl Pts',(34.977233598576,84.4138849829118,111.896404218966));
#48800=CARTESIAN_POINT('Ctrl Pts',(32.7927518356436,87.0882864345648,111.738455695774));
#48801=CARTESIAN_POINT('Ctrl Pts',(33.837985116608,90.3794672386964,111.580507172581));
#48802=CARTESIAN_POINT('Ctrl Pts',(37.1652522149781,91.3034138569667,111.422558649389));
#48803=CARTESIAN_POINT('Ctrl Pts',(39.7578212468625,89.0224119911016,111.264610126197));
#48804=CARTESIAN_POINT('Ctrl Pts',(39.2650887205849,85.6045766594567,111.106661603004));
#48805=CARTESIAN_POINT('Ctrl Pts',(36.1338002317116,84.1487552082432,110.948713079812));
#48806=CARTESIAN_POINT('Ctrl Pts',(33.2029998197368,85.9748966709376,110.790764556619));
#48807=CARTESIAN_POINT('Ctrl Pts',(33.129955080972,89.4272941219325,110.632816033427));
#48808=CARTESIAN_POINT('Ctrl Pts',(35.980893460476,91.3757637943158,110.474867510234));
#48809=CARTESIAN_POINT('Ctrl Pts',(39.1709558328596,90.0536874920861,110.316918987042));
#48810=CARTESIAN_POINT('Ctrl Pts',(39.8078096748032,86.6597515977284,110.158970463849));
#48811=CARTESIAN_POINT('Ctrl Pts',(37.3140389596571,84.2711345475141,110.001021940657));
#48812=CARTESIAN_POINT('Ctrl Pts',(33.9506697855998,85.0535228098446,109.843073417464));
#48813=CARTESIAN_POINT('Ctrl Pts',(32.7671666177649,88.2975486695631,109.685124894272));
#48814=CARTESIAN_POINT('Ctrl Pts',(34.836575933406,91.0619526923221,109.527176371079));
#48815=CARTESIAN_POINT('Ctrl Pts',(38.2826269365773,90.8403335175675,109.369227847887));
#48816=CARTESIAN_POINT('Ctrl Pts',(39.9808906224645,87.8336271456654,109.211279324694));
#48817=CARTESIAN_POINT('Ctrl Pts',(38.3916016557803,84.7679214934147,109.053330801502));
#48818=CARTESIAN_POINT('Ctrl Pts',(34.9557226837823,84.4228013221572,108.89538227831));
#48819=CARTESIAN_POINT('Ctrl Pts',(32.7884551664283,87.1111710709882,108.737433755117));
#48820=CARTESIAN_POINT('Ctrl Pts',(33.8548059727263,90.3955790130086,108.579485231925));
#48821=CARTESIAN_POINT('Ctrl Pts',(37.1879239641774,91.2981289902626,108.421536708732));
#48822=CARTESIAN_POINT('Ctrl Pts',(39.7658203407947,89.0005544503459,108.26358818554));
#48823=CARTESIAN_POINT('Ctrl Pts',(39.2510963194207,85.5858974977915,108.105639662347));
#48824=CARTESIAN_POINT('Ctrl Pts',(36.1106391940357,84.1503270588856,107.947691139155));
#48825=CARTESIAN_POINT('Ctrl Pts',(33.1913890620005,85.9950130069465,107.789742615962));
#48826=CARTESIAN_POINT('Ctrl Pts',(33.1409986346373,89.4482948656848,107.63179409277));
#48827=CARTESIAN_POINT('Ctrl Pts',(36.0033916785668,91.377417939733,107.473845569577));
#48828=CARTESIAN_POINT('Ctrl Pts',(39.1869515218405,90.0369600534397,107.315897046385));
#48829=CARTESIAN_POINT('Ctrl Pts',(39.7977189680597,86.63477600283,107.157948523192));
#48830=CARTESIAN_POINT('Ctrl Pts',(38.1309639469874,85.0619266872038,107.052649507731));
#48831=CARTESIAN_POINT('Ctrl Pts',(37.1487253572157,84.7993326348264,107.));
#48832=CARTESIAN_POINT('Ctrl Pts',(38.2683920713486,89.4045427919472,122.));
#48833=CARTESIAN_POINT('Ctrl Pts',(38.3300002321833,89.3466462487923,122.));
#48834=CARTESIAN_POINT('Ctrl Pts',(38.3882392376497,89.285598943331,122.));
#48835=CARTESIAN_POINT('Ctrl Pts',(38.4431114755178,89.2217856950428,122.));
#48836=CARTESIAN_POINT('Ctrl Pts',(38.4994366457555,89.1562827701958,122.));
#48837=CARTESIAN_POINT('Ctrl Pts',(38.5522148311301,89.08786505576,122.));
#48838=CARTESIAN_POINT('Ctrl Pts',(38.6014231063109,89.0169002051877,122.));
#48839=CARTESIAN_POINT('Ctrl Pts',(38.6519809945774,88.9439890337863,122.));
#48840=CARTESIAN_POINT('Ctrl Pts',(38.6987709992573,88.8683885355143,122.));
#48841=CARTESIAN_POINT('Ctrl Pts',(38.7417341886229,88.7904544724489,122.));
#48842=CARTESIAN_POINT('Ctrl Pts',(38.7606441828022,88.7561522546505,122.));
#48843=CARTESIAN_POINT('Ctrl Pts',(38.778812335652,88.7213974646771,122.));
#48844=CARTESIAN_POINT('Ctrl Pts',(38.7962311971065,88.6862183602815,122.));
#48845=CARTESIAN_POINT('Ctrl Pts',(38.8061620426653,88.6661620406672,122.));
#48846=CARTESIAN_POINT('Ctrl Pts',(38.8158493123712,88.6459677823628,122.));
#48847=CARTESIAN_POINT('Ctrl Pts',(38.8252913913176,88.6256406734547,122.));
#48848=CARTESIAN_POINT('Ctrl Pts',(38.8337969724246,88.6073296770662,122.));
#48849=CARTESIAN_POINT('Ctrl Pts',(38.8421059629712,88.5889051485111,122.));
#48850=CARTESIAN_POINT('Ctrl Pts',(38.8502035219805,88.5704025618327,122.));
#48851=CARTESIAN_POINT('Ctrl Pts',(38.8867651008279,88.4868608697069,122.));
#48852=CARTESIAN_POINT('Ctrl Pts',(38.9190665018293,88.4016356337446,122.));
#48853=CARTESIAN_POINT('Ctrl Pts',(38.9470826910293,88.3151256326902,122.));
#48854=CARTESIAN_POINT('Ctrl Pts',(38.9755619804946,88.2271856439894,122.));
#48855=CARTESIAN_POINT('Ctrl Pts',(38.9996137137859,88.1379173104662,122.));
#48856=CARTESIAN_POINT('Ctrl Pts',(39.0191725198821,88.0477023902482,122.));
#48857=CARTESIAN_POINT('Ctrl Pts',(39.0381409703695,87.9602104830752,122.));
#48858=CARTESIAN_POINT('Ctrl Pts',(39.0528837825619,87.871827352317,122.));
#48859=CARTESIAN_POINT('Ctrl Pts',(39.0633005852989,87.7828793552042,122.));
#48860=CARTESIAN_POINT('Ctrl Pts',(39.0676694118452,87.7455743988912,122.));
#48861=CARTESIAN_POINT('Ctrl Pts',(39.0712767865467,87.7081698916346,122.));
#48862=CARTESIAN_POINT('Ctrl Pts',(39.0741129699685,87.6706892912553,122.));
#48863=CARTESIAN_POINT('Ctrl Pts',(39.0758920905351,87.6471779391791,122.));
#48864=CARTESIAN_POINT('Ctrl Pts',(39.077367720881,87.6236366391684,122.));
#48865=CARTESIAN_POINT('Ctrl Pts',(39.0785371609356,87.6000711486457,122.));
#48866=CARTESIAN_POINT('Ctrl Pts',(39.0792215402202,87.5862801608281,122.));
#48867=CARTESIAN_POINT('Ctrl Pts',(39.0798007649429,87.5724858346905,122.));
#48868=CARTESIAN_POINT('Ctrl Pts',(39.0802743343143,87.5586971611392,122.));
#48869=CARTESIAN_POINT('Ctrl Pts',(39.0836016907244,87.4618162518133,122.));
#48870=CARTESIAN_POINT('Ctrl Pts',(39.0817231359907,87.3651003513936,122.));
#48871=CARTESIAN_POINT('Ctrl Pts',(39.0745742900295,87.2689692279916,122.));
#48872=CARTESIAN_POINT('Ctrl Pts',(39.0674254440683,87.1728381045895,122.));
#48873=CARTESIAN_POINT('Ctrl Pts',(39.0550067371896,87.0772907141668,122.));
#48874=CARTESIAN_POINT('Ctrl Pts',(39.0372013263777,86.9827280393604,122.));
#48875=CARTESIAN_POINT('Ctrl Pts',(39.0201432921301,86.8921346033293,122.));
#48876=CARTESIAN_POINT('Ctrl Pts',(38.9981414058761,86.802443982858,122.));
#48877=CARTESIAN_POINT('Ctrl Pts',(38.9714702759697,86.7138955165579,122.));
#48878=CARTESIAN_POINT('Ctrl Pts',(38.9626009237809,86.6844491625357,122.));
#48879=CARTESIAN_POINT('Ctrl Pts',(38.9532147870399,86.6551291509939,122.));
#48880=CARTESIAN_POINT('Ctrl Pts',(38.9433207158183,86.6259444580485,122.));
#48881=CARTESIAN_POINT('Ctrl Pts',(38.9340003533245,86.5984520424969,122.));
#48882=CARTESIAN_POINT('Ctrl Pts',(38.9242292476095,86.571079706562,122.));
#48883=CARTESIAN_POINT('Ctrl Pts',(38.9140143220638,86.543835078612,122.));
#48884=CARTESIAN_POINT('Ctrl Pts',(38.9088566065269,86.5300787335221,122.));
#48885=CARTESIAN_POINT('Ctrl Pts',(38.9035888157279,86.5163632215208,122.));
#48886=CARTESIAN_POINT('Ctrl Pts',(38.8982136191598,86.502692859895,122.));
#48887=CARTESIAN_POINT('Ctrl Pts',(38.863962295366,86.4155838627646,122.));
#48888=CARTESIAN_POINT('Ctrl Pts',(38.8253374735071,86.3302636867753,122.));
#48889=CARTESIAN_POINT('Ctrl Pts',(38.7826691385711,86.2469667458681,122.));
#48890=CARTESIAN_POINT('Ctrl Pts',(38.7384393433969,86.1606215289644,122.));
#48891=CARTESIAN_POINT('Ctrl Pts',(38.6898645431327,86.0764496078788,122.));
#48892=CARTESIAN_POINT('Ctrl Pts',(38.6372564475687,85.994715560652,122.));
#48893=CARTESIAN_POINT('Ctrl Pts',(38.5840854062126,85.9121068982645,122.));
#48894=CARTESIAN_POINT('Ctrl Pts',(38.5267938741405,85.8319877413674,122.));
#48895=CARTESIAN_POINT('Ctrl Pts',(38.465652167204,85.7546466173903,122.));
#48896=CARTESIAN_POINT('Ctrl Pts',(38.4429632638252,85.7259463180847,122.));
#48897=CARTESIAN_POINT('Ctrl Pts',(38.4197436959574,85.6976287837773,122.));
#48898=CARTESIAN_POINT('Ctrl Pts',(38.3960056824848,85.6697096466582,122.));
#48899=CARTESIAN_POINT('Ctrl Pts',(38.3752500837481,85.6452982354931,122.));
#48900=CARTESIAN_POINT('Ctrl Pts',(38.3540981153553,85.621191407387,122.));
#48901=CARTESIAN_POINT('Ctrl Pts',(38.3325574553569,85.5973999946169,122.));
#48902=CARTESIAN_POINT('Ctrl Pts',(38.3207944345455,85.5844078725757,122.));
#48903=CARTESIAN_POINT('Ctrl Pts',(38.3089201790621,85.5715150612789,122.));
#48904=CARTESIAN_POINT('Ctrl Pts',(38.2969420121577,85.5587291809691,122.));
#48905=CARTESIAN_POINT('Ctrl Pts',(38.227931255996,85.4850648819642,122.));
#48906=CARTESIAN_POINT('Ctrl Pts',(38.1554181021943,85.4148851154279,122.));
#48907=CARTESIAN_POINT('Ctrl Pts',(38.0797110708892,85.3484810946605,122.));
#48908=CARTESIAN_POINT('Ctrl Pts',(38.0175169755689,85.2939295170056,122.));
#48909=CARTESIAN_POINT('Ctrl Pts',(37.9531663080692,85.2419261717527,122.));
#48910=CARTESIAN_POINT('Ctrl Pts',(37.8868078351083,85.192645848132,122.));
#48911=CARTESIAN_POINT('Ctrl Pts',(37.8621902138447,85.1743638671202,122.));
#48912=CARTESIAN_POINT('Ctrl Pts',(37.8372960861632,85.1564567893229,122.));
#48913=CARTESIAN_POINT('Ctrl Pts',(37.8121324405853,85.138934103667,122.));
#48914=CARTESIAN_POINT('Ctrl Pts',(37.7953216774585,85.1272279414182,122.));
#48915=CARTESIAN_POINT('Ctrl Pts',(37.7783894916928,85.1156927037062,122.));
#48916=CARTESIAN_POINT('Ctrl Pts',(37.7613530274051,85.1043410428558,122.));
#48917=CARTESIAN_POINT('Ctrl Pts',(37.6764425826325,85.0477638942505,122.));
#48918=CARTESIAN_POINT('Ctrl Pts',(37.5888628573917,84.9956860424815,122.));
#48919=CARTESIAN_POINT('Ctrl Pts',(37.4989042083555,84.9484154024461,122.));
#48920=CARTESIAN_POINT('Ctrl Pts',(37.4154461766131,84.9045606467465,122.));
#48921=CARTESIAN_POINT('Ctrl Pts',(37.3299397994821,84.864843173691,122.));
#48922=CARTESIAN_POINT('Ctrl Pts',(37.2425892169811,84.8295379073505,122.));
#48923=CARTESIAN_POINT('Ctrl Pts',(37.2121590462802,84.8172386730395,122.));
#48924=CARTESIAN_POINT('Ctrl Pts',(37.1815048545845,84.805475196943,122.));
#48925=CARTESIAN_POINT('Ctrl Pts',(37.1506395481981,84.7942437566138,122.));
#48926=CARTESIAN_POINT('Ctrl Pts',(33.836758858704,87.7663573595953,120.387416697508));
#48927=CARTESIAN_POINT('Ctrl Pts',(33.8351764988534,87.5919909257225,120.398449387697));
#48928=CARTESIAN_POINT('Ctrl Pts',(33.8517620939745,87.4179235371324,120.409482077886));
#48929=CARTESIAN_POINT('Ctrl Pts',(33.8876336552307,87.2479258898714,120.420514768075));
#48930=CARTESIAN_POINT('Ctrl Pts',(34.0588176556247,86.4366738479587,120.473164275806));
#48931=CARTESIAN_POINT('Ctrl Pts',(34.6692065633861,85.7181032071684,120.525813783537));
#48932=CARTESIAN_POINT('Ctrl Pts',(35.4420915227883,85.4179579283101,120.578463291268));
#48933=CARTESIAN_POINT('Ctrl Pts',(36.2149764821905,85.1178126494518,120.631112798999));
#48934=CARTESIAN_POINT('Ctrl Pts',(37.1503574932336,85.2360927325255,120.683762306729));
#48935=CARTESIAN_POINT('Ctrl Pts',(37.8241903566274,85.7191964419531,120.73641181446));
#48936=CARTESIAN_POINT('Ctrl Pts',(38.4980232200213,86.2023001513807,120.789061322191));
#48937=CARTESIAN_POINT('Ctrl Pts',(38.910307935766,87.050227487162,120.841710829922));
#48938=CARTESIAN_POINT('Ctrl Pts',(38.8741485771328,87.8785449389051,120.894360337653));
#48939=CARTESIAN_POINT('Ctrl Pts',(38.8379892184997,88.7068623906482,120.947009845384));
#48940=CARTESIAN_POINT('Ctrl Pts',(38.3533857854887,89.5155699583531,120.999659353114));
#48941=CARTESIAN_POINT('Ctrl Pts',(37.6400113138389,89.9381316467014,121.052308860845));
#48942=CARTESIAN_POINT('Ctrl Pts',(36.9266368421891,90.3606933350496,121.104958368576));
#48943=CARTESIAN_POINT('Ctrl Pts',(35.9844913319006,90.3971091440414,121.157607876307));
#48944=CARTESIAN_POINT('Ctrl Pts',(35.2407120680214,90.0307074467537,121.210257384038));
#48945=CARTESIAN_POINT('Ctrl Pts',(34.4969328041422,89.6643057494661,121.262906891768));
#48946=CARTESIAN_POINT('Ctrl Pts',(33.9515197866723,88.895086545899,121.315556399499));
#48947=CARTESIAN_POINT('Ctrl Pts',(33.851666089534,88.0720990746519,121.36820590723));
#48948=CARTESIAN_POINT('Ctrl Pts',(33.8395211932385,87.9720016543538,121.374609503989));
#48949=CARTESIAN_POINT('Ctrl Pts',(33.8339675024891,87.8711088344579,121.381013100749));
#48950=CARTESIAN_POINT('Ctrl Pts',(33.8347232656258,87.7701345030551,121.387416697508));
#48951=CARTESIAN_POINT('Ctrl Pts',(35.5611267921505,84.7993326348266,122.));
#48952=CARTESIAN_POINT('Ctrl Pts',(34.5788882023788,85.0619266872043,121.947350492269));
#48953=CARTESIAN_POINT('Ctrl Pts',(32.9121325517709,86.6347716463917,121.842051476808));
#48954=CARTESIAN_POINT('Ctrl Pts',(33.5229011708227,90.0369611826565,121.684102953615));
#48955=CARTESIAN_POINT('Ctrl Pts',(36.7064604291151,91.377416630034,121.526154430423));
#48956=CARTESIAN_POINT('Ctrl Pts',(39.5688530544509,89.4482951162593,121.36820590723));
#48957=CARTESIAN_POINT('Ctrl Pts',(39.5184627418672,85.9950129791182,121.210257384038));
#48958=CARTESIAN_POINT('Ctrl Pts',(36.5992128862014,84.1503276493198,121.052308860845));
#48959=CARTESIAN_POINT('Ctrl Pts',(33.4587562194708,85.585897700957,120.894360337653));
#48960=CARTESIAN_POINT('Ctrl Pts',(32.9440322230719,89.0005543330621,120.73641181446));
#48961=CARTESIAN_POINT('Ctrl Pts',(35.5219282988626,91.2981285259009,120.578463291268));
#48962=CARTESIAN_POINT('Ctrl Pts',(38.8550458568218,90.3955786925481,120.420514768075));
#48963=CARTESIAN_POINT('Ctrl Pts',(39.9213965365604,87.1111711483864,120.262566244883));
#48964=CARTESIAN_POINT('Ctrl Pts',(37.7541292878677,84.4228017462871,120.10461772169));
#48965=CARTESIAN_POINT('Ctrl Pts',(34.3182507508869,84.7679218698591,119.946669198498));
#48966=CARTESIAN_POINT('Ctrl Pts',(32.7289619830976,87.8336271382101,119.788720675305));
#48967=CARTESIAN_POINT('Ctrl Pts',(34.4272254557842,90.8403331303497,119.630772152113));
#48968=CARTESIAN_POINT('Ctrl Pts',(37.873276024629,91.0619522777656,119.47282362892));
#48969=CARTESIAN_POINT('Ctrl Pts',(39.9426850798466,88.2975486028455,119.314875105728));
#48970=CARTESIAN_POINT('Ctrl Pts',(38.7591820609565,85.0535231518079,119.156926582535));
#48971=CARTESIAN_POINT('Ctrl Pts',(35.3958133105107,84.2711349879319,118.998978059343));
#48972=CARTESIAN_POINT('Ctrl Pts',(32.9020429093888,86.6597517373779,118.841029536151));
#48973=CARTESIAN_POINT('Ctrl Pts',(33.5388966711455,90.0536872043056,118.683081012958));
#48974=CARTESIAN_POINT('Ctrl Pts',(36.7289586417865,91.3757633400502,118.525132489766));
#48975=CARTESIAN_POINT('Ctrl Pts',(39.5798966622645,89.4272939130391,118.367183966573));
#48976=CARTESIAN_POINT('Ctrl Pts',(39.5068519326957,85.9748968968193,118.209235443381));
#48977=CARTESIAN_POINT('Ctrl Pts',(36.5760518898075,84.1487556640973,118.051286920188));
#48978=CARTESIAN_POINT('Ctrl Pts',(33.4447637952687,85.6045769319753,117.893338396996));
#48979=CARTESIAN_POINT('Ctrl Pts',(32.9520313310439,89.0224118332001,117.735389873803));
#48980=CARTESIAN_POINT('Ctrl Pts',(35.5446000364372,91.3034134118094,117.577441350611));
#48981=CARTESIAN_POINT('Ctrl Pts',(38.8718667157924,90.3794669098942,117.419492827418));
#48982=CARTESIAN_POINT('Ctrl Pts',(39.9170998651258,87.0882865202323,117.261544304226));
#48983=CARTESIAN_POINT('Ctrl Pts',(37.7326183772922,84.4138854053773,117.103595781033));
#48984=CARTESIAN_POINT('Ctrl Pts',(34.2990251792965,84.7810617179477,116.945647257841));
#48985=CARTESIAN_POINT('Ctrl Pts',(32.729454795751,87.8569078624924,116.787698734649));
#48986=CARTESIAN_POINT('Ctrl Pts',(34.446988957088,90.8526476873878,116.629750211456));
#48987=CARTESIAN_POINT('Ctrl Pts',(37.894391675665,91.0521350047077,116.471801688264));
#48988=CARTESIAN_POINT('Ctrl Pts',(39.9460077545616,88.2745007309714,116.313853165071));
#48989=CARTESIAN_POINT('Ctrl Pts',(38.7416992921252,85.0381413842478,116.155904641879));
#48990=CARTESIAN_POINT('Ctrl Pts',(35.3733761438603,84.2773655547908,115.997956118686));
#48991=CARTESIAN_POINT('Ctrl Pts',(32.8949944653812,86.6819455492183,115.840007595494));
#48992=CARTESIAN_POINT('Ctrl Pts',(33.5536275479934,90.0717218185778,115.682059072301));
#48993=CARTESIAN_POINT('Ctrl Pts',(36.752112807112,91.3732873148253,115.524110549109));
#48994=CARTESIAN_POINT('Ctrl Pts',(39.5904809358262,89.4065521878392,115.366162025916));
#48995=CARTESIAN_POINT('Ctrl Pts',(39.4952698768951,85.954695361712,115.208213502724));
#48996=CARTESIAN_POINT('Ctrl Pts',(36.5528046017381,84.1474104372141,115.050264979531));
#48997=CARTESIAN_POINT('Ctrl Pts',(33.4309288843041,85.6233076893012,114.892316456339));
#48998=CARTESIAN_POINT('Ctrl Pts',(32.9601524900325,89.0442359668917,114.734367933146));
#48999=CARTESIAN_POINT('Ctrl Pts',(35.5673140575926,91.308543643525,114.576419409954));
#49000=CARTESIAN_POINT('Ctrl Pts',(38.8885794869123,90.3632518146024,114.418470886761));
#49001=CARTESIAN_POINT('Ctrl Pts',(39.9126584249495,87.0654278316568,114.260522363569));
#49002=CARTESIAN_POINT('Ctrl Pts',(37.7110496445387,84.4051084012425,114.102573840377));
#49003=CARTESIAN_POINT('Ctrl Pts',(34.2798848679742,84.7943242409579,113.944625317184));
#49004=CARTESIAN_POINT('Ctrl Pts',(32.7300968440076,87.8801851863978,113.786676793992));
#49005=CARTESIAN_POINT('Ctrl Pts',(34.4668312392973,90.8648349705502,113.628728270799));
#49006=CARTESIAN_POINT('Ctrl Pts',(37.915443798023,91.0421824081436,113.470779747607));
#49007=CARTESIAN_POINT('Ctrl Pts',(39.9491823979981,88.2514319712908,113.312831224414));
#49008=CARTESIAN_POINT('Ctrl Pts',(38.7241181039884,85.0228722042484,113.154882701222));
#49009=CARTESIAN_POINT('Ctrl Pts',(35.3509794527264,84.2837400555871,112.996934178029));
#49010=CARTESIAN_POINT('Ctrl Pts',(32.8880886699367,86.7041841648099,112.838985654837));
#49011=CARTESIAN_POINT('Ctrl Pts',(33.5684739229375,90.0896614725645,112.681037131644));
#49012=CARTESIAN_POINT('Ctrl Pts',(36.7752505958151,91.3706626685477,112.523088608452));
#49013=CARTESIAN_POINT('Ctrl Pts',(39.6009318089752,89.3857429282516,112.365140085259));
#49014=CARTESIAN_POINT('Ctrl Pts',(39.4835583456547,85.9345686115981,112.207191562067));
#49015=CARTESIAN_POINT('Ctrl Pts',(36.5295491552939,84.1462145087741,112.049243038874));
#49016=CARTESIAN_POINT('Ctrl Pts',(33.4172145286647,85.6421268944799,111.891294515682));
#49017=CARTESIAN_POINT('Ctrl Pts',(32.9684136143526,89.0660075047125,111.733345992489));
#49018=CARTESIAN_POINT('Ctrl Pts',(35.5900605517025,91.3135279228,111.575397469297));
#49019=CARTESIAN_POINT('Ctrl Pts',(38.9051877964048,90.346929740897,111.417448946105));
#49020=CARTESIAN_POINT('Ctrl Pts',(39.9080703007288,87.0425981327984,111.259500422912));
#49021=CARTESIAN_POINT('Ctrl Pts',(37.6894249992898,84.3964700708273,111.10155189972));
#49022=CARTESIAN_POINT('Ctrl Pts',(34.2608301098696,84.8077093905011,110.943603376527));
#49023=CARTESIAN_POINT('Ctrl Pts',(32.7308883426774,87.9034579077955,110.785654853335));
#49024=CARTESIAN_POINT('Ctrl Pts',(34.4867513670091,90.8768945953326,110.627706330142));
#49025=CARTESIAN_POINT('Ctrl Pts',(37.9364315807433,91.0320948408579,110.46975780695));
#49026=CARTESIAN_POINT('Ctrl Pts',(39.9522088516144,88.2283433032996,110.311809283757));
#49027=CARTESIAN_POINT('Ctrl Pts',(38.7064392347119,85.0077162267496,110.153860760565));
#49028=CARTESIAN_POINT('Ctrl Pts',(35.3286241543516,84.290258236255,109.995912237372));
#49029=CARTESIAN_POINT('Ctrl Pts',(32.8813258101548,86.7264666596099,109.83796371418));
#49030=CARTESIAN_POINT('Ctrl Pts',(33.5834351839898,90.1075054373259,109.680015190987));
#49031=CARTESIAN_POINT('Ctrl Pts',(36.7983710512446,91.3678894898621,109.522066667795));
#49032=CARTESIAN_POINT('Ctrl Pts',(39.6112488575384,89.3648670312859,109.364118144603));
#49033=CARTESIAN_POINT('Ctrl Pts',(39.4717178074565,85.914517396569,109.20616962141));
#49034=CARTESIAN_POINT('Ctrl Pts',(36.5062865391415,84.1451680917577,109.048221098218));
#49035=CARTESIAN_POINT('Ctrl Pts',(33.4036212322619,85.6610334351557,108.890272575025));
#49036=CARTESIAN_POINT('Ctrl Pts',(32.976814489993,89.0877262408462,108.732324051833));
#49037=CARTESIAN_POINT('Ctrl Pts',(35.6128383205754,91.3183646214857,108.57437552864));
#49038=CARTESIAN_POINT('Ctrl Pts',(38.9216914949492,90.3305042873106,108.416427005448));
#49039=CARTESIAN_POINT('Ctrl Pts',(39.9033345805337,87.019792348641,108.258478482255));
#49040=CARTESIAN_POINT('Ctrl Pts',(37.667747597468,84.3879831424088,108.100529959063));
#49041=CARTESIAN_POINT('Ctrl Pts',(34.2418570341057,84.8211911721592,107.94258143587));
#49042=CARTESIAN_POINT('Ctrl Pts',(32.7318388349523,87.9267773882983,107.784632912678));
#49043=CARTESIAN_POINT('Ctrl Pts',(34.5067288269183,90.8887184689395,107.626684389486));
#49044=CARTESIAN_POINT('Ctrl Pts',(37.957394655155,91.0220939825006,107.468735866293));
#49045=CARTESIAN_POINT('Ctrl Pts',(39.9550037460998,88.2047806129811,107.310787343101));
#49046=CARTESIAN_POINT('Ctrl Pts',(38.6888349059059,84.9936098257745,107.152838819908));
#49047=CARTESIAN_POINT('Ctrl Pts',(35.305967918485,84.2949816679675,106.994890296715));
#49048=CARTESIAN_POINT('Ctrl Pts',(32.8754909437191,86.7527679934688,106.836941773523));
#49049=CARTESIAN_POINT('Ctrl Pts',(33.3581428529919,88.9930721690106,106.731642758061));
#49050=CARTESIAN_POINT('Ctrl Pts',(34.018863416988,89.7658571455036,106.678993250331));
#49051=CARTESIAN_POINT('Ctrl Pts',(35.6089932203364,84.9783780187302,122.10700224989));
#49052=CARTESIAN_POINT('Ctrl Pts',(34.6859840276596,85.2251375401039,122.054352742159));
#49053=CARTESIAN_POINT('Ctrl Pts',(33.1197344387336,86.7031392915142,121.949053726697));
#49054=CARTESIAN_POINT('Ctrl Pts',(33.6936734550314,89.9001753781653,121.791105203505));
#49055=CARTESIAN_POINT('Ctrl Pts',(36.6852627607604,91.1598008023617,121.633156680312));
#49056=CARTESIAN_POINT('Ctrl Pts',(39.3750519156026,89.3470061213681,121.47520815712));
#49057=CARTESIAN_POINT('Ctrl Pts',(39.327700159908,86.1019583390072,121.317259633928));
#49058=CARTESIAN_POINT('Ctrl Pts',(36.5844822894654,84.36850830484,121.159311110735));
#49059=CARTESIAN_POINT('Ctrl Pts',(33.6333964710297,85.7175128829444,121.001362587543));
#49060=CARTESIAN_POINT('Ctrl Pts',(33.1497105465355,88.926264294351,120.84341406435));
#49061=CARTESIAN_POINT('Ctrl Pts',(35.5721584125611,91.0852938040143,120.685465541158));
#49062=CARTESIAN_POINT('Ctrl Pts',(38.7042875900392,90.2371681024705,120.527517017965));
#49063=CARTESIAN_POINT('Ctrl Pts',(39.7063368785371,87.1508117046191,120.369568494773));
#49064=CARTESIAN_POINT('Ctrl Pts',(37.6697567498784,84.6245520999892,120.21161997158));
#49065=CARTESIAN_POINT('Ctrl Pts',(34.4410631233212,84.9488613360056,120.053671448388));
#49066=CARTESIAN_POINT('Ctrl Pts',(32.9476091318338,87.8297032965965,119.895722925195));
#49067=CARTESIAN_POINT('Ctrl Pts',(34.5434666080111,90.6551036619663,119.737774402003));
#49068=CARTESIAN_POINT('Ctrl Pts',(37.7817188886635,90.8633590822565,119.57982587881));
#49069=CARTESIAN_POINT('Ctrl Pts',(39.7263417137742,88.2656501032049,119.421877355618));
#49070=CARTESIAN_POINT('Ctrl Pts',(38.6142044210923,85.2172407414007,119.263928832425));
#49071=CARTESIAN_POINT('Ctrl Pts',(35.4536482106658,84.4820309104909,119.105980309233));
#49072=CARTESIAN_POINT('Ctrl Pts',(33.110253206,86.7266130725836,118.948031786041));
#49073=CARTESIAN_POINT('Ctrl Pts',(33.7087044200059,89.9158928137251,118.790083262848));
#49074=CARTESIAN_POINT('Ctrl Pts',(36.7064043218137,91.1582472064541,118.632134739656));
#49075=CARTESIAN_POINT('Ctrl Pts',(39.3854295892538,89.3272712994712,118.474186216463));
#49076=CARTESIAN_POINT('Ctrl Pts',(39.3167894873777,86.0830552648703,118.316237693271));
#49077=CARTESIAN_POINT('Ctrl Pts',(36.5627179108249,84.3670311109829,118.158289170078));
#49078=CARTESIAN_POINT('Ctrl Pts',(33.6202477958494,85.7350657485328,118.000340646886));
#49079=CARTESIAN_POINT('Ctrl Pts',(33.1572273049567,88.946803778104,117.842392123693));
#49080=CARTESIAN_POINT('Ctrl Pts',(35.5934630348934,91.0902600090959,117.684443600501));
#49081=CARTESIAN_POINT('Ctrl Pts',(38.7200941441904,90.222027867038,117.526495077308));
#49082=CARTESIAN_POINT('Ctrl Pts',(39.7022992981841,87.1293070290982,117.368546554116));
#49083=CARTESIAN_POINT('Ctrl Pts',(37.6495429561925,84.6161734181593,117.210598030923));
#49084=CARTESIAN_POINT('Ctrl Pts',(34.4229968617254,84.9612088457679,117.052649507731));
#49085=CARTESIAN_POINT('Ctrl Pts',(32.9480722276783,87.8515801834838,116.894700984538));
#49086=CARTESIAN_POINT('Ctrl Pts',(34.562038361934,90.6666756460731,116.736752461346));
#49087=CARTESIAN_POINT('Ctrl Pts',(37.8015612571253,90.8541337948632,116.578803938153));
#49088=CARTESIAN_POINT('Ctrl Pts',(39.7294640298165,88.2439920276285,116.420855414961));
#49089=CARTESIAN_POINT('Ctrl Pts',(38.5977758705214,85.2027865008471,116.262906891769));
#49090=CARTESIAN_POINT('Ctrl Pts',(35.432564014533,84.4878857715667,116.104958368576));
#49091=CARTESIAN_POINT('Ctrl Pts',(33.1036297861092,86.7474685883031,115.947009845383));
#49092=CARTESIAN_POINT('Ctrl Pts',(33.722547018829,89.9328399332263,115.789061322191));
#49093=CARTESIAN_POINT('Ctrl Pts',(36.7281622813021,91.1559204865843,115.631112798999));
#49094=CARTESIAN_POINT('Ctrl Pts',(39.3953756267003,89.3077803089614,115.473164275806));
#49095=CARTESIAN_POINT('Ctrl Pts',(39.3059058343779,86.0640718907652,115.315215752614));
#49096=CARTESIAN_POINT('Ctrl Pts',(36.540872443933,84.3657670018423,115.157267229421));
#49097=CARTESIAN_POINT('Ctrl Pts',(33.6072471357927,85.7526670333709,114.999318706229));
#49098=CARTESIAN_POINT('Ctrl Pts',(33.1648587546674,88.9673119074215,114.841370183036));
#49099=CARTESIAN_POINT('Ctrl Pts',(35.6148073910889,91.0950808856969,114.683421659844));
#49100=CARTESIAN_POINT('Ctrl Pts',(38.7357991282334,90.2067905487629,114.525473136651));
#49101=CARTESIAN_POINT('Ctrl Pts',(39.6981256787049,87.1078267289883,114.367524613459));
#49102=CARTESIAN_POINT('Ctrl Pts',(37.6292748270299,84.6079256710386,114.209576090266));
#49103=CARTESIAN_POINT('Ctrl Pts',(34.4050107191677,84.9736716331029,114.051627567074));
#49104=CARTESIAN_POINT('Ctrl Pts',(32.948675560157,87.8734538750383,113.893679043881));
#49105=CARTESIAN_POINT('Ctrl Pts',(34.580684146241,90.6781280309721,113.735730520689));
#49106=CARTESIAN_POINT('Ctrl Pts',(37.8213439277149,90.8447813440276,113.577781997497));
#49107=CARTESIAN_POINT('Ctrl Pts',(39.7324472409282,88.2223143237889,113.419833474304));
#49108=CARTESIAN_POINT('Ctrl Pts',(38.5812548353702,85.1884380587774,113.261884951112));
#49109=CARTESIAN_POINT('Ctrl Pts',(35.4115178532262,84.4938758873033,113.103936427919));
#49110=CARTESIAN_POINT('Ctrl Pts',(33.0971404130134,86.7683662060889,112.945987904727));
#49111=CARTESIAN_POINT('Ctrl Pts',(33.7364981511649,89.949697818587,112.788039381534));
#49112=CARTESIAN_POINT('Ctrl Pts',(36.7499048516853,91.1534541075731,112.630090858342));
#49113=CARTESIAN_POINT('Ctrl Pts',(39.4051963078346,89.2882258564159,112.472142335149));
#49114=CARTESIAN_POINT('Ctrl Pts',(39.2949005133615,86.0451587920869,112.314193811957));
#49115=CARTESIAN_POINT('Ctrl Pts',(36.5190193106196,84.3646431883867,112.156245288764));
#49116=CARTESIAN_POINT('Ctrl Pts',(33.5943597615248,85.7703514326194,111.998296765572));
#49117=CARTESIAN_POINT('Ctrl Pts',(33.1726217297416,88.987770612421,111.840348242379));
#49118=CARTESIAN_POINT('Ctrl Pts',(35.6361822621062,91.0997646108504,111.682399719187));
#49119=CARTESIAN_POINT('Ctrl Pts',(38.7514059497287,90.1914527029174,111.524451195994));
#49120=CARTESIAN_POINT('Ctrl Pts',(39.6938142202905,87.0863736705035,111.366502672802));
#49121=CARTESIAN_POINT('Ctrl Pts',(37.6089541569189,84.5998082355544,111.20855414961));
#49122=CARTESIAN_POINT('Ctrl Pts',(34.3871049709332,84.9862496525397,111.050605626417));
#49123=CARTESIAN_POINT('Ctrl Pts',(32.9494193311266,87.8953232416183,110.892657103225));
#49124=CARTESIAN_POINT('Ctrl Pts',(34.5994030819342,90.6894604553447,110.734708580032));
#49125=CARTESIAN_POINT('Ctrl Pts',(37.8410661383737,90.8353020612612,110.57676005684));
#49126=CARTESIAN_POINT('Ctrl Pts',(39.7352911981278,88.2006179121182,110.418811533647));
#49127=CARTESIAN_POINT('Ctrl Pts',(38.5646420092929,85.17419599305,110.260863010455));
#49128=CARTESIAN_POINT('Ctrl Pts',(35.3905105886778,84.5000010189553,110.102914487262));
#49129=CARTESIAN_POINT('Ctrl Pts',(33.0907853565002,86.7893050571483,109.94496596407));
#49130=CARTESIAN_POINT('Ctrl Pts',(33.7505572419288,89.9664657848225,109.787017440877));
#49131=CARTESIAN_POINT('Ctrl Pts',(36.7716311339984,91.1508481527202,109.629068917685));
#49132=CARTESIAN_POINT('Ctrl Pts',(39.4148912340616,89.2686087847539,109.471120394492));
#49133=CARTESIAN_POINT('Ctrl Pts',(39.2837739645606,86.0263166736965,109.3131718713));
#49134=CARTESIAN_POINT('Ctrl Pts',(36.4971594399344,84.3636598707533,109.155223348107));
#49135=CARTESIAN_POINT('Ctrl Pts',(33.5815861465709,85.7881179009981,108.997274824915));
#49136=CARTESIAN_POINT('Ctrl Pts',(33.1805160290731,89.0081796996972,108.839326301723));
#49137=CARTESIAN_POINT('Ctrl Pts',(35.6575865220053,91.1043096545859,108.68137777853));
#49138=CARTESIAN_POINT('Ctrl Pts',(38.7669144683598,90.1760177110405,108.523429255338));
#49139=CARTESIAN_POINT('Ctrl Pts',(39.6893640660006,87.0649430846534,108.365480732145));
#49140=CARTESIAN_POINT('Ctrl Pts',(37.5885839114783,84.5918330724633,108.207532208953));
#49141=CARTESIAN_POINT('Ctrl Pts',(34.36927597956,84.9989184771347,108.04958368576));
#49142=CARTESIAN_POINT('Ctrl Pts',(32.9503125083204,87.9172365477096,107.891635162568));
#49143=CARTESIAN_POINT('Ctrl Pts',(34.6181758926694,90.7005713444361,107.733686639375));
#49144=CARTESIAN_POINT('Ctrl Pts',(37.8607651306453,90.8259042588387,107.575738116183));
#49145=CARTESIAN_POINT('Ctrl Pts',(39.7379175593087,88.1784760618644,107.41778959299));
#49146=CARTESIAN_POINT('Ctrl Pts',(38.5480992288646,85.1609402139439,107.259841069798));
#49147=CARTESIAN_POINT('Ctrl Pts',(35.369220533294,84.5044396257634,107.101892546605));
#49148=CARTESIAN_POINT('Ctrl Pts',(33.0853023349469,86.8140204095934,106.943944023413));
#49149=CARTESIAN_POINT('Ctrl Pts',(33.5388501325603,88.9192333079159,106.838645007951));
#49150=CARTESIAN_POINT('Ctrl Pts',(34.159728970665,89.6454190276517,106.78599550022));
#49151=CARTESIAN_POINT('Ctrl Pts',(35.6568596485223,85.1574234026337,122.21400449978));
#49152=CARTESIAN_POINT('Ctrl Pts',(34.7930798529404,85.3883483930035,122.161354992049));
#49153=CARTESIAN_POINT('Ctrl Pts',(33.3273363256962,86.7715069366368,122.056055976587));
#49154=CARTESIAN_POINT('Ctrl Pts',(33.8644457392402,89.7633895736742,121.898107453395));
#49155=CARTESIAN_POINT('Ctrl Pts',(36.6640650924058,90.9421849746893,121.740158930202));
#49156=CARTESIAN_POINT('Ctrl Pts',(39.1812507767543,89.245717126477,121.58221040701));
#49157=CARTESIAN_POINT('Ctrl Pts',(39.1369375779489,86.2089036988962,121.424261883817));
#49158=CARTESIAN_POINT('Ctrl Pts',(36.5697516927295,84.5866889603602,121.266313360625));
#49159=CARTESIAN_POINT('Ctrl Pts',(33.8080367225885,85.8491280649318,121.108364837432));
#49160=CARTESIAN_POINT('Ctrl Pts',(33.3553888699991,88.8519742556397,120.95041631424));
#49161=CARTESIAN_POINT('Ctrl Pts',(35.6223885262595,90.8724590821279,120.792467791047));
#49162=CARTESIAN_POINT('Ctrl Pts',(38.5535293232566,90.0787575123929,120.634519267855));
#49163=CARTESIAN_POINT('Ctrl Pts',(39.4912772205139,87.1904522608518,120.476570744663));
#49164=CARTESIAN_POINT('Ctrl Pts',(37.5853842118891,84.8263024536913,120.31862222147));
#49165=CARTESIAN_POINT('Ctrl Pts',(34.5638754957556,85.1298008021523,120.160673698278));
#49166=CARTESIAN_POINT('Ctrl Pts',(33.1662562805699,87.8257794549828,120.002725175085));
#49167=CARTESIAN_POINT('Ctrl Pts',(34.659707760238,90.4698741935831,119.844776651893));
#49168=CARTESIAN_POINT('Ctrl Pts',(37.690161752698,90.6647658867473,119.6868281287));
#49169=CARTESIAN_POINT('Ctrl Pts',(39.5099983477018,88.2337516035643,119.528879605508));
#49170=CARTESIAN_POINT('Ctrl Pts',(38.4692267812281,85.3809583309936,119.370931082315));
#49171=CARTESIAN_POINT('Ctrl Pts',(35.5114831108209,84.69292683305,119.212982559123));
#49172=CARTESIAN_POINT('Ctrl Pts',(33.3184635026112,86.7934744077893,119.05503403593));
#49173=CARTESIAN_POINT('Ctrl Pts',(33.8785121688663,89.7780984231445,118.897085512738));
#49174=CARTESIAN_POINT('Ctrl Pts',(36.6838500018409,90.9407310728582,118.739136989545));
#49175=CARTESIAN_POINT('Ctrl Pts',(39.1909625162432,89.2272486859031,118.581188466353));
#49176=CARTESIAN_POINT('Ctrl Pts',(39.1267270420596,86.1912136329214,118.42323994316));
#49177=CARTESIAN_POINT('Ctrl Pts',(36.5493839318423,84.5853065578684,118.265291419968));
#49178=CARTESIAN_POINT('Ctrl Pts',(33.7957317964302,85.8655545650902,118.107342896775));
#49179=CARTESIAN_POINT('Ctrl Pts',(33.3624232788696,88.871195723008,117.949394373583));
#49180=CARTESIAN_POINT('Ctrl Pts',(35.6423260333496,90.8771066063823,117.79144585039));
#49181=CARTESIAN_POINT('Ctrl Pts',(38.5683215725883,90.0645888241819,117.633497327198));
#49182=CARTESIAN_POINT('Ctrl Pts',(39.4874987312424,87.1703275379639,117.475548804005));
#49183=CARTESIAN_POINT('Ctrl Pts',(37.5664675350927,84.8184614309413,117.317600280813));
#49184=CARTESIAN_POINT('Ctrl Pts',(34.5469685441542,85.1413559735884,117.159651757621));
#49185=CARTESIAN_POINT('Ctrl Pts',(33.1666896596057,87.846252504475,117.001703234428));
#49186=CARTESIAN_POINT('Ctrl Pts',(34.6770877667801,90.4807036047585,116.843754711236));
#49187=CARTESIAN_POINT('Ctrl Pts',(37.7087308385855,90.6561325850187,116.685806188043));
#49188=CARTESIAN_POINT('Ctrl Pts',(39.5129203050714,88.2134833242854,116.527857664851));
#49189=CARTESIAN_POINT('Ctrl Pts',(38.4538524489176,85.3674316174465,116.369909141658));
#49190=CARTESIAN_POINT('Ctrl Pts',(35.4917518852057,84.6984059883427,116.211960618466));
#49191=CARTESIAN_POINT('Ctrl Pts',(33.3122651068371,86.8129916273879,116.054012095273));
#49192=CARTESIAN_POINT('Ctrl Pts',(33.8914664896646,89.7939580478747,115.896063572081));
#49193=CARTESIAN_POINT('Ctrl Pts',(36.7042117554922,90.9385536583433,115.738115048888));
#49194=CARTESIAN_POINT('Ctrl Pts',(39.2002703175744,89.2090084300835,115.580166525696));
#49195=CARTESIAN_POINT('Ctrl Pts',(39.1165417918607,86.1734484198183,115.422218002503));
#49196=CARTESIAN_POINT('Ctrl Pts',(36.5289402861278,84.5841235664707,115.264269479311));
#49197=CARTESIAN_POINT('Ctrl Pts',(33.7835653872813,85.8820263774406,115.106320956119));
#49198=CARTESIAN_POINT('Ctrl Pts',(33.3695650193023,88.8903878479511,114.948372432926));
#49199=CARTESIAN_POINT('Ctrl Pts',(35.6623007245852,90.8816181278689,114.790423909734));
#49200=CARTESIAN_POINT('Ctrl Pts',(38.5830187695545,90.0503292829234,114.632475386541));
#49201=CARTESIAN_POINT('Ctrl Pts',(39.4835929324604,87.1502256263198,114.474526863349));
#49202=CARTESIAN_POINT('Ctrl Pts',(37.5475000095212,84.8107429408348,114.316578340156));
#49203=CARTESIAN_POINT('Ctrl Pts',(34.5301365703613,85.153019025248,114.158629816964));
#49204=CARTESIAN_POINT('Ctrl Pts',(33.1672542763064,87.8667225636788,114.000681293771));
#49205=CARTESIAN_POINT('Ctrl Pts',(34.6945370531848,90.491421091394,113.842732770579));
#49206=CARTESIAN_POINT('Ctrl Pts',(37.7272440574067,90.6473802799116,113.684784247386));
#49207=CARTESIAN_POINT('Ctrl Pts',(39.5157120838583,88.1931966762869,113.526835724194));
#49208=CARTESIAN_POINT('Ctrl Pts',(38.4383915667521,85.3540039133063,113.368887201001));
#49209=CARTESIAN_POINT('Ctrl Pts',(35.472056253726,84.7040117190196,113.210938677809));
#49210=CARTESIAN_POINT('Ctrl Pts',(33.3061921560902,86.8325482473677,113.052990154616));
#49211=CARTESIAN_POINT('Ctrl Pts',(33.9045223793923,89.8097341646095,112.895041631424));
#49212=CARTESIAN_POINT('Ctrl Pts',(36.7245591075554,90.9362455465985,112.737093108232));
#49213=CARTESIAN_POINT('Ctrl Pts',(39.2094608066942,89.1907087845802,112.579144585039));
#49214=CARTESIAN_POINT('Ctrl Pts',(39.1062426810682,86.1557489725758,112.421196061847));
#49215=CARTESIAN_POINT('Ctrl Pts',(36.5084894659453,84.5830718679992,112.263247538654));
#49216=CARTESIAN_POINT('Ctrl Pts',(33.7715049943849,85.898575970759,112.105299015462));
#49217=CARTESIAN_POINT('Ctrl Pts',(33.3768298451305,88.9095337201295,111.947350492269));
#49218=CARTESIAN_POINT('Ctrl Pts',(35.6823039725099,90.8860012989009,111.789401969077));
#49219=CARTESIAN_POINT('Ctrl Pts',(38.5976241030526,90.0359756649375,111.631453445884));
#49220=CARTESIAN_POINT('Ctrl Pts',(39.4795581398523,87.1301492082086,111.473504922692));
#49221=CARTESIAN_POINT('Ctrl Pts',(37.5284833145479,84.8031464002815,111.315556399499));
#49222=CARTESIAN_POINT('Ctrl Pts',(34.5133798319967,85.1647899145784,111.157607876307));
#49223=CARTESIAN_POINT('Ctrl Pts',(33.1679503195757,87.8871885754409,110.999659353114));
#49224=CARTESIAN_POINT('Ctrl Pts',(34.7120547968593,90.5020263153568,110.841710829922));
#49225=CARTESIAN_POINT('Ctrl Pts',(37.7457006960041,90.6385092816646,110.683762306729));
#49226=CARTESIAN_POINT('Ctrl Pts',(39.5183735446411,88.1728925209367,110.525813783537));
#49227=CARTESIAN_POINT('Ctrl Pts',(38.422844783874,85.3406757593505,110.367865260344));
#49228=CARTESIAN_POINT('Ctrl Pts',(35.4523970230039,84.7097438016556,110.209916737152));
#49229=CARTESIAN_POINT('Ctrl Pts',(33.3002449028457,86.8521434546867,110.05196821396));
#49230=CARTESIAN_POINT('Ctrl Pts',(33.9176792998676,89.8254261323192,109.894019690767));
#49231=CARTESIAN_POINT('Ctrl Pts',(36.7448912167523,90.9338068155782,109.736071167575));
#49232=CARTESIAN_POINT('Ctrl Pts',(39.2185336105849,89.1723505382218,109.578122644382));
#49233=CARTESIAN_POINT('Ctrl Pts',(39.0958301216647,86.1381159508238,109.42017412119));
#49234=CARTESIAN_POINT('Ctrl Pts',(36.4880323407273,84.5821516497489,109.262225597997));
#49235=CARTESIAN_POINT('Ctrl Pts',(33.75955106088,85.9152023668404,109.104277074805));
#49236=CARTESIAN_POINT('Ctrl Pts',(33.3842175681532,88.9286331585482,108.946328551612));
#49237=CARTESIAN_POINT('Ctrl Pts',(35.7023347234351,90.890254687686,108.78838002842));
#49238=CARTESIAN_POINT('Ctrl Pts',(38.6121374417704,90.0215311347704,108.630431505227));
#49239=CARTESIAN_POINT('Ctrl Pts',(39.4753935514674,87.1100938206657,108.472482982035));
#49240=CARTESIAN_POINT('Ctrl Pts',(37.5094202254886,84.7956830025177,108.314534458842));
#49241=CARTESIAN_POINT('Ctrl Pts',(34.4966949250142,85.17664578211,108.15658593565));
#49242=CARTESIAN_POINT('Ctrl Pts',(33.1687861816885,87.907695707121,107.998637412457));
#49243=CARTESIAN_POINT('Ctrl Pts',(34.7296229584204,90.5124242199326,107.840688889265));
#49244=CARTESIAN_POINT('Ctrl Pts',(37.7641356061356,90.6297145351769,107.682740366072));
#49245=CARTESIAN_POINT('Ctrl Pts',(39.5208313725176,88.1521715107477,107.52479184288));
#49246=CARTESIAN_POINT('Ctrl Pts',(38.4073635518233,85.3282706021133,107.366843319688));
#49247=CARTESIAN_POINT('Ctrl Pts',(35.432473148103,84.7138975835592,107.208894796495));
#49248=CARTESIAN_POINT('Ctrl Pts',(33.2951137261748,86.8752728257181,107.050946273303));
#49249=CARTESIAN_POINT('Ctrl Pts',(33.7195574121287,88.8453944468211,106.945647257841));
#49250=CARTESIAN_POINT('Ctrl Pts',(34.300594524342,89.5249809097997,106.89299775011));
#49251=CARTESIAN_POINT('Ctrl Pts',(35.7047260767083,85.3364687865372,122.321006749669));
#49252=CARTESIAN_POINT('Ctrl Pts',(34.9001756782212,85.5515592459031,122.268357241939));
#49253=CARTESIAN_POINT('Ctrl Pts',(33.534938212659,86.8398745817594,122.163058226477));
#49254=CARTESIAN_POINT('Ctrl Pts',(34.0352180234489,89.6266037691829,122.005109703284));
#49255=CARTESIAN_POINT('Ctrl Pts',(36.6428674240512,90.7245691470171,121.847161180092));
#49256=CARTESIAN_POINT('Ctrl Pts',(38.987449637906,89.1444281315857,121.6892126569));
#49257=CARTESIAN_POINT('Ctrl Pts',(38.9461749959898,86.3158490587852,121.531264133707));
#49258=CARTESIAN_POINT('Ctrl Pts',(36.5550210959935,84.8048696158805,121.373315610515));
#49259=CARTESIAN_POINT('Ctrl Pts',(33.9826769741474,85.9807432469191,121.215367087322));
#49260=CARTESIAN_POINT('Ctrl Pts',(33.5610671934627,88.7776842169286,121.05741856413));
#49261=CARTESIAN_POINT('Ctrl Pts',(35.672618639958,90.6596243602414,120.899470040937));
#49262=CARTESIAN_POINT('Ctrl Pts',(38.402771056474,89.9203469223153,120.741521517745));
#49263=CARTESIAN_POINT('Ctrl Pts',(39.2762175624906,87.2300928170844,120.583572994552));
#49264=CARTESIAN_POINT('Ctrl Pts',(37.5010116738998,85.0280528073935,120.42562447136));
#49265=CARTESIAN_POINT('Ctrl Pts',(34.6866878681899,85.3107402682988,120.267675948167));
#49266=CARTESIAN_POINT('Ctrl Pts',(33.3849034293061,87.8218556133692,120.109727424975));
#49267=CARTESIAN_POINT('Ctrl Pts',(34.7759489124649,90.2846447251997,119.951778901782));
#49268=CARTESIAN_POINT('Ctrl Pts',(37.5986046167326,90.4661726912383,119.79383037859));
#49269=CARTESIAN_POINT('Ctrl Pts',(39.2936549816293,88.2018531039237,119.635881855397));
#49270=CARTESIAN_POINT('Ctrl Pts',(38.3242491413639,85.5446759205865,119.477933332205));
#49271=CARTESIAN_POINT('Ctrl Pts',(35.569318010976,84.9038227556091,119.319984809012));
#49272=CARTESIAN_POINT('Ctrl Pts',(33.5266737992225,86.860335742995,119.16203628582));
#49273=CARTESIAN_POINT('Ctrl Pts',(34.0483199177267,89.640304032564,119.004087762628));
#49274=CARTESIAN_POINT('Ctrl Pts',(36.6612956818681,90.7232149392622,118.846139239435));
#49275=CARTESIAN_POINT('Ctrl Pts',(38.9964954432325,89.1272260723352,118.688190716243));
#49276=CARTESIAN_POINT('Ctrl Pts',(38.9366645967416,86.2993720009723,118.53024219305));
#49277=CARTESIAN_POINT('Ctrl Pts',(36.5360499528598,84.803582004754,118.372293669858));
#49278=CARTESIAN_POINT('Ctrl Pts',(33.9712157970109,85.9960433816476,118.214345146665));
#49279=CARTESIAN_POINT('Ctrl Pts',(33.5676192527825,88.795587667912,118.056396623473));
#49280=CARTESIAN_POINT('Ctrl Pts',(35.6911890318057,90.6639532036688,117.89844810028));
#49281=CARTESIAN_POINT('Ctrl Pts',(38.4165490009863,89.9071497813258,117.740499577088));
#49282=CARTESIAN_POINT('Ctrl Pts',(39.2726981643007,87.2113480468297,117.582551053895));
#49283=CARTESIAN_POINT('Ctrl Pts',(37.4833921139929,85.0207494437233,117.424602530703));
#49284=CARTESIAN_POINT('Ctrl Pts',(34.670940226583,85.3215031014086,117.266654007511));
#49285=CARTESIAN_POINT('Ctrl Pts',(33.3853070915332,87.8409248254664,117.108705484318));
#49286=CARTESIAN_POINT('Ctrl Pts',(34.7921371716262,90.2947315634439,116.950756961126));
#49287=CARTESIAN_POINT('Ctrl Pts',(37.6159004200458,90.4581313751741,116.792808437933));
#49288=CARTESIAN_POINT('Ctrl Pts',(39.2963765803263,88.1829746209424,116.634859914741));
#49289=CARTESIAN_POINT('Ctrl Pts',(38.3099290273138,85.5320767340458,116.476911391548));
#49290=CARTESIAN_POINT('Ctrl Pts',(35.5509397558784,84.9089262051186,116.318962868356));
#49291=CARTESIAN_POINT('Ctrl Pts',(33.5209004275651,86.8785146664726,116.161014345163));
#49292=CARTESIAN_POINT('Ctrl Pts',(34.0603859605002,89.6550761625235,116.003065821971));
#49293=CARTESIAN_POINT('Ctrl Pts',(36.6802612296823,90.7211868301021,115.845117298778));
#49294=CARTESIAN_POINT('Ctrl Pts',(39.0051650084485,89.1102365512059,115.687168775586));
#49295=CARTESIAN_POINT('Ctrl Pts',(38.9271777493435,86.2828249488715,115.529220252393));
#49296=CARTESIAN_POINT('Ctrl Pts',(36.5170081283227,84.8024801310989,115.371271729201));
#49297=CARTESIAN_POINT('Ctrl Pts',(33.95988363877,86.0113857215104,115.213323206008));
#49298=CARTESIAN_POINT('Ctrl Pts',(33.5742712839372,88.8134637884809,115.055374682816));
#49299=CARTESIAN_POINT('Ctrl Pts',(35.7097940580815,90.6681553700408,114.897426159623));
#49300=CARTESIAN_POINT('Ctrl Pts',(38.4302384108755,89.8938680170839,114.739477636431));
#49301=CARTESIAN_POINT('Ctrl Pts',(39.2690601862158,87.1926245236512,114.581529113238));
#49302=CARTESIAN_POINT('Ctrl Pts',(37.4657251920124,85.0135602106309,114.423580590046));
#49303=CARTESIAN_POINT('Ctrl Pts',(34.6552624215549,85.3323664173931,114.265632066854));
#49304=CARTESIAN_POINT('Ctrl Pts',(33.3858329924558,87.8599912523192,114.107683543661));
#49305=CARTESIAN_POINT('Ctrl Pts',(34.8083899601285,90.3047141518159,113.949735020469));
#49306=CARTESIAN_POINT('Ctrl Pts',(37.6331441870985,90.4499792157957,113.791786497276));
#49307=CARTESIAN_POINT('Ctrl Pts',(39.2989769267884,88.1640790287851,113.633837974084));
#49308=CARTESIAN_POINT('Ctrl Pts',(38.295528298134,85.5195697678351,113.475889450891));
#49309=CARTESIAN_POINT('Ctrl Pts',(35.5325946542257,84.9141475507359,113.317940927699));
#49310=CARTESIAN_POINT('Ctrl Pts',(33.5152438991669,86.8967302886466,113.159992404506));
#49311=CARTESIAN_POINT('Ctrl Pts',(34.0725466076197,89.669770510632,113.002043881314));
#49312=CARTESIAN_POINT('Ctrl Pts',(36.6992133634256,90.719036985624,112.844095358121));
#49313=CARTESIAN_POINT('Ctrl Pts',(39.0137253055536,89.0931917127443,112.686146834929));
#49314=CARTESIAN_POINT('Ctrl Pts',(38.917584848775,86.2663391530647,112.528198311737));
#49315=CARTESIAN_POINT('Ctrl Pts',(36.497959621271,84.8015005476119,112.370249788544));
#49316=CARTESIAN_POINT('Ctrl Pts',(33.9486502272449,86.0268005088984,112.212301265351));
#49317=CARTESIAN_POINT('Ctrl Pts',(33.5810379605196,88.831296827838,112.054352742159));
#49318=CARTESIAN_POINT('Ctrl Pts',(35.7284256829136,90.6722379869513,111.896404218967));
#49319=CARTESIAN_POINT('Ctrl Pts',(38.4438422563765,89.8804986269578,111.738455695774));
#49320=CARTESIAN_POINT('Ctrl Pts',(39.265302059414,87.1739247459138,111.580507172582));
#49321=CARTESIAN_POINT('Ctrl Pts',(37.448012472177,85.0064845650086,111.422558649389));
#49322=CARTESIAN_POINT('Ctrl Pts',(34.6396546930603,85.3433301766171,111.264610126197));
#49323=CARTESIAN_POINT('Ctrl Pts',(33.3864813080249,87.8790539092635,111.106661603004));
#49324=CARTESIAN_POINT('Ctrl Pts',(34.8247065117844,90.3145921753689,110.948713079812));
#49325=CARTESIAN_POINT('Ctrl Pts',(37.6503352536344,90.4417165020679,110.790764556619));
#49326=CARTESIAN_POINT('Ctrl Pts',(39.3014558911545,88.1451671297553,110.632816033427));
#49327=CARTESIAN_POINT('Ctrl Pts',(38.2810475584549,85.507155525651,110.474867510234));
#49328=CARTESIAN_POINT('Ctrl Pts',(35.5142834573301,84.919486584356,110.316918987042));
#49329=CARTESIAN_POINT('Ctrl Pts',(33.5097044491911,86.9149818522253,110.158970463849));
#49330=CARTESIAN_POINT('Ctrl Pts',(34.0848013578066,89.6843864798158,110.001021940657));
#49331=CARTESIAN_POINT('Ctrl Pts',(36.7181512995062,90.7167654784365,109.843073417464));
#49332=CARTESIAN_POINT('Ctrl Pts',(39.0221759871081,89.0760922916896,109.685124894272));
#49333=CARTESIAN_POINT('Ctrl Pts',(38.9078862787688,86.2499152279515,109.52717637108));
#49334=CARTESIAN_POINT('Ctrl Pts',(36.4789052415203,84.8006434287444,109.369227847887));
#49335=CARTESIAN_POINT('Ctrl Pts',(33.937515975189,86.0422868326829,109.211279324695));
#49336=CARTESIAN_POINT('Ctrl Pts',(33.5879191072333,88.8490866173992,109.053330801502));
#49337=CARTESIAN_POINT('Ctrl Pts',(35.747082924865,90.6761997207862,108.89538227831));
#49338=CARTESIAN_POINT('Ctrl Pts',(38.457360415181,89.8670445585003,108.737433755117));
#49339=CARTESIAN_POINT('Ctrl Pts',(39.2614230369343,87.155244556678,108.579485231925));
#49340=CARTESIAN_POINT('Ctrl Pts',(37.4302565394989,84.9995329325722,108.421536708732));
#49341=CARTESIAN_POINT('Ctrl Pts',(34.6241138704685,85.3543730870854,108.26358818554));
#49342=CARTESIAN_POINT('Ctrl Pts',(33.3872598550566,87.8981548665324,108.105639662347));
#49343=CARTESIAN_POINT('Ctrl Pts',(34.8410700241714,90.3242770954292,107.947691139155));
#49344=CARTESIAN_POINT('Ctrl Pts',(37.6675060816258,90.433524811515,107.789742615962));
#49345=CARTESIAN_POINT('Ctrl Pts',(39.3037451857265,88.125866959631,107.63179409277));
#49346=CARTESIAN_POINT('Ctrl Pts',(38.2666278747819,85.4956009902827,107.473845569577));
#49347=CARTESIAN_POINT('Ctrl Pts',(35.495725762912,84.9233555413549,107.315897046385));
#49348=CARTESIAN_POINT('Ctrl Pts',(33.5049251174026,86.9365252418428,107.157948523192));
#49349=CARTESIAN_POINT('Ctrl Pts',(33.9002646916971,88.7715555857264,107.052649507731));
#49350=CARTESIAN_POINT('Ctrl Pts',(34.441460078019,89.4045427919478,107.));
#49351=CARTESIAN_POINT('Ctrl Pts',(33.8399314485466,87.7703173734778,121.112583302492));
#49352=CARTESIAN_POINT('Ctrl Pts',(33.8380185825139,88.0618702121891,121.094195056371));
#49353=CARTESIAN_POINT('Ctrl Pts',(33.8848898739967,88.3528282009691,121.07580681025));
#49354=CARTESIAN_POINT('Ctrl Pts',(33.983260731326,88.6251840791458,121.05741856413));
#49355=CARTESIAN_POINT('Ctrl Pts',(34.2649176756278,89.4049975980328,121.004769056399));
#49356=CARTESIAN_POINT('Ctrl Pts',(34.9687681577929,90.0323109791371,120.952119548668));
#49357=CARTESIAN_POINT('Ctrl Pts',(35.7757188016281,90.2227547633682,120.899470040937));
#49358=CARTESIAN_POINT('Ctrl Pts',(36.5826694454633,90.4131985475994,120.846820533206));
#49359=CARTESIAN_POINT('Ctrl Pts',(37.4927202509686,90.1667727349573,120.794171025476));
#49360=CARTESIAN_POINT('Ctrl Pts',(38.0933200713907,89.5951841444312,120.741521517745));
#49361=CARTESIAN_POINT('Ctrl Pts',(38.6939198918129,89.023595553905,120.688872010014));
#49362=CARTESIAN_POINT('Ctrl Pts',(38.9850687271518,88.1268441854947,120.636222502283));
#49363=CARTESIAN_POINT('Ctrl Pts',(38.8347754967227,87.3114618330078,120.583572994552));
#49364=CARTESIAN_POINT('Ctrl Pts',(38.6844822662937,86.4960794805208,120.530923486821));
#49365=CARTESIAN_POINT('Ctrl Pts',(38.0927469700967,85.7620661439571,120.478273979091));
#49366=CARTESIAN_POINT('Ctrl Pts',(37.3278253543799,85.4421740524928,120.42562447136));
#49367=CARTESIAN_POINT('Ctrl Pts',(36.5629037386632,85.1222819610286,120.372974963629));
#49368=CARTESIAN_POINT('Ctrl Pts',(35.6247958034265,85.2165111146637,120.320325455898));
#49369=CARTESIAN_POINT('Ctrl Pts',(34.9387777626609,85.6821449156596,120.267675948167));
#49370=CARTESIAN_POINT('Ctrl Pts',(34.265163658693,86.1393595616258,120.215978399609));
#49371=CARTESIAN_POINT('Ctrl Pts',(33.8346057561187,86.9546694932317,120.16428085105));
#49372=CARTESIAN_POINT('Ctrl Pts',(33.833340462721,87.7688288397412,120.112583302492));
#49373=CARTESIAN_POINT('Ctrl Pts',(35.5611267921505,84.7993326348266,122.));
#49374=CARTESIAN_POINT('Ctrl Pts',(35.4680767340868,84.8333707617182,122.));
#49375=CARTESIAN_POINT('Ctrl Pts',(35.3770918409722,84.8721775875453,122.));
#49376=CARTESIAN_POINT('Ctrl Pts',(35.2883805979929,84.9154247896511,122.));
#49377=CARTESIAN_POINT('Ctrl Pts',(35.197702396015,84.9596308947154,122.));
#49378=CARTESIAN_POINT('Ctrl Pts',(35.109399119487,85.0084770849584,122.));
#49379=CARTESIAN_POINT('Ctrl Pts',(35.0237223483213,85.0616582525317,122.));
#49380=CARTESIAN_POINT('Ctrl Pts',(34.9412909170175,85.112824977209,122.));
#49381=CARTESIAN_POINT('Ctrl Pts',(34.8612904976022,85.168005366865,122.));
#49382=CARTESIAN_POINT('Ctrl Pts',(34.7839781170505,85.2269577350007,122.));
#49383=CARTESIAN_POINT('Ctrl Pts',(34.7163297840678,85.2785410571195,122.));
#49384=CARTESIAN_POINT('Ctrl Pts',(34.6507397710755,85.3330129976211,122.));
#49385=CARTESIAN_POINT('Ctrl Pts',(34.5874048868897,85.3902243446383,122.));
#49386=CARTESIAN_POINT('Ctrl Pts',(34.5732684409796,85.4029940074072,122.));
#49387=CARTESIAN_POINT('Ctrl Pts',(34.5592417005919,85.4159028804059,122.));
#49388=CARTESIAN_POINT('Ctrl Pts',(34.5453464389343,85.4289307716471,122.));
#49389=CARTESIAN_POINT('Ctrl Pts',(34.4729163426157,85.4968396344438,122.));
#49390=CARTESIAN_POINT('Ctrl Pts',(34.4039519336089,85.5680704126807,122.));
#49391=CARTESIAN_POINT('Ctrl Pts',(34.33869316176,85.6423323835084,122.));
#49392=CARTESIAN_POINT('Ctrl Pts',(34.2737934142962,85.7161857984033,122.));
#49393=CARTESIAN_POINT('Ctrl Pts',(34.2125581562074,85.7930379420743,122.));
#49394=CARTESIAN_POINT('Ctrl Pts',(34.1552670083591,85.8726296318035,122.));
#49395=CARTESIAN_POINT('Ctrl Pts',(34.1001040937713,85.9492646748656,122.));
#49396=CARTESIAN_POINT('Ctrl Pts',(34.0485975400135,86.0284402461049,122.));
#49397=CARTESIAN_POINT('Ctrl Pts',(34.0010417953143,86.1099385723801,122.));
#49398=CARTESIAN_POINT('Ctrl Pts',(33.9810954653113,86.144121456506,122.));
#49399=CARTESIAN_POINT('Ctrl Pts',(33.9618447387099,86.1787130708316,122.));
#49400=CARTESIAN_POINT('Ctrl Pts',(33.9433139257018,86.2136976438174,122.));
#49401=CARTESIAN_POINT('Ctrl Pts',(33.9304313899784,86.2380187575787,122.));
#49402=CARTESIAN_POINT('Ctrl Pts',(33.9178968184969,86.2625297896542,122.));
#49403=CARTESIAN_POINT('Ctrl Pts',(33.9057188451145,86.2872254467939,122.));
#49404=CARTESIAN_POINT('Ctrl Pts',(33.8978104958471,86.3032627525029,122.));
#49405=CARTESIAN_POINT('Ctrl Pts',(33.8900514222255,86.3193805307655,122.));
#49406=CARTESIAN_POINT('Ctrl Pts',(33.8824541646778,86.335555142464,122.));
#49407=CARTESIAN_POINT('Ctrl Pts',(33.8403338623352,86.4252295454634,122.));
#49408=CARTESIAN_POINT('Ctrl Pts',(33.8031123934132,86.5167875390704,122.));
#49409=CARTESIAN_POINT('Ctrl Pts',(33.7710810415748,86.6099567585531,122.));
#49410=CARTESIAN_POINT('Ctrl Pts',(33.7412012885639,86.696867647622,122.));
#49411=CARTESIAN_POINT('Ctrl Pts',(33.715837986679,86.7851813667476,122.));
#49412=CARTESIAN_POINT('Ctrl Pts',(33.6952781137301,86.8746855295874,122.));
#49413=CARTESIAN_POINT('Ctrl Pts',(33.6937976263072,86.881130597984,122.));
#49414=CARTESIAN_POINT('Ctrl Pts',(33.6923420683187,86.8875818402717,122.));
#49415=CARTESIAN_POINT('Ctrl Pts',(33.6909115575437,86.8940391774638,122.));
#49416=CARTESIAN_POINT('Ctrl Pts',(33.6703053385859,86.987055816269,122.));
#49417=CARTESIAN_POINT('Ctrl Pts',(33.6548921451018,87.081338120739,122.));
#49418=CARTESIAN_POINT('Ctrl Pts',(33.6445950569561,87.1764782244295,122.));
#49419=CARTESIAN_POINT('Ctrl Pts',(33.6387985396345,87.2300352350339,122.));
#49420=CARTESIAN_POINT('Ctrl Pts',(33.6346241821948,87.2838638828705,122.));
#49421=CARTESIAN_POINT('Ctrl Pts',(33.6320650250057,87.3378887730391,122.));
#49422=CARTESIAN_POINT('Ctrl Pts',(33.6314041425466,87.3518402811434,122.));
#49423=CARTESIAN_POINT('Ctrl Pts',(33.6308510967089,87.3658042773908,122.));
#49424=CARTESIAN_POINT('Ctrl Pts',(33.6304060090372,87.3797660938872,122.));
#49425=CARTESIAN_POINT('Ctrl Pts',(33.6274345999427,87.4729752999515,122.));
#49426=CARTESIAN_POINT('Ctrl Pts',(33.6292623454294,87.5662427431663,122.));
#49427=CARTESIAN_POINT('Ctrl Pts',(33.6357543510792,87.6591933437351,122.));
#49428=CARTESIAN_POINT('Ctrl Pts',(33.6422571510453,87.7522984941045,122.));
#49429=CARTESIAN_POINT('Ctrl Pts',(33.6534401126504,87.8450867269761,122.));
#49430=CARTESIAN_POINT('Ctrl Pts',(33.6692186001989,87.9371689927436,122.));
#49431=CARTESIAN_POINT('Ctrl Pts',(33.6847714909114,88.0279346894962,122.));
#49432=CARTESIAN_POINT('Ctrl Pts',(33.7047898966492,88.1180153063821,122.));
#49433=CARTESIAN_POINT('Ctrl Pts',(33.7292357852524,88.2070130445517,122.));
#49434=CARTESIAN_POINT('Ctrl Pts',(33.7383345490649,88.2401380175319,122.));
#49435=CARTESIAN_POINT('Ctrl Pts',(33.7480470632381,88.2731126593096,122.));
#49436=CARTESIAN_POINT('Ctrl Pts',(33.7583727282114,88.305915192543,122.));
#49437=CARTESIAN_POINT('Ctrl Pts',(33.7653672088676,88.3281352321018,122.));
#49438=CARTESIAN_POINT('Ctrl Pts',(33.7726430513325,88.3502762836458,122.));
#49439=CARTESIAN_POINT('Ctrl Pts',(33.7802002483622,88.3723313649238,122.));
#49440=CARTESIAN_POINT('Ctrl Pts',(33.7847163076137,88.3855111263426,122.));
#49441=CARTESIAN_POINT('Ctrl Pts',(33.7893324946004,88.3986590147143,122.));
#49442=CARTESIAN_POINT('Ctrl Pts',(33.7940453374235,88.4117643917557,122.));
#49443=CARTESIAN_POINT('Ctrl Pts',(33.8256770944825,88.4997253355632,122.));
#49444=CARTESIAN_POINT('Ctrl Pts',(33.8616980723005,88.5858885320335,122.));
#49445=CARTESIAN_POINT('Ctrl Pts',(33.9020437068047,88.6698397368365,122.));
#49446=CARTESIAN_POINT('Ctrl Pts',(33.9323029326829,88.7328031404388,122.));
#49447=CARTESIAN_POINT('Ctrl Pts',(33.964995825274,88.7945218067863,122.));
#49448=CARTESIAN_POINT('Ctrl Pts',(34.0001111084258,88.8548054454097,122.));
#49449=CARTESIAN_POINT('Ctrl Pts',(34.0135804337297,88.8779287087366,122.));
#49450=CARTESIAN_POINT('Ctrl Pts',(34.0274062973137,88.900840676073,122.));
#49451=CARTESIAN_POINT('Ctrl Pts',(34.0415885432314,88.9235299643773,122.));
#49452=CARTESIAN_POINT('Ctrl Pts',(34.0517128286096,88.939727175394,122.));
#49453=CARTESIAN_POINT('Ctrl Pts',(34.0620195670163,88.9558119726629,122.));
#49454=CARTESIAN_POINT('Ctrl Pts',(34.0724986266519,88.971765210655,122.));
#49455=CARTESIAN_POINT('Ctrl Pts',(34.1196852037718,89.0436016846323,122.));
#49456=CARTESIAN_POINT('Ctrl Pts',(34.1704067057004,89.1128447071754,122.));
#49457=CARTESIAN_POINT('Ctrl Pts',(34.2246302409937,89.1791422786934,122.));
#49458=CARTESIAN_POINT('Ctrl Pts',(34.2734266590585,89.2388042686205,122.));
#49459=CARTESIAN_POINT('Ctrl Pts',(34.3250597723479,89.2960808303433,122.));
#49460=CARTESIAN_POINT('Ctrl Pts',(34.3795261020684,89.3506856242928,122.));
#49461=CARTESIAN_POINT('Ctrl Pts',(34.398608673689,89.3698167076009,122.));
#49462=CARTESIAN_POINT('Ctrl Pts',(34.4180391901862,89.3886195422968,122.));
#49463=CARTESIAN_POINT('Ctrl Pts',(34.437807076635,89.4070896409747,122.));
#49464=CARTESIAN_POINT('Origin',(36.3549260746835,87.7685555885722,114.));
#49465=CARTESIAN_POINT('Origin',(87.7685555885722,-36.3549260746835,107.));
#49466=CARTESIAN_POINT('Ctrl Pts',(85.8550895919077,-34.718938871308,107.));
#49467=CARTESIAN_POINT('Ctrl Pts',(85.7929520057252,-34.7773329442881,107.));
#49468=CARTESIAN_POINT('Ctrl Pts',(85.7341897911883,-34.8389809220769,107.));
#49469=CARTESIAN_POINT('Ctrl Pts',(85.6788149294007,-34.9035063296324,107.));
#49470=CARTESIAN_POINT('Ctrl Pts',(85.6220849950857,-34.9696107317763,107.));
#49471=CARTESIAN_POINT('Ctrl Pts',(85.5689097568226,-35.0387356044574,107.));
#49472=CARTESIAN_POINT('Ctrl Pts',(85.5193309848105,-35.1105224280004,107.));
#49473=CARTESIAN_POINT('Ctrl Pts',(85.5063931427471,-35.1292555782486,107.));
#49474=CARTESIAN_POINT('Ctrl Pts',(85.493700382435,-35.1481702177695,107.));
#49475=CARTESIAN_POINT('Ctrl Pts',(85.4812538215899,-35.1672604086816,107.));
#49476=CARTESIAN_POINT('Ctrl Pts',(85.4710839964377,-35.1828586053331,107.));
#49477=CARTESIAN_POINT('Ctrl Pts',(85.4610780981857,-35.1985749107462,107.));
#49478=CARTESIAN_POINT('Ctrl Pts',(85.4512455841464,-35.2143914910608,107.));
#49479=CARTESIAN_POINT('Ctrl Pts',(85.4038014085985,-35.2907101833113,107.));
#49480=CARTESIAN_POINT('Ctrl Pts',(85.3603407964668,-35.3694362324884,107.));
#49481=CARTESIAN_POINT('Ctrl Pts',(85.3208984357077,-35.4501770885667,107.));
#49482=CARTESIAN_POINT('Ctrl Pts',(85.2890699426178,-35.5153319051215,107.));
#49483=CARTESIAN_POINT('Ctrl Pts',(85.2598585869202,-35.5817998282397,107.));
#49484=CARTESIAN_POINT('Ctrl Pts',(85.2332997549837,-35.6493923856423,107.));
#49485=CARTESIAN_POINT('Ctrl Pts',(85.2226981116036,-35.6763736998223,107.));
#49486=CARTESIAN_POINT('Ctrl Pts',(85.2125193083794,-35.7035343666522,107.));
#49487=CARTESIAN_POINT('Ctrl Pts',(85.2027663566685,-35.7308629441227,107.));
#49488=CARTESIAN_POINT('Ctrl Pts',(85.1975254516455,-35.7455483935316,107.));
#49489=CARTESIAN_POINT('Ctrl Pts',(85.1924078966035,-35.7602815101748,107.));
#49490=CARTESIAN_POINT('Ctrl Pts',(85.1874181581136,-35.7750480411479,107.));
#49491=CARTESIAN_POINT('Ctrl Pts',(85.1578793261422,-35.8624646618987,107.));
#49492=CARTESIAN_POINT('Ctrl Pts',(85.1327759615655,-35.9511623852848,107.));
#49493=CARTESIAN_POINT('Ctrl Pts',(85.112140634563,-36.0407434031081,107.));
#49494=CARTESIAN_POINT('Ctrl Pts',(85.0911838525134,-36.1317199050104,107.));
#49495=CARTESIAN_POINT('Ctrl Pts',(85.0748348968748,-36.2236082408856,107.));
#49496=CARTESIAN_POINT('Ctrl Pts',(85.0631697088413,-36.3160249059585,107.));
#49497=CARTESIAN_POINT('Ctrl Pts',(85.0515952389178,-36.4077228629263,107.));
#49498=CARTESIAN_POINT('Ctrl Pts',(85.0446316260211,-36.4999418935486,107.));
#49499=CARTESIAN_POINT('Ctrl Pts',(85.0423999978617,-36.5923265809498,107.));
#49500=CARTESIAN_POINT('Ctrl Pts',(85.041289386105,-36.6383035594764,107.));
#49501=CARTESIAN_POINT('Ctrl Pts',(85.041351528784,-36.6843217800467,107.));
#49502=CARTESIAN_POINT('Ctrl Pts',(85.0426061541673,-36.7303381327728,107.));
#49503=CARTESIAN_POINT('Ctrl Pts',(85.0429759351538,-36.7439007248693,107.));
#49504=CARTESIAN_POINT('Ctrl Pts',(85.0434493271816,-36.7574631553908,107.));
#49505=CARTESIAN_POINT('Ctrl Pts',(85.0440268917257,-36.7710243206044,107.));
#49506=CARTESIAN_POINT('Ctrl Pts',(85.0446473903427,-36.7855935741113,107.));
#49507=CARTESIAN_POINT('Ctrl Pts',(85.0453877221699,-36.8001515800913,107.));
#49508=CARTESIAN_POINT('Ctrl Pts',(85.0462479357691,-36.81469441234,107.));
#49509=CARTESIAN_POINT('Ctrl Pts',(85.0518997327028,-36.9102440930122,107.));
#49510=CARTESIAN_POINT('Ctrl Pts',(85.0627241729578,-37.0051720608794,107.));
#49511=CARTESIAN_POINT('Ctrl Pts',(85.0787917132112,-37.0990826739641,107.));
#49512=CARTESIAN_POINT('Ctrl Pts',(85.0811720250204,-37.1129949802541,107.));
#49513=CARTESIAN_POINT('Ctrl Pts',(85.0836674925339,-37.1268849924206,107.));
#49514=CARTESIAN_POINT('Ctrl Pts',(85.0862784373429,-37.1407514548178,107.));
#49515=CARTESIAN_POINT('Ctrl Pts',(85.1032240769739,-37.2307480238492,107.));
#49516=CARTESIAN_POINT('Ctrl Pts',(85.125029602379,-37.3197524279253,107.));
#49517=CARTESIAN_POINT('Ctrl Pts',(85.1513924630333,-37.4075324179485,107.));
#49518=CARTESIAN_POINT('Ctrl Pts',(85.1783512727901,-37.4972967300434,107.));
#49519=CARTESIAN_POINT('Ctrl Pts',(85.2100759987119,-37.5857813453147,107.));
#49520=CARTESIAN_POINT('Ctrl Pts',(85.2462973464537,-37.6727342179368,107.));
#49521=CARTESIAN_POINT('Ctrl Pts',(85.2587874244706,-37.7027178665459,107.));
#49522=CARTESIAN_POINT('Ctrl Pts',(85.2718126244585,-37.7325193017317,107.));
#49523=CARTESIAN_POINT('Ctrl Pts',(85.2853632768146,-37.7621278496479,107.));
#49524=CARTESIAN_POINT('Ctrl Pts',(85.2920542822302,-37.776747880422,107.));
#49525=CARTESIAN_POINT('Ctrl Pts',(85.2988734117231,-37.7913208786982,107.));
#49526=CARTESIAN_POINT('Ctrl Pts',(85.3058195604008,-37.8058455369217,107.));
#49527=CARTESIAN_POINT('Ctrl Pts',(85.3113133364161,-37.8173332292649,107.));
#49528=CARTESIAN_POINT('Ctrl Pts',(85.3168861277483,-37.8287896584371,107.));
#49529=CARTESIAN_POINT('Ctrl Pts',(85.3225327933933,-37.8402052475552,107.));
#49530=CARTESIAN_POINT('Ctrl Pts',(85.3652567183844,-37.9265781273875,107.));
#49531=CARTESIAN_POINT('Ctrl Pts',(85.4122715037245,-38.0107526954899,107.));
#49532=CARTESIAN_POINT('Ctrl Pts',(85.4632344929551,-38.0924793134259,107.));
#49533=CARTESIAN_POINT('Ctrl Pts',(85.5152082030099,-38.175826770247,107.));
#49534=CARTESIAN_POINT('Ctrl Pts',(85.5712885886939,-38.2566289878826,107.));
#49535=CARTESIAN_POINT('Ctrl Pts',(85.6311672093088,-38.3346141495021,107.));
#49536=CARTESIAN_POINT('Ctrl Pts',(85.6915326709731,-38.4132333667752,107.));
#49537=CARTESIAN_POINT('Ctrl Pts',(85.755758840285,-38.488990370614,107.));
#49538=CARTESIAN_POINT('Ctrl Pts',(85.8235790230849,-38.5615873806944,107.));
#49539=CARTESIAN_POINT('Ctrl Pts',(85.8605797386839,-38.601194194071,107.));
#49540=CARTESIAN_POINT('Ctrl Pts',(85.8986510202273,-38.6398600347398,107.));
#49541=CARTESIAN_POINT('Ctrl Pts',(85.9377549083663,-38.677532768249,107.));
#49542=CARTESIAN_POINT('Ctrl Pts',(85.9497220449507,-38.6890619222251,107.));
#49543=CARTESIAN_POINT('Ctrl Pts',(85.9617859169551,-38.7004980423369,107.));
#49544=CARTESIAN_POINT('Ctrl Pts',(85.9739454993829,-38.7118395722585,107.));
#49545=CARTESIAN_POINT('Ctrl Pts',(85.9844912868876,-38.7216758775132,107.));
#49546=CARTESIAN_POINT('Ctrl Pts',(85.995107953485,-38.7314399182998,107.));
#49547=CARTESIAN_POINT('Ctrl Pts',(86.0057857170979,-38.7411226995933,107.));
#49548=CARTESIAN_POINT('Ctrl Pts',(86.0813601784838,-38.8096549323251,107.));
#49549=CARTESIAN_POINT('Ctrl Pts',(86.1601113614648,-38.8742308219701,107.));
#49550=CARTESIAN_POINT('Ctrl Pts',(86.2417119176664,-38.9345685954586,107.));
#49551=CARTESIAN_POINT('Ctrl Pts',(86.3234166776699,-38.9949834202038,107.));
#49552=CARTESIAN_POINT('Ctrl Pts',(86.4079786662187,-39.0511501363062,107.));
#49553=CARTESIAN_POINT('Ctrl Pts',(86.4951145538286,-39.1027600899502,107.));
#49554=CARTESIAN_POINT('Ctrl Pts',(86.5805182077147,-39.1533440541351,107.));
#49555=CARTESIAN_POINT('Ctrl Pts',(86.6683951053336,-39.1995513068559,107.));
#49556=CARTESIAN_POINT('Ctrl Pts',(86.7585125705286,-39.2410554346124,107.));
#49557=CARTESIAN_POINT('Ctrl Pts',(86.7988626922243,-39.2596389200914,107.));
#49558=CARTESIAN_POINT('Ctrl Pts',(86.8396624052801,-39.2772789765588,107.));
#49559=CARTESIAN_POINT('Ctrl Pts',(86.8808925773498,-39.2939433559961,107.));
#49560=CARTESIAN_POINT('Ctrl Pts',(86.9113122273115,-39.3062383468696,107.));
#49561=CARTESIAN_POINT('Ctrl Pts',(86.9419662212818,-39.3180021842847,107.));
#49562=CARTESIAN_POINT('Ctrl Pts',(86.9728422903212,-39.3292375489681,107.));
#49563=CARTESIAN_POINT('Ctrl Pts',(88.5623548711045,-39.3241490284294,107.));
#49564=CARTESIAN_POINT('Ctrl Pts',(88.657188760456,-39.2894583680844,107.));
#49565=CARTESIAN_POINT('Ctrl Pts',(88.7499794959736,-39.2497768208657,107.));
#49566=CARTESIAN_POINT('Ctrl Pts',(88.8404861547626,-39.2054247380955,107.));
#49567=CARTESIAN_POINT('Ctrl Pts',(88.9322657038653,-39.1604488853474,107.));
#49568=CARTESIAN_POINT('Ctrl Pts',(89.0216971461717,-39.1106694981297,107.));
#49569=CARTESIAN_POINT('Ctrl Pts',(89.1084952256704,-39.0563799521656,107.));
#49570=CARTESIAN_POINT('Ctrl Pts',(89.1330082394292,-39.0410478112373,107.));
#49571=CARTESIAN_POINT('Ctrl Pts',(89.1573109820009,-39.0253557402474,107.));
#49572=CARTESIAN_POINT('Ctrl Pts',(89.1813964317758,-39.009309891666,107.));
#49573=CARTESIAN_POINT('Ctrl Pts',(89.2007259962726,-38.9964324379353,107.));
#49574=CARTESIAN_POINT('Ctrl Pts',(89.2199177127268,-38.9833254998213,107.));
#49575=CARTESIAN_POINT('Ctrl Pts',(89.2389486655507,-38.9700060224475,107.));
#49576=CARTESIAN_POINT('Ctrl Pts',(89.3216557642,-38.912120569244,107.));
#49577=CARTESIAN_POINT('Ctrl Pts',(89.4014080028997,-38.8501729673376,107.));
#49578=CARTESIAN_POINT('Ctrl Pts',(89.4779390201902,-38.7844605786764,107.));
#49579=CARTESIAN_POINT('Ctrl Pts',(89.5369322084152,-38.7338068248096,107.));
#49580=CARTESIAN_POINT('Ctrl Pts',(89.5940107289622,-38.6809151435346,107.));
#49581=CARTESIAN_POINT('Ctrl Pts',(89.6490350139468,-38.6259099657521,107.));
#49582=CARTESIAN_POINT('Ctrl Pts',(89.6783237536614,-38.5966313965626,107.));
#49583=CARTESIAN_POINT('Ctrl Pts',(89.7070301904271,-38.5667538616209,107.));
#49584=CARTESIAN_POINT('Ctrl Pts',(89.7351312539879,-38.5362952954457,107.));
#49585=CARTESIAN_POINT('Ctrl Pts',(89.7447672571528,-38.5258508921785,107.));
#49586=CARTESIAN_POINT('Ctrl Pts',(89.7543313446827,-38.5153388769912,107.));
#49587=CARTESIAN_POINT('Ctrl Pts',(89.7638159499299,-38.5047675856174,107.));
#49588=CARTESIAN_POINT('Ctrl Pts',(89.8296131402258,-38.4314317690959,107.));
#49589=CARTESIAN_POINT('Ctrl Pts',(89.8916781800482,-38.3551493287763,107.));
#49590=CARTESIAN_POINT('Ctrl Pts',(89.9497673009232,-38.2761988239649,107.));
#49591=CARTESIAN_POINT('Ctrl Pts',(90.0073299643537,-38.1979638417915,107.));
#49592=CARTESIAN_POINT('Ctrl Pts',(90.0609888830627,-38.1171081523236,107.));
#49593=CARTESIAN_POINT('Ctrl Pts',(90.1104611132468,-38.0338804239825,107.));
#49594=CARTESIAN_POINT('Ctrl Pts',(90.1585190532459,-37.9530319730435,107.));
#49595=CARTESIAN_POINT('Ctrl Pts',(90.2026264658774,-37.8699444672167,107.));
#49596=CARTESIAN_POINT('Ctrl Pts',(90.2424761999497,-37.784835528788,107.));
#49597=CARTESIAN_POINT('Ctrl Pts',(90.2632806160433,-37.7404025655683,107.));
#49598=CARTESIAN_POINT('Ctrl Pts',(90.2829237462882,-37.6954185336514,107.));
#49599=CARTESIAN_POINT('Ctrl Pts',(90.3013561905801,-37.649914163883,107.));
#49600=CARTESIAN_POINT('Ctrl Pts',(90.3084142720207,-37.6324898037361,107.));
#49601=CARTESIAN_POINT('Ctrl Pts',(90.3152947941375,-37.6149891503516,107.));
#49602=CARTESIAN_POINT('Ctrl Pts',(90.3219948213491,-37.5974139378534,107.));
#49603=CARTESIAN_POINT('Ctrl Pts',(90.3272365572998,-37.5836640499377,107.));
#49604=CARTESIAN_POINT('Ctrl Pts',(90.3323679171457,-37.5698680261879,107.));
#49605=CARTESIAN_POINT('Ctrl Pts',(90.3373823657084,-37.5560414099326,107.));
#49606=CARTESIAN_POINT('Ctrl Pts',(90.3690660536423,-37.4686782254983,107.));
#49607=CARTESIAN_POINT('Ctrl Pts',(90.396140915987,-37.3799541005099,107.));
#49608=CARTESIAN_POINT('Ctrl Pts',(90.4183556967036,-37.290092587238,107.));
#49609=CARTESIAN_POINT('Ctrl Pts',(90.4233396687901,-37.2699318087223,107.));
#49610=CARTESIAN_POINT('Ctrl Pts',(90.4280788071154,-37.2497137405306,107.));
#49611=CARTESIAN_POINT('Ctrl Pts',(90.432569913541,-37.2294408516372,107.));
#49612=CARTESIAN_POINT('Ctrl Pts',(90.4529356667892,-37.1375096850815,107.));
#49613=CARTESIAN_POINT('Ctrl Pts',(90.4682052082885,-37.0444509023185,107.));
#49614=CARTESIAN_POINT('Ctrl Pts',(90.4784883629424,-36.9506560897443,107.));
#49615=CARTESIAN_POINT('Ctrl Pts',(90.4892222257724,-36.852750273269,107.));
#49616=CARTESIAN_POINT('Ctrl Pts',(90.4945230058311,-36.7540412554223,107.));
#49617=CARTESIAN_POINT('Ctrl Pts',(90.4944581501752,-36.654989052644,107.));
#49618=CARTESIAN_POINT('Ctrl Pts',(90.4944327816927,-36.616244489274,107.));
#49619=CARTESIAN_POINT('Ctrl Pts',(90.4935858683382,-36.5774476751947,107.));
#49620=CARTESIAN_POINT('Ctrl Pts',(90.4919192227104,-36.5386273681288,107.));
#49621=CARTESIAN_POINT('Ctrl Pts',(90.4913861838263,-36.526211571505,107.));
#49622=CARTESIAN_POINT('Ctrl Pts',(90.4907692984578,-36.5137946831277,107.));
#49623=CARTESIAN_POINT('Ctrl Pts',(90.4900693277303,-36.5013873123494,107.));
#49624=CARTESIAN_POINT('Ctrl Pts',(90.4848301144401,-36.4085193404114,107.));
#49625=CARTESIAN_POINT('Ctrl Pts',(90.4749344807815,-36.3160346027814,107.));
#49626=CARTESIAN_POINT('Ctrl Pts',(90.460505885687,-36.2243046763152,107.));
#49627=CARTESIAN_POINT('Ctrl Pts',(90.4461112789299,-36.132790831018,107.));
#49628=CARTESIAN_POINT('Ctrl Pts',(90.4272046315754,-36.0420272996474,107.));
#49629=CARTESIAN_POINT('Ctrl Pts',(90.403859856107,-35.9523999917909,107.));
#49630=CARTESIAN_POINT('Ctrl Pts',(90.38091122944,-35.8642936131306,107.));
#49631=CARTESIAN_POINT('Ctrl Pts',(90.3536733546584,-35.7772844376027,107.));
#49632=CARTESIAN_POINT('Ctrl Pts',(90.3221760039316,-35.69176815752,107.));
#49633=CARTESIAN_POINT('Ctrl Pts',(90.3063345620639,-35.6487581535541,107.));
#49634=CARTESIAN_POINT('Ctrl Pts',(90.2894150702694,-35.6061263179827,107.));
#49635=CARTESIAN_POINT('Ctrl Pts',(90.2714178987872,-35.5639267820646,107.));
#49636=CARTESIAN_POINT('Ctrl Pts',(90.2658521882548,-35.5508763756854,107.));
#49637=CARTESIAN_POINT('Ctrl Pts',(90.2601833945565,-35.537867334519,107.));
#49638=CARTESIAN_POINT('Ctrl Pts',(90.2544114877658,-35.5249013171903,107.));
#49639=CARTESIAN_POINT('Ctrl Pts',(90.2487320296277,-35.5121429766095,107.));
#49640=CARTESIAN_POINT('Ctrl Pts',(90.2429562163594,-35.4994341571851,107.));
#49641=CARTESIAN_POINT('Ctrl Pts',(90.2370858376439,-35.4867793444242,107.));
#49642=CARTESIAN_POINT('Ctrl Pts',(90.1996060377885,-35.4059839013239,107.));
#49643=CARTESIAN_POINT('Ctrl Pts',(90.1582560808094,-35.3273452367495,107.));
#49644=CARTESIAN_POINT('Ctrl Pts',(90.1131056428511,-35.2512109414872,107.));
#49645=CARTESIAN_POINT('Ctrl Pts',(90.0687126367815,-35.1763538551657,107.));
#49646=CARTESIAN_POINT('Ctrl Pts',(90.0206451378295,-35.1039171481911,107.));
#49647=CARTESIAN_POINT('Ctrl Pts',(89.9689331610032,-35.0342653872491,107.));
#49648=CARTESIAN_POINT('Ctrl Pts',(89.9187987000732,-34.9667384099034,107.));
#49649=CARTESIAN_POINT('Ctrl Pts',(89.8652382823866,-34.9018286150414,107.));
#49650=CARTESIAN_POINT('Ctrl Pts',(89.8082515482804,-34.8399084971231,107.));
#49651=CARTESIAN_POINT('Ctrl Pts',(89.7872839743132,-34.8171257447357,107.));
#49652=CARTESIAN_POINT('Ctrl Pts',(89.7658523072769,-34.7947481639537,107.));
#49653=CARTESIAN_POINT('Ctrl Pts',(89.7439557180669,-34.7727959191418,107.));
#49654=CARTESIAN_POINT('Ctrl Pts',(89.7248782826417,-34.7536699936919,107.));
#49655=CARTESIAN_POINT('Ctrl Pts',(89.7054479137747,-34.7348669548371,107.));
#49656=CARTESIAN_POINT('Ctrl Pts',(89.6856747483211,-34.7163919311051,107.));
#49657=CARTESIAN_POINT('Origin',(87.7685555885722,-36.3549260746835,124.208423447177));
#49658=CARTESIAN_POINT('Ctrl Pts',(84.691755941294,-36.3529984690253,121.708423447177));
#49659=CARTESIAN_POINT('Ctrl Pts',(84.6908332620481,-36.2297235581181,121.702019850418));
#49660=CARTESIAN_POINT('Ctrl Pts',(84.7533597477157,-35.0938166732982,121.642966745928));
#49661=CARTESIAN_POINT('Ctrl Pts',(86.1660867790185,-33.1013875491387,121.531264133707));
#49662=CARTESIAN_POINT('Ctrl Pts',(89.6167530478622,-33.2347627935352,121.373315610515));
#49663=CARTESIAN_POINT('Ctrl Pts',(91.3916431606975,-36.1967043155478,121.215367087322));
#49664=CARTESIAN_POINT('Ctrl Pts',(89.8816248388871,-39.3022907437215,121.05741856413));
#49665=CARTESIAN_POINT('Ctrl Pts',(86.455733936694,-39.7354988616288,120.899470040937));
#49666=CARTESIAN_POINT('Ctrl Pts',(84.8091869094529,-37.7971275491863,120.783138335286));
#49667=CARTESIAN_POINT('Ctrl Pts',(84.6923092768517,-36.5704857478685,120.719456137367));
#49668=CARTESIAN_POINT('Ctrl Pts',(84.6942411071791,-36.3576097921547,120.708423447177));
#49669=CARTESIAN_POINT('Ctrl Pts',(84.6982768768212,-36.3579423122256,121.791576552823));
#49670=CARTESIAN_POINT('Ctrl Pts',(84.7032618946881,-35.6649235243351,121.755752019753));
#49671=CARTESIAN_POINT('Ctrl Pts',(85.2756495863919,-33.9437323409503,121.667277978953));
#49672=CARTESIAN_POINT('Ctrl Pts',(88.1200899288066,-32.7460654788916,121.526154430423));
#49673=CARTESIAN_POINT('Ctrl Pts',(90.9824824119093,-34.6751864614649,121.36820590723));
#49674=CARTESIAN_POINT('Ctrl Pts',(90.9320921383769,-38.128468693812,121.210257384038));
#49675=CARTESIAN_POINT('Ctrl Pts',(88.0128423765734,-39.9731538131696,121.052308860845));
#49676=CARTESIAN_POINT('Ctrl Pts',(85.237995407928,-38.7047118441066,120.912748583773));
#49677=CARTESIAN_POINT('Ctrl Pts',(84.7024656403392,-37.0159744647791,120.825837814433));
#49678=CARTESIAN_POINT('Ctrl Pts',(84.69811441609,-36.3527751945784,120.791576552823));
#49679=CARTESIAN_POINT('Ctrl Pts',(89.6820215852375,-34.7189388713087,122.));
#49680=CARTESIAN_POINT('Ctrl Pts',(90.223216971559,-35.3519260775303,121.947350492269));
#49681=CARTESIAN_POINT('Ctrl Pts',(90.618554680914,-37.1869584406053,121.842051476808));
#49682=CARTESIAN_POINT('Ctrl Pts',(88.6277565795612,-39.2001257327075,121.684102953615));
#49683=CARTESIAN_POINT('Ctrl Pts',(85.8568533037203,-38.6278813322613,121.526154430423));
#49684=CARTESIAN_POINT('Ctrl Pts',(84.8197363293867,-35.9976144118095,121.36820590723));
#49685=CARTESIAN_POINT('Ctrl Pts',(86.455975393989,-33.6899567439338,121.210257384038));
#49686=CARTESIAN_POINT('Ctrl Pts',(89.282411812344,-33.7992042395474,121.052308860845));
#49687=CARTESIAN_POINT('Ctrl Pts',(90.7362220804628,-36.2253268299709,120.894360337653));
#49688=CARTESIAN_POINT('Ctrl Pts',(89.4993679645826,-38.7691087830952,120.73641181446));
#49689=CARTESIAN_POINT('Ctrl Pts',(86.6932250180163,-39.1239490098176,120.578463291268));
#49690=CARTESIAN_POINT('Ctrl Pts',(84.8620583484337,-36.9682371583514,120.420514768075));
#49691=CARTESIAN_POINT('Ctrl Pts',(85.6661210457745,-34.2564369070682,120.262566244883));
#49692=CARTESIAN_POINT('Ctrl Pts',(88.376398796949,-33.4472816613919,120.10461772169));
#49693=CARTESIAN_POINT('Ctrl Pts',(90.5355628215429,-35.2743949431641,119.946669198498));
#49694=CARTESIAN_POINT('Ctrl Pts',(90.1859659201536,-38.0811949957465,119.788720675306));
#49695=CARTESIAN_POINT('Ctrl Pts',(87.6445764098185,-39.3228385196818,119.630772152113));
#49696=CARTESIAN_POINT('Ctrl Pts',(85.2155951394299,-37.8735665809373,119.47282362892));
#49697=CARTESIAN_POINT('Ctrl Pts',(85.101305420113,-35.047389246126,119.314875105728));
#49698=CARTESIAN_POINT('Ctrl Pts',(87.4053303288848,-33.4067159017789,119.156926582536));
#49699=CARTESIAN_POINT('Ctrl Pts',(90.0386805233624,-34.4390949995566,118.998978059343));
#49700=CARTESIAN_POINT('Ctrl Pts',(90.613777487181,-37.2084998929576,118.841029536151));
#49701=CARTESIAN_POINT('Ctrl Pts',(88.6091982866193,-39.2039953523912,118.683081012958));
#49702=CARTESIAN_POINT('Ctrl Pts',(85.8424339199087,-38.6163263546765,118.525132489766));
#49703=CARTESIAN_POINT('Ctrl Pts',(84.82202548926,-35.9783144973492,118.367183966573));
#49704=CARTESIAN_POINT('Ctrl Pts',(86.4731462852742,-33.6817649045862,118.209235443381));
#49705=CARTESIAN_POINT('Ctrl Pts',(89.2987752983603,-33.8088892434902,118.051286920188));
#49706=CARTESIAN_POINT('Ctrl Pts',(90.7370006401761,-36.2444277433863,117.893338396996));
#49707=CARTESIAN_POINT('Ctrl Pts',(89.4838271348459,-38.7801517194402,117.735389873803));
#49708=CARTESIAN_POINT('Ctrl Pts',(86.6754690861509,-39.1169973633819,117.577441350611));
#49709=CARTESIAN_POINT('Ctrl Pts',(84.8581793244705,-36.9495569744204,117.419492827418));
#49710=CARTESIAN_POINT('Ctrl Pts',(85.679639206362,-34.2429828335689,117.261544304226));
#49711=CARTESIAN_POINT('Ctrl Pts',(88.3950560404819,-33.4512433975761,117.103595781033));
#49712=CARTESIAN_POINT('Ctrl Pts',(90.5424439690061,-35.2921847334048,116.945647257841));
#49713=CARTESIAN_POINT('Ctrl Pts',(90.174831666992,-38.0966813215517,116.787698734649));
#49714=CARTESIAN_POINT('Ctrl Pts',(87.6255220282537,-39.3219814004557,116.629750211456));
#49715=CARTESIAN_POINT('Ctrl Pts',(85.2058965684871,-37.8571426543901,116.471801688264));
#49716=CARTESIAN_POINT('Ctrl Pts',(85.1097561024807,-35.0302898233568,116.313853165071));
#49717=CARTESIAN_POINT('Ctrl Pts',(87.4242682667827,-33.4044443944109,116.155904641879));
#49718=CARTESIAN_POINT('Ctrl Pts',(90.0509352747254,-34.4537109701243,115.997956118686));
#49719=CARTESIAN_POINT('Ctrl Pts',(90.6082380366736,-37.2267514582979,115.840007595494));
#49720=CARTESIAN_POINT('Ctrl Pts',(88.5908870879659,-39.2093343865188,115.682059072301));
#49721=CARTESIAN_POINT('Ctrl Pts',(85.8279531788398,-38.6039121113032,115.524110549109));
#49722=CARTESIAN_POINT('Ctrl Pts',(84.824504453864,-35.9594025965029,115.366162025916));
#49723=CARTESIAN_POINT('Ctrl Pts',(86.4903373534603,-33.6735021900661,115.208213502724));
#49724=CARTESIAN_POINT('Ctrl Pts',(89.3150918515823,-33.818767267991,115.050264979531));
#49725=CARTESIAN_POINT('Ctrl Pts',(90.7376489558074,-36.2634904021606,114.892316456339));
#49726=CARTESIAN_POINT('Ctrl Pts',(89.4682194048531,-38.7911154797165,114.734367933146));
#49727=CARTESIAN_POINT('Ctrl Pts',(86.6577563646153,-39.1099217170804,114.576419409954));
#49728=CARTESIAN_POINT('Ctrl Pts',(84.8544211973079,-36.9308571948879,114.418470886761));
#49729=CARTESIAN_POINT('Ctrl Pts',(85.6932430531688,-34.2296134421594,114.260522363569));
#49730=CARTESIAN_POINT('Ctrl Pts',(88.4136876671025,-33.4553260148786,114.102573840377));
#49731=CARTESIAN_POINT('Ctrl Pts',(90.5492106462378,-35.3100177744735,113.944625317184));
#49732=CARTESIAN_POINT('Ctrl Pts',(90.1635982543887,-38.1120961104195,113.786676793992));
#49733=CARTESIAN_POINT('Ctrl Pts',(87.6064735193736,-39.3210018168745,113.628728270799));
#49734=CARTESIAN_POINT('Ctrl Pts',(85.1963036669977,-37.8406568570009,113.470779747607));
#49735=CARTESIAN_POINT('Ctrl Pts',(85.1183164004075,-35.0132449832592,113.312831224414));
#49736=CARTESIAN_POINT('Ctrl Pts',(87.443220402345,-33.4022945497262,113.154882701222));
#49737=CARTESIAN_POINT('Ctrl Pts',(90.0630959230123,-34.4684053196434,112.996934178029));
#49738=CARTESIAN_POINT('Ctrl Pts',(90.6025815077325,-37.2449670822204,112.838985654837));
#49739=CARTESIAN_POINT('Ctrl Pts',(88.5725419845522,-39.2145557326372,112.681037131644));
#49740=CARTESIAN_POINT('Ctrl Pts',(85.8135524482776,-38.5914051438921,112.523088608452));
#49741=CARTESIAN_POINT('Ctrl Pts',(84.8271048005757,-35.9405070025316,112.365140085259));
#49742=CARTESIAN_POINT('Ctrl Pts',(86.5075811221681,-33.6653500299051,112.207191562067));
#49743=CARTESIAN_POINT('Ctrl Pts',(89.3313446416448,-33.8287498573211,112.049243038874));
#49744=CARTESIAN_POINT('Ctrl Pts',(90.7381748567804,-36.2825568308435,111.891294515682));
#49745=CARTESIAN_POINT('Ctrl Pts',(89.4525415983201,-38.8019787967437,111.73334599249));
#49746=CARTESIAN_POINT('Ctrl Pts',(86.6400894409389,-39.1027324832979,111.575397469297));
#49747=CARTESIAN_POINT('Ctrl Pts',(84.8507832188739,-36.9121336699122,111.417448946105));
#49748=CARTESIAN_POINT('Ctrl Pts',(85.706932464372,-34.2163316766427,111.259500422912));
#49749=CARTESIAN_POINT('Ctrl Pts',(88.432292695164,-33.4595281816538,111.10155189972));
#49750=CARTESIAN_POINT('Ctrl Pts',(90.5558626780312,-35.3278938967584,110.943603376527));
#49751=CARTESIAN_POINT('Ctrl Pts',(90.1522660950599,-38.1274384517549,110.785654853335));
#49752=CARTESIAN_POINT('Ctrl Pts',(87.587431693009,-39.3198999431135,110.627706330142));
#49753=CARTESIAN_POINT('Ctrl Pts',(85.1868168186886,-37.8241098033121,110.46975780695));
#49754=CARTESIAN_POINT('Ctrl Pts',(85.1269859664566,-34.9962554604981,110.311809283757));
#49755=CARTESIAN_POINT('Ctrl Pts',(87.4621859519783,-33.4002664403736,110.153860760565));
#49756=CARTESIAN_POINT('Ctrl Pts',(90.0751619669469,-34.4831774510166,109.995912237372));
#49757=CARTESIAN_POINT('Ctrl Pts',(90.5968081355154,-37.263146007451,109.83796371418));
#49758=CARTESIAN_POINT('Ctrl Pts',(88.5541637277013,-39.2196591826207,109.680015190987));
#49759=CARTESIAN_POINT('Ctrl Pts',(85.7992323328324,-38.5788059561733,109.522066667795));
#49760=CARTESIAN_POINT('Ctrl Pts',(84.8298263995735,-35.9216285176768,109.364118144602));
#49761=CARTESIAN_POINT('Ctrl Pts',(86.5248769270656,-33.6573087131898,109.20616962141));
#49762=CARTESIAN_POINT('Ctrl Pts',(89.3475329025042,-33.8388366962972,109.048221098218));
#49763=CARTESIAN_POINT('Ctrl Pts',(90.7385785187742,-36.3016260452323,108.890272575025));
#49764=CARTESIAN_POINT('Ctrl Pts',(89.4367939557108,-38.812741629989,108.732324051833));
#49765=CARTESIAN_POINT('Ctrl Pts',(86.6224698783981,-39.095429120668,108.57437552864));
#49766=CARTESIAN_POINT('Ctrl Pts',(84.8472638220703,-36.8933888944926,108.416427005448));
#49767=CARTESIAN_POINT('Ctrl Pts',(85.7207104071022,-34.2031345408651,108.258478482255));
#49768=CARTESIAN_POINT('Ctrl Pts',(88.4508630942718,-33.4638570130842,108.100529959063));
#49769=CARTESIAN_POINT('Ctrl Pts',(90.5624147285815,-35.3457973731139,107.94258143587));
#49770=CARTESIAN_POINT('Ctrl Pts',(90.140804932313,-38.1427385431604,107.784632912678));
#49771=CARTESIAN_POINT('Ctrl Pts',(87.5684605240929,-39.3186124160521,107.626684389485));
#49772=CARTESIAN_POINT('Ctrl Pts',(85.1773064515634,-37.8076325870251,107.468735866293));
#49773=CARTESIAN_POINT('Ctrl Pts',(85.1360317379698,-34.9790536882396,107.3107873431));
#49774=CARTESIAN_POINT('Ctrl Pts',(87.4806142131685,-33.3989116983333,107.152838819908));
#49775=CARTESIAN_POINT('Ctrl Pts',(90.0882639790973,-34.4968785995462,106.994890296715));
#49776=CARTESIAN_POINT('Ctrl Pts',(90.5885430574506,-37.283604361099,106.836941773523));
#49777=CARTESIAN_POINT('Ctrl Pts',(89.223305985034,-38.5719224173531,106.731642758061));
#49778=CARTESIAN_POINT('Ctrl Pts',(88.4187555865469,-38.7870128767187,106.678993250331));
#49779=CARTESIAN_POINT('Ctrl Pts',(89.8228871389145,-34.5985007534568,122.10700224989));
#49780=CARTESIAN_POINT('Ctrl Pts',(90.4039242511275,-35.2780872164357,122.054352742159));
#49781=CARTESIAN_POINT('Ctrl Pts',(90.8283659348487,-37.2482110053789,121.949053726697));
#49782=CARTESIAN_POINT('Ctrl Pts',(88.6910092443729,-39.4095836618517,121.791105203505));
#49783=CARTESIAN_POINT('Ctrl Pts',(85.7161175909924,-38.7952117689661,121.633156680312));
#49784=CARTESIAN_POINT('Ctrl Pts',(84.6026501316896,-35.9713098392101,121.47520815712));
#49785=CARTESIAN_POINT('Ctrl Pts',(86.3593458556655,-33.4937670123354,121.317259633928));
#49786=CARTESIAN_POINT('Ctrl Pts',(89.3938588908501,-33.6110570908767,121.159311110735));
#49787=CARTESIAN_POINT('Ctrl Pts',(90.9546957738743,-36.2157859918298,121.001362587543));
#49788=CARTESIAN_POINT('Ctrl Pts',(89.6267869226841,-38.946836103304,120.84341406435));
#49789=CARTESIAN_POINT('Ctrl Pts',(86.6140613242422,-39.3277989604213,120.685465541158));
#49790=CARTESIAN_POINT('Ctrl Pts',(84.6480878134429,-37.0133878981752,120.527517017965));
#49791=CARTESIAN_POINT('Ctrl Pts',(85.5113440042922,-34.1019503162447,120.369568494773));
#49792=CARTESIAN_POINT('Ctrl Pts',(88.4211470026898,-33.2332266737997,120.21161997158));
#49793=CARTESIAN_POINT('Ctrl Pts',(90.7392643801702,-35.1948483944551,120.053671448388));
#49794=CARTESIAN_POINT('Ctrl Pts',(90.3639308515484,-38.2082794737486,119.895722925195));
#49795=CARTESIAN_POINT('Ctrl Pts',(87.6354493097342,-39.5413303196711,119.737774402003));
#49796=CARTESIAN_POINT('Ctrl Pts',(85.0276512784935,-37.9853658687859,119.57982587881));
#49797=CARTESIAN_POINT('Ctrl Pts',(84.9049477777875,-34.9511309903593,119.421877355618));
#49798=CARTESIAN_POINT('Ctrl Pts',(87.378590409072,-33.1896745438001,119.263928832425));
#49799=CARTESIAN_POINT('Ctrl Pts',(90.2058025973435,-34.2980553335162,119.105980309233));
#49800=CARTESIAN_POINT('Ctrl Pts',(90.8232370536329,-37.2713382965273,118.948031786041));
#49801=CARTESIAN_POINT('Ctrl Pts',(88.6710847268857,-39.4137381552255,118.790083262848));
#49802=CARTESIAN_POINT('Ctrl Pts',(85.7006366808786,-38.7828061369573,118.632134739656));
#49803=CARTESIAN_POINT('Ctrl Pts',(84.605107814951,-35.9505891035064,118.474186216463));
#49804=CARTESIAN_POINT('Ctrl Pts',(86.3777808337504,-33.4849721060991,118.316237693271));
#49805=CARTESIAN_POINT('Ctrl Pts',(89.4114270240989,-33.6214550855102,118.158289170078));
#49806=CARTESIAN_POINT('Ctrl Pts',(90.9555316496024,-36.2362930764281,118.000340646886));
#49807=CARTESIAN_POINT('Ctrl Pts',(89.6101020080307,-38.9586919986172,117.842392123693));
#49808=CARTESIAN_POINT('Ctrl Pts',(86.5949982360553,-39.3203355476276,117.684443600501));
#49809=CARTESIAN_POINT('Ctrl Pts',(84.6439232234655,-36.9933325163275,117.526495077308));
#49810=CARTESIAN_POINT('Ctrl Pts',(85.5258573449243,-34.0875057806646,117.368546554116));
#49811=CARTESIAN_POINT('Ctrl Pts',(88.4411777553128,-33.2374800651071,117.210598030923));
#49812=CARTESIAN_POINT('Ctrl Pts',(90.7466521039974,-35.2139478336032,117.052649507731));
#49813=CARTESIAN_POINT('Ctrl Pts',(90.3519769168565,-38.2249058719997,116.894700984538));
#49814=CARTESIAN_POINT('Ctrl Pts',(87.6149921825685,-39.5404101010355,116.736752461346));
#49815=CARTESIAN_POINT('Ctrl Pts',(85.0172387180843,-37.9677328454945,116.578803938154));
#49816=CARTESIAN_POINT('Ctrl Pts',(84.9140205825513,-34.9327727421602,116.420855414961));
#49817=CARTESIAN_POINT('Ctrl Pts',(87.3989225202199,-33.1872358125861,116.262906891769));
#49818=CARTESIAN_POINT('Ctrl Pts',(90.2189595190818,-34.3137473027115,116.104958368576));
#49819=CARTESIAN_POINT('Ctrl Pts',(90.8172897998176,-37.2909335057378,115.947009845384));
#49820=CARTESIAN_POINT('Ctrl Pts',(88.6514254942766,-39.4194702384063,115.789061322191));
#49821=CARTESIAN_POINT('Ctrl Pts',(85.6850898965081,-38.7694779817249,115.631112798999));
#49822=CARTESIAN_POINT('Ctrl Pts',(84.6077692759893,-35.9302849462058,115.473164275806));
#49823=CARTESIAN_POINT('Ctrl Pts',(86.3962374741195,-33.4761011070012,115.315215752614));
#49824=CARTESIAN_POINT('Ctrl Pts',(89.428944769455,-33.6320603104907,115.157267229421));
#49825=CARTESIAN_POINT('Ctrl Pts',(90.9562276929385,-36.2567590901549,114.999318706229));
#49826=CARTESIAN_POINT('Ctrl Pts',(89.5933452680577,-38.9704628890774,114.841370183036));
#49827=CARTESIAN_POINT('Ctrl Pts',(86.5759815392568,-39.3127390063453,114.683421659844));
#49828=CARTESIAN_POINT('Ctrl Pts',(84.63988843047,-36.9732560962893,114.525473136651));
#49829=CARTESIAN_POINT('Ctrl Pts',(85.5404626798244,-34.0731521613009,114.367524613459));
#49830=CARTESIAN_POINT('Ctrl Pts',(88.4611810051576,-33.2418632365599,114.209576090266));
#49831=CARTESIAN_POINT('Ctrl Pts',(90.7539169305229,-35.2330937076193,114.051627567074));
#49832=CARTESIAN_POINT('Ctrl Pts',(90.3399165228022,-38.2414554669066,113.893679043881));
#49833=CARTESIAN_POINT('Ctrl Pts',(87.5945413604231,-39.5393584024631,113.735730520689));
#49834=CARTESIAN_POINT('Ctrl Pts',(85.0069396063031,-37.9500333965531,113.577781997497));
#49835=CARTESIAN_POINT('Ctrl Pts',(84.9232110725532,-34.9144730949001,113.419833474304));
#49836=CARTESIAN_POINT('Ctrl Pts',(87.4192698742361,-33.1849277006198,113.261884951112));
#49837=CARTESIAN_POINT('Ctrl Pts',(90.2320154100628,-34.3295234209606,113.103936427919));
#49838=CARTESIAN_POINT('Ctrl Pts',(90.8112168484876,-37.3104901275948,112.945987904727));
#49839=CARTESIAN_POINT('Ctrl Pts',(88.6317298609064,-39.4250759696213,112.788039381534));
#49840=CARTESIAN_POINT('Ctrl Pts',(85.6696290128585,-38.7560502762959,112.630090858342));
#49841=CARTESIAN_POINT('Ctrl Pts',(84.6105610550442,-35.90999829626,112.472142335149));
#49842=CARTESIAN_POINT('Ctrl Pts',(86.4147506947176,-33.4673488010541,112.314193811957));
#49843=CARTESIAN_POINT('Ctrl Pts',(89.4463940575345,-33.6427777981548,112.156245288764));
#49844=CARTESIAN_POINT('Ctrl Pts',(90.9567923096934,-36.2772291513235,111.998296765572));
#49845=CARTESIAN_POINT('Ctrl Pts',(89.5765132926491,-38.9821259418566,111.840348242379));
#49846=CARTESIAN_POINT('Ctrl Pts',(86.5570140118646,-39.3050205154978,111.682399719187));
#49847=CARTESIAN_POINT('Ctrl Pts',(84.635982631313,-36.9531541827155,111.524451195994));
#49848=CARTESIAN_POINT('Ctrl Pts',(85.5551598782013,-34.0588926186737,111.366502672802));
#49849=CARTESIAN_POINT('Ctrl Pts',(88.4811556983105,-33.2463747584794,111.208554149609));
#49850=CARTESIAN_POINT('Ctrl Pts',(90.7610586716412,-35.2522858344048,111.050605626417));
#49851=CARTESIAN_POINT('Ctrl Pts',(90.3277501124856,-38.2579272808382,110.892657103225));
#49852=CARTESIAN_POINT('Ctrl Pts',(87.5740977127464,-39.5381754109516,110.734708580032));
#49853=CARTESIAN_POINT('Ctrl Pts',(84.9967543551262,-37.9322681817453,110.57676005684));
#49854=CARTESIAN_POINT('Ctrl Pts',(84.9325188747787,-34.8962328373287,110.418811533647));
#49855=CARTESIAN_POINT('Ctrl Pts',(87.4396316298405,-33.182750285898,110.260863010455));
#49856=CARTESIAN_POINT('Ctrl Pts',(90.2449697321076,-34.3453830472088,110.102914487262));
#49857=CARTESIAN_POINT('Ctrl Pts',(90.8050184521126,-37.3300073490754,109.94496596407));
#49858=CARTESIAN_POINT('Ctrl Pts',(88.6119986334088,-39.4305551254228,109.787017440877));
#49859=CARTESIAN_POINT('Ctrl Pts',(85.65425467905,-38.7425235614839,109.629068917685));
#49860=CARTESIAN_POINT('Ctrl Pts',(84.6134830127371,-35.8897300149696,109.471120394492));
#49861=CARTESIAN_POINT('Ctrl Pts',(86.4333197823059,-33.4587154986263,109.3131718713));
#49862=CARTESIAN_POINT('Ctrl Pts',(89.4637740659,-33.6536072101161,109.155223348107));
#49863=CARTESIAN_POINT('Ctrl Pts',(90.9572256884785,-36.297702203276,108.997274824915));
#49864=CARTESIAN_POINT('Ctrl Pts',(89.5596063399716,-38.9936811134381,108.839326301722));
#49865=CARTESIAN_POINT('Ctrl Pts',(86.5380973322402,-39.2971794938646,108.68137777853));
#49866=CARTESIAN_POINT('Ctrl Pts',(84.6322041435302,-36.9330294542826,108.523429255337));
#49867=CARTESIAN_POINT('Ctrl Pts',(85.5699521256195,-34.0447239360583,108.365480732145));
#49868=CARTESIAN_POINT('Ctrl Pts',(88.5010932131953,-33.2510222698536,108.207532208953));
#49869=CARTESIAN_POINT('Ctrl Pts',(90.7680930710965,-35.2715073290129,108.04958368576));
#49870=CARTESIAN_POINT('Ctrl Pts',(90.3154452017761,-38.2743537344842,107.891635162568));
#49871=CARTESIAN_POINT('Ctrl Pts',(87.5537299241789,-39.5367930987136,107.733686639375));
#49872=CARTESIAN_POINT('Ctrl Pts',(84.9865438537246,-37.9145779456297,107.575738116183));
#49873=CARTESIAN_POINT('Ctrl Pts',(84.9422305779652,-34.8777647048748,107.41778959299));
#49874=CARTESIAN_POINT('Ctrl Pts',(87.4594165428971,-33.1812958104484,107.259841069798));
#49875=CARTESIAN_POINT('Ctrl Pts',(90.2590362882839,-34.3600928469906,107.101892546605));
#49876=CARTESIAN_POINT('Ctrl Pts',(90.7961449154706,-37.3519718059513,106.943944023413));
#49877=CARTESIAN_POINT('Ctrl Pts',(89.3304018103147,-38.7351332702527,106.838645007951));
#49878=CARTESIAN_POINT('Ctrl Pts',(88.4666220147327,-38.9660582606223,106.78599550022));
#49879=CARTESIAN_POINT('Ctrl Pts',(89.9637526925915,-34.478062635605,122.21400449978));
#49880=CARTESIAN_POINT('Ctrl Pts',(90.5846315306959,-35.204248355341,122.161354992049));
#49881=CARTESIAN_POINT('Ctrl Pts',(91.0381771887835,-37.3094635701525,122.056055976587));
#49882=CARTESIAN_POINT('Ctrl Pts',(88.7542619091845,-39.6190415909959,121.898107453395));
#49883=CARTESIAN_POINT('Ctrl Pts',(85.5753818782645,-38.962542205671,121.740158930202));
#49884=CARTESIAN_POINT('Ctrl Pts',(84.3855639339925,-35.9450052666105,121.58221040701));
#49885=CARTESIAN_POINT('Ctrl Pts',(86.262716317342,-33.297577280737,121.424261883817));
#49886=CARTESIAN_POINT('Ctrl Pts',(89.5053059693561,-33.4229099422059,121.266313360625));
#49887=CARTESIAN_POINT('Ctrl Pts',(91.1731694672859,-36.2062451536888,121.108364837432));
#49888=CARTESIAN_POINT('Ctrl Pts',(89.7542058807856,-39.1245634235127,120.95041631424));
#49889=CARTESIAN_POINT('Ctrl Pts',(86.5348976304681,-39.5316489110251,120.792467791048));
#49890=CARTESIAN_POINT('Ctrl Pts',(84.4341172784523,-37.058538637999,120.634519267855));
#49891=CARTESIAN_POINT('Ctrl Pts',(85.3565669628098,-33.9474637254213,120.476570744663));
#49892=CARTESIAN_POINT('Ctrl Pts',(88.4658952084306,-33.0191716862075,120.31862222147));
#49893=CARTESIAN_POINT('Ctrl Pts',(90.9429659387973,-35.1153018457461,120.160673698277));
#49894=CARTESIAN_POINT('Ctrl Pts',(90.5418957829432,-38.3353639517507,120.002725175085));
#49895=CARTESIAN_POINT('Ctrl Pts',(87.6263222096498,-39.7598221196604,119.844776651893));
#49896=CARTESIAN_POINT('Ctrl Pts',(84.8397074175569,-38.0971651566346,119.6868281287));
#49897=CARTESIAN_POINT('Ctrl Pts',(84.7085901354619,-34.8548727345926,119.528879605508));
#49898=CARTESIAN_POINT('Ctrl Pts',(87.3518504892593,-32.9726331858213,119.370931082315));
#49899=CARTESIAN_POINT('Ctrl Pts',(90.3729246713247,-34.1570156674757,119.212982559123));
#49900=CARTESIAN_POINT('Ctrl Pts',(91.0326966200846,-37.3341767000971,119.05503403593));
#49901=CARTESIAN_POINT('Ctrl Pts',(88.7329711671524,-39.6234809580597,118.897085512738));
#49902=CARTESIAN_POINT('Ctrl Pts',(85.5588394418481,-38.9492859192382,118.739136989545));
#49903=CARTESIAN_POINT('Ctrl Pts',(84.3881901406422,-35.9228637096635,118.581188466353));
#49904=CARTESIAN_POINT('Ctrl Pts',(86.2824153822265,-33.2881793076119,118.42323994316));
#49905=CARTESIAN_POINT('Ctrl Pts',(89.5240787498378,-33.4340209275303,118.265291419968));
#49906=CARTESIAN_POINT('Ctrl Pts',(91.1740626590286,-36.22815840947,118.107342896775));
#49907=CARTESIAN_POINT('Ctrl Pts',(89.7363768812154,-39.1372322777943,117.949394373583));
#49908=CARTESIAN_POINT('Ctrl Pts',(86.5145273859598,-39.5236737318734,117.791445850391));
#49909=CARTESIAN_POINT('Ctrl Pts',(84.4296671224604,-37.0371080582347,117.633497327198));
#49910=CARTESIAN_POINT('Ctrl Pts',(85.3720754834864,-33.9320287277603,117.475548804006));
#49911=CARTESIAN_POINT('Ctrl Pts',(88.487299470144,-33.0237167326382,117.317600280813));
#49912=CARTESIAN_POINT('Ctrl Pts',(90.9508602389886,-35.1357109338017,117.159651757621));
#49913=CARTESIAN_POINT('Ctrl Pts',(90.5291221667209,-38.3531304224478,117.001703234428));
#49914=CARTESIAN_POINT('Ctrl Pts',(87.6044623368834,-39.7588388016154,116.843754711236));
#49915=CARTESIAN_POINT('Ctrl Pts',(84.8285808676813,-38.0783230365991,116.685806188043));
#49916=CARTESIAN_POINT('Ctrl Pts',(84.718285062622,-34.8352556609635,116.527857664851));
#49917=CARTESIAN_POINT('Ctrl Pts',(87.3735767736571,-32.9700272307613,116.369909141658));
#49918=CARTESIAN_POINT('Ctrl Pts',(90.3869837634382,-34.1737836352987,116.211960618466));
#49919=CARTESIAN_POINT('Ctrl Pts',(91.0263415629614,-37.3551155531776,116.054012095273));
#49920=CARTESIAN_POINT('Ctrl Pts',(88.7119639005876,-39.6296060902939,115.896063572081));
#49921=CARTESIAN_POINT('Ctrl Pts',(85.5422266141761,-38.9350438521467,115.738115048888));
#49922=CARTESIAN_POINT('Ctrl Pts',(84.3910340981148,-35.9011672959088,115.580166525696));
#49923=CARTESIAN_POINT('Ctrl Pts',(86.3021375947785,-33.2787000239364,115.422218002504));
#49924=CARTESIAN_POINT('Ctrl Pts',(89.5427976873277,-33.4453533529904,115.264269479311));
#49925=CARTESIAN_POINT('Ctrl Pts',(91.1748064300696,-36.2500277781493,115.106320956119));
#49926=CARTESIAN_POINT('Ctrl Pts',(89.7184711312623,-39.1498102984383,114.948372432926));
#49927=CARTESIAN_POINT('Ctrl Pts',(86.4942067138983,-39.5155562956101,114.790423909734));
#49928=CARTESIAN_POINT('Ctrl Pts',(84.4253556636322,-37.0156549976906,114.632475386541));
#49929=CARTESIAN_POINT('Ctrl Pts',(85.3876823064798,-33.9166908804425,114.474526863349));
#49930=CARTESIAN_POINT('Ctrl Pts',(88.508674343213,-33.0284004582413,114.316578340156));
#49931=CARTESIAN_POINT('Ctrl Pts',(90.9586232148078,-35.156169640765,114.158629816964));
#49932=CARTESIAN_POINT('Ctrl Pts',(90.5162347912159,-38.3708148233938,114.000681293771));
#49933=CARTESIAN_POINT('Ctrl Pts',(87.5826092014724,-39.7577149880517,113.842732770579));
#49934=CARTESIAN_POINT('Ctrl Pts',(84.8175755456086,-38.0594099361054,113.684784247386));
#49935=CARTESIAN_POINT('Ctrl Pts',(84.7281057446989,-34.8157012065411,113.526835724194));
#49936=CARTESIAN_POINT('Ctrl Pts',(87.3953193461272,-32.9675608515133,113.368887201001));
#49937=CARTESIAN_POINT('Ctrl Pts',(90.4009348971133,-34.1906415222777,113.210938677809));
#49938=CARTESIAN_POINT('Ctrl Pts',(91.0198521892427,-37.3760131729692,113.052990154616));
#49939=CARTESIAN_POINT('Ctrl Pts',(88.6909177372605,-39.6355962066054,112.895041631424));
#49940=CARTESIAN_POINT('Ctrl Pts',(85.5257055774393,-38.9206954086998,112.737093108231));
#49941=CARTESIAN_POINT('Ctrl Pts',(84.3940173095128,-35.8794895899884,112.579144585039));
#49942=CARTESIAN_POINT('Ctrl Pts',(86.321920267267,-33.2693475722032,112.421196061847));
#49943=CARTESIAN_POINT('Ctrl Pts',(89.5614434734244,-33.4568057389885,112.263247538654));
#49944=CARTESIAN_POINT('Ctrl Pts',(91.1754097626062,-36.2719014718034,112.105299015462));
#49945=CARTESIAN_POINT('Ctrl Pts',(89.7004849869781,-39.1622730869696,111.947350492269));
#49946=CARTESIAN_POINT('Ctrl Pts',(86.4739385827902,-39.5073085476977,111.789401969077));
#49947=CARTESIAN_POINT('Ctrl Pts',(84.4211820437524,-36.9941746955189,111.631453445884));
#49948=CARTESIAN_POINT('Ctrl Pts',(85.4033872920303,-33.9014535607047,111.473504922692));
#49949=CARTESIAN_POINT('Ctrl Pts',(88.5300187014573,-33.0332213353051,111.315556399499));
#49950=CARTESIAN_POINT('Ctrl Pts',(90.9662546652511,-35.176677772051,111.157607876307));
#49951=CARTESIAN_POINT('Ctrl Pts',(90.5032341299113,-38.3884161099215,110.999659353114));
#49952=CARTESIAN_POINT('Ctrl Pts',(87.5607637324837,-39.7564508787897,110.841710829922));
#49953=CARTESIAN_POINT('Ctrl Pts',(84.8066918915637,-38.0404265601786,110.683762306729));
#49954=CARTESIAN_POINT('Ctrl Pts',(84.738051783101,-34.7962102141593,110.525813783537));
#49955=CARTESIAN_POINT('Ctrl Pts',(87.4170773077025,-32.9652341314225,110.367865260344));
#49956=CARTESIAN_POINT('Ctrl Pts',(90.4147774972684,-34.2075886434009,110.209916737152));
#49957=CARTESIAN_POINT('Ctrl Pts',(91.0132287687098,-37.3968686906999,110.051968213959));
#49958=CARTESIAN_POINT('Ctrl Pts',(88.6698335391163,-39.6414510682249,109.894019690767));
#49959=CARTESIAN_POINT('Ctrl Pts',(85.5092770252676,-38.9062411667946,109.736071167575));
#49960=CARTESIAN_POINT('Ctrl Pts',(84.3971396259005,-35.8578315122625,109.578122644382));
#49961=CARTESIAN_POINT('Ctrl Pts',(86.3417626375461,-33.2601222840629,109.42017412119));
#49962=CARTESIAN_POINT('Ctrl Pts',(89.5800152292957,-33.4683777239349,109.262225597997));
#49963=CARTESIAN_POINT('Ctrl Pts',(91.1758728581828,-36.2937783613198,109.104277074805));
#49964=CARTESIAN_POINT('Ctrl Pts',(89.6824187242323,-39.1746205968873,108.946328551612));
#49965=CARTESIAN_POINT('Ctrl Pts',(86.4537247860825,-39.4989298670612,108.78838002842));
#49966=CARTESIAN_POINT('Ctrl Pts',(84.41714446499,-36.9726700140725,108.630431505227));
#49967=CARTESIAN_POINT('Ctrl Pts',(85.4191938441369,-33.8863133312516,108.472482982035));
#49968=CARTESIAN_POINT('Ctrl Pts',(88.5513233321187,-33.038187526623,108.314534458842));
#49969=CARTESIAN_POINT('Ctrl Pts',(90.9737714136116,-35.1972172849119,108.15658593565));
#49970=CARTESIAN_POINT('Ctrl Pts',(90.4900854712392,-38.405968925808,107.998637412458));
#49971=CARTESIAN_POINT('Ctrl Pts',(87.5389993242649,-39.7549737813751,107.840688889265));
#49972=CARTESIAN_POINT('Ctrl Pts',(84.795781255886,-38.0215233042344,107.682740366073));
#49973=CARTESIAN_POINT('Ctrl Pts',(84.7484294179605,-34.77647572151,107.52479184288));
#49974=CARTESIAN_POINT('Ctrl Pts',(87.4382188726258,-32.9636799225635,107.366843319688));
#49975=CARTESIAN_POINT('Ctrl Pts',(90.4298085974705,-34.223307094435,107.208894796495));
#49976=CARTESIAN_POINT('Ctrl Pts',(91.0037467734906,-37.4203392508036,107.050946273303));
#49977=CARTESIAN_POINT('Ctrl Pts',(89.4374976355955,-38.8983441231523,106.945647257841));
#49978=CARTESIAN_POINT('Ctrl Pts',(88.5144884429186,-39.1451036445258,106.89299775011));
#49979=CARTESIAN_POINT('Ctrl Pts',(90.1046182462686,-34.3576245177531,122.321006749669));
#49980=CARTESIAN_POINT('Ctrl Pts',(90.7653388102644,-35.1304094942464,122.268357241939));
#49981=CARTESIAN_POINT('Ctrl Pts',(91.2479884427182,-37.3707161349261,122.163058226477));
#49982=CARTESIAN_POINT('Ctrl Pts',(88.8175145739961,-39.82849952014,122.005109703284));
#49983=CARTESIAN_POINT('Ctrl Pts',(85.4346461655366,-39.1298726423758,121.847161180092));
#49984=CARTESIAN_POINT('Ctrl Pts',(84.1684777362954,-35.918700694011,121.6892126569));
#49985=CARTESIAN_POINT('Ctrl Pts',(86.1660867790185,-33.1013875491387,121.531264133707));
#49986=CARTESIAN_POINT('Ctrl Pts',(89.6167530478622,-33.2347627935352,121.373315610515));
#49987=CARTESIAN_POINT('Ctrl Pts',(91.3916431606975,-36.1967043155478,121.215367087322));
#49988=CARTESIAN_POINT('Ctrl Pts',(89.8816248388871,-39.3022907437215,121.05741856413));
#49989=CARTESIAN_POINT('Ctrl Pts',(86.455733936694,-39.7354988616288,120.899470040937));
#49990=CARTESIAN_POINT('Ctrl Pts',(84.2201467434616,-37.1036893778229,120.741521517745));
#49991=CARTESIAN_POINT('Ctrl Pts',(85.2017899213274,-33.7929771345978,120.583572994552));
#49992=CARTESIAN_POINT('Ctrl Pts',(88.5106434141715,-32.8051166986153,120.42562447136));
#49993=CARTESIAN_POINT('Ctrl Pts',(91.1466674974244,-35.0357552970371,120.267675948167));
#49994=CARTESIAN_POINT('Ctrl Pts',(90.7198607143381,-38.4624484297529,120.109727424975));
#49995=CARTESIAN_POINT('Ctrl Pts',(87.6171951095654,-39.9783139196497,119.951778901782));
#49996=CARTESIAN_POINT('Ctrl Pts',(84.6517635566205,-38.2089644444833,119.79383037859));
#49997=CARTESIAN_POINT('Ctrl Pts',(84.5122324931363,-34.7586144788259,119.635881855397));
#49998=CARTESIAN_POINT('Ctrl Pts',(87.3251105694465,-32.7555918278425,119.477933332205));
#49999=CARTESIAN_POINT('Ctrl Pts',(90.540046745306,-34.0159760014353,119.319984809013));
#50000=CARTESIAN_POINT('Ctrl Pts',(91.2421561865363,-37.3970151036668,119.16203628582));
#50001=CARTESIAN_POINT('Ctrl Pts',(88.7948576074191,-39.8332237608939,119.004087762628));
#50002=CARTESIAN_POINT('Ctrl Pts',(85.4170422028178,-39.115765701519,118.846139239435));
#50003=CARTESIAN_POINT('Ctrl Pts',(84.1712724663333,-35.8951383158207,118.688190716243));
#50004=CARTESIAN_POINT('Ctrl Pts',(86.1870499307028,-33.0913865091248,118.53024219305));
#50005=CARTESIAN_POINT('Ctrl Pts',(89.6367304755765,-33.2465867695503,118.372293669858));
#50006=CARTESIAN_POINT('Ctrl Pts',(91.3925936684549,-36.2200237425119,118.214345146665));
#50007=CARTESIAN_POINT('Ctrl Pts',(89.8626517544002,-39.3157725569713,118.056396623473));
#50008=CARTESIAN_POINT('Ctrl Pts',(86.4340565358644,-39.7270119161192,117.89844810028));
#50009=CARTESIAN_POINT('Ctrl Pts',(84.2154110214554,-37.0808836001418,117.740499577088));
#50010=CARTESIAN_POINT('Ctrl Pts',(85.2182936220487,-33.776551674856,117.582551053895));
#50011=CARTESIAN_POINT('Ctrl Pts',(88.5334211849751,-32.8099534001692,117.424602530703));
#50012=CARTESIAN_POINT('Ctrl Pts',(91.1550683739797,-35.0574740340002,117.26665400751));
#50013=CARTESIAN_POINT('Ctrl Pts',(90.7062674165854,-38.4813549728958,117.108705484318));
#50014=CARTESIAN_POINT('Ctrl Pts',(87.5939324911983,-39.9772675021952,116.950756961125));
#50015=CARTESIAN_POINT('Ctrl Pts',(84.6399230172785,-38.1889132277036,116.792808437933));
#50016=CARTESIAN_POINT('Ctrl Pts',(84.5225495426926,-34.7377385797668,116.63485991474));
#50017=CARTESIAN_POINT('Ctrl Pts',(87.3482310270943,-32.7528186489366,116.476911391548));
#50018=CARTESIAN_POINT('Ctrl Pts',(90.5550080077946,-34.0338199678859,116.318962868355));
#50019=CARTESIAN_POINT('Ctrl Pts',(91.2353933261053,-37.4192976006176,116.161014345163));
#50020=CARTESIAN_POINT('Ctrl Pts',(88.7725023068986,-39.8397419421814,116.003065821971));
#50021=CARTESIAN_POINT('Ctrl Pts',(85.3993633318442,-39.1006097225685,115.845117298778));
#50022=CARTESIAN_POINT('Ctrl Pts',(84.1742989202403,-35.8720496456117,115.687168775586));
#50023=CARTESIAN_POINT('Ctrl Pts',(86.2080377154374,-33.0812989408716,115.529220252393));
#50024=CARTESIAN_POINT('Ctrl Pts',(89.6566506052006,-33.2586463954901,115.371271729201));
#50025=CARTESIAN_POINT('Ctrl Pts',(91.3933851672007,-36.2432964661436,115.213323206008));
#50026=CARTESIAN_POINT('Ctrl Pts',(89.8435969944667,-39.3291577077992,115.055374682816));
#50027=CARTESIAN_POINT('Ctrl Pts',(86.4124318885398,-39.718373584875,114.897426159624));
#50028=CARTESIAN_POINT('Ctrl Pts',(84.2108228967943,-37.058053899092,114.739477636431));
#50029=CARTESIAN_POINT('Ctrl Pts',(85.2349019331354,-33.760229599584,114.581529113239));
#50030=CARTESIAN_POINT('Ctrl Pts',(88.5561676812683,-32.8149376799226,114.423580590046));
#50031=CARTESIAN_POINT('Ctrl Pts',(91.1633294990928,-35.0792455739108,114.265632066854));
#50032=CARTESIAN_POINT('Ctrl Pts',(90.6925530596296,-38.5001741798809,114.107683543661));
#50033=CARTESIAN_POINT('Ctrl Pts',(87.5706770425218,-39.9760715736404,113.949735020469));
#50034=CARTESIAN_POINT('Ctrl Pts',(84.6282114849141,-38.1687864756576,113.791786497276));
#50035=CARTESIAN_POINT('Ctrl Pts',(84.5330004168447,-34.716929318182,113.633837974084));
#50036=CARTESIAN_POINT('Ctrl Pts',(87.3713688180184,-32.7501940024069,113.475889450891));
#50037=CARTESIAN_POINT('Ctrl Pts',(90.5698543841637,-34.0517596235948,113.317940927699));
#50038=CARTESIAN_POINT('Ctrl Pts',(91.2284875299979,-37.4415362183437,113.159992404506));
#50039=CARTESIAN_POINT('Ctrl Pts',(88.7501056136147,-39.8461164435895,113.002043881314));
#50040=CARTESIAN_POINT('Ctrl Pts',(85.38178214202,-39.0853405411036,112.844095358121));
#50041=CARTESIAN_POINT('Ctrl Pts',(84.1774735639814,-35.8489808837167,112.686146834929));
#50042=CARTESIAN_POINT('Ctrl Pts',(86.2290898398163,-33.0713463433522,112.528198311736));
#50043=CARTESIAN_POINT('Ctrl Pts',(89.6764928893144,-33.2708336798222,112.370249788544));
#50044=CARTESIAN_POINT('Ctrl Pts',(91.3940272155189,-36.2665737922834,112.212301265351));
#50045=CARTESIAN_POINT('Ctrl Pts',(89.8244566813072,-39.3424202320825,112.054352742159));
#50046=CARTESIAN_POINT('Ctrl Pts',(86.3908631537158,-39.7095965798975,111.896404218966));
#50047=CARTESIAN_POINT('Ctrl Pts',(84.2063814561917,-37.0351952083222,111.738455695774));
#50048=CARTESIAN_POINT('Ctrl Pts',(85.2516147058595,-33.7440145027357,111.580507172582));
#50049=CARTESIAN_POINT('Ctrl Pts',(88.5788817046039,-32.8200679121307,111.422558649389));
#50050=CARTESIAN_POINT('Ctrl Pts',(91.1714506588609,-35.1010697096973,111.264610126197));
#50051=CARTESIAN_POINT('Ctrl Pts',(90.6787181473369,-38.5189049390048,111.106661603004));
#50052=CARTESIAN_POINT('Ctrl Pts',(87.5474297522212,-39.9747263466277,110.948713079812));
#50053=CARTESIAN_POINT('Ctrl Pts',(84.6166294280013,-38.1485849386119,110.790764556619));
#50054=CARTESIAN_POINT('Ctrl Pts',(84.5435846914231,-34.6961875909898,110.632816033427));
#50055=CARTESIAN_POINT('Ctrl Pts',(87.3945229855647,-32.747717976947,110.474867510234));
#50056=CARTESIAN_POINT('Ctrl Pts',(90.584585262429,-34.069794239593,110.316918987042));
#50057=CARTESIAN_POINT('Ctrl Pts',(91.221439085307,-37.4637300323244,110.158970463849));
#50058=CARTESIAN_POINT('Ctrl Pts',(88.7276684448237,-39.8523470110271,110.001021940657));
#50059=CARTESIAN_POINT('Ctrl Pts',(85.3642993714853,-39.0699587721052,109.843073417464));
#50060=CARTESIAN_POINT('Ctrl Pts',(84.1807962390639,-35.8259330095553,109.685124894272));
#50061=CARTESIAN_POINT('Ctrl Pts',(86.2502054927865,-33.0615290694994,109.527176371079));
#50062=CARTESIAN_POINT('Ctrl Pts',(89.6962563926914,-33.2831482377538,109.369227847887));
#50063=CARTESIAN_POINT('Ctrl Pts',(91.3945200278872,-36.2898545193635,109.211279324695));
#50064=CARTESIAN_POINT('Ctrl Pts',(89.805231108493,-39.3555600803365,109.053330801502));
#50065=CARTESIAN_POINT('Ctrl Pts',(86.3693522399246,-39.7006802402578,108.89538227831));
#50066=CARTESIAN_POINT('Ctrl Pts',(84.2020847864498,-37.0123105738625,108.737433755117));
#50067=CARTESIAN_POINT('Ctrl Pts',(85.2684355626542,-33.7279027264448,108.579485231925));
#50068=CARTESIAN_POINT('Ctrl Pts',(88.6015534510421,-32.8253527833924,108.421536708732));
#50069=CARTESIAN_POINT('Ctrl Pts',(91.1794497561267,-35.1229272408109,108.26358818554));
#50070=CARTESIAN_POINT('Ctrl Pts',(90.6647257407023,-38.5375841171318,108.105639662347));
#50071=CARTESIAN_POINT('Ctrl Pts',(87.5242687243508,-39.9731544640366,107.947691139155));
#50072=CARTESIAN_POINT('Ctrl Pts',(84.6050186580472,-38.1284686628391,107.789742615962));
#50073=CARTESIAN_POINT('Ctrl Pts',(84.5546282579559,-34.6751867381451,107.63179409277));
#50074=CARTESIAN_POINT('Ctrl Pts',(87.4170212023543,-32.7460640346786,107.473845569577));
#50075=CARTESIAN_POINT('Ctrl Pts',(90.6005809066571,-34.0865213418793,107.315897046385));
#50076=CARTESIAN_POINT('Ctrl Pts',(91.2113486315107,-37.4887066956559,107.157948523193));
#50077=CARTESIAN_POINT('Ctrl Pts',(89.5445934608762,-39.0615549760519,107.052649507731));
#50078=CARTESIAN_POINT('Ctrl Pts',(88.5623548711045,-39.3241490284294,107.));
#50079=CARTESIAN_POINT('Ctrl Pts',(89.6820215852375,-34.7189388713087,122.));
#50080=CARTESIAN_POINT('Ctrl Pts',(89.7436297646655,-34.7768354319368,122.));
#50081=CARTESIAN_POINT('Ctrl Pts',(89.8018687896484,-34.8378827535703,122.));
#50082=CARTESIAN_POINT('Ctrl Pts',(89.8567410473575,-34.9016960170172,122.));
#50083=CARTESIAN_POINT('Ctrl Pts',(89.9130662359688,-34.9671989551066,122.));
#50084=CARTESIAN_POINT('Ctrl Pts',(89.9658444403112,-35.0356166815112,122.));
#50085=CARTESIAN_POINT('Ctrl Pts',(90.0150527344221,-35.1065815431353,122.));
#50086=CARTESIAN_POINT('Ctrl Pts',(90.0656106252208,-35.1794927014953,122.));
#50087=CARTESIAN_POINT('Ctrl Pts',(90.1124006349142,-35.2550931839603,122.));
#50088=CARTESIAN_POINT('Ctrl Pts',(90.1553638311491,-35.3330272291937,122.));
#50089=CARTESIAN_POINT('Ctrl Pts',(90.1742738139209,-35.3673294129661,122.));
#50090=CARTESIAN_POINT('Ctrl Pts',(90.1924419568553,-35.4020841678299,122.));
#50091=CARTESIAN_POINT('Ctrl Pts',(90.2098608098524,-35.4372632361576,122.));
#50092=CARTESIAN_POINT('Ctrl Pts',(90.2197916550143,-35.4573195441454,122.));
#50093=CARTESIAN_POINT('Ctrl Pts',(90.2294789245804,-35.4775137906346,122.));
#50094=CARTESIAN_POINT('Ctrl Pts',(90.2389210036363,-35.4978408875546,122.));
#50095=CARTESIAN_POINT('Ctrl Pts',(90.2474265875847,-35.516151879049,122.));
#50096=CARTESIAN_POINT('Ctrl Pts',(90.2557355810474,-35.5345764026367,122.));
#50097=CARTESIAN_POINT('Ctrl Pts',(90.2638331430362,-35.5530789842928,122.));
#50098=CARTESIAN_POINT('Ctrl Pts',(90.3003947448764,-35.6366206755408,122.));
#50099=CARTESIAN_POINT('Ctrl Pts',(90.332696167958,-35.721845910373,122.));
#50100=CARTESIAN_POINT('Ctrl Pts',(90.3607123776603,-35.8083559104926,122.));
#50101=CARTESIAN_POINT('Ctrl Pts',(90.3891916851232,-35.8962958894621,122.));
#50102=CARTESIAN_POINT('Ctrl Pts',(90.4132434356667,-35.9855642131905,122.));
#50103=CARTESIAN_POINT('Ctrl Pts',(90.4328022575856,-36.0757791241328,122.));
#50104=CARTESIAN_POINT('Ctrl Pts',(90.4517707201329,-36.1632710071569,122.));
#50105=CARTESIAN_POINT('Ctrl Pts',(90.4665135445043,-36.2516541139452,122.));
#50106=CARTESIAN_POINT('Ctrl Pts',(90.4769303589594,-36.3406020879646,122.));
#50107=CARTESIAN_POINT('Ctrl Pts',(90.4812991889115,-36.3779070217092,122.));
#50108=CARTESIAN_POINT('Ctrl Pts',(90.4849065674636,-36.4153115064826,122.));
#50109=CARTESIAN_POINT('Ctrl Pts',(90.4877427551487,-36.45279208454,122.));
#50110=CARTESIAN_POINT('Ctrl Pts',(90.4895218789421,-36.4763034299149,122.));
#50111=CARTESIAN_POINT('Ctrl Pts',(90.4909975124888,-36.4998447233063,122.));
#50112=CARTESIAN_POINT('Ctrl Pts',(90.4921669557079,-36.5234102073052,122.));
#50113=CARTESIAN_POINT('Ctrl Pts',(90.4928513370157,-36.5372011947559,122.));
#50114=CARTESIAN_POINT('Ctrl Pts',(90.4934305636957,-36.550995520558,122.));
#50115=CARTESIAN_POINT('Ctrl Pts',(90.4939041349555,-36.5647841938125,122.));
#50116=CARTESIAN_POINT('Ctrl Pts',(90.4972315041031,-36.6616650855928,122.));
#50117=CARTESIAN_POINT('Ctrl Pts',(90.4953529603836,-36.7583809703611,122.));
#50118=CARTESIAN_POINT('Ctrl Pts',(90.4882041230073,-36.854512080775,122.));
#50119=CARTESIAN_POINT('Ctrl Pts',(90.481055285631,-36.9506431911888,122.));
#50120=CARTESIAN_POINT('Ctrl Pts',(90.4686365849094,-37.0461905712847,122.));
#50121=CARTESIAN_POINT('Ctrl Pts',(90.4508311771209,-37.1407532391955,122.));
#50122=CARTESIAN_POINT('Ctrl Pts',(90.4337731476271,-37.2313466587568,122.));
#50123=CARTESIAN_POINT('Ctrl Pts',(90.4117712643279,-37.3210372661022,122.));
#50124=CARTESIAN_POINT('Ctrl Pts',(90.3851001359725,-37.4095857222218,122.));
#50125=CARTESIAN_POINT('Ctrl Pts',(90.3762307867704,-37.4390320646551,122.));
#50126=CARTESIAN_POINT('Ctrl Pts',(90.3668446531488,-37.4683520650043,122.));
#50127=CARTESIAN_POINT('Ctrl Pts',(90.3569505851863,-37.4975367471472,122.));
#50128=CARTESIAN_POINT('Ctrl Pts',(90.3476302477942,-37.5250290875361,122.));
#50129=CARTESIAN_POINT('Ctrl Pts',(90.3378591694355,-37.5524013492222,122.));
#50130=CARTESIAN_POINT('Ctrl Pts',(90.327644273459,-37.5796459038865,122.));
#50131=CARTESIAN_POINT('Ctrl Pts',(90.32248652871,-37.5934023297063,122.));
#50132=CARTESIAN_POINT('Ctrl Pts',(90.3172187072603,-37.6071179222931,122.));
#50133=CARTESIAN_POINT('Ctrl Pts',(90.3118434787871,-37.6207883639188,122.));
#50134=CARTESIAN_POINT('Ctrl Pts',(90.2775921562166,-37.7078973506603,122.));
#50135=CARTESIAN_POINT('Ctrl Pts',(90.2389673349269,-37.7932175192191,122.));
#50136=CARTESIAN_POINT('Ctrl Pts',(90.1962990002629,-37.8765144552663,122.));
#50137=CARTESIAN_POINT('Ctrl Pts',(90.1520692008913,-37.9628596758764,122.));
#50138=CARTESIAN_POINT('Ctrl Pts',(90.1034943952308,-38.0470316029905,122.));
#50139=CARTESIAN_POINT('Ctrl Pts',(90.0508862935642,-38.1287656580968,122.));
#50140=CARTESIAN_POINT('Ctrl Pts',(89.9977152427445,-38.2113743335685,122.));
#50141=CARTESIAN_POINT('Ctrl Pts',(89.9404236999765,-38.2914935051329,122.));
#50142=CARTESIAN_POINT('Ctrl Pts',(89.8792819816606,-38.3688346448537,122.));
#50143=CARTESIAN_POINT('Ctrl Pts',(89.8565930994489,-38.3975349178845,122.));
#50144=CARTESIAN_POINT('Ctrl Pts',(89.8333735538416,-38.4258524269221,122.));
#50145=CARTESIAN_POINT('Ctrl Pts',(89.8096355637098,-38.4537715398041,122.));
#50146=CARTESIAN_POINT('Ctrl Pts',(89.7888801267933,-38.4781827634574,122.));
#50147=CARTESIAN_POINT('Ctrl Pts',(89.7677283264474,-38.502289408991,122.));
#50148=CARTESIAN_POINT('Ctrl Pts',(89.7461878405604,-38.5260806443712,122.));
#50149=CARTESIAN_POINT('Ctrl Pts',(89.7344246098016,-38.5390730064415,122.));
#50150=CARTESIAN_POINT('Ctrl Pts',(89.7225501398425,-38.5519660547785,122.));
#50151=CARTESIAN_POINT('Ctrl Pts',(89.7105717549045,-38.5647521680861,122.));
#50152=CARTESIAN_POINT('Ctrl Pts',(89.6415609858971,-38.638416482311,122.));
#50153=CARTESIAN_POINT('Ctrl Pts',(89.5690478192282,-38.7085962647208,122.));
#50154=CARTESIAN_POINT('Ctrl Pts',(89.4933407755827,-38.7750003014946,122.));
#50155=CARTESIAN_POINT('Ctrl Pts',(89.4311466614727,-38.8295518998876,122.));
#50156=CARTESIAN_POINT('Ctrl Pts',(89.3667959749386,-38.8815552652603,122.));
#50157=CARTESIAN_POINT('Ctrl Pts',(89.300437483061,-38.9308356080291,122.));
#50158=CARTESIAN_POINT('Ctrl Pts',(89.2758198860226,-38.9491175729423,122.));
#50159=CARTESIAN_POINT('Ctrl Pts',(89.2509257832841,-38.9670246354587,122.));
#50160=CARTESIAN_POINT('Ctrl Pts',(89.2257621633589,-38.9845473066697,122.));
#50161=CARTESIAN_POINT('Ctrl Pts',(89.2089513436832,-38.9962535105799,122.));
#50162=CARTESIAN_POINT('Ctrl Pts',(89.1920191005935,-39.0077887888468,122.));
#50163=CARTESIAN_POINT('Ctrl Pts',(89.1749825783546,-39.0191404890314,122.));
#50164=CARTESIAN_POINT('Ctrl Pts',(89.0900721174774,-39.0757176519581,122.));
#50165=CARTESIAN_POINT('Ctrl Pts',(89.0024923773335,-39.127795516944,122.));
#50166=CARTESIAN_POINT('Ctrl Pts',(88.9125337151644,-39.1750661685274,122.));
#50167=CARTESIAN_POINT('Ctrl Pts',(88.8290756762026,-39.2189209323319,122.));
#50168=CARTESIAN_POINT('Ctrl Pts',(88.7435692936185,-39.2586384125487,122.));
#50169=CARTESIAN_POINT('Ctrl Pts',(88.6562187078536,-39.2939436847022,122.));
#50170=CARTESIAN_POINT('Ctrl Pts',(88.6257885343039,-39.3062429217301,122.));
#50171=CARTESIAN_POINT('Ctrl Pts',(88.5951343400001,-39.3180064003196,122.));
#50172=CARTESIAN_POINT('Ctrl Pts',(88.5642690312354,-39.3292378429292,122.));
#50173=CARTESIAN_POINT('Ctrl Pts',(85.2503884478834,-36.3571243043025,120.387416697508));
#50174=CARTESIAN_POINT('Ctrl Pts',(85.2488060880821,-36.5314907329699,120.398449387697));
#50175=CARTESIAN_POINT('Ctrl Pts',(85.2653916827167,-36.7055581163151,120.409482077886));
#50176=CARTESIAN_POINT('Ctrl Pts',(85.3012632429209,-36.8755557583819,120.420514768075));
#50177=CARTESIAN_POINT('Ctrl Pts',(85.4724472382946,-37.6868077755068,120.473164275806));
#50178=CARTESIAN_POINT('Ctrl Pts',(86.0828361281554,-38.4053783926622,120.525813783537));
#50179=CARTESIAN_POINT('Ctrl Pts',(86.8557210641803,-38.7055236634528,120.578463291268));
#50180=CARTESIAN_POINT('Ctrl Pts',(87.6286060002051,-39.0056689342435,120.631112798999));
#50181=CARTESIAN_POINT('Ctrl Pts',(88.5639869823939,-38.8873888586693,120.683762306729));
#50182=CARTESIAN_POINT('Ctrl Pts',(89.2378198261349,-38.4042851620282,120.73641181446));
#50183=CARTESIAN_POINT('Ctrl Pts',(89.911652669876,-37.9211814653871,120.789061322191));
#50184=CARTESIAN_POINT('Ctrl Pts',(90.3239373751694,-37.073254147679,120.841710829922));
#50185=CARTESIAN_POINT('Ctrl Pts',(90.2877780164629,-36.2449367237544,120.894360337653));
#50186=CARTESIAN_POINT('Ctrl Pts',(90.2516186577565,-35.4166192998297,120.947009845384));
#50187=CARTESIAN_POINT('Ctrl Pts',(89.7670152350502,-34.6079117696885,120.999659353114));
#50188=CARTESIAN_POINT('Ctrl Pts',(89.0536407873046,-34.1853500886824,121.052308860845));
#50189=CARTESIAN_POINT('Ctrl Pts',(88.340266339559,-33.7627884076762,121.104958368576));
#50190=CARTESIAN_POINT('Ctrl Pts',(87.398120866774,-33.726372575805,121.157607876307));
#50191=CARTESIAN_POINT('Ctrl Pts',(86.6543416196145,-34.092774271182,121.210257384038));
#50192=CARTESIAN_POINT('Ctrl Pts',(85.9105623724549,-34.4591759665591,121.262906891768));
#50193=CARTESIAN_POINT('Ctrl Pts',(85.3651493509208,-35.2283951891843,121.315556399499));
#50194=CARTESIAN_POINT('Ctrl Pts',(85.2652956692094,-36.0513826205722,121.36820590723));
#50195=CARTESIAN_POINT('Ctrl Pts',(85.2531507747902,-36.1514800360225,121.374609503989));
#50196=CARTESIAN_POINT('Ctrl Pts',(85.2475970862054,-36.2523728501989,121.381013100749));
#50197=CARTESIAN_POINT('Ctrl Pts',(85.2483528516199,-36.3533471753035,121.387416697508));
#50198=CARTESIAN_POINT('Ctrl Pts',(86.9747563060389,-39.3241490284291,122.));
#50199=CARTESIAN_POINT('Ctrl Pts',(85.9925177162673,-39.0615549760513,121.947350492269));
#50200=CARTESIAN_POINT('Ctrl Pts',(84.3257618514341,-37.4887114986967,121.842051476808));
#50201=CARTESIAN_POINT('Ctrl Pts',(84.9365308695941,-34.0865200954889,121.684102953615));
#50202=CARTESIAN_POINT('Ctrl Pts',(88.1200899288066,-32.7460654788916,121.526154430423));
#50203=CARTESIAN_POINT('Ctrl Pts',(90.9824824119093,-34.6751864614649,121.36820590723));
#50204=CARTESIAN_POINT('Ctrl Pts',(90.9320921383769,-38.128468693812,121.210257384038));
#50205=CARTESIAN_POINT('Ctrl Pts',(88.0128423765734,-39.9731538131696,121.052308860845));
#50206=CARTESIAN_POINT('Ctrl Pts',(84.8723858657462,-38.5375838933282,120.894360337653));
#50207=CARTESIAN_POINT('Ctrl Pts',(84.3576618778048,-35.1229273700108,120.73641181446));
#50208=CARTESIAN_POINT('Ctrl Pts',(86.935557851387,-32.8253532951761,120.578463291268));
#50209=CARTESIAN_POINT('Ctrl Pts',(90.2686752620247,-33.7279030795955,120.420514768075));
#50210=CARTESIAN_POINT('Ctrl Pts',(91.3350258987628,-37.0123104885738,120.262566244883));
#50211=CARTESIAN_POINT('Ctrl Pts',(89.167758741363,-39.7006797728369,120.10461772169));
#50212=CARTESIAN_POINT('Ctrl Pts',(85.7318803522126,-39.3555596654746,119.946669198498));
#50213=CARTESIAN_POINT('Ctrl Pts',(84.1425916520107,-36.2898545275783,119.788720675305));
#50214=CARTESIAN_POINT('Ctrl Pts',(85.8408550522478,-33.2831486644916,119.630772152113));
#50215=CARTESIAN_POINT('Ctrl Pts',(89.2869054734986,-33.0615295263651,119.472823628921));
#50216=CARTESIAN_POINT('Ctrl Pts',(91.3563144402191,-35.8259330830824,119.314875105728));
#50217=CARTESIAN_POINT('Ctrl Pts',(90.1728114719436,-39.0699583952412,119.156926582536));
#50218=CARTESIAN_POINT('Ctrl Pts',(86.8094428654503,-39.8523465256606,118.998978059343));
#50219=CARTESIAN_POINT('Ctrl Pts',(84.3156725710403,-37.4637298784219,118.841029536151));
#50220=CARTESIAN_POINT('Ctrl Pts',(84.9525263055479,-34.0697945567443,118.683081012958));
#50221=CARTESIAN_POINT('Ctrl Pts',(88.1425881396678,-32.7477184775748,118.525132489766));
#50222=CARTESIAN_POINT('Ctrl Pts',(90.9935260381413,-34.6961878212031,118.367183966573));
#50223=CARTESIAN_POINT('Ctrl Pts',(90.9204813116975,-38.1485846896768,118.209235443381));
#50224=CARTESIAN_POINT('Ctrl Pts',(87.9896813942331,-39.9747258442494,118.051286920188));
#50225=CARTESIAN_POINT('Ctrl Pts',(84.8583934336975,-38.5189046386728,117.893338396996));
#50226=CARTESIAN_POINT('Ctrl Pts',(84.3656609905594,-35.1010698837144,117.735389873803));
#50227=CARTESIAN_POINT('Ctrl Pts',(86.9582295850041,-32.8200684027204,117.577441350611));
#50228=CARTESIAN_POINT('Ctrl Pts',(90.2854961219689,-33.7440148650956,117.419492827418));
#50229=CARTESIAN_POINT('Ctrl Pts',(91.3307292265714,-37.0351951139114,117.261544304226));
#50230=CARTESIAN_POINT('Ctrl Pts',(89.1462478322224,-39.7095961143156,117.103595781033));
#50231=CARTESIAN_POINT('Ctrl Pts',(85.7126547811673,-39.3424198174583,116.945647257841));
#50232=CARTESIAN_POINT('Ctrl Pts',(84.1430844647916,-36.2665738045441,116.787698734649));
#50233=CARTESIAN_POINT('Ctrl Pts',(85.860618552627,-33.2708341078515,116.629750211456));
#50234=CARTESIAN_POINT('Ctrl Pts',(89.3080211236725,-33.0713467990688,116.471801688264));
#50235=CARTESIAN_POINT('Ctrl Pts',(91.3596371147702,-35.8489809539364,116.313853165071));
#50236=CARTESIAN_POINT('Ctrl Pts',(90.1553287038718,-39.0853401621602,116.155904641879));
#50237=CARTESIAN_POINT('Ctrl Pts',(86.7870056997543,-39.8461159590596,115.997956118686));
#50238=CARTESIAN_POINT('Ctrl Pts',(84.3086241273375,-37.4415360675358,115.840007595494));
#50239=CARTESIAN_POINT('Ctrl Pts',(84.9672571817637,-34.0517599432419,115.682059072301));
#50240=CARTESIAN_POINT('Ctrl Pts',(88.1657423040033,-32.7501945026947,115.524110549109));
#50241=CARTESIAN_POINT('Ctrl Pts',(91.0041103112496,-34.7169295455148,115.366162025916));
#50242=CARTESIAN_POINT('Ctrl Pts',(90.9088992563929,-38.1687862239197,115.208213502724));
#50243=CARTESIAN_POINT('Ctrl Pts',(87.9664341071585,-39.9760710710749,115.050264979531));
#50244=CARTESIAN_POINT('Ctrl Pts',(84.8445585233251,-38.5001738821487,114.892316456339));
#50245=CARTESIAN_POINT('Ctrl Pts',(84.3737821492005,-35.0792457509566,114.734367933146));
#50246=CARTESIAN_POINT('Ctrl Pts',(86.9809436051873,-32.8149381712244,114.576419409954));
#50247=CARTESIAN_POINT('Ctrl Pts',(90.3022088923736,-33.7602299596934,114.418470886762));
#50248=CARTESIAN_POINT('Ctrl Pts',(91.3262877865851,-37.0580538015087,114.260522363569));
#50249=CARTESIAN_POINT('Ctrl Pts',(89.124679100392,-39.7183731180749,114.102573840377));
#50250=CARTESIAN_POINT('Ctrl Pts',(85.6935144706641,-39.3291572950157,113.944625317184));
#50251=CARTESIAN_POINT('Ctrl Pts',(84.1437265130207,-36.2432964816349,113.786676793992));
#50252=CARTESIAN_POINT('Ctrl Pts',(85.8804608339871,-33.2586468252107,113.628728270799));
#50253=CARTESIAN_POINT('Ctrl Pts',(89.3290732451296,-33.0812993952069,113.470779747607));
#50254=CARTESIAN_POINT('Ctrl Pts',(91.3628117580707,-35.8720497126298,113.312831224414));
#50255=CARTESIAN_POINT('Ctrl Pts',(90.1377475164876,-39.100609341506,113.154882701222));
#50256=CARTESIAN_POINT('Ctrl Pts',(86.7646090095788,-39.8397414585361,112.996934178029));
#50257=CARTESIAN_POINT('Ctrl Pts',(84.3017183321886,-37.419297452896,112.838985654837));
#50258=CARTESIAN_POINT('Ctrl Pts',(84.9821035560724,-34.0338202900228,112.681037131644));
#50259=CARTESIAN_POINT('Ctrl Pts',(88.1888800917162,-32.7528191488601,112.523088608452));
#50260=CARTESIAN_POINT('Ctrl Pts',(91.0145611839512,-34.7377388042116,112.365140085259));
#50261=CARTESIAN_POINT('Ctrl Pts',(90.8971877256538,-38.1889129731724,112.207191562067));
#50262=CARTESIAN_POINT('Ctrl Pts',(87.9431786617096,-39.9772669994637,112.049243038874));
#50263=CARTESIAN_POINT('Ctrl Pts',(84.8308441682727,-38.4813546777754,111.891294515682));
#50264=CARTESIAN_POINT('Ctrl Pts',(84.382043273167,-35.0574742140675,111.733345992489));
#50265=CARTESIAN_POINT('Ctrl Pts',(87.0036900983236,-32.8099538921628,111.575397469297));
#50266=CARTESIAN_POINT('Ctrl Pts',(90.3188172011552,-33.7765520327001,111.417448946105));
#50267=CARTESIAN_POINT('Ctrl Pts',(91.3216996625609,-37.0808834993901,111.259500422912));
#50268=CARTESIAN_POINT('Ctrl Pts',(89.1030544560686,-39.7270114481203,111.10155189972));
#50269=CARTESIAN_POINT('Ctrl Pts',(85.6744597133751,-39.3157721460453,110.943603376527));
#50270=CARTESIAN_POINT('Ctrl Pts',(84.1445180116567,-36.2200237612334,110.785654853335));
#50271=CARTESIAN_POINT('Ctrl Pts',(85.9003809608462,-33.2465872009442,110.627706330142));
#50272=CARTESIAN_POINT('Ctrl Pts',(89.3500610269517,-33.0913869620613,110.46975780695));
#50273=CARTESIAN_POINT('Ctrl Pts',(91.3658382115574,-35.895138379632,110.311809283757));
#50274=CARTESIAN_POINT('Ctrl Pts',(90.1200686479678,-39.1157653183575,110.153860760565));
#50275=CARTESIAN_POINT('Ctrl Pts',(86.7422537121608,-39.8332232781445,109.995912237372));
#50276=CARTESIAN_POINT('Ctrl Pts',(84.2949554726962,-37.397014959055,109.83796371418));
#50277=CARTESIAN_POINT('Ctrl Pts',(84.9970648164843,-34.0159763260146,109.680015190987));
#50278=CARTESIAN_POINT('Ctrl Pts',(88.2120005461565,-32.7555923274475,109.522066667795));
#50279=CARTESIAN_POINT('Ctrl Pts',(91.0248782320717,-34.7586147002439,109.364118144602));
#50280=CARTESIAN_POINT('Ctrl Pts',(90.8853471879654,-38.2089641874212,109.20616962141));
#50281=CARTESIAN_POINT('Ctrl Pts',(87.9199160465446,-39.9783134162844,109.048221098218));
#50282=CARTESIAN_POINT('Ctrl Pts',(84.8172508724717,-38.4624481382004,108.890272575025));
#50283=CARTESIAN_POINT('Ctrl Pts',(84.3904441483993,-35.0357554783023,108.732324051833));
#50284=CARTESIAN_POINT('Ctrl Pts',(87.0264678663363,-32.8051171947587,108.57437552864));
#50285=CARTESIAN_POINT('Ctrl Pts',(90.3353208987278,-33.792977483537,108.416427005448));
#50286=CARTESIAN_POINT('Ctrl Pts',(91.3169639431757,-37.1036892864445,108.258478482255));
#50287=CARTESIAN_POINT('Ctrl Pts',(89.0813770537997,-39.7354983689013,108.100529959063));
#50288=CARTESIAN_POINT('Ctrl Pts',(85.6554866415101,-39.302290378503,107.94258143587));
#50289=CARTESIAN_POINT('Ctrl Pts',(84.1454684970089,-36.1967042568066,107.784632912678));
#50290=CARTESIAN_POINT('Ctrl Pts',(85.9203584351496,-33.2347633730889,107.626684389485));
#50291=CARTESIAN_POINT('Ctrl Pts',(89.3710240668315,-33.1013877392709,107.468735866293));
#50292=CARTESIAN_POINT('Ctrl Pts',(91.3686331795228,-35.9187012093704,107.3107873431));
#50293=CARTESIAN_POINT('Ctrl Pts',(90.1024641556487,-39.1298714782457,107.152838819908));
#50294=CARTESIAN_POINT('Ctrl Pts',(86.7195978028781,-39.8285002079331,106.994890296716));
#50295=CARTESIAN_POINT('Ctrl Pts',(84.2891194416926,-37.3707125699518,106.836941773523));
#50296=CARTESIAN_POINT('Ctrl Pts',(84.7717723668806,-35.1304094942453,106.731642758061));
#50297=CARTESIAN_POINT('Ctrl Pts',(85.4324929308767,-34.3576245177522,106.678993250331));
#50298=CARTESIAN_POINT('Ctrl Pts',(87.0226227342249,-39.1451036445255,122.10700224989));
#50299=CARTESIAN_POINT('Ctrl Pts',(86.0996135415481,-38.8983441231517,122.054352742159));
#50300=CARTESIAN_POINT('Ctrl Pts',(84.5333637513147,-37.4203437642191,121.949053726697));
#50301=CARTESIAN_POINT('Ctrl Pts',(85.1073031426544,-34.2233059232024,121.791105203505));
#50302=CARTESIAN_POINT('Ctrl Pts',(88.0988922613081,-32.9636812796899,121.633156680312));
#50303=CARTESIAN_POINT('Ctrl Pts',(90.7886812824939,-34.7764754615136,121.47520815712));
#50304=CARTESIAN_POINT('Ctrl Pts',(90.7413295634957,-38.0215233333396,121.317259633928));
#50305=CARTESIAN_POINT('Ctrl Pts',(87.9981117812556,-39.7549731697557,121.159311110735));
#50306=CARTESIAN_POINT('Ctrl Pts',(85.047026109322,-38.4059687154998,121.001362587542));
#50307=CARTESIAN_POINT('Ctrl Pts',(84.5633401927755,-35.197217406321,120.84341406435));
#50308=CARTESIAN_POINT('Ctrl Pts',(86.9857879627557,-33.038188007546,120.685465541157));
#50309=CARTESIAN_POINT('Ctrl Pts',(90.1179170017959,-33.8863136631071,120.527517017965));
#50310=CARTESIAN_POINT('Ctrl Pts',(91.1199662498861,-36.9726699339268,120.369568494773));
#50311=CARTESIAN_POINT('Ctrl Pts',(89.0833862070155,-39.498929427826,120.21161997158));
#50312=CARTESIAN_POINT('Ctrl Pts',(85.8546927193744,-39.1746202070418,120.053671448388));
#50313=CARTESIAN_POINT('Ctrl Pts',(84.361238791399,-36.2937783690392,119.895722925195));
#50314=CARTESIAN_POINT('Ctrl Pts',(85.9570961994953,-33.4683781249403,119.737774402003));
#50315=CARTESIAN_POINT('Ctrl Pts',(89.1953483414539,-33.2601227133794,119.57982587881));
#50316=CARTESIAN_POINT('Ctrl Pts',(91.1399710834037,-35.8578315813559,119.421877355618));
#50317=CARTESIAN_POINT('Ctrl Pts',(90.0278338382846,-38.9062408126556,119.263928832425));
#50318=CARTESIAN_POINT('Ctrl Pts',(86.8672777631298,-39.6414506121262,119.105980309233));
#50319=CARTESIAN_POINT('Ctrl Pts',(84.5238828587414,-37.3968685460779,118.94803178604));
#50320=CARTESIAN_POINT('Ctrl Pts',(85.1223340471412,-34.2075889414278,118.790083262848));
#50321=CARTESIAN_POINT('Ctrl Pts',(88.1200338206604,-32.9652346018622,118.632134739655));
#50322=CARTESIAN_POINT('Ctrl Pts',(90.7990589734528,-34.7962104304906,118.474186216463));
#50323=CARTESIAN_POINT('Ctrl Pts',(90.7304188745133,-38.0404263262544,118.316237693271));
#50324=CARTESIAN_POINT('Ctrl Pts',(87.976347415821,-39.756450406705,118.158289170078));
#50325=CARTESIAN_POINT('Ctrl Pts',(85.0338774267685,-38.3884158276996,118.000340646886));
#50326=CARTESIAN_POINT('Ctrl Pts',(84.5708569556909,-35.1766779355748,117.842392123693));
#50327=CARTESIAN_POINT('Ctrl Pts',(87.0070925813691,-33.033221796312,117.684443600501));
#50328=CARTESIAN_POINT('Ctrl Pts',(90.133723556862,-33.9014539012141,117.526495077308));
#50329=CARTESIAN_POINT('Ctrl Pts',(91.115928668822,-36.9941746068011,117.368546554116));
#50330=CARTESIAN_POINT('Ctrl Pts',(89.0631724146781,-39.5073081101905,117.210598030923));
#50331=CARTESIAN_POINT('Ctrl Pts',(85.8366264582907,-39.1622726973474,117.052649507731));
#50332=CARTESIAN_POINT('Ctrl Pts',(84.3617018873633,-36.2719014833249,116.894700984538));
#50333=CARTESIAN_POINT('Ctrl Pts',(85.9756679525495,-33.4568061412075,116.736752461346));
#50334=CARTESIAN_POINT('Ctrl Pts',(89.2151907091054,-33.2693480004399,116.578803938154));
#50335=CARTESIAN_POINT('Ctrl Pts',(91.1430933992921,-35.8794896559737,116.420855414961));
#50336=CARTESIAN_POINT('Ctrl Pts',(90.0114052884273,-38.9206950526068,116.262906891769));
#50337=CARTESIAN_POINT('Ctrl Pts',(86.846193567894,-39.6355957512928,116.104958368576));
#50338=CARTESIAN_POINT('Ctrl Pts',(84.5172594391369,-37.3760130312551,115.947009845384));
#50339=CARTESIAN_POINT('Ctrl Pts',(85.1361766453704,-34.1906418226499,115.789061322191));
#50340=CARTESIAN_POINT('Ctrl Pts',(88.1417917792184,-32.9675613216336,115.631112798999));
#50341=CARTESIAN_POINT('Ctrl Pts',(90.8090050104732,-34.8157014201656,115.473164275806));
#50342=CARTESIAN_POINT('Ctrl Pts',(90.7195352219795,-38.0594096995474,115.315215752614));
#50343=CARTESIAN_POINT('Ctrl Pts',(87.954501949864,-39.7577145157911,115.157267229421));
#50344=CARTESIAN_POINT('Ctrl Pts',(85.0208767672683,-38.370814543615,114.999318706229));
#50345=CARTESIAN_POINT('Ctrl Pts',(84.5784884050749,-35.1561698071348,114.841370183036));
#50346=CARTESIAN_POINT('Ctrl Pts',(87.0284369366511,-33.0284009199174,114.683421659844));
#50347=CARTESIAN_POINT('Ctrl Pts',(90.1494285402328,-33.9166912188371,114.525473136651));
#50348=CARTESIAN_POINT('Ctrl Pts',(91.1117550495216,-37.0156549059918,114.367524613459));
#50349=CARTESIAN_POINT('Ctrl Pts',(89.0429042863828,-39.5155558569582,114.209576090266));
#50350=CARTESIAN_POINT('Ctrl Pts',(85.818640316503,-39.1498099105458,114.051627567074));
#50351=CARTESIAN_POINT('Ctrl Pts',(84.3623052198161,-36.2500277927064,113.893679043881));
#50352=CARTESIAN_POINT('Ctrl Pts',(85.9943137360584,-33.4453537567987,113.735730520689));
#50353=CARTESIAN_POINT('Ctrl Pts',(89.2349733788484,-33.2787004508751,113.577781997497));
#50354=CARTESIAN_POINT('Ctrl Pts',(91.146076610276,-35.9011673588856,113.419833474304));
#50355=CARTESIAN_POINT('Ctrl Pts',(89.9948842539832,-38.9350434940625,113.261884951112));
#50356=CARTESIAN_POINT('Ctrl Pts',(86.8251474074879,-39.6296056358126,113.103936427919));
#50357=CARTESIAN_POINT('Ctrl Pts',(84.5107700663189,-37.3551154143638,112.945987904727));
#50358=CARTESIAN_POINT('Ctrl Pts',(85.1501277771093,-34.1737839380106,112.788039381534));
#50359=CARTESIAN_POINT('Ctrl Pts',(88.163534348671,-32.9700277005393,112.630090858342));
#50360=CARTESIAN_POINT('Ctrl Pts',(90.8188256911872,-34.8352558718741,112.472142335149));
#50361=CARTESIAN_POINT('Ctrl Pts',(90.7085299014341,-38.0783227974162,112.314193811957));
#50362=CARTESIAN_POINT('Ctrl Pts',(87.9326488174859,-39.7588383291988,112.156245288764));
#50363=CARTESIAN_POINT('Ctrl Pts',(85.0079893935519,-38.3531301451233,111.998296765572));
#50364=CARTESIAN_POINT('Ctrl Pts',(84.5862513798169,-35.1357111030109,111.840348242379));
#50365=CARTESIAN_POINT('Ctrl Pts',(87.0498118067535,-33.0237171949643,111.682399719187));
#50366=CARTESIAN_POINT('Ctrl Pts',(90.1650353610602,-33.9320290640263,111.524451195994));
#50367=CARTESIAN_POINT('Ctrl Pts',(91.1074435912917,-37.0371079635583,111.366502672802));
#50368=CARTESIAN_POINT('Ctrl Pts',(89.0225836171414,-39.523673292095,111.208554149609));
#50369=CARTESIAN_POINT('Ctrl Pts',(85.8007345690348,-39.1372318916473,111.050605626417));
#50370=CARTESIAN_POINT('Ctrl Pts',(84.3630489907538,-36.2281584270626,110.892657103224));
#50371=CARTESIAN_POINT('Ctrl Pts',(86.0130326709505,-33.4340213329109,110.734708580032));
#50372=CARTESIAN_POINT('Ctrl Pts',(89.2546955886631,-33.2881797332362,110.57676005684));
#50373=CARTESIAN_POINT('Ctrl Pts',(91.1489205673539,-35.922863769627,110.418811533647));
#50374=CARTESIAN_POINT('Ctrl Pts',(89.978271428617,-38.9492855591815,110.260863010455));
#50375=CARTESIAN_POINT('Ctrl Pts',(86.8041401438386,-39.6234805044202,110.102914487262));
#50376=CARTESIAN_POINT('Ctrl Pts',(84.5044150100778,-37.3341765642054,109.94496596407));
#50377=CARTESIAN_POINT('Ctrl Pts',(85.1641868672712,-34.1570159724828,109.787017440877));
#50378=CARTESIAN_POINT('Ctrl Pts',(88.1852606300547,-32.9726336552999,109.629068917685));
#50379=CARTESIAN_POINT('Ctrl Pts',(90.8285206169981,-34.854872942659,109.471120394492));
#50380=CARTESIAN_POINT('Ctrl Pts',(90.6974033531124,-38.0971649150734,109.3131718713));
#50381=CARTESIAN_POINT('Ctrl Pts',(87.9107889477286,-39.7598216466482,109.155223348107));
#50382=CARTESIAN_POINT('Ctrl Pts',(84.9952157791636,-38.335363677779,108.997274824915));
#50383=CARTESIAN_POINT('Ctrl Pts',(84.5941456787648,-35.1153020160809,108.839326301722));
#50384=CARTESIAN_POINT('Ctrl Pts',(87.0712160658443,-33.0191721524332,108.68137777853));
#50385=CARTESIAN_POINT('Ctrl Pts',(90.180543878778,-33.9474640533193,108.523429255338));
#50386=CARTESIAN_POINT('Ctrl Pts',(91.1029934377628,-37.0585385521308,108.365480732145));
#50387=CARTESIAN_POINT('Ctrl Pts',(89.0022133712807,-39.5316484480093,108.207532208953));
#50388=CARTESIAN_POINT('Ctrl Pts',(85.7829055813253,-39.124563080317,108.04958368576));
#50389=CARTESIAN_POINT('Ctrl Pts',(84.3639421614424,-36.2062450984898,107.891635162568));
#50390=CARTESIAN_POINT('Ctrl Pts',(86.0318054952116,-33.4229104868122,107.733686639375));
#50391=CARTESIAN_POINT('Ctrl Pts',(89.2743945484854,-33.2975774594042,107.575738116183));
#50392=CARTESIAN_POINT('Ctrl Pts',(91.1515469975838,-35.9450057508935,107.41778959299));
#50393=CARTESIAN_POINT('Ctrl Pts',(89.9617284945354,-38.9625411117384,107.259841069798));
#50394=CARTESIAN_POINT('Ctrl Pts',(86.7828503953456,-39.6190422373148,107.101892546605));
#50395=CARTESIAN_POINT('Ctrl Pts',(84.4989308941805,-37.3094602201476,106.943944023413));
#50396=CARTESIAN_POINT('Ctrl Pts',(84.952479646449,-35.2042483553399,106.838645007951));
#50397=CARTESIAN_POINT('Ctrl Pts',(85.5733584845537,-34.4780626356041,106.78599550022));
#50398=CARTESIAN_POINT('Ctrl Pts',(87.0704891624108,-38.966058260622,122.21400449978));
#50399=CARTESIAN_POINT('Ctrl Pts',(86.2067093668289,-38.7351332702521,122.161354992049));
#50400=CARTESIAN_POINT('Ctrl Pts',(84.7409656511953,-37.3519760297414,122.056055976587));
#50401=CARTESIAN_POINT('Ctrl Pts',(85.2780754157145,-34.3600917509159,121.898107453395));
#50402=CARTESIAN_POINT('Ctrl Pts',(88.0776945938096,-33.1812970804881,121.740158930202));
#50403=CARTESIAN_POINT('Ctrl Pts',(90.5948801530784,-34.8777644615624,121.58221040701));
#50404=CARTESIAN_POINT('Ctrl Pts',(90.5505669886146,-37.9145779728672,121.424261883817));
#50405=CARTESIAN_POINT('Ctrl Pts',(87.9833811859376,-39.5367925263418,121.266313360625));
#50406=CARTESIAN_POINT('Ctrl Pts',(85.2216663528979,-38.2743535376715,121.108364837432));
#50407=CARTESIAN_POINT('Ctrl Pts',(84.7690185077461,-35.2715074426312,120.95041631424));
#50408=CARTESIAN_POINT('Ctrl Pts',(87.0360180741243,-33.2510227199158,120.792467791047));
#50409=CARTESIAN_POINT('Ctrl Pts',(89.9671587415673,-34.0447242466188,120.634519267855));
#50410=CARTESIAN_POINT('Ctrl Pts',(90.9049066010096,-36.9330293792797,120.476570744662));
#50411=CARTESIAN_POINT('Ctrl Pts',(88.999013672668,-39.2971790828151,120.31862222147));
#50412=CARTESIAN_POINT('Ctrl Pts',(85.9775050865362,-38.9936807486089,120.160673698277));
#50413=CARTESIAN_POINT('Ctrl Pts',(84.579885930787,-36.2977022105001,120.002725175085));
#50414=CARTESIAN_POINT('Ctrl Pts',(86.0733373467429,-33.6536075853888,119.844776651893));
#50415=CARTESIAN_POINT('Ctrl Pts',(89.1037912094091,-33.4587159003937,119.6868281287));
#50416=CARTESIAN_POINT('Ctrl Pts',(90.9236277265884,-35.8897300796293,119.528879605508));
#50417=CARTESIAN_POINT('Ctrl Pts',(89.8828562046253,-38.7425232300701,119.370931082315));
#50418=CARTESIAN_POINT('Ctrl Pts',(86.9251126608097,-39.4305546985919,119.212982559123));
#50419=CARTESIAN_POINT('Ctrl Pts',(84.7320931464425,-37.3300072137338,119.05503403593));
#50420=CARTESIAN_POINT('Ctrl Pts',(85.2921417887346,-34.3453833261113,118.897085512738));
#50421=CARTESIAN_POINT('Ctrl Pts',(88.0974795016528,-33.1827507261497,118.739136989545));
#50422=CARTESIAN_POINT('Ctrl Pts',(90.6045919087642,-34.896233039778,118.581188466353));
#50423=CARTESIAN_POINT('Ctrl Pts',(90.540356437329,-37.932267962832,118.42323994316));
#50424=CARTESIAN_POINT('Ctrl Pts',(87.9630134374091,-39.5381749691605,118.265291419968));
#50425=CARTESIAN_POINT('Ctrl Pts',(85.2093614198393,-38.2579270167265,118.107342896775));
#50426=CARTESIAN_POINT('Ctrl Pts',(84.7760529208225,-35.2522859874351,117.949394373583));
#50427=CARTESIAN_POINT('Ctrl Pts',(87.055955577734,-33.2463751899036,117.791445850391));
#50428=CARTESIAN_POINT('Ctrl Pts',(89.9819509917552,-34.0588929373327,117.633497327198));
#50429=CARTESIAN_POINT('Ctrl Pts',(90.9011281110726,-36.9531540996908,117.475548804005));
#50430=CARTESIAN_POINT('Ctrl Pts',(88.9800969971335,-39.3050201060654,117.317600280813));
#50431=CARTESIAN_POINT('Ctrl Pts',(85.9605981354142,-38.9821255772365,117.159651757621));
#50432=CARTESIAN_POINT('Ctrl Pts',(84.5803193099349,-36.2772291621056,117.001703234428));
#50433=CARTESIAN_POINT('Ctrl Pts',(86.0907173524721,-33.6427781745634,116.843754711236));
#50434=CARTESIAN_POINT('Ctrl Pts',(89.1223602945383,-33.4673492018109,116.685806188043));
#50435=CARTESIAN_POINT('Ctrl Pts',(90.926549683814,-35.9099983580111,116.527857664851));
#50436=CARTESIAN_POINT('Ctrl Pts',(89.8674818729827,-38.7560499430534,116.369909141658));
#50437=CARTESIAN_POINT('Ctrl Pts',(86.9053814360339,-39.4250755435261,116.211960618466));
#50438=CARTESIAN_POINT('Ctrl Pts',(84.7258947509363,-37.3104899949744,116.054012095273));
#50439=CARTESIAN_POINT('Ctrl Pts',(85.3050961089771,-34.329523702058,115.896063572081));
#50440=CARTESIAN_POINT('Ctrl Pts',(88.1178412544334,-33.1849281405724,115.738115048888));
#50441=CARTESIAN_POINT('Ctrl Pts',(90.6138997096969,-34.9144732948164,115.580166525696));
#50442=CARTESIAN_POINT('Ctrl Pts',(90.5301711875661,-37.950033175175,115.422218002503));
#50443=CARTESIAN_POINT('Ctrl Pts',(87.9425697925695,-39.5393579605074,115.264269479311));
#50444=CARTESIAN_POINT('Ctrl Pts',(85.1971950112113,-38.2414552050812,115.106320956119));
#50445=CARTESIAN_POINT('Ctrl Pts',(84.7831946609494,-35.2330938633132,114.948372432926));
#50446=CARTESIAN_POINT('Ctrl Pts',(87.075930268115,-33.2418636686103,114.790423909734));
#50447=CARTESIAN_POINT('Ctrl Pts',(89.9966481880921,-34.0731524779808,114.632475386541));
#50448=CARTESIAN_POINT('Ctrl Pts',(90.8972223124579,-36.9732560104747,114.474526863349));
#50449=CARTESIAN_POINT('Ctrl Pts',(88.9611294723736,-39.3127385958416,114.316578340156));
#50450=CARTESIAN_POINT('Ctrl Pts',(85.9437661623417,-38.9704625260759,114.158629816964));
#50451=CARTESIAN_POINT('Ctrl Pts',(84.5808839266114,-36.256759103778,114.000681293771));
#50452=CARTESIAN_POINT('Ctrl Pts',(86.1081666381298,-33.6320606883866,113.842732770579));
#50453=CARTESIAN_POINT('Ctrl Pts',(89.1408735125671,-33.4761015065434,113.684784247386));
#50454=CARTESIAN_POINT('Ctrl Pts',(90.9293414624814,-35.9302850051414,113.526835724194));
#50455=CARTESIAN_POINT('Ctrl Pts',(89.8520209914789,-38.7694776466189,113.368887201001));
#50456=CARTESIAN_POINT('Ctrl Pts',(86.8856858053969,-39.4194698130891,113.210938677809));
#50457=CARTESIAN_POINT('Ctrl Pts',(84.7198218004494,-37.2909333758316,113.052990154616));
#50458=CARTESIAN_POINT('Ctrl Pts',(85.318151998146,-34.3137475859984,112.895041631424));
#50459=CARTESIAN_POINT('Ctrl Pts',(88.1381886056259,-33.1872362522184,112.737093108232));
#50460=CARTESIAN_POINT('Ctrl Pts',(90.6230901984232,-34.9327729395367,112.579144585039));
#50461=CARTESIAN_POINT('Ctrl Pts',(90.5198720772144,-37.96773262166,112.421196061847));
#50462=CARTESIAN_POINT('Ctrl Pts',(87.9221189732622,-39.5404096589339,112.263247538654));
#50463=CARTESIAN_POINT('Ctrl Pts',(85.185134618831,-38.2249056124711,112.105299015462));
#50464=CARTESIAN_POINT('Ctrl Pts',(84.7904594864668,-35.2139479919543,111.947350492269));
#50465=CARTESIAN_POINT('Ctrl Pts',(87.0959335151835,-33.2374804977659,111.789401969077));
#50466=CARTESIAN_POINT('Ctrl Pts',(90.0112535209652,-34.0875060953524,111.631453445884));
#50467=CARTESIAN_POINT('Ctrl Pts',(90.8931875200224,-36.9933324277266,111.473504922692));
#50468=CARTESIAN_POINT('Ctrl Pts',(88.9421127782144,-39.3203351360697,111.315556399499));
#50469=CARTESIAN_POINT('Ctrl Pts',(85.9270094246943,-38.9586916372493,111.157607876307));
#50470=CARTESIAN_POINT('Ctrl Pts',(84.5815799698509,-36.2362930928918,110.999659353114));
#50471=CARTESIAN_POINT('Ctrl Pts',(86.1256843810546,-33.6214554648776,110.841710829922));
#50472=CARTESIAN_POINT('Ctrl Pts',(89.1593301503747,-33.484972504411,110.683762306729));
#50473=CARTESIAN_POINT('Ctrl Pts',(90.9320029231501,-35.950589159622,110.525813783537));
#50474=CARTESIAN_POINT('Ctrl Pts',(89.8364742092662,-38.7828058000054,110.367865260344));
#50475=CARTESIAN_POINT('Ctrl Pts',(86.8660265755163,-39.413737730696,110.209916737152));
#50476=CARTESIAN_POINT('Ctrl Pts',(84.7138745474594,-37.2713381693559,110.051968213959));
#50477=CARTESIAN_POINT('Ctrl Pts',(85.3313089180581,-34.298055618951,109.894019690767));
#50478=CARTESIAN_POINT('Ctrl Pts',(88.1585207139529,-33.1896749831523,109.736071167575));
#50479=CARTESIAN_POINT('Ctrl Pts',(90.6321630019245,-34.9511311850741,109.578122644382));
#50480=CARTESIAN_POINT('Ctrl Pts',(90.5094595182593,-37.9853656427257,109.42017412119));
#50481=CARTESIAN_POINT('Ctrl Pts',(87.9016618489127,-39.5413298770121,109.262225597997));
#50482=CARTESIAN_POINT('Ctrl Pts',(85.1731806858554,-38.2082792173576,109.104277074805));
#50483=CARTESIAN_POINT('Ctrl Pts',(84.7978472091305,-35.1948485538596,108.946328551612));
#50484=CARTESIAN_POINT('Ctrl Pts',(87.1159642653522,-33.2332271101078,108.78838002842));
#50485=CARTESIAN_POINT('Ctrl Pts',(90.0257668588284,-34.1019506231015,108.630431505227));
#50486=CARTESIAN_POINT('Ctrl Pts',(90.8890229323498,-37.0133878178172,108.472482982035));
#50487=CARTESIAN_POINT('Ctrl Pts',(88.9230496887618,-39.3277985271172,108.314534458842));
#50488=CARTESIAN_POINT('Ctrl Pts',(85.9103245211404,-38.946835782131,108.15658593565));
#50489=CARTESIAN_POINT('Ctrl Pts',(84.582415825876,-36.2157859401729,107.998637412457));
#50490=CARTESIAN_POINT('Ctrl Pts',(86.1432525552737,-33.6110576005356,107.840688889265));
#50491=CARTESIAN_POINT('Ctrl Pts',(89.1777650301391,-33.4937671795376,107.682740366073));
#50492=CARTESIAN_POINT('Ctrl Pts',(90.9344608156447,-35.9713102924167,107.52479184288));
#50493=CARTESIAN_POINT('Ctrl Pts',(89.8209928334223,-38.7952107452311,107.366843319688));
#50494=CARTESIAN_POINT('Ctrl Pts',(86.846102987813,-39.4095842666964,107.208894796495));
#50495=CARTESIAN_POINT('Ctrl Pts',(84.7087423466685,-37.2482078703435,107.050946273303));
#50496=CARTESIAN_POINT('Ctrl Pts',(85.1331869260174,-35.2780872164347,106.945647257841));
#50497=CARTESIAN_POINT('Ctrl Pts',(85.7142240382307,-34.5985007534561,106.89299775011));
#50498=CARTESIAN_POINT('Ctrl Pts',(87.1183555905968,-38.7870128767185,122.321006749669));
#50499=CARTESIAN_POINT('Ctrl Pts',(86.3138051921097,-38.5719224173526,122.268357241939));
#50500=CARTESIAN_POINT('Ctrl Pts',(84.9485675510758,-37.2836082952637,122.163058226477));
#50501=CARTESIAN_POINT('Ctrl Pts',(85.4488476887748,-34.4968775786294,122.005109703285));
#50502=CARTESIAN_POINT('Ctrl Pts',(88.056496926311,-33.3989128812863,121.847161180092));
#50503=CARTESIAN_POINT('Ctrl Pts',(90.401079023663,-34.9790534616111,121.6892126569));
#50504=CARTESIAN_POINT('Ctrl Pts',(90.3598044137333,-37.8076326123949,121.531264133707));
#50505=CARTESIAN_POINT('Ctrl Pts',(87.9686505906198,-39.3186118829278,121.373315610515));
#50506=CARTESIAN_POINT('Ctrl Pts',(85.3963065964737,-38.1427383598431,121.215367087322));
#50507=CARTESIAN_POINT('Ctrl Pts',(84.9746968227168,-35.3457974789413,121.05741856413));
#50508=CARTESIAN_POINT('Ctrl Pts',(87.086248185493,-33.4638574322856,120.899470040937));
#50509=CARTESIAN_POINT('Ctrl Pts',(89.8164004813384,-34.2031348301304,120.741521517745));
#50510=CARTESIAN_POINT('Ctrl Pts',(90.6898469521331,-36.8933888246327,120.583572994552));
#50511=CARTESIAN_POINT('Ctrl Pts',(88.9146411383204,-39.0954287378041,120.42562447136));
#50512=CARTESIAN_POINT('Ctrl Pts',(86.1003174536982,-38.8127412901761,120.267675948167));
#50513=CARTESIAN_POINT('Ctrl Pts',(84.798533070175,-36.3016260519611,120.109727424975));
#50514=CARTESIAN_POINT('Ctrl Pts',(86.1895784939907,-33.8388370458375,119.951778901782));
#50515=CARTESIAN_POINT('Ctrl Pts',(89.0122340773642,-33.657309087408,119.79383037859));
#50516=CARTESIAN_POINT('Ctrl Pts',(90.7072843697732,-35.9216285779027,119.635881855397));
#50517=CARTESIAN_POINT('Ctrl Pts',(89.737878570966,-38.5788056474845,119.477933332205));
#50518=CARTESIAN_POINT('Ctrl Pts',(86.9829475584895,-39.2196587850576,119.319984809012));
#50519=CARTESIAN_POINT('Ctrl Pts',(84.9403034341435,-37.2631458813898,119.16203628582));
#50520=CARTESIAN_POINT('Ctrl Pts',(85.4619495303279,-34.4831777107948,119.004087762628));
#50521=CARTESIAN_POINT('Ctrl Pts',(88.0749251826453,-33.4002668504372,118.846139239435));
#50522=CARTESIAN_POINT('Ctrl Pts',(90.4101248440757,-34.9962556490655,118.688190716243));
#50523=CARTESIAN_POINT('Ctrl Pts',(90.3502940001447,-37.8241095994096,118.53024219305));
#50524=CARTESIAN_POINT('Ctrl Pts',(87.9496794589972,-39.319899531616,118.372293669858));
#50525=CARTESIAN_POINT('Ctrl Pts',(85.3848454129102,-38.1274382057533,118.214345146665));
#50526=CARTESIAN_POINT('Ctrl Pts',(84.981248885954,-35.3278940392956,118.056396623473));
#50527=CARTESIAN_POINT('Ctrl Pts',(87.1048185740992,-33.4595285834953,117.89844810028));
#50528=CARTESIAN_POINT('Ctrl Pts',(89.8301784266481,-34.2163319734512,117.740499577088));
#50529=CARTESIAN_POINT('Ctrl Pts',(90.6863275533235,-36.9121335925805,117.582551053895));
#50530=CARTESIAN_POINT('Ctrl Pts',(88.8970215795888,-39.1027321019403,117.424602530703));
#50531=CARTESIAN_POINT('Ctrl Pts',(86.0845698125377,-38.8019784571255,117.26665400751));
#50532=CARTESIAN_POINT('Ctrl Pts',(84.7989367325066,-36.2825568408863,117.108705484318));
#50533=CARTESIAN_POINT('Ctrl Pts',(86.2057667523946,-33.8287502079193,116.950756961126));
#50534=CARTESIAN_POINT('Ctrl Pts',(89.0295298799712,-33.665350403182,116.792808437933));
#50535=CARTESIAN_POINT('Ctrl Pts',(90.7100059683359,-35.9405070600484,116.634859914741));
#50536=CARTESIAN_POINT('Ctrl Pts',(89.7235584575382,-38.5914048335001,116.476911391548));
#50537=CARTESIAN_POINT('Ctrl Pts',(86.9645693041736,-39.2145553357593,116.318962868356));
#50538=CARTESIAN_POINT('Ctrl Pts',(84.9345300627357,-37.2449669586938,116.161014345163));
#50539=CARTESIAN_POINT('Ctrl Pts',(85.4740155725839,-34.4684055814659,116.003065821971));
#50540=CARTESIAN_POINT('Ctrl Pts',(88.0938907296483,-33.4022949595113,115.845117298778));
#50541=CARTESIAN_POINT('Ctrl Pts',(90.4187944089205,-35.0132451694672,115.687168775586));
#50542=CARTESIAN_POINT('Ctrl Pts',(90.3408071531528,-37.8406566508026,115.529220252393));
#50543=CARTESIAN_POINT('Ctrl Pts',(87.930637635275,-39.3210014052237,115.371271729201));
#50544=CARTESIAN_POINT('Ctrl Pts',(85.3735132551544,-38.1120958665474,115.213323206008));
#50545=CARTESIAN_POINT('Ctrl Pts',(84.9879009168238,-35.3100179194915,115.055374682816));
#50546=CARTESIAN_POINT('Ctrl Pts',(87.1234235995788,-33.4553264173033,114.897426159623));
#50547=CARTESIAN_POINT('Ctrl Pts',(89.8438678359514,-34.2296137371245,114.739477636431));
#50548=CARTESIAN_POINT('Ctrl Pts',(90.6826895753943,-36.9308571149577,114.581529113239));
#50549=CARTESIAN_POINT('Ctrl Pts',(88.8793546583644,-39.1099213347251,114.423580590046));
#50550=CARTESIAN_POINT('Ctrl Pts',(86.0688920081806,-38.791115141606,114.265632066854));
#50551=CARTESIAN_POINT('Ctrl Pts',(84.7994626334068,-36.2634904148495,114.107683543661));
#50552=CARTESIAN_POINT('Ctrl Pts',(86.2220195402012,-33.8187676199746,113.949735020469));
#50553=CARTESIAN_POINT('Ctrl Pts',(89.0467736462859,-33.6735025622116,113.791786497276));
#50554=CARTESIAN_POINT('Ctrl Pts',(90.7126063146866,-35.9594026513973,113.633837974084));
#50555=CARTESIAN_POINT('Ctrl Pts',(89.7091577289746,-38.6039117991753,113.475889450891));
#50556=CARTESIAN_POINT('Ctrl Pts',(86.946224203306,-39.2093339903656,113.317940927699));
#50557=CARTESIAN_POINT('Ctrl Pts',(84.9288735345797,-37.2267513372994,113.159992404506));
#50558=CARTESIAN_POINT('Ctrl Pts',(85.4861762191828,-34.4537112339862,113.002043881314));
#50559=CARTESIAN_POINT('Ctrl Pts',(88.1128428625806,-33.4044448038976,112.844095358121));
#50560=CARTESIAN_POINT('Ctrl Pts',(90.4273547056591,-35.0302900071992,112.686146834929));
#50561=CARTESIAN_POINT('Ctrl Pts',(90.3312142529948,-37.8571424459038,112.528198311737));
#50562=CARTESIAN_POINT('Ctrl Pts',(87.9115891290386,-39.3219809886689,112.370249788544));
#50563=CARTESIAN_POINT('Ctrl Pts',(85.3622798441101,-38.0966810798189,112.212301265352));
#50564=CARTESIAN_POINT('Ctrl Pts',(84.9946675931167,-35.2921848808977,112.054352742159));
#50565=CARTESIAN_POINT('Ctrl Pts',(87.1420552236133,-33.4512438005674,111.896404218967));
#50566=CARTESIAN_POINT('Ctrl Pts',(89.8574716808703,-34.2429831266786,111.738455695774));
#50567=CARTESIAN_POINT('Ctrl Pts',(90.6789314487532,-36.9495568918948,111.580507172582));
#50568=CARTESIAN_POINT('Ctrl Pts',(88.8616419392871,-39.1169969800445,111.422558649389));
#50569=CARTESIAN_POINT('Ctrl Pts',(86.0532842803539,-38.7801513828512,111.264610126197));
#50570=CARTESIAN_POINT('Ctrl Pts',(84.8001109489481,-36.244427758721,111.106661603004));
#50571=CARTESIAN_POINT('Ctrl Pts',(86.2383360911588,-33.8088895968443,110.948713079812));
#50572=CARTESIAN_POINT('Ctrl Pts',(89.0639647120862,-33.6817652755859,110.790764556619));
#50573=CARTESIAN_POINT('Ctrl Pts',(90.7150852789466,-35.9783145496169,110.632816033427));
#50574=CARTESIAN_POINT('Ctrl Pts',(89.6946769899154,-38.6163260408294,110.474867510234));
#50575=CARTESIAN_POINT('Ctrl Pts',(86.9279130071941,-39.2039949569718,110.316918987042));
#50576=CARTESIAN_POINT('Ctrl Pts',(84.9233340848409,-37.2084997745063,110.158970463849));
#50577=CARTESIAN_POINT('Ctrl Pts',(85.4984309688452,-34.4390952654192,110.001021940657));
#50578=CARTESIAN_POINT('Ctrl Pts',(88.131780797851,-33.4067163110047,109.843073417464));
#50579=CARTESIAN_POINT('Ctrl Pts',(90.4358053868511,-35.0473894274892,109.685124894272));
#50580=CARTESIAN_POINT('Ctrl Pts',(90.3215156834062,-37.873566370378,109.52717637108));
#50581=CARTESIAN_POINT('Ctrl Pts',(87.8925347500967,-39.322838107376,109.369227847887));
#50582=CARTESIAN_POINT('Ctrl Pts',(85.3511455925472,-38.0811947569362,109.211279324695));
#50583=CARTESIAN_POINT('Ctrl Pts',(85.0015487394962,-35.2743950916382,109.053330801502));
#50584=CARTESIAN_POINT('Ctrl Pts',(87.1607124648601,-33.4472820677823,108.89538227831));
#50585=CARTESIAN_POINT('Ctrl Pts',(89.8709898388786,-34.2564371928838,108.737433755117));
#50586=CARTESIAN_POINT('Ctrl Pts',(90.675052426937,-36.9682370835035,108.579485231925));
#50587=CARTESIAN_POINT('Ctrl Pts',(88.8438860062427,-39.1239486062252,108.421536708732));
#50588=CARTESIAN_POINT('Ctrl Pts',(86.0377434609558,-38.7691084839451,108.26358818554));
#50589=CARTESIAN_POINT('Ctrl Pts',(84.8008894903094,-36.225326781856,108.105639662347));
#50590=CARTESIAN_POINT('Ctrl Pts',(86.254699615336,-33.799204714259,107.947691139155));
#50591=CARTESIAN_POINT('Ctrl Pts',(89.0811355117927,-33.6899568996709,107.789742615962));
#50592=CARTESIAN_POINT('Ctrl Pts',(90.7173746337058,-35.9976148339398,107.63179409277));
#50593=CARTESIAN_POINT('Ctrl Pts',(89.6802571723091,-38.6278803787238,107.473845569577));
#50594=CARTESIAN_POINT('Ctrl Pts',(86.9093555802804,-39.200126296078,107.315897046385));
#50595=CARTESIAN_POINT('Ctrl Pts',(84.9185537991564,-37.1869555205393,107.157948523193));
#50596=CARTESIAN_POINT('Ctrl Pts',(85.3138942055859,-35.3519260775293,107.052649507731));
#50597=CARTESIAN_POINT('Ctrl Pts',(85.8550895919077,-34.718938871308,107.));
#50598=CARTESIAN_POINT('Ctrl Pts',(85.2535610703604,-36.3531642914838,121.112583302492));
#50599=CARTESIAN_POINT('Ctrl Pts',(85.2516482037573,-36.0616114634661,121.094195056371));
#50600=CARTESIAN_POINT('Ctrl Pts',(85.298519492613,-35.7706534853458,121.07580681025));
#50601=CARTESIAN_POINT('Ctrl Pts',(85.3968903454723,-35.4982976179823,121.05741856413));
#50602=CARTESIAN_POINT('Ctrl Pts',(85.6785472769755,-34.7184841300561,121.004769056399));
#50603=CARTESIAN_POINT('Ctrl Pts',(86.3823977312343,-34.0911707811709,120.952119548668));
#50604=CARTESIAN_POINT('Ctrl Pts',(87.1893483410045,-33.9007270063691,120.899470040937));
#50605=CARTESIAN_POINT('Ctrl Pts',(87.9962989507748,-33.7102832315672,120.846820533206));
#50606=CARTESIAN_POINT('Ctrl Pts',(88.9063497160566,-33.9567090308488,120.794171025476));
#50607=CARTESIAN_POINT('Ctrl Pts',(89.5069495104966,-34.52829759624,120.741521517745));
#50608=CARTESIAN_POINT('Ctrl Pts',(90.1075493049366,-35.0998861616311,120.688872010014));
#50609=CARTESIAN_POINT('Ctrl Pts',(90.3986981285349,-35.9966374931319,120.636222502283));
#50610=CARTESIAN_POINT('Ctrl Pts',(90.2484049046985,-36.8120198110775,120.583572994552));
#50611=CARTESIAN_POINT('Ctrl Pts',(90.0981116808622,-37.6274021290232,120.530923486821));
#50612=CARTESIAN_POINT('Ctrl Pts',(89.5063764095913,-38.3614154334136,120.478273979091));
#50613=CARTESIAN_POINT('Ctrl Pts',(88.7414548265188,-38.6813075110042,120.42562447136));
#50614=CARTESIAN_POINT('Ctrl Pts',(87.9765332434463,-39.0011995885948,120.372974963629));
#50615=CARTESIAN_POINT('Ctrl Pts',(87.0384253485722,-38.9069704393855,120.320325455898));
#50616=CARTESIAN_POINT('Ctrl Pts',(86.3524073372147,-38.4413366584116,120.267675948167));
#50617=CARTESIAN_POINT('Ctrl Pts',(85.6787932621231,-37.9841220321056,120.215978399609));
#50618=CARTESIAN_POINT('Ctrl Pts',(85.2482353778633,-37.1688121351973,120.16428085105));
#50619=CARTESIAN_POINT('Ctrl Pts',(85.2469700844899,-36.3546528234761,120.112583302492));
#50620=CARTESIAN_POINT('Ctrl Pts',(86.9747563060389,-39.3241490284291,122.));
#50621=CARTESIAN_POINT('Ctrl Pts',(86.8817062191854,-39.290110891006,122.));
#50622=CARTESIAN_POINT('Ctrl Pts',(86.7907212975493,-39.2513040586725,122.));
#50623=CARTESIAN_POINT('Ctrl Pts',(86.7020100267322,-39.2080568530126,122.));
#50624=CARTESIAN_POINT('Ctrl Pts',(86.6113318105991,-39.1638507512867,122.));
#50625=CARTESIAN_POINT('Ctrl Pts',(86.5230285198804,-39.1150045689307,122.));
#50626=CARTESIAN_POINT('Ctrl Pts',(86.4373517348404,-39.0618234125105,122.));
#50627=CARTESIAN_POINT('Ctrl Pts',(86.3549203075593,-39.0106567093467,122.));
#50628=CARTESIAN_POINT('Ctrl Pts',(86.2749198914356,-38.9554763459202,122.));
#50629=CARTESIAN_POINT('Ctrl Pts',(86.197607513613,-38.8965240074405,122.));
#50630=CARTESIAN_POINT('Ctrl Pts',(86.1299591830182,-38.8449407112708,122.));
#50631=CARTESIAN_POINT('Ctrl Pts',(86.0643691719831,-38.7904687993429,122.));
#50632=CARTESIAN_POINT('Ctrl Pts',(86.0010342894347,-38.7332574826561,122.));
#50633=CARTESIAN_POINT('Ctrl Pts',(85.986897867521,-38.7204878480034,122.));
#50634=CARTESIAN_POINT('Ctrl Pts',(85.9728711507639,-38.7075790036905,122.));
#50635=CARTESIAN_POINT('Ctrl Pts',(85.9589759122883,-38.6945511416087,122.));
#50636=CARTESIAN_POINT('Ctrl Pts',(85.8865458109709,-38.6266423128259,122.));
#50637=CARTESIAN_POINT('Ctrl Pts',(85.8175813968922,-38.5554115699911,122.));
#50638=CARTESIAN_POINT('Ctrl Pts',(85.7523226201221,-38.4811496345928,122.));
#50639=CARTESIAN_POINT('Ctrl Pts',(85.687422873419,-38.4072962613675,122.));
#50640=CARTESIAN_POINT('Ctrl Pts',(85.6261876156017,-38.3304441599178,122.));
#50641=CARTESIAN_POINT('Ctrl Pts',(85.5688964676845,-38.2508525115488,122.));
#50642=CARTESIAN_POINT('Ctrl Pts',(85.5137335478701,-38.1742175011415,122.));
#50643=CARTESIAN_POINT('Ctrl Pts',(85.4622269892531,-38.0950419612856,122.));
#50644=CARTESIAN_POINT('Ctrl Pts',(85.4146712402722,-38.0135436638871,122.));
#50645=CARTESIAN_POINT('Ctrl Pts',(85.3947249112917,-37.9793607967031,122.));
#50646=CARTESIAN_POINT('Ctrl Pts',(85.375474185618,-37.9447691989933,122.));
#50647=CARTESIAN_POINT('Ctrl Pts',(85.3569433734486,-37.9097846421959,122.));
#50648=CARTESIAN_POINT('Ctrl Pts',(85.3440608433971,-37.8854635492962,122.));
#50649=CARTESIAN_POINT('Ctrl Pts',(85.3315262772696,-37.8609525380258,122.));
#50650=CARTESIAN_POINT('Ctrl Pts',(85.3193483089147,-37.8362569015937,122.));
#50651=CARTESIAN_POINT('Ctrl Pts',(85.3114399504896,-37.8202195841407,122.));
#50652=CARTESIAN_POINT('Ctrl Pts',(85.3036808680344,-37.8041017938262,122.));
#50653=CARTESIAN_POINT('Ctrl Pts',(85.2960836020132,-37.7879271698132,122.));
#50654=CARTESIAN_POINT('Ctrl Pts',(85.2539632958679,-37.6982527904632,122.));
#50655=CARTESIAN_POINT('Ctrl Pts',(85.2167418241088,-37.6066948163004,122.));
#50656=CARTESIAN_POINT('Ctrl Pts',(85.1847104706482,-37.5135256106319,122.));
#50657=CARTESIAN_POINT('Ctrl Pts',(85.1548307191947,-37.4266147433807,122.));
#50658=CARTESIAN_POINT('Ctrl Pts',(85.1294674189967,-37.3383010414635,122.));
#50659=CARTESIAN_POINT('Ctrl Pts',(85.1089075479901,-37.2487968899418,122.));
#50660=CARTESIAN_POINT('Ctrl Pts',(85.1074270584421,-37.2423518125,122.));
#50661=CARTESIAN_POINT('Ctrl Pts',(85.105971498406,-37.2359005611176,122.));
#50662=CARTESIAN_POINT('Ctrl Pts',(85.1045409856617,-37.2294432147812,122.));
#50663=CARTESIAN_POINT('Ctrl Pts',(85.0839347678633,-37.1364265775401,122.));
#50664=CARTESIAN_POINT('Ctrl Pts',(85.0685215768674,-37.04214426797,122.));
#50665=CARTESIAN_POINT('Ctrl Pts',(85.0582244923225,-36.9470041536375,122.));
#50666=CARTESIAN_POINT('Ctrl Pts',(85.0524279776539,-36.8934471428256,122.));
#50667=CARTESIAN_POINT('Ctrl Pts',(85.0482536228696,-36.8396184930835,122.));
#50668=CARTESIAN_POINT('Ctrl Pts',(85.0456944683025,-36.7855935994856,122.));
#50669=CARTESIAN_POINT('Ctrl Pts',(85.0450335864434,-36.7716420888667,122.));
#50670=CARTESIAN_POINT('Ctrl Pts',(85.0444805412283,-36.7576780899949,122.));
#50671=CARTESIAN_POINT('Ctrl Pts',(85.0440354542009,-36.7437162707763,122.));
#50672=CARTESIAN_POINT('Ctrl Pts',(85.0410640494509,-36.6505070478834,122.));
#50673=CARTESIAN_POINT('Ctrl Pts',(85.0428918001145,-36.557239583447,122.));
#50674=CARTESIAN_POINT('Ctrl Pts',(85.0493838115575,-36.4642889583755,122.));
#50675=CARTESIAN_POINT('Ctrl Pts',(85.0558866172978,-36.3711837838725,122.));
#50676=CARTESIAN_POINT('Ctrl Pts',(85.0670695852548,-36.27839552357,122.));
#50677=CARTESIAN_POINT('Ctrl Pts',(85.0828480795227,-36.1863132281589,122.));
#50678=CARTESIAN_POINT('Ctrl Pts',(85.0984009758062,-36.0955475083282,122.));
#50679=CARTESIAN_POINT('Ctrl Pts',(85.1184193868686,-36.0054668661199,122.));
#50680=CARTESIAN_POINT('Ctrl Pts',(85.1428652803547,-35.9164691013446,122.));
#50681=CARTESIAN_POINT('Ctrl Pts',(85.1519640438232,-35.8833441263305,122.));
#50682=CARTESIAN_POINT('Ctrl Pts',(85.1616765572995,-35.8503694822698,122.));
#50683=CARTESIAN_POINT('Ctrl Pts',(85.1720022212126,-35.817566946539,122.));
#50684=CARTESIAN_POINT('Ctrl Pts',(85.1789966596367,-35.7953470371703,122.));
#50685=CARTESIAN_POINT('Ctrl Pts',(85.1862724563629,-35.7732061147807,122.));
#50686=CARTESIAN_POINT('Ctrl Pts',(85.1938296041438,-35.751151161507,122.));
#50687=CARTESIAN_POINT('Ctrl Pts',(85.1983456598534,-35.737971401028,122.));
#50688=CARTESIAN_POINT('Ctrl Pts',(85.2029618432749,-35.7248235133138,122.));
#50689=CARTESIAN_POINT('Ctrl Pts',(85.2076746824257,-35.7117181369059,122.));
#50690=CARTESIAN_POINT('Ctrl Pts',(85.2393064450318,-35.6237571133841,122.));
#50691=CARTESIAN_POINT('Ctrl Pts',(85.2753274324375,-35.5375938379398,122.));
#50692=CARTESIAN_POINT('Ctrl Pts',(85.3156730801928,-35.4536425565309,122.));
#50693=CARTESIAN_POINT('Ctrl Pts',(85.3459323160092,-35.3906790954742,122.));
#50694=CARTESIAN_POINT('Ctrl Pts',(85.3786252206014,-35.3289603730047,122.));
#50695=CARTESIAN_POINT('Ctrl Pts',(85.4137405176868,-35.268676680312,122.));
#50696=CARTESIAN_POINT('Ctrl Pts',(85.4272098015241,-35.2455534766078,122.));
#50697=CARTESIAN_POINT('Ctrl Pts',(85.4410356214481,-35.2226415677282,122.));
#50698=CARTESIAN_POINT('Ctrl Pts',(85.4552178215069,-35.1999523366376,122.));
#50699=CARTESIAN_POINT('Ctrl Pts',(85.4653422141899,-35.1837549424194,122.));
#50700=CARTESIAN_POINT('Ctrl Pts',(85.475649063879,-35.1676699643451,122.));
#50701=CARTESIAN_POINT('Ctrl Pts',(85.4861282385094,-35.1517165484869,122.));
#50702=CARTESIAN_POINT('Ctrl Pts',(85.5333148151565,-35.0798800626262,122.));
#50703=CARTESIAN_POINT('Ctrl Pts',(85.584036314847,-35.0106370295489,122.));
#50704=CARTESIAN_POINT('Ctrl Pts',(85.6382598459827,-34.9443394496007,122.));
#50705=CARTESIAN_POINT('Ctrl Pts',(85.6870562587959,-34.8846774539338,122.));
#50706=CARTESIAN_POINT('Ctrl Pts',(85.7386893651034,-34.8274008880271,122.));
#50707=CARTESIAN_POINT('Ctrl Pts',(85.7931556859771,-34.772796091989,122.));
#50708=CARTESIAN_POINT('Ctrl Pts',(85.8122382584008,-34.7536650040366,122.));
#50709=CARTESIAN_POINT('Ctrl Pts',(85.8316687756141,-34.734862165088,122.));
#50710=CARTESIAN_POINT('Ctrl Pts',(85.8514366626951,-34.7163920625308,122.));
#50711=CARTESIAN_POINT('Origin',(87.7685555885722,-36.3549260746835,114.));
#50712=CARTESIAN_POINT('Origin',(-87.7685555885722,36.3549260746835,107.));
#50713=CARTESIAN_POINT('Ctrl Pts',(-89.6820215852368,37.9909132780591,107.));
#50714=CARTESIAN_POINT('Ctrl Pts',(-89.744159122969,37.9325192506103,107.));
#50715=CARTESIAN_POINT('Ctrl Pts',(-89.8029212860977,37.8708713145233,107.));
#50716=CARTESIAN_POINT('Ctrl Pts',(-89.8582960951973,37.8063459457027,107.));
#50717=CARTESIAN_POINT('Ctrl Pts',(-89.915025983506,37.7402415739533,107.));
#50718=CARTESIAN_POINT('Ctrl Pts',(-89.9682011734176,37.671116727705,107.));
#50719=CARTESIAN_POINT('Ctrl Pts',(-90.0177798965015,37.599329927726,107.));
#50720=CARTESIAN_POINT('Ctrl Pts',(-90.0307176306391,37.580596921409,107.));
#50721=CARTESIAN_POINT('Ctrl Pts',(-90.0434102865912,37.5616824282935,107.));
#50722=CARTESIAN_POINT('Ctrl Pts',(-90.0558567466988,37.5425923861499,107.));
#50723=CARTESIAN_POINT('Ctrl Pts',(-90.066026731285,37.5269939402728,107.));
#50724=CARTESIAN_POINT('Ctrl Pts',(-90.0760327837056,37.5112773814265,107.));
#50725=CARTESIAN_POINT('Ctrl Pts',(-90.0858654462594,37.4954605442615,107.));
#50726=CARTESIAN_POINT('Ctrl Pts',(-90.1333095652244,37.4191418564184,107.));
#50727=CARTESIAN_POINT('Ctrl Pts',(-90.1767701202724,37.3404158089311,107.));
#50728=CARTESIAN_POINT('Ctrl Pts',(-90.21621242528,37.2596749530829,107.));
#50729=CARTESIAN_POINT('Ctrl Pts',(-90.2480408931,37.1945200963464,107.));
#50730=CARTESIAN_POINT('Ctrl Pts',(-90.2772522211522,37.1280521304697,107.));
#50731=CARTESIAN_POINT('Ctrl Pts',(-90.3038110239626,37.0604595287346,107.));
#50732=CARTESIAN_POINT('Ctrl Pts',(-90.3144125005572,37.0334785917407,107.));
#50733=CARTESIAN_POINT('Ctrl Pts',(-90.3245911491353,37.0063183070948,107.));
#50734=CARTESIAN_POINT('Ctrl Pts',(-90.3343439585311,36.9789901163685,107.));
#50735=CARTESIAN_POINT('Ctrl Pts',(-90.3395848995591,36.9643045596036,107.));
#50736=CARTESIAN_POINT('Ctrl Pts',(-90.3447024891032,36.9495713342223,107.));
#50737=CARTESIAN_POINT('Ctrl Pts',(-90.3496922602842,36.934804694045,107.));
#50738=CARTESIAN_POINT('Ctrl Pts',(-90.3792310648457,36.8473880806567,107.));
#50739=CARTESIAN_POINT('Ctrl Pts',(-90.4043344064517,36.7586903635531,107.));
#50740=CARTESIAN_POINT('Ctrl Pts',(-90.4249697169135,36.6691093523015,107.));
#50741=CARTESIAN_POINT('Ctrl Pts',(-90.4459264940065,36.5781328056661,107.));
#50742=CARTESIAN_POINT('Ctrl Pts',(-90.4622754461125,36.486244424327,107.));
#50743=CARTESIAN_POINT('Ctrl Pts',(-90.4739406340489,36.393827715093,107.));
#50744=CARTESIAN_POINT('Ctrl Pts',(-90.4855151071126,36.3021296886663,107.));
#50745=CARTESIAN_POINT('Ctrl Pts',(-90.4924787239518,36.209910589573,107.));
#50746=CARTESIAN_POINT('Ctrl Pts',(-90.4947103587392,36.1175258369092,107.));
#50747=CARTESIAN_POINT('Ctrl Pts',(-90.4958209757943,36.0715487431124,107.));
#50748=CARTESIAN_POINT('Ctrl Pts',(-90.4957588348561,36.0255304079173,107.));
#50749=CARTESIAN_POINT('Ctrl Pts',(-90.4945042077797,35.9795139417161,107.));
#50750=CARTESIAN_POINT('Ctrl Pts',(-90.4941344323082,35.9659515367551,107.));
#50751=CARTESIAN_POINT('Ctrl Pts',(-90.4936610488672,35.9523892934637,107.));
#50752=CARTESIAN_POINT('Ctrl Pts',(-90.4930834960119,35.9388283155341,107.));
#50753=CARTESIAN_POINT('Ctrl Pts',(-90.4924629860478,35.9242587019428,107.));
#50754=CARTESIAN_POINT('Ctrl Pts',(-90.4917226371359,35.9097003351427,107.));
#50755=CARTESIAN_POINT('Ctrl Pts',(-90.4908624008004,35.895157143613,107.));
#50756=CARTESIAN_POINT('Ctrl Pts',(-90.4852105919944,35.7996074271386,107.));
#50757=CARTESIAN_POINT('Ctrl Pts',(-90.4743861465461,35.7046794298511,107.));
#50758=CARTESIAN_POINT('Ctrl Pts',(-90.4583186096772,35.6107687957121,107.));
#50759=CARTESIAN_POINT('Ctrl Pts',(-90.455938277629,35.5968563650806,107.));
#50760=CARTESIAN_POINT('Ctrl Pts',(-90.4534427880579,35.5829662291446,107.));
#50761=CARTESIAN_POINT('Ctrl Pts',(-90.4508318193706,35.5690996435893,107.));
#50762=CARTESIAN_POINT('Ctrl Pts',(-90.4338861650802,35.4791030204387,107.));
#50763=CARTESIAN_POINT('Ctrl Pts',(-90.4120806288724,35.3900985715579,107.));
#50764=CARTESIAN_POINT('Ctrl Pts',(-90.3857177602916,35.3023185449965,107.));
#50765=CARTESIAN_POINT('Ctrl Pts',(-90.3587589471203,35.2125542111576,107.));
#50766=CARTESIAN_POINT('Ctrl Pts',(-90.3270342224501,35.1240695823419,107.));
#50767=CARTESIAN_POINT('Ctrl Pts',(-90.2908128794366,35.0371167032257,107.));
#50768=CARTESIAN_POINT('Ctrl Pts',(-90.2783227526108,35.0071329312927,107.));
#50769=CARTESIAN_POINT('Ctrl Pts',(-90.2652974999059,34.9773313750936,107.));
#50770=CARTESIAN_POINT('Ctrl Pts',(-90.2517467909923,34.9477227085599,107.));
#50771=CARTESIAN_POINT('Ctrl Pts',(-90.2450557286484,34.9331025558462,107.));
#50772=CARTESIAN_POINT('Ctrl Pts',(-90.2382365401799,34.9185294366221,107.));
#50773=CARTESIAN_POINT('Ctrl Pts',(-90.2312903305009,34.9040046584706,107.));
#50774=CARTESIAN_POINT('Ctrl Pts',(-90.2257965562483,34.8925169758462,107.));
#50775=CARTESIAN_POINT('Ctrl Pts',(-90.2202237670946,34.8810605569674,107.));
#50776=CARTESIAN_POINT('Ctrl Pts',(-90.2145771037702,34.8696449781357,107.));
#50777=CARTESIAN_POINT('Ctrl Pts',(-90.1718531587215,34.7832721000849,107.));
#50778=CARTESIAN_POINT('Ctrl Pts',(-90.124838355933,34.6990975417634,107.));
#50779=CARTESIAN_POINT('Ctrl Pts',(-90.0738753505963,34.6173709404504,107.));
#50780=CARTESIAN_POINT('Ctrl Pts',(-90.0219016348831,34.5340235178487,107.));
#50781=CARTESIAN_POINT('Ctrl Pts',(-89.965821246638,34.453221340495,107.));
#50782=CARTESIAN_POINT('Ctrl Pts',(-89.9059426250489,34.3752362239655,107.));
#50783=CARTESIAN_POINT('Ctrl Pts',(-89.845577174311,34.2966170676586,107.));
#50784=CARTESIAN_POINT('Ctrl Pts',(-89.7813510190625,34.2208601285459,107.));
#50785=CARTESIAN_POINT('Ctrl Pts',(-89.7135308517992,34.1482631856065,107.));
#50786=CARTESIAN_POINT('Ctrl Pts',(-89.676530180774,34.1086564475,107.));
#50787=CARTESIAN_POINT('Ctrl Pts',(-89.6384589463324,34.0699906809862,107.));
#50788=CARTESIAN_POINT('Ctrl Pts',(-89.5993551074488,34.0323180201534,107.));
#50789=CARTESIAN_POINT('Ctrl Pts',(-89.587387522292,34.0207884417418,107.));
#50790=CARTESIAN_POINT('Ctrl Pts',(-89.5753231944213,34.0093519042645,107.));
#50791=CARTESIAN_POINT('Ctrl Pts',(-89.5631631489415,33.9980099642189,107.));
#50792=CARTESIAN_POINT('Ctrl Pts',(-89.5526173715299,33.9881736872628,107.));
#50793=CARTESIAN_POINT('Ctrl Pts',(-89.5420007164926,33.9784096758184,107.));
#50794=CARTESIAN_POINT('Ctrl Pts',(-89.5313229644313,33.9687269234992,107.));
#50795=CARTESIAN_POINT('Ctrl Pts',(-89.4557484807192,33.9001948014544,107.));
#50796=CARTESIAN_POINT('Ctrl Pts',(-89.3769972770167,33.8356190256038,107.));
#50797=CARTESIAN_POINT('Ctrl Pts',(-89.2953966997877,33.7752813677694,107.));
#50798=CARTESIAN_POINT('Ctrl Pts',(-89.2136919343842,33.7148666704013,107.));
#50799=CARTESIAN_POINT('Ctrl Pts',(-89.1291299412249,33.6587000819157,107.));
#50800=CARTESIAN_POINT('Ctrl Pts',(-89.0419940478043,33.6070902548594,107.));
#50801=CARTESIAN_POINT('Ctrl Pts',(-88.9565903904741,33.5565064160789,107.));
#50802=CARTESIAN_POINT('Ctrl Pts',(-88.8687134883914,33.5102992875464,107.));
#50803=CARTESIAN_POINT('Ctrl Pts',(-88.7785960158935,33.4687952816358,107.));
#50804=CARTESIAN_POINT('Ctrl Pts',(-88.7382467607252,33.4502122513025,107.));
#50805=CARTESIAN_POINT('Ctrl Pts',(-88.6974479330077,33.4325726088462,107.));
#50806=CARTESIAN_POINT('Ctrl Pts',(-88.6562186636994,33.4159086000809,107.));
#50807=CARTESIAN_POINT('Ctrl Pts',(-88.625799021521,33.4036136166285,107.));
#50808=CARTESIAN_POINT('Ctrl Pts',(-88.5951450346788,33.3918497860248,107.));
#50809=CARTESIAN_POINT('Ctrl Pts',(-88.5642689721408,33.3806144275731,107.));
#50810=CARTESIAN_POINT('Ctrl Pts',(-86.97475630604,33.3857031209377,107.));
#50811=CARTESIAN_POINT('Ctrl Pts',(-86.8799223806133,33.4203937944791,107.));
#50812=CARTESIAN_POINT('Ctrl Pts',(-86.7871316088213,33.4600753465665,107.));
#50813=CARTESIAN_POINT('Ctrl Pts',(-86.6966249142161,33.5044274278858,107.));
#50814=CARTESIAN_POINT('Ctrl Pts',(-86.6048453543519,33.5494032666378,107.));
#50815=CARTESIAN_POINT('Ctrl Pts',(-86.5154139004472,33.5991826306842,107.));
#50816=CARTESIAN_POINT('Ctrl Pts',(-86.4286158090018,33.6534721466289,107.));
#50817=CARTESIAN_POINT('Ctrl Pts',(-86.4041027850013,33.6688042833748,107.));
#50818=CARTESIAN_POINT('Ctrl Pts',(-86.3798000322781,33.6844963498378,107.));
#50819=CARTESIAN_POINT('Ctrl Pts',(-86.355714572459,33.7005421935948,107.));
#50820=CARTESIAN_POINT('Ctrl Pts',(-86.3363850476719,33.7134196116288,107.));
#50821=CARTESIAN_POINT('Ctrl Pts',(-86.3171933703453,33.7265265126986,107.));
#50822=CARTESIAN_POINT('Ctrl Pts',(-86.2981624559498,33.7398459518088,107.));
#50823=CARTESIAN_POINT('Ctrl Pts',(-86.2154553522762,33.7977313591239,107.));
#50824=CARTESIAN_POINT('Ctrl Pts',(-86.135703107737,33.8596789089563,107.));
#50825=CARTESIAN_POINT('Ctrl Pts',(-86.0591720841681,33.9253912417443,107.));
#50826=CARTESIAN_POINT('Ctrl Pts',(-86.0001788915497,33.9760449521586,107.));
#50827=CARTESIAN_POINT('Ctrl Pts',(-85.9431003663192,34.0289365876881,107.));
#50828=CARTESIAN_POINT('Ctrl Pts',(-85.8880760765311,34.0839417185279,107.));
#50829=CARTESIAN_POINT('Ctrl Pts',(-85.8587873250428,34.1132202719441,107.));
#50830=CARTESIAN_POINT('Ctrl Pts',(-85.8300808768359,34.1430977911502,107.));
#50831=CARTESIAN_POINT('Ctrl Pts',(-85.8019798022141,34.1735563417783,107.));
#50832=CARTESIAN_POINT('Ctrl Pts',(-85.7923437973743,34.1840007374187,107.));
#50833=CARTESIAN_POINT('Ctrl Pts',(-85.7827797082033,34.1945127449497,107.));
#50834=CARTESIAN_POINT('Ctrl Pts',(-85.7732951013283,34.205084028674,107.));
#50835=CARTESIAN_POINT('Ctrl Pts',(-85.7074979076647,34.2784197832977,107.));
#50836=CARTESIAN_POINT('Ctrl Pts',(-85.6454328643358,34.354702161135,107.));
#50837=CARTESIAN_POINT('Ctrl Pts',(-85.5873437401534,34.4336526051709,107.));
#50838=CARTESIAN_POINT('Ctrl Pts',(-85.5297810737241,34.5118875267408,107.));
#50839=CARTESIAN_POINT('Ctrl Pts',(-85.4761221521735,34.5927431572512,107.));
#50840=CARTESIAN_POINT('Ctrl Pts',(-85.4266499196299,34.6759708305421,107.));
#50841=CARTESIAN_POINT('Ctrl Pts',(-85.3785919815987,34.7568192208378,107.));
#50842=CARTESIAN_POINT('Ctrl Pts',(-85.33448457069,34.839906669308,107.));
#50843=CARTESIAN_POINT('Ctrl Pts',(-85.2946348383161,34.9250155558773,107.));
#50844=CARTESIAN_POINT('Ctrl Pts',(-85.2738304203819,34.9694484978478,107.));
#50845=CARTESIAN_POINT('Ctrl Pts',(-85.2541872885939,35.0144325101597,107.));
#50846=CARTESIAN_POINT('Ctrl Pts',(-85.2357548431069,35.0599368622838,107.));
#50847=CARTESIAN_POINT('Ctrl Pts',(-85.2286967575318,35.0773612247515,107.));
#50848=CARTESIAN_POINT('Ctrl Pts',(-85.2218162315165,35.0948618808238,107.));
#50849=CARTESIAN_POINT('Ctrl Pts',(-85.2151162006499,35.1124370963924,107.));
#50850=CARTESIAN_POINT('Ctrl Pts',(-85.2098744667648,35.1261869737912,107.));
#50851=CARTESIAN_POINT('Ctrl Pts',(-85.2047431089301,35.1399829871612,107.));
#50852=CARTESIAN_POINT('Ctrl Pts',(-85.1997286623157,35.1538095932101,107.));
#50853=CARTESIAN_POINT('Ctrl Pts',(-85.1680449784376,35.2411727359168,107.));
#50854=CARTESIAN_POINT('Ctrl Pts',(-85.1409701200769,35.329896826678,107.));
#50855=CARTESIAN_POINT('Ctrl Pts',(-85.1187553434742,35.419758315364,107.));
#50856=CARTESIAN_POINT('Ctrl Pts',(-85.1137713688799,35.4399191022416,107.));
#50857=CARTESIAN_POINT('Ctrl Pts',(-85.1090322283903,35.4601371793599,107.));
#50858=CARTESIAN_POINT('Ctrl Pts',(-85.1045411201527,35.4804100777641,107.));
#50859=CARTESIAN_POINT('Ctrl Pts',(-85.0841753696162,35.5723412381177,107.));
#50860=CARTESIAN_POINT('Ctrl Pts',(-85.0689058325994,35.6654000254775,107.));
#50861=CARTESIAN_POINT('Ctrl Pts',(-85.058622683849,35.7591948516197,107.));
#50862=CARTESIAN_POINT('Ctrl Pts',(-85.0478888270477,35.8571006834755,107.));
#50863=CARTESIAN_POINT('Ctrl Pts',(-85.0425880547018,35.9558097265016,107.));
#50864=CARTESIAN_POINT('Ctrl Pts',(-85.0426529193585,36.054861962213,107.));
#50865=CARTESIAN_POINT('Ctrl Pts',(-85.0426782913636,36.0936065414948,107.));
#50866=CARTESIAN_POINT('Ctrl Pts',(-85.0435252085663,36.1324033726805,107.));
#50867=CARTESIAN_POINT('Ctrl Pts',(-85.0451918583437,36.1712236979182,107.));
#50868=CARTESIAN_POINT('Ctrl Pts',(-85.0457248984063,36.1836394968929,107.));
#50869=CARTESIAN_POINT('Ctrl Pts',(-85.0463417849372,36.1960563877264,107.));
#50870=CARTESIAN_POINT('Ctrl Pts',(-85.0470417568095,36.2084637610652,107.));
#50871=CARTESIAN_POINT('Ctrl Pts',(-85.0522809798664,36.3013317733989,107.));
#50872=CARTESIAN_POINT('Ctrl Pts',(-85.0621766244509,36.3938165570659,107.));
#50873=CARTESIAN_POINT('Ctrl Pts',(-85.0766052312734,36.4855465333652,107.));
#50874=CARTESIAN_POINT('Ctrl Pts',(-85.0909998491431,36.5770604246414,107.));
#50875=CARTESIAN_POINT('Ctrl Pts',(-85.1099065080408,36.6678240058344,107.));
#50876=CARTESIAN_POINT('Ctrl Pts',(-85.1332512951455,36.7574513655987,107.));
#50877=CARTESIAN_POINT('Ctrl Pts',(-85.1561999302651,36.8455577838216,107.));
#50878=CARTESIAN_POINT('Ctrl Pts',(-85.1834378124742,36.9325670012153,107.));
#50879=CARTESIAN_POINT('Ctrl Pts',(-85.2149351692827,37.0180833239309,107.));
#50880=CARTESIAN_POINT('Ctrl Pts',(-85.2307766169503,37.0610933567811,107.));
#50881=CARTESIAN_POINT('Ctrl Pts',(-85.2476961145767,37.1037252212997,107.));
#50882=CARTESIAN_POINT('Ctrl Pts',(-85.265693291879,37.1459247860001,107.));
#50883=CARTESIAN_POINT('Ctrl Pts',(-85.2712589937397,37.158975176727,107.));
#50884=CARTESIAN_POINT('Ctrl Pts',(-85.2769277783773,37.1719842023805,107.));
#50885=CARTESIAN_POINT('Ctrl Pts',(-85.2826996757167,37.184950204339,107.));
#50886=CARTESIAN_POINT('Ctrl Pts',(-85.2883791458889,37.1977085777205,107.));
#50887=CARTESIAN_POINT('Ctrl Pts',(-85.2941549715906,37.2104174298264,107.));
#50888=CARTESIAN_POINT('Ctrl Pts',(-85.3000253630705,37.2230722749883,107.));
#50889=CARTESIAN_POINT('Ctrl Pts',(-85.3375051695688,37.3038677635949,107.));
#50890=CARTESIAN_POINT('Ctrl Pts',(-85.3788551320423,37.382506472753,107.));
#50891=CARTESIAN_POINT('Ctrl Pts',(-85.4240055740443,37.4586408101418,107.));
#50892=CARTESIAN_POINT('Ctrl Pts',(-85.4683985786282,37.5334979286735,107.));
#50893=CARTESIAN_POINT('Ctrl Pts',(-85.5164660737889,37.6059346660804,107.));
#50894=CARTESIAN_POINT('Ctrl Pts',(-85.5681780442174,37.6755864543237,107.));
#50895=CARTESIAN_POINT('Ctrl Pts',(-85.6183124904752,37.7431134467302,107.));
#50896=CARTESIAN_POINT('Ctrl Pts',(-85.6718728898827,37.8080232545947,107.));
#50897=CARTESIAN_POINT('Ctrl Pts',(-85.7288596017871,37.8699433823759,107.));
#50898=CARTESIAN_POINT('Ctrl Pts',(-85.7498272219443,37.892726197457,107.));
#50899=CARTESIAN_POINT('Ctrl Pts',(-85.7712589370451,37.915103838407,107.));
#50900=CARTESIAN_POINT('Ctrl Pts',(-85.7931555761837,37.9370561406484,107.));
#50901=CARTESIAN_POINT('Ctrl Pts',(-85.8122330129516,37.9561820738691,107.));
#50902=CARTESIAN_POINT('Ctrl Pts',(-85.8316633830167,37.9749851198425,107.));
#50903=CARTESIAN_POINT('Ctrl Pts',(-85.8514365495281,37.9934601500705,107.));
#50904=CARTESIAN_POINT('Origin',(-87.7685555885722,36.3549260746835,124.208423447177));
#50905=CARTESIAN_POINT('Ctrl Pts',(-90.8453550251768,36.3568536361305,121.708423447177));
#50906=CARTESIAN_POINT('Ctrl Pts',(-90.8462777110879,36.4801285286213,121.702019850418));
#50907=CARTESIAN_POINT('Ctrl Pts',(-90.783751283825,37.6160352592255,121.642966745928));
#50908=CARTESIAN_POINT('Ctrl Pts',(-89.371024227111,39.6084645019137,121.531264133707));
#50909=CARTESIAN_POINT('Ctrl Pts',(-85.9203582871986,39.4750890566271,121.373315610515));
#50910=CARTESIAN_POINT('Ctrl Pts',(-84.1454682646258,36.5131478641077,121.215367087322));
#50911=CARTESIAN_POINT('Ctrl Pts',(-85.6554864948497,33.4075615942697,121.05741856413));
#50912=CARTESIAN_POINT('Ctrl Pts',(-89.0813771440687,32.974353542169,120.899470040937));
#50913=CARTESIAN_POINT('Ctrl Pts',(-90.7279240557369,34.9127247019801,120.783138335286));
#50914=CARTESIAN_POINT('Ctrl Pts',(-90.8448016801335,36.1393664148291,120.719456137367));
#50915=CARTESIAN_POINT('Ctrl Pts',(-90.84286984995,36.3522423553315,120.708423447177));
#50916=CARTESIAN_POINT('Ctrl Pts',(-90.8388342008425,36.3519111454271,121.791576552823));
#50917=CARTESIAN_POINT('Ctrl Pts',(-90.833849270346,37.0449295945579,121.755752019753));
#50918=CARTESIAN_POINT('Ctrl Pts',(-90.2614619032149,38.7661192425051,121.667277978953));
#50919=CARTESIAN_POINT('Ctrl Pts',(-87.4170212212397,39.9637875212778,121.526154430423));
#50920=CARTESIAN_POINT('Ctrl Pts',(-84.554628466517,38.0346655247349,121.36820590723));
#50921=CARTESIAN_POINT('Ctrl Pts',(-84.6050188146032,34.5813834739332,121.210257384038));
#50922=CARTESIAN_POINT('Ctrl Pts',(-87.5242687556742,32.7366979528604,121.052308860845));
#50923=CARTESIAN_POINT('Ctrl Pts',(-90.2991159873621,34.0051401442305,120.912748583773));
#50924=CARTESIAN_POINT('Ctrl Pts',(-90.8346457908973,35.6938776421048,120.825837814433));
#50925=CARTESIAN_POINT('Ctrl Pts',(-90.8389970126702,36.3570769587632,120.791576552823));
#50926=CARTESIAN_POINT('Ctrl Pts',(-85.855089591907,37.9909132780583,122.));
#50927=CARTESIAN_POINT('Ctrl Pts',(-85.3138942055855,37.3579260718368,121.947350492269));
#50928=CARTESIAN_POINT('Ctrl Pts',(-84.918555104032,35.5228952161373,121.842051476807));
#50929=CARTESIAN_POINT('Ctrl Pts',(-86.9093551045068,33.5097261262742,121.684102953615));
#50930=CARTESIAN_POINT('Ctrl Pts',(-89.6802575115698,34.0819713092507,121.526154430423));
#50931=CARTESIAN_POINT('Ctrl Pts',(-90.7173747371113,36.7122375197466,121.36820590723));
#50932=CARTESIAN_POINT('Ctrl Pts',(-89.0811356430773,39.0198953249038,121.210257384038));
#50933=CARTESIAN_POINT('Ctrl Pts',(-86.2546994941495,38.9106476647415,121.052308860845));
#50934=CARTESIAN_POINT('Ctrl Pts',(-84.8008892999648,36.4845253442053,120.894360337653));
#50935=CARTESIAN_POINT('Ctrl Pts',(-86.0377433408264,33.9407435207737,120.73641181446));
#50936=CARTESIAN_POINT('Ctrl Pts',(-88.843886080182,33.5859033479533,120.578463291268));
#50937=CARTESIAN_POINT('Ctrl Pts',(-90.675052621233,35.7416150296742,120.420514768075));
#50938=CARTESIAN_POINT('Ctrl Pts',(-89.8709899803276,38.4534150947004,120.262566244883));
#50939=CARTESIAN_POINT('Ctrl Pts',(-87.1607124239154,39.2625702781167,120.10461772169));
#50940=CARTESIAN_POINT('Ctrl Pts',(-85.0015485538449,37.4354571295292,119.946669198498));
#50941=CARTESIAN_POINT('Ctrl Pts',(-85.3511454302727,34.6286572769424,119.788720675305));
#50942=CARTESIAN_POINT('Ctrl Pts',(-87.8925347584294,33.3870138425999,119.630772152113));
#50943=CARTESIAN_POINT('Ctrl Pts',(-90.3215158547498,34.8362856771634,119.472823628921));
#50944=CARTESIAN_POINT('Ctrl Pts',(-90.4358055658698,37.6624628095854,119.314875105728));
#50945=CARTESIAN_POINT('Ctrl Pts',(-88.131780822228,39.3031360362638,119.156926582536));
#50946=CARTESIAN_POINT('Ctrl Pts',(-85.4984308164805,38.2707570125183,118.998978059343));
#50947=CARTESIAN_POINT('Ctrl Pts',(-84.9233338938786,35.5013523175772,118.841029536151));
#50948=CARTESIAN_POINT('Ctrl Pts',(-86.9279129507738,33.5058570011705,118.683081012958));
#50949=CARTESIAN_POINT('Ctrl Pts',(-89.6946771191916,34.0935259567618,118.525132489766));
#50950=CARTESIAN_POINT('Ctrl Pts',(-90.7150854767087,36.7315376250273,118.367183966573));
#50951=CARTESIAN_POINT('Ctrl Pts',(-89.0639647990291,39.0280870531966,118.209235443381));
#50952=CARTESIAN_POINT('Ctrl Pts',(-86.2383359884542,38.9009627234043,118.051286920188));
#50953=CARTESIAN_POINT('Ctrl Pts',(-84.8001107497149,36.4654243980613,117.893338396996));
#50954=CARTESIAN_POINT('Ctrl Pts',(-86.053284165231,33.9297006037413,117.735389873803));
#50955=CARTESIAN_POINT('Ctrl Pts',(-88.8616420126528,33.5928549839411,117.577441350611));
#50956=CARTESIAN_POINT('Ctrl Pts',(-90.6789316440892,35.7602952175635,117.419492827418));
#50957=CARTESIAN_POINT('Ctrl Pts',(-89.8574718210711,38.4668691644366,117.261544304226));
#50958=CARTESIAN_POINT('Ctrl Pts',(-87.1420551815635,39.2586085436859,117.103595781033));
#50959=CARTESIAN_POINT('Ctrl Pts',(-84.9946674069412,37.4176673397963,116.945647257841));
#50960=CARTESIAN_POINT('Ctrl Pts',(-85.3622796826088,34.6131709526458,116.787698734649));
#50961=CARTESIAN_POINT('Ctrl Pts',(-87.9115891386397,33.3878709615584,116.629750211456));
#50962=CARTESIAN_POINT('Ctrl Pts',(-90.3312144249933,34.8527096026399,116.471801688264));
#50963=CARTESIAN_POINT('Ctrl Pts',(-90.4273548841092,37.6795622310744,116.313853165071));
#50964=CARTESIAN_POINT('Ctrl Pts',(-88.1128428856871,39.305407543497,116.155904641879));
#50965=CARTESIAN_POINT('Ctrl Pts',(-85.4861760659956,38.2561410429839,115.997956118686));
#50966=CARTESIAN_POINT('Ctrl Pts',(-84.9288733439891,35.4831007535523,115.840007595494));
#50967=CARTESIAN_POINT('Ctrl Pts',(-86.9462241481147,33.5005179674218,115.682059072301));
#50968=CARTESIAN_POINT('Ctrl Pts',(-89.7091578592229,34.1059401992473,115.524110549109));
#50969=CARTESIAN_POINT('Ctrl Pts',(-90.7126065122823,36.7504495245173,115.366162025916));
#50970=CARTESIAN_POINT('Ctrl Pts',(-89.0467737320752,39.036349767125,115.208213502724));
#50971=CARTESIAN_POINT('Ctrl Pts',(-86.2220194364013,38.8910846996112,115.050264979531));
#50972=CARTESIAN_POINT('Ctrl Pts',(-84.7994624341302,36.4463617406534,114.892316456339));
#50973=CARTESIAN_POINT('Ctrl Pts',(-86.0688918941051,33.9187368442507,114.734367933146));
#50974=CARTESIAN_POINT('Ctrl Pts',(-88.879354732919,33.5999306297355,114.576419409954));
#50975=CARTESIAN_POINT('Ctrl Pts',(-90.6826897709824,35.7789949957557,114.418470886762));
#50976=CARTESIAN_POINT('Ctrl Pts',(-89.8438679752394,38.4802385548879,114.260522363569));
#50977=CARTESIAN_POINT('Ctrl Pts',(-87.1234235562783,39.254525926676,114.102573840377));
#50978=CARTESIAN_POINT('Ctrl Pts',(-84.9879007301944,37.3998343000056,113.944625317184));
#50979=CARTESIAN_POINT('Ctrl Pts',(-85.373513094407,34.5977561648829,113.786676793992));
#50980=CARTESIAN_POINT('Ctrl Pts',(-87.9306376461546,33.3888505450693,113.628728270799));
#50981=CARTESIAN_POINT('Ctrl Pts',(-90.3408073257951,34.8691953988476,113.470779747607));
#50982=CARTESIAN_POINT('Ctrl Pts',(-90.418794586796,37.6966070699504,113.312831224414));
#50983=CARTESIAN_POINT('Ctrl Pts',(-88.0938907514829,39.3075573880276,113.154882701222));
#50984=CARTESIAN_POINT('Ctrl Pts',(-85.4740154185804,38.2414466945179,112.996934178029));
#50985=CARTESIAN_POINT('Ctrl Pts',(-84.9345298725249,35.4648851309353,112.838985654837));
#50986=CARTESIAN_POINT('Ctrl Pts',(-86.9645692502135,33.4952966216777,112.681037131644));
#50987=CARTESIAN_POINT('Ctrl Pts',(-89.7235585887529,34.118447165762,112.523088608452));
#50988=CARTESIAN_POINT('Ctrl Pts',(-90.7100061657571,36.7693451171343,112.365140085259));
#50989=CARTESIAN_POINT('Ctrl Pts',(-89.029529964603,39.0445019267018,112.207191562067));
#50990=CARTESIAN_POINT('Ctrl Pts',(-86.2057666475039,38.8811021109965,112.049243038874));
#50991=CARTESIAN_POINT('Ctrl Pts',(-84.7989365331946,36.4272953133369,111.891294515682));
#50992=CARTESIAN_POINT('Ctrl Pts',(-86.0845696995146,33.907873528002,111.733345992489));
#50993=CARTESIAN_POINT('Ctrl Pts',(-88.8970216553292,33.6071198630027,111.575397469297));
#50994=CARTESIAN_POINT('Ctrl Pts',(-90.6863277491557,35.7977185193896,111.417448946105));
#50995=CARTESIAN_POINT('Ctrl Pts',(-89.8301785650173,38.4935203194527,111.259500422912));
#50996=CARTESIAN_POINT('Ctrl Pts',(-87.1048185295501,39.250323760202,111.10155189972));
#50997=CARTESIAN_POINT('Ctrl Pts',(-84.9812486988779,37.3819581790018,110.943603376527));
#50998=CARTESIAN_POINT('Ctrl Pts',(-85.3848452529235,34.5824138246471,110.785654853335));
#50999=CARTESIAN_POINT('Ctrl Pts',(-87.9496794711547,33.3899524187512,110.627706330142));
#51000=CARTESIAN_POINT('Ctrl Pts',(-90.3502941734241,34.8857424513509,110.46975780695));
#51001=CARTESIAN_POINT('Ctrl Pts',(-90.4101250213688,37.7135965914931,110.311809283757));
#51002=CARTESIAN_POINT('Ctrl Pts',(-88.0749252032079,39.3095854972364,110.153860760565));
#51003=CARTESIAN_POINT('Ctrl Pts',(-85.4619493755126,38.2266745642004,109.995912237372));
#51004=CARTESIAN_POINT('Ctrl Pts',(-84.9403032443241,35.4467062070136,109.83796371418));
#51005=CARTESIAN_POINT('Ctrl Pts',(-86.9829475057552,33.4901931720481,109.680015190987));
#51006=CARTESIAN_POINT('Ctrl Pts',(-89.7378787031565,34.1310463526011,109.522066667795));
#51007=CARTESIAN_POINT('Ctrl Pts',(-90.7072845669837,36.7882236005902,109.364118144602));
#51008=CARTESIAN_POINT('Ctrl Pts',(-89.0122341608886,39.0525432429309,109.20616962141));
#51009=CARTESIAN_POINT('Ctrl Pts',(-86.1895783879121,38.871015272567,109.048221098218));
#51010=CARTESIAN_POINT('Ctrl Pts',(-84.7985328710269,36.4082261006589,108.890272575025));
#51011=CARTESIAN_POINT('Ctrl Pts',(-86.1003173413752,33.8971106948583,108.732324051833));
#51012=CARTESIAN_POINT('Ctrl Pts',(-88.9146412159036,33.6144232264086,108.57437552864));
#51013=CARTESIAN_POINT('Ctrl Pts',(-90.6898471469939,35.8164632909541,108.416427005448));
#51014=CARTESIAN_POINT('Ctrl Pts',(-89.8164006209573,38.5067174591193,108.258478482255));
#51015=CARTESIAN_POINT('Ctrl Pts',(-87.0862481358614,39.2459949198183,108.100529959063));
#51016=CARTESIAN_POINT('Ctrl Pts',(-84.9746966417824,37.3640547215823,107.94258143587));
#51017=CARTESIAN_POINT('Ctrl Pts',(-85.3963064264104,34.5671137009093,107.784632912678));
#51018=CARTESIAN_POINT('Ctrl Pts',(-87.9686506208259,33.391240008553,107.626684389485));
#51019=CARTESIAN_POINT('Ctrl Pts',(-90.3598045645273,34.9022195493604,107.468735866293));
#51020=CARTESIAN_POINT('Ctrl Pts',(-90.4010792246134,37.7307985779511,107.3107873431));
#51021=CARTESIAN_POINT('Ctrl Pts',(-88.0564969445425,39.3109398404868,107.152838819908));
#51022=CARTESIAN_POINT('Ctrl Pts',(-85.4488474513176,38.2129740762705,106.994890296715));
#51023=CARTESIAN_POINT('Ctrl Pts',(-84.9485678262205,35.4262457574378,106.836941773523));
#51024=CARTESIAN_POINT('Ctrl Pts',(-86.3138051921105,34.137929732014,106.731642758061));
#51025=CARTESIAN_POINT('Ctrl Pts',(-87.1183555905977,33.9228392726483,106.678993250331));
#51026=CARTESIAN_POINT('Ctrl Pts',(-85.71422403823,38.1113513959102,122.10700224989));
#51027=CARTESIAN_POINT('Ctrl Pts',(-85.133186926017,37.4317649329314,122.054352742159));
#51028=CARTESIAN_POINT('Ctrl Pts',(-84.7087437476064,35.4616427623337,121.949053726697));
#51029=CARTESIAN_POINT('Ctrl Pts',(-86.8461024770139,33.3002681757525,121.791105203505));
#51030=CARTESIAN_POINT('Ctrl Pts',(-89.8209931976587,33.9146409087766,121.633156680313));
#51031=CARTESIAN_POINT('Ctrl Pts',(-90.9344609266627,36.7385420763113,121.47520815712));
#51032=CARTESIAN_POINT('Ctrl Pts',(-89.1777651710886,39.2160850505738,121.317259633928));
#51033=CARTESIAN_POINT('Ctrl Pts',(-86.1432524251657,39.09879479537,121.159311110735));
#51034=CARTESIAN_POINT('Ctrl Pts',(-84.5824156215186,36.4940661841728,121.001362587543));
#51035=CARTESIAN_POINT('Ctrl Pts',(-85.9103243921675,33.763016211939,120.84341406435));
#51036=CARTESIAN_POINT('Ctrl Pts',(-88.9230497681442,33.3820534126919,120.685465541158));
#51037=CARTESIAN_POINT('Ctrl Pts',(-90.8890231409496,35.6964642926964,120.527517017965));
#51038=CARTESIAN_POINT('Ctrl Pts',(-90.0257670106906,38.6079016746579,120.369568494773));
#51039=CARTESIAN_POINT('Ctrl Pts',(-87.1159642213932,39.4766252502595,120.21161997158));
#51040=CARTESIAN_POINT('Ctrl Pts',(-84.797847009812,37.5150036725937,120.053671448388));
#51041=CARTESIAN_POINT('Ctrl Pts',(-85.1731805116345,34.501572808019,119.895722925195));
#51042=CARTESIAN_POINT('Ctrl Pts',(-87.9016618578588,33.168522058285,119.737774402003));
#51043=CARTESIAN_POINT('Ctrl Pts',(-90.5094597022168,34.7244863973195,119.57982587881));
#51044=CARTESIAN_POINT('Ctrl Pts',(-90.6321631941225,37.7587210584574,119.421877355618));
#51045=CARTESIAN_POINT('Ctrl Pts',(-88.1585207401243,39.5201773786853,119.263928832425));
#51046=CARTESIAN_POINT('Ctrl Pts',(-85.3313087544768,38.4117966684516,119.105980309233));
#51047=CARTESIAN_POINT('Ctrl Pts',(-84.7138743424387,35.4385139185105,118.94803178604));
#51048=CARTESIAN_POINT('Ctrl Pts',(-86.8660265149425,33.2961142133687,118.790083262848));
#51049=CARTESIAN_POINT('Ctrl Pts',(-89.8364743480595,33.9270461864123,118.632134739655));
#51050=CARTESIAN_POINT('Ctrl Pts',(-90.9320031354711,36.7592630168832,118.474186216463));
#51051=CARTESIAN_POINT('Ctrl Pts',(-89.1593302437182,39.2248798375797,118.316237693271));
#51052=CARTESIAN_POINT('Ctrl Pts',(-86.1256842707891,39.088396867951,118.158289170078));
#51053=CARTESIAN_POINT('Ctrl Pts',(-84.5815797559506,36.4735590644364,118.000340646886));
#51054=CARTESIAN_POINT('Ctrl Pts',(-85.9270093010962,33.7511603373601,117.842392123693));
#51055=CARTESIAN_POINT('Ctrl Pts',(-88.942112856981,33.3895168142684,117.684443600501));
#51056=CARTESIAN_POINT('Ctrl Pts',(-90.8931877297387,35.7165196787937,117.526495077308));
#51057=CARTESIAN_POINT('Ctrl Pts',(-90.0112536714875,38.6223462061979,117.368546554116));
#51058=CARTESIAN_POINT('Ctrl Pts',(-87.095933470038,39.4723718608345,117.210598030923));
#51059=CARTESIAN_POINT('Ctrl Pts',(-84.7904592865855,37.4959042339906,117.052649507731));
#51060=CARTESIAN_POINT('Ctrl Pts',(-85.1851344454402,34.4849464113876,116.894700984538));
#51061=CARTESIAN_POINT('Ctrl Pts',(-87.9221189835702,33.1694422766331,116.736752461346));
#51062=CARTESIAN_POINT('Ctrl Pts',(-90.5198722618751,34.7421194194613,116.578803938153));
#51063=CARTESIAN_POINT('Ctrl Pts',(-90.6230903900105,37.7770793052821,116.420855414961));
#51064=CARTESIAN_POINT('Ctrl Pts',(-88.1381886304332,39.5226161097546,116.262906891769));
#51065=CARTESIAN_POINT('Ctrl Pts',(-85.3181518336815,38.3961047003655,116.104958368576));
#51066=CARTESIAN_POINT('Ctrl Pts',(-84.7198215958278,35.4189187107123,115.947009845384));
#51067=CARTESIAN_POINT('Ctrl Pts',(-86.8856857461426,33.2903821305947,115.789061322191));
#51068=CARTESIAN_POINT('Ctrl Pts',(-89.8520211313158,33.9403743406915,115.631112798999));
#51069=CARTESIAN_POINT('Ctrl Pts',(-90.9293416746237,36.7795671727275,115.473164275806));
#51070=CARTESIAN_POINT('Ctrl Pts',(-89.1408736046719,39.2337508360423,115.315215752614));
#51071=CARTESIAN_POINT('Ctrl Pts',(-86.1081665266886,39.0777916437303,115.157267229421));
#51072=CARTESIAN_POINT('Ctrl Pts',(-84.5808837126644,36.4530930521766,114.999318706229));
#51073=CARTESIAN_POINT('Ctrl Pts',(-85.9437660398683,33.7393894477435,114.841370183036));
#51074=CARTESIAN_POINT('Ctrl Pts',(-88.9611295524168,33.3971133550064,114.683421659844));
#51075=CARTESIAN_POINT('Ctrl Pts',(-90.8972225224448,35.7365960973931,114.525473136651));
#51076=CARTESIAN_POINT('Ctrl Pts',(-89.9966483376343,38.6366998245329,114.367524613459));
#51077=CARTESIAN_POINT('Ctrl Pts',(-87.0759302216267,39.4679886896959,114.209576090266));
#51078=CARTESIAN_POINT('Ctrl Pts',(-84.7831944605806,37.4767583613467,114.051627567074));
#51079=CARTESIAN_POINT('Ctrl Pts',(-85.1971948386299,34.4683968176668,113.893679043881));
#51080=CARTESIAN_POINT('Ctrl Pts',(-87.94256980425,33.1704939751301,113.735730520689));
#51081=CARTESIAN_POINT('Ctrl Pts',(-90.530171372918,34.7598188671343,113.577781997496));
#51082=CARTESIAN_POINT('Ctrl Pts',(-90.6138999006673,37.7953789512305,113.419833474304));
#51083=CARTESIAN_POINT('Ctrl Pts',(-88.1178412778752,39.5249242215556,113.261884951112));
#51084=CARTESIAN_POINT('Ctrl Pts',(-85.3050959436363,38.3803285832472,113.103936427919));
#51085=CARTESIAN_POINT('Ctrl Pts',(-84.7258945467225,35.3993620902569,112.945987904727));
#51086=CARTESIAN_POINT('Ctrl Pts',(-86.9053813781013,33.2847763997814,112.788039381534));
#51087=CARTESIAN_POINT('Ctrl Pts',(-89.8674820138573,33.9538020451582,112.630090858342));
#51088=CARTESIAN_POINT('Ctrl Pts',(-90.9265498957688,36.7998538212194,112.472142335149));
#51089=CARTESIAN_POINT('Ctrl Pts',(-89.1223603854006,39.2425031413621,112.314193811957));
#51090=CARTESIAN_POINT('Ctrl Pts',(-86.0907172398595,39.0670741568343,112.156245288764));
#51091=CARTESIAN_POINT('Ctrl Pts',(-84.5803190959501,36.4326229924751,111.998296765572));
#51092=CARTESIAN_POINT('Ctrl Pts',(-85.9605980140705,33.7277263958002,111.840348242379));
#51093=CARTESIAN_POINT('Ctrl Pts',(-88.9800970784496,33.4048318453007,111.682399719187));
#51094=CARTESIAN_POINT('Ctrl Pts',(-90.9011283213218,35.7566980095261,111.524451195994));
#51095=CARTESIAN_POINT('Ctrl Pts',(-89.9819511403106,38.6509593661381,111.366502672802));
#51096=CARTESIAN_POINT('Ctrl Pts',(-87.0559555299054,39.4634771680998,111.208554149609));
#51097=CARTESIAN_POINT('Ctrl Pts',(-84.7760527199742,37.4575662359367,111.050605626417));
#51098=CARTESIAN_POINT('Ctrl Pts',(-85.2093612480747,34.4519250049159,110.892657103225));
#51099=CARTESIAN_POINT('Ctrl Pts',(-87.9630134504616,33.1716769665567,110.734708580032));
#51100=CARTESIAN_POINT('Ctrl Pts',(-90.5403566233648,34.7775840806693,110.57676005684));
#51101=CARTESIAN_POINT('Ctrl Pts',(-90.6045920991094,37.8136192074939,110.418811533647));
#51102=CARTESIAN_POINT('Ctrl Pts',(-88.0974795237292,39.5271016361228,110.260863010455));
#51103=CARTESIAN_POINT('Ctrl Pts',(-85.2921416225221,38.3644689581323,110.102914487262));
#51104=CARTESIAN_POINT('Ctrl Pts',(-84.7320929426489,35.3798448701815,109.94496596407));
#51105=CARTESIAN_POINT('Ctrl Pts',(-86.9251126041933,33.2792972443598,109.787017440877));
#51106=CARTESIAN_POINT('Ctrl Pts',(-89.8828563465474,33.9673287590258,109.629068917685));
#51107=CARTESIAN_POINT('Ctrl Pts',(-90.9236279383172,36.8201221010078,109.471120394492));
#51108=CARTESIAN_POINT('Ctrl Pts',(-89.1037912990822,39.2511364432679,109.3131718713));
#51109=CARTESIAN_POINT('Ctrl Pts',(-86.0733372328554,39.0562447454598,109.155223348107));
#51110=CARTESIAN_POINT('Ctrl Pts',(-84.5798857169778,36.4121499423593,108.997274824915));
#51111=CARTESIAN_POINT('Ctrl Pts',(-85.9775049659444,33.7161712243276,108.839326301723));
#51112=CARTESIAN_POINT('Ctrl Pts',(-88.9990137559626,33.412672867767,108.68137777853));
#51113=CARTESIAN_POINT('Ctrl Pts',(-90.9049068102157,35.7768227338202,108.523429255338));
#51114=CARTESIAN_POINT('Ctrl Pts',(-89.9671588914646,38.6651280529288,108.365480732145));
#51115=CARTESIAN_POINT('Ctrl Pts',(-87.0360180208389,39.4588296471133,108.207532208953));
#51116=CARTESIAN_POINT('Ctrl Pts',(-84.7690183134918,37.4383447616585,108.04958368576));
#51117=CARTESIAN_POINT('Ctrl Pts',(-85.2216661703148,34.4354985165574,107.891635162568));
#51118=CARTESIAN_POINT('Ctrl Pts',(-87.9833812183675,33.1730593461539,107.733686639375));
#51119=CARTESIAN_POINT('Ctrl Pts',(-90.5505671505095,34.7952741898001,107.575738116183));
#51120=CARTESIAN_POINT('Ctrl Pts',(-90.5948803688225,37.8320875699162,107.41778959299));
#51121=CARTESIAN_POINT('Ctrl Pts',(-88.0776946133833,39.5285556834245,107.259841069798));
#51122=CARTESIAN_POINT('Ctrl Pts',(-85.2780751607762,38.3497598675822,107.101892546605));
#51123=CARTESIAN_POINT('Ctrl Pts',(-84.7409659465956,35.3578781630799,106.943944023413));
#51124=CARTESIAN_POINT('Ctrl Pts',(-86.2067093668298,33.9747188791143,106.838645007951));
#51125=CARTESIAN_POINT('Ctrl Pts',(-87.0704891624118,33.7437938887448,106.78599550022));
#51126=CARTESIAN_POINT('Ctrl Pts',(-85.573358484553,38.2317895137621,122.21400449978));
#51127=CARTESIAN_POINT('Ctrl Pts',(-84.9524796464486,37.505603794026,122.161354992049));
#51128=CARTESIAN_POINT('Ctrl Pts',(-84.4989323911808,35.4003903085301,122.056055976587));
#51129=CARTESIAN_POINT('Ctrl Pts',(-86.782849849521,33.0908102252307,121.898107453395));
#51130=CARTESIAN_POINT('Ctrl Pts',(-89.9617288837476,33.7473105083025,121.740158930202));
#51131=CARTESIAN_POINT('Ctrl Pts',(-91.1515471162143,36.764846632876,121.58221040701));
#51132=CARTESIAN_POINT('Ctrl Pts',(-89.2743946990997,39.4122747762438,121.424261883817));
#51133=CARTESIAN_POINT('Ctrl Pts',(-86.0318053561822,39.2869419259985,121.266313360625));
#51134=CARTESIAN_POINT('Ctrl Pts',(-84.3639419430722,36.5036070241402,121.108364837432));
#51135=CARTESIAN_POINT('Ctrl Pts',(-85.7829054435086,33.5852889031044,120.95041631424));
#51136=CARTESIAN_POINT('Ctrl Pts',(-89.0022134561064,33.1782034774305,120.792467791047));
#51137=CARTESIAN_POINT('Ctrl Pts',(-91.1029936606662,35.6513135557185,120.634519267855));
#51138=CARTESIAN_POINT('Ctrl Pts',(-90.1805440410535,38.7623882546154,120.476570744662));
#51139=CARTESIAN_POINT('Ctrl Pts',(-87.0712160188709,39.6906802224024,120.31862222147));
#51140=CARTESIAN_POINT('Ctrl Pts',(-84.5941454657791,37.5945502156581,120.160673698277));
#51141=CARTESIAN_POINT('Ctrl Pts',(-84.9952155929964,34.3744883390956,120.002725175085));
#51142=CARTESIAN_POINT('Ctrl Pts',(-87.9107889572882,32.9500302739701,119.844776651893));
#51143=CARTESIAN_POINT('Ctrl Pts',(-90.6974035496838,34.6126871174756,119.6868281287));
#51144=CARTESIAN_POINT('Ctrl Pts',(-90.8285208223751,37.8549793073293,119.528879605508));
#51145=CARTESIAN_POINT('Ctrl Pts',(-88.1852606580207,39.7372187211068,119.370931082315));
#51146=CARTESIAN_POINT('Ctrl Pts',(-85.1641866924731,38.5528363243849,119.212982559123));
#51147=CARTESIAN_POINT('Ctrl Pts',(-84.5044147909987,35.3756755194439,119.05503403593));
#51148=CARTESIAN_POINT('Ctrl Pts',(-86.8041400791112,33.0863714255669,118.897085512738));
#51149=CARTESIAN_POINT('Ctrl Pts',(-89.9782715769274,33.7605664160628,118.739136989545));
#51150=CARTESIAN_POINT('Ctrl Pts',(-91.1489207942337,36.786988408739,118.581188466353));
#51151=CARTESIAN_POINT('Ctrl Pts',(-89.2546956884071,39.4216726219628,118.42323994316));
#51152=CARTESIAN_POINT('Ctrl Pts',(-86.013032553124,39.2758310124976,118.265291419968));
#51153=CARTESIAN_POINT('Ctrl Pts',(-84.3630487621863,36.4816937308115,118.107342896775));
#51154=CARTESIAN_POINT('Ctrl Pts',(-85.8007344369615,33.5726200709789,117.949394373583));
#51155=CARTESIAN_POINT('Ctrl Pts',(-89.0225837013092,33.1861786445957,117.79144585039));
#51156=CARTESIAN_POINT('Ctrl Pts',(-91.1074438153881,35.6727441400239,117.633497327198));
#51157=CARTESIAN_POINT('Ctrl Pts',(-90.1650355219039,38.7778232479593,117.475548804006));
#51158=CARTESIAN_POINT('Ctrl Pts',(-87.0498117585123,39.6861351779832,117.317600280813));
#51159=CARTESIAN_POINT('Ctrl Pts',(-84.5862511662297,37.574141128185,117.159651757621));
#51160=CARTESIAN_POINT('Ctrl Pts',(-85.0079892082717,34.3567218701293,117.001703234428));
#51161=CARTESIAN_POINT('Ctrl Pts',(-87.9326488285006,32.9510135917079,116.843754711236));
#51162=CARTESIAN_POINT('Ctrl Pts',(-90.708530098757,34.6315292362828,116.685806188043));
#51163=CARTESIAN_POINT('Ctrl Pts',(-90.8188258959115,37.8745963794897,116.527857664851));
#51164=CARTESIAN_POINT('Ctrl Pts',(-88.1635343751796,39.7398246760122,116.369909141658));
#51165=CARTESIAN_POINT('Ctrl Pts',(-85.1501276013673,38.5360683577472,116.211960618466));
#51166=CARTESIAN_POINT('Ctrl Pts',(-84.5107698476665,35.3547366678723,116.054012095273));
#51167=CARTESIAN_POINT('Ctrl Pts',(-86.8251473441704,33.0802462937674,115.896063572081));
#51168=CARTESIAN_POINT('Ctrl Pts',(-89.9948844034088,33.7748084821357,115.738115048888));
#51169=CARTESIAN_POINT('Ctrl Pts',(-91.1460768369648,36.8086848209377,115.580166525696));
#51170=CARTESIAN_POINT('Ctrl Pts',(-89.2349734772688,39.4311519049595,115.422218002504));
#51171=CARTESIAN_POINT('Ctrl Pts',(-85.9943136169755,39.2644985878494,115.264269479311));
#51172=CARTESIAN_POINT('Ctrl Pts',(-84.3623049911988,36.4598243636998,115.106320956119));
#51173=CARTESIAN_POINT('Ctrl Pts',(-85.8186401856314,33.5600420512363,114.948372432926));
#51174=CARTESIAN_POINT('Ctrl Pts',(-89.0429043719145,33.1942960802773,114.790423909734));
#51175=CARTESIAN_POINT('Ctrl Pts',(-91.1117552739073,35.6941971990304,114.632475386541));
#51176=CARTESIAN_POINT('Ctrl Pts',(-90.1494287000289,38.7931610941779,114.474526863349));
#51177=CARTESIAN_POINT('Ctrl Pts',(-87.0284368869753,39.6814514527158,114.316578340156));
#51178=CARTESIAN_POINT('Ctrl Pts',(-84.5784881909668,37.5536824226879,114.158629816964));
#51179=CARTESIAN_POINT('Ctrl Pts',(-85.020876582853,34.3390374704508,114.000681293771));
#51180=CARTESIAN_POINT('Ctrl Pts',(-87.9545019623453,32.952137405191,113.842732770579));
#51181=CARTESIAN_POINT('Ctrl Pts',(-90.7195354200411,34.650442335421,113.684784247386));
#51182=CARTESIAN_POINT('Ctrl Pts',(-90.8090052145385,37.8941508325107,113.526835724194));
#51183=CARTESIAN_POINT('Ctrl Pts',(-88.1417918042676,39.7422910550834,113.368887201001));
#51184=CARTESIAN_POINT('Ctrl Pts',(-85.1361764686922,38.5192104719765,113.210938677809));
#51185=CARTESIAN_POINT('Ctrl Pts',(-84.5172592209201,35.3338390495785,113.052990154617));
#51186=CARTESIAN_POINT('Ctrl Pts',(-86.846193505989,33.0742561778852,112.895041631424));
#51187=CARTESIAN_POINT('Ctrl Pts',(-90.0114054389617,33.7891569245543,112.737093108232));
#51188=CARTESIAN_POINT('Ctrl Pts',(-91.1430936257806,36.8303625253044,112.579144585039));
#51189=CARTESIAN_POINT('Ctrl Pts',(-89.2151908061982,39.4405043560225,112.421196061847));
#51190=CARTESIAN_POINT('Ctrl Pts',(-85.975667832215,39.2530462026721,112.263247538654));
#51191=CARTESIAN_POINT('Ctrl Pts',(-84.3617016587055,36.4379506716133,112.105299015462));
#51192=CARTESIAN_POINT('Ctrl Pts',(-85.8366263286264,33.5475792635982,111.947350492269));
#51193=CARTESIAN_POINT('Ctrl Pts',(-89.06317250157,33.2025438275986,111.789401969077));
#51194=CARTESIAN_POINT('Ctrl Pts',(-91.115928893488,35.7156774996627,111.631453445884));
#51195=CARTESIAN_POINT('Ctrl Pts',(-90.133723715604,38.8083984128235,111.473504922692));
#51196=CARTESIAN_POINT('Ctrl Pts',(-87.0070925302608,39.6766305759976,111.315556399499));
#51197=CARTESIAN_POINT('Ctrl Pts',(-84.5708567410705,37.5331742928717,111.157607876307));
#51198=CARTESIAN_POINT('Ctrl Pts',(-85.0338772432258,34.3214361851846,110.999659353114));
#51199=CARTESIAN_POINT('Ctrl Pts',(-87.9763474297686,32.9534015143623,110.841710829922));
#51200=CARTESIAN_POINT('Ctrl Pts',(-90.7304190733056,34.6694257099876,110.683762306729));
#51201=CARTESIAN_POINT('Ctrl Pts',(-90.7990591768499,37.9136418234947,110.525813783537));
#51202=CARTESIAN_POINT('Ctrl Pts',(-88.1200338442505,39.7446177750092,110.367865260345));
#51203=CARTESIAN_POINT('Ctrl Pts',(-85.1223338695316,38.5022633520643,110.209916737152));
#51204=CARTESIAN_POINT('Ctrl Pts',(-84.5238826409736,35.3129835333494,110.05196821396));
#51205=CARTESIAN_POINT('Ctrl Pts',(-86.8672777026315,33.0684013166716,109.894019690767));
#51206=CARTESIAN_POINT('Ctrl Pts',(-90.027833989938,33.8036111654504,109.736071167575));
#51207=CARTESIAN_POINT('Ctrl Pts',(-91.1399713096509,36.8520206014254,109.578122644382));
#51208=CARTESIAN_POINT('Ctrl Pts',(-89.1953484372759,39.449729643605,109.42017412119));
#51209=CARTESIAN_POINT('Ctrl Pts',(-85.9570960777986,39.2414742183526,109.262225597997));
#51210=CARTESIAN_POINT('Ctrl Pts',(-84.3612385629288,36.4160737840598,109.104277074805));
#51211=CARTESIAN_POINT('Ctrl Pts',(-85.8546925905136,33.535231753797,108.946328551612));
#51212=CARTESIAN_POINT('Ctrl Pts',(-89.0833862960218,33.2109225091254,108.78838002842));
#51213=CARTESIAN_POINT('Ctrl Pts',(-91.1199664734373,35.7371821766864,108.630431505227));
#51214=CARTESIAN_POINT('Ctrl Pts',(-90.117917161972,38.8235386467383,108.472482982035));
#51215=CARTESIAN_POINT('Ctrl Pts',(-86.9857879058164,39.6716643744082,108.314534458842));
#51216=CARTESIAN_POINT('Ctrl Pts',(-84.5633399852011,37.5126348017347,108.15658593565));
#51217=CARTESIAN_POINT('Ctrl Pts',(-85.0470259142193,34.3038833322054,107.998637412457));
#51218=CARTESIAN_POINT('Ctrl Pts',(-87.9981118159091,32.9548786837549,107.840688889265));
#51219=CARTESIAN_POINT('Ctrl Pts',(-90.7413297364918,34.6883288302397,107.682740366073));
#51220=CARTESIAN_POINT('Ctrl Pts',(-90.7886815130315,37.9333765618813,107.52479184288));
#51221=CARTESIAN_POINT('Ctrl Pts',(-88.0988922822239,39.7461715263621,107.366843319688));
#51222=CARTESIAN_POINT('Ctrl Pts',(-85.1073028702349,38.486545658894,107.208894796495));
#51223=CARTESIAN_POINT('Ctrl Pts',(-84.5333640669706,35.2895105687219,107.050946273303));
#51224=CARTESIAN_POINT('Ctrl Pts',(-86.099613541549,33.8115080262147,106.945647257841));
#51225=CARTESIAN_POINT('Ctrl Pts',(-87.0226227342259,33.5647485048412,106.89299775011));
#51226=CARTESIAN_POINT('Ctrl Pts',(-85.4324929308759,38.352227631614,122.321006749669));
#51227=CARTESIAN_POINT('Ctrl Pts',(-84.7717723668801,37.5794426551206,122.268357241939));
#51228=CARTESIAN_POINT('Ctrl Pts',(-84.2891210347552,35.3391378547265,122.163058226477));
#51229=CARTESIAN_POINT('Ctrl Pts',(-86.719597222028,32.881352274709,122.005109703284));
#51230=CARTESIAN_POINT('Ctrl Pts',(-90.1024645698366,33.5799801078284,121.847161180092));
#51231=CARTESIAN_POINT('Ctrl Pts',(-91.3686333057658,36.7911511894407,121.6892126569));
#51232=CARTESIAN_POINT('Ctrl Pts',(-89.371024227111,39.6084645019137,121.531264133707));
#51233=CARTESIAN_POINT('Ctrl Pts',(-85.9203582871986,39.4750890566271,121.373315610515));
#51234=CARTESIAN_POINT('Ctrl Pts',(-84.1454682646258,36.5131478641077,121.215367087322));
#51235=CARTESIAN_POINT('Ctrl Pts',(-85.6554864948497,33.4075615942697,121.05741856413));
#51236=CARTESIAN_POINT('Ctrl Pts',(-89.0813771440687,32.974353542169,120.899470040937));
#51237=CARTESIAN_POINT('Ctrl Pts',(-91.3169641803828,35.6061628187407,120.741521517745));
#51238=CARTESIAN_POINT('Ctrl Pts',(-90.3353210714164,38.916874834573,120.583572994552));
#51239=CARTESIAN_POINT('Ctrl Pts',(-87.0264678163487,39.9047351945452,120.42562447136));
#51240=CARTESIAN_POINT('Ctrl Pts',(-84.3904439217461,37.6740967587225,120.267675948167));
#51241=CARTESIAN_POINT('Ctrl Pts',(-84.8172506743583,34.2474038701722,120.109727424975));
#51242=CARTESIAN_POINT('Ctrl Pts',(-87.9199160567175,32.7315384896552,119.951778901782));
#51243=CARTESIAN_POINT('Ctrl Pts',(-90.8853473971509,34.5008878376316,119.79383037859));
#51244=CARTESIAN_POINT('Ctrl Pts',(-91.0248784506275,37.9512375562013,119.635881855397));
#51245=CARTESIAN_POINT('Ctrl Pts',(-88.2120005759172,39.9542600635284,119.477933332205));
#51246=CARTESIAN_POINT('Ctrl Pts',(-84.9970646304694,38.6938759803182,119.319984809012));
#51247=CARTESIAN_POINT('Ctrl Pts',(-84.2949552395589,35.3128371203772,119.16203628582));
#51248=CARTESIAN_POINT('Ctrl Pts',(-86.7422536432798,32.8766286377651,119.004087762628));
#51249=CARTESIAN_POINT('Ctrl Pts',(-90.1200688057952,33.5940866457133,118.846139239435));
#51250=CARTESIAN_POINT('Ctrl Pts',(-91.3658384529962,36.8147138005949,118.688190716243));
#51251=CARTESIAN_POINT('Ctrl Pts',(-89.3500611330962,39.6184654063458,118.53024219305));
#51252=CARTESIAN_POINT('Ctrl Pts',(-85.9003808354589,39.4632651570443,118.372293669858));
#51253=CARTESIAN_POINT('Ctrl Pts',(-84.144517768422,36.4898283971866,118.214345146665));
#51254=CARTESIAN_POINT('Ctrl Pts',(-85.6744595728268,33.3940798045978,118.056396623473));
#51255=CARTESIAN_POINT('Ctrl Pts',(-89.1030545456374,32.9828404749231,117.89844810028));
#51256=CARTESIAN_POINT('Ctrl Pts',(-91.3216999010375,35.6289686012542,117.740499577088));
#51257=CARTESIAN_POINT('Ctrl Pts',(-90.3188173723202,38.9333002897206,117.582551053895));
#51258=CARTESIAN_POINT('Ctrl Pts',(-87.0036900469868,39.8998984951319,117.424602530703));
#51259=CARTESIAN_POINT('Ctrl Pts',(-84.3820430458739,37.6523780223793,117.26665400751));
#51260=CARTESIAN_POINT('Ctrl Pts',(-84.8308439711031,34.228497328871,117.108705484318));
#51261=CARTESIAN_POINT('Ctrl Pts',(-87.9431786734311,32.7325849067827,116.950756961125));
#51262=CARTESIAN_POINT('Ctrl Pts',(-90.8971879356389,34.5209390531042,116.792808437933));
#51263=CARTESIAN_POINT('Ctrl Pts',(-91.0145614018127,37.9721134536974,116.634859914741));
#51264=CARTESIAN_POINT('Ctrl Pts',(-88.1888801199258,39.9570332422698,116.476911391548));
#51265=CARTESIAN_POINT('Ctrl Pts',(-84.9821033690532,38.6760320151288,116.318962868356));
#51266=CARTESIAN_POINT('Ctrl Pts',(-84.3017180995052,35.2905546250324,116.161014345163));
#51267=CARTESIAN_POINT('Ctrl Pts',(-86.7646089421984,32.8701104569402,116.003065821971));
#51268=CARTESIAN_POINT('Ctrl Pts',(-90.1377476755016,33.6092426235799,115.845117298778));
#51269=CARTESIAN_POINT('Ctrl Pts',(-91.3628119993062,36.8378024691479,115.687168775586));
#51270=CARTESIAN_POINT('Ctrl Pts',(-89.3290733498657,39.6285529738767,115.529220252393));
#51271=CARTESIAN_POINT('Ctrl Pts',(-85.8804607072626,39.4512055319686,115.371271729201));
#51272=CARTESIAN_POINT('Ctrl Pts',(-84.143726269733,36.466555675223,115.213323206008));
#51273=CARTESIAN_POINT('Ctrl Pts',(-85.6935143313946,33.3806946547291,115.055374682816));
#51274=CARTESIAN_POINT('Ctrl Pts',(-89.1246791914122,32.9914788055483,114.897426159624));
#51275=CARTESIAN_POINT('Ctrl Pts',(-91.3262880253696,35.6517983006678,114.739477636431));
#51276=CARTESIAN_POINT('Ctrl Pts',(-90.3022090624238,38.9496223638228,114.581529113239));
#51277=CARTESIAN_POINT('Ctrl Pts',(-86.9809435523238,39.8949142157357,114.423580590046));
#51278=CARTESIAN_POINT('Ctrl Pts',(-84.373781921353,37.630606484029,114.265632066854));
#51279=CARTESIAN_POINT('Ctrl Pts',(-84.8445583270759,34.2096781232347,114.107683543661));
#51280=CARTESIAN_POINT('Ctrl Pts',(-87.9664341204409,32.7337808352518,113.949735020469));
#51281=CARTESIAN_POINT('Ctrl Pts',(-90.9088994671639,34.5410658037077,113.791786497276));
#51282=CARTESIAN_POINT('Ctrl Pts',(-91.0041105284097,37.9929227137908,113.633837974084));
#51283=CARTESIAN_POINT('Ctrl Pts',(-88.16574233066,39.9596578886113,113.475889450891));
#51284=CARTESIAN_POINT('Ctrl Pts',(-84.9672569937481,38.6580923607057,113.317940927699));
#51285=CARTESIAN_POINT('Ctrl Pts',(-84.3086238951178,35.2683160089,113.159992404506));
#51286=CARTESIAN_POINT('Ctrl Pts',(-86.7870056338769,32.863735955989,113.002043881314));
#51287=CARTESIAN_POINT('Ctrl Pts',(-90.155328864066,33.6245118039505,112.844095358121));
#51288=CARTESIAN_POINT('Ctrl Pts',(-91.3596373557926,36.8608712293895,112.686146834929));
#51289=CARTESIAN_POINT('Ctrl Pts',(-89.3080212269955,39.6385055706828,112.528198311736));
#51290=CARTESIAN_POINT('Ctrl Pts',(-85.8606184245708,39.4390182485099,112.370249788544));
#51291=CARTESIAN_POINT('Ctrl Pts',(-84.1430842214608,36.4432783507515,112.212301265351));
#51292=CARTESIAN_POINT('Ctrl Pts',(-85.7126546431824,33.3674321313963,112.054352742159));
#51293=CARTESIAN_POINT('Ctrl Pts',(-89.1462479246903,33.0002558098966,111.896404218967));
#51294=CARTESIAN_POINT('Ctrl Pts',(-91.330729465654,35.6746569897993,111.738455695774));
#51295=CARTESIAN_POINT('Ctrl Pts',(-90.2854962908975,38.9658374595089,111.580507172582));
#51296=CARTESIAN_POINT('Ctrl Pts',(-86.9582295306161,39.8897839838954,111.422558649389));
#51297=CARTESIAN_POINT('Ctrl Pts',(-84.3656607621669,37.6087823498066,111.264610126197));
#51298=CARTESIAN_POINT('Ctrl Pts',(-84.858393238377,34.1909473654533,111.106661603004));
#51299=CARTESIAN_POINT('Ctrl Pts',(-87.9896814090755,32.7351260621679,110.948713079812));
#51300=CARTESIAN_POINT('Ctrl Pts',(-90.9204815232464,34.561267339306,110.790764556619));
#51301=CARTESIAN_POINT('Ctrl Pts',(-90.9935262545903,38.0136644394956,110.632816033427));
#51302=CARTESIAN_POINT('Ctrl Pts',(-88.1425881647719,39.9621339138956,110.474867510234));
#51303=CARTESIAN_POINT('Ctrl Pts',(-84.952526116541,38.6400577459963,110.316918987042));
#51304=CARTESIAN_POINT('Ctrl Pts',(-84.3156723392984,35.2461221965173,110.158970463849));
#51305=CARTESIAN_POINT('Ctrl Pts',(-86.8094428010696,32.8575053889834,110.001021940657));
#51306=CARTESIAN_POINT('Ctrl Pts',(-90.1728116333289,33.6398935718751,109.843073417464));
#51307=CARTESIAN_POINT('Ctrl Pts',(-91.3563146809844,36.883919101843,109.685124894272));
#51308=CARTESIAN_POINT('Ctrl Pts',(-89.2869055754696,39.648322843942,109.52717637108));
#51309=CARTESIAN_POINT('Ctrl Pts',(-85.8408549227417,39.4267036912455,109.369227847887));
#51310=CARTESIAN_POINT('Ctrl Pts',(-84.1425914088798,36.4199976257601,109.211279324695));
#51311=CARTESIAN_POINT('Ctrl Pts',(-85.7318802150827,33.3542922832663,109.053330801502));
#51312=CARTESIAN_POINT('Ctrl Pts',(-89.1677588360808,33.0091721504837,108.89538227831));
#51313=CARTESIAN_POINT('Ctrl Pts',(-91.3350261366591,35.6975416195525,108.737433755117));
#51314=CARTESIAN_POINT('Ctrl Pts',(-90.2686754324792,38.9819492405478,108.579485231925));
#51315=CARTESIAN_POINT('Ctrl Pts',(-86.9355577907939,39.8844991017031,108.421536708732));
#51316=CARTESIAN_POINT('Ctrl Pts',(-84.3576616569105,37.5869248418109,108.26358818554));
#51317=CARTESIAN_POINT('Ctrl Pts',(-84.8723856581236,34.1722681478534,108.105639662347));
#51318=CARTESIAN_POINT('Ctrl Pts',(-88.0128424134507,32.7366980213559,107.947691139155));
#51319=CARTESIAN_POINT('Ctrl Pts',(-90.932092322474,34.5813834706793,107.789742615963));
#51320=CARTESIAN_POINT('Ctrl Pts',(-90.9824826572406,38.0346655538465,107.63179409277));
#51321=CARTESIAN_POINT('Ctrl Pts',(-88.1200899510646,39.9637873692998,107.473845569578));
#51322=CARTESIAN_POINT('Ctrl Pts',(-84.9365305796935,38.6233314502058,107.315897046385));
#51323=CARTESIAN_POINT('Ctrl Pts',(-84.3257621873457,35.2211429743639,107.157948523192));
#51324=CARTESIAN_POINT('Ctrl Pts',(-85.9925177162683,33.6482971733151,107.052649507731));
#51325=CARTESIAN_POINT('Ctrl Pts',(-86.97475630604,33.3857031209377,107.));
#51326=CARTESIAN_POINT('Ctrl Pts',(-85.855089591907,37.9909132780583,122.));
#51327=CARTESIAN_POINT('Ctrl Pts',(-85.7934813679502,37.9330166755841,122.));
#51328=CARTESIAN_POINT('Ctrl Pts',(-85.7352422962271,37.8719693152205,122.));
#51329=CARTESIAN_POINT('Ctrl Pts',(-85.6803699910001,37.8081560154705,122.));
#51330=CARTESIAN_POINT('Ctrl Pts',(-85.624044758381,37.7426530456618,122.));
#51331=CARTESIAN_POINT('Ctrl Pts',(-85.5712665086079,37.6742352905882,122.));
#51332=CARTESIAN_POINT('Ctrl Pts',(-85.522058169157,37.6032704024903,122.));
#51333=CARTESIAN_POINT('Ctrl Pts',(-85.471500272293,37.530359275363,122.));
#51334=CARTESIAN_POINT('Ctrl Pts',(-85.4247102505921,37.4547588307541,122.));
#51335=CARTESIAN_POINT('Ctrl Pts',(-85.3817470379049,37.3768248282257,122.));
#51336=CARTESIAN_POINT('Ctrl Pts',(-85.3628370824531,37.3425227259429,122.));
#51337=CARTESIAN_POINT('Ctrl Pts',(-85.3446689632654,37.3077680551632,122.));
#51338=CARTESIAN_POINT('Ctrl Pts',(-85.327250130523,37.2725890732149,122.));
#51339=CARTESIAN_POINT('Ctrl Pts',(-85.3173192863124,37.2525327930737,122.));
#51340=CARTESIAN_POINT('Ctrl Pts',(-85.3076320170822,37.2323385748829,122.));
#51341=CARTESIAN_POINT('Ctrl Pts',(-85.2981899377649,37.2120115066752,122.));
#51342=CARTESIAN_POINT('Ctrl Pts',(-85.2896843470291,37.1937005269402,122.));
#51343=CARTESIAN_POINT('Ctrl Pts',(-85.2813753465996,37.1752760152876,122.));
#51344=CARTESIAN_POINT('Ctrl Pts',(-85.2732777774911,37.1567734456981,122.));
#51345=CARTESIAN_POINT('Ctrl Pts',(-85.2367161205784,37.0732317565482,122.));
#51346=CARTESIAN_POINT('Ctrl Pts',(-85.2044146446107,36.9880065244174,122.));
#51347=CARTESIAN_POINT('Ctrl Pts',(-85.1763983858018,36.9014965265309,122.));
#51348=CARTESIAN_POINT('Ctrl Pts',(-85.1479190352312,36.8135565708614,122.));
#51349=CARTESIAN_POINT('Ctrl Pts',(-85.1238672433657,36.7242882705842,122.));
#51350=CARTESIAN_POINT('Ctrl Pts',(-85.1043083835495,36.6340733818492,122.));
#51351=CARTESIAN_POINT('Ctrl Pts',(-85.0853398921155,36.5465815566475,122.));
#51352=CARTESIAN_POINT('Ctrl Pts',(-85.0705970385735,36.4581985072518,122.));
#51353=CARTESIAN_POINT('Ctrl Pts',(-85.0601801960536,36.3692505885246,122.));
#51354=CARTESIAN_POINT('Ctrl Pts',(-85.0558113579426,36.3319457088082,122.));
#51355=CARTESIAN_POINT('Ctrl Pts',(-85.0522039701671,36.2945412778582,122.));
#51356=CARTESIAN_POINT('Ctrl Pts',(-85.0493677722714,36.2570607532382,122.));
#51357=CARTESIAN_POINT('Ctrl Pts',(-85.0475886407492,36.2335494238905,122.));
#51358=CARTESIAN_POINT('Ctrl Pts',(-85.0461129995367,36.2100081463298,122.));
#51359=CARTESIAN_POINT('Ctrl Pts',(-85.0449435487391,36.1864426779331,122.));
#51360=CARTESIAN_POINT('Ctrl Pts',(-85.0442591625791,36.1726516912063,122.));
#51361=CARTESIAN_POINT('Ctrl Pts',(-85.043679931207,36.1588573660533,122.));
#51362=CARTESIAN_POINT('Ctrl Pts',(-85.0432063554223,36.1450686933549,122.));
#51363=CARTESIAN_POINT('Ctrl Pts',(-85.0398789557942,36.0481878436707,122.));
#51364=CARTESIAN_POINT('Ctrl Pts',(-85.0417574731529,35.9514719964611,122.));
#51365=CARTESIAN_POINT('Ctrl Pts',(-85.0489062899786,35.8553409172261,122.));
#51366=CARTESIAN_POINT('Ctrl Pts',(-85.0560551068044,35.7592098379912,122.));
#51367=CARTESIAN_POINT('Ctrl Pts',(-85.0684737927824,35.6636624826983,122.));
#51368=CARTESIAN_POINT('Ctrl Pts',(-85.0862791933242,35.5690998313702,122.));
#51369=CARTESIAN_POINT('Ctrl Pts',(-85.1033372114407,35.4785064512488,122.));
#51370=CARTESIAN_POINT('Ctrl Pts',(-85.1253390876716,35.3888158753331,122.));
#51371=CARTESIAN_POINT('Ctrl Pts',(-85.1520102123209,35.3002674435879,122.));
#51372=CARTESIAN_POINT('Ctrl Pts',(-85.1608795543707,35.2708211289146,122.));
#51373=CARTESIAN_POINT('Ctrl Pts',(-85.1702656805221,35.2415011553756,122.));
#51374=CARTESIAN_POINT('Ctrl Pts',(-85.1801597406793,35.2123164991087,122.));
#51375=CARTESIAN_POINT('Ctrl Pts',(-85.1894800179375,35.1848243387849,122.));
#51376=CARTESIAN_POINT('Ctrl Pts',(-85.1992510307603,35.157452254975,122.));
#51377=CARTESIAN_POINT('Ctrl Pts',(-85.2094658558997,35.1302078758792,122.));
#51378=CARTESIAN_POINT('Ctrl Pts',(-85.2146236706355,35.1164512566469,122.));
#51379=CARTESIAN_POINT('Ctrl Pts',(-85.219891565519,35.1027354709933,122.));
#51380=CARTESIAN_POINT('Ctrl Pts',(-85.2252668704309,35.089064837704,122.));
#51381=CARTESIAN_POINT('Ctrl Pts',(-85.2595181900841,35.0019558758258,122.));
#51382=CARTESIAN_POINT('Ctrl Pts',(-85.298143010024,34.9166357250449,122.));
#51383=CARTESIAN_POINT('Ctrl Pts',(-85.3408113440508,34.8333388006193,122.));
#51384=CARTESIAN_POINT('Ctrl Pts',(-85.3850411534874,34.7469935711176,122.));
#51385=CARTESIAN_POINT('Ctrl Pts',(-85.4336159720851,34.6628216295505,122.));
#51386=CARTESIAN_POINT('Ctrl Pts',(-85.4862240883796,34.5810875555579,122.));
#51387=CARTESIAN_POINT('Ctrl Pts',(-85.5393951618781,34.498478848733,122.));
#51388=CARTESIAN_POINT('Ctrl Pts',(-85.5966867302764,34.418359642024,122.));
#51389=CARTESIAN_POINT('Ctrl Pts',(-85.6578284758595,34.3410184645814,122.));
#51390=CARTESIAN_POINT('Ctrl Pts',(-85.6805173073739,34.3123182544813,122.));
#51391=CARTESIAN_POINT('Ctrl Pts',(-85.7037367996653,34.2840008059673,122.));
#51392=CARTESIAN_POINT('Ctrl Pts',(-85.7274747338933,34.2560817511357,122.));
#51393=CARTESIAN_POINT('Ctrl Pts',(-85.7482297832317,34.2316709765946,122.));
#51394=CARTESIAN_POINT('Ctrl Pts',(-85.7693811810863,34.207564768343,122.));
#51395=CARTESIAN_POINT('Ctrl Pts',(-85.7909212499565,34.1837739578324,122.));
#51396=CARTESIAN_POINT('Ctrl Pts',(-85.8026849836044,34.1707810208181,122.));
#51397=CARTESIAN_POINT('Ctrl Pts',(-85.8145599672992,34.157887404697,122.));
#51398=CARTESIAN_POINT('Ctrl Pts',(-85.8265388744956,34.1451007332879,122.));
#51399=CARTESIAN_POINT('Ctrl Pts',(-85.895549674298,34.0714363825852,122.));
#51400=CARTESIAN_POINT('Ctrl Pts',(-85.9680628718138,34.0012565621351,122.));
#51401=CARTESIAN_POINT('Ctrl Pts',(-86.043769945045,33.9348524870057,122.));
#51402=CARTESIAN_POINT('Ctrl Pts',(-86.1059641041579,33.8803008389485,122.));
#51403=CARTESIAN_POINT('Ctrl Pts',(-86.1703148362795,33.8282974253922,122.));
#51404=CARTESIAN_POINT('Ctrl Pts',(-86.2366733734612,33.7790170367676,122.));
#51405=CARTESIAN_POINT('Ctrl Pts',(-86.2612909125297,33.7607351103751,122.));
#51406=CARTESIAN_POINT('Ctrl Pts',(-86.2861849555798,33.7428280844223,122.));
#51407=CARTESIAN_POINT('Ctrl Pts',(-86.3113485141177,33.7253054477748,122.));
#51408=CARTESIAN_POINT('Ctrl Pts',(-86.3281594689655,33.7135991442704,122.));
#51409=CARTESIAN_POINT('Ctrl Pts',(-86.3450918490799,33.7020637690538,122.));
#51410=CARTESIAN_POINT('Ctrl Pts',(-86.3621285098423,33.6907119748374,122.));
#51411=CARTESIAN_POINT('Ctrl Pts',(-86.4470390092949,33.6341347775783,122.));
#51412=CARTESIAN_POINT('Ctrl Pts',(-86.5346187851364,33.5820568809078,122.));
#51413=CARTESIAN_POINT('Ctrl Pts',(-86.6245774787622,33.534786201639,122.));
#51414=CARTESIAN_POINT('Ctrl Pts',(-86.7080355351971,33.4909314183033,122.));
#51415=CARTESIAN_POINT('Ctrl Pts',(-86.7935419310316,33.4512139208354,122.));
#51416=CARTESIAN_POINT('Ctrl Pts',(-86.8808925248099,33.4159086346823,122.));
#51417=CARTESIAN_POINT('Ctrl Pts',(-86.9113227051827,33.4036093911479,122.));
#51418=CARTESIAN_POINT('Ctrl Pts',(-86.941976905733,33.3918459065886,122.));
#51419=CARTESIAN_POINT('Ctrl Pts',(-86.9728422201938,33.3806144585182,122.));
#51420=CARTESIAN_POINT('Ctrl Pts',(-90.2867225490468,36.352727843524,120.387416697508));
#51421=CARTESIAN_POINT('Ctrl Pts',(-90.2883049087302,36.1783614273162,120.398449387697));
#51422=CARTESIAN_POINT('Ctrl Pts',(-90.2717193152599,36.0042940565252,120.409482077886));
#51423=CARTESIAN_POINT('Ctrl Pts',(-90.2358477575736,35.8342964268918,120.420514768075));
#51424=CARTESIAN_POINT('Ctrl Pts',(-90.064663774216,35.0230444691006,120.473164275806));
#51425=CARTESIAN_POINT('Ctrl Pts',(-89.454274927199,34.304473908527,120.525813783537));
#51426=CARTESIAN_POINT('Ctrl Pts',(-88.6813900471312,34.0043286570435,120.578463291268));
#51427=CARTESIAN_POINT('Ctrl Pts',(-87.9085051670634,33.7041834055601,120.631112798999));
#51428=CARTESIAN_POINT('Ctrl Pts',(-86.9731242539449,33.8224634631669,120.683762306729));
#51429=CARTESIAN_POINT('Ctrl Pts',(-86.2992914572421,34.3055671292089,120.73641181446));
#51430=CARTESIAN_POINT('Ctrl Pts',(-85.6254586605392,34.7886707952509,120.789061322191));
#51431=CARTESIAN_POINT('Ctrl Pts',(-85.213173980252,35.6365980697281,120.841710829922));
#51432=CARTESIAN_POINT('Ctrl Pts',(-85.2493333391392,36.4649154270561,120.894360337653));
#51433=CARTESIAN_POINT('Ctrl Pts',(-85.2854926980264,37.293232784384,120.947009845384));
#51434=CARTESIAN_POINT('Ctrl Pts',(-85.7700960960879,38.1019402245628,120.999659353114));
#51435=CARTESIAN_POINT('Ctrl Pts',(-86.4834704866067,38.5245018880125,121.052308860845));
#51436=CARTESIAN_POINT('Ctrl Pts',(-87.1968448771254,38.9470635514623,121.104958368576));
#51437=CARTESIAN_POINT('Ctrl Pts',(-88.1389902601014,38.983479438183,121.157607876307));
#51438=CARTESIAN_POINT('Ctrl Pts',(-88.8827694672617,38.6170777473505,121.210257384038));
#51439=CARTESIAN_POINT('Ctrl Pts',(-89.626548674422,38.250676056518,121.262906891768));
#51440=CARTESIAN_POINT('Ctrl Pts',(-90.1719617057666,37.4814567881323,121.315556399499));
#51441=CARTESIAN_POINT('Ctrl Pts',(-90.2718153505154,36.6584694521901,121.36820590723));
#51442=CARTESIAN_POINT('Ctrl Pts',(-90.2839602404389,36.5583720483486,121.374609503989));
#51443=CARTESIAN_POINT('Ctrl Pts',(-90.289513923836,36.4574792478699,121.381013100749));
#51444=CARTESIAN_POINT('Ctrl Pts',(-90.2887581529621,36.3565049378502,121.387416697508));
#51445=CARTESIAN_POINT('Ctrl Pts',(-88.5623548711056,33.385703120938,122.));
#51446=CARTESIAN_POINT('Ctrl Pts',(-89.5445934608772,33.6482971733158,121.947350492269));
#51447=CARTESIAN_POINT('Ctrl Pts',(-91.2113489167469,35.2211434798136,121.842051476807));
#51448=CARTESIAN_POINT('Ctrl Pts',(-90.6005806604956,38.6233313190636,121.684102953615));
#51449=CARTESIAN_POINT('Ctrl Pts',(-87.4170212212397,39.9637875212778,121.526154430423));
#51450=CARTESIAN_POINT('Ctrl Pts',(-84.554628466517,38.0346655247349,121.36820590723));
#51451=CARTESIAN_POINT('Ctrl Pts',(-84.6050188146032,34.5813834739332,121.210257384038));
#51452=CARTESIAN_POINT('Ctrl Pts',(-87.5242687556742,32.7366979528604,121.052308860845));
#51453=CARTESIAN_POINT('Ctrl Pts',(-90.6647255642019,34.1722681242997,120.894360337653));
#51454=CARTESIAN_POINT('Ctrl Pts',(-91.1794495683065,37.5869248554102,120.73641181446));
#51455=CARTESIAN_POINT('Ctrl Pts',(-88.601553399534,39.8844991555637,120.578463291268));
#51456=CARTESIAN_POINT('Ctrl Pts',(-85.2684357075705,38.981949277713,120.420514768075));
#51457=CARTESIAN_POINT('Ctrl Pts',(-84.202084988714,35.697541610575,120.262566244883));
#51458=CARTESIAN_POINT('Ctrl Pts',(-86.3693523204529,33.0091721012914,120.10461772169));
#51459=CARTESIAN_POINT('Ctrl Pts',(-89.8052309919053,33.3542922396066,119.946669198498));
#51460=CARTESIAN_POINT('Ctrl Pts',(-91.3945198211751,36.4199976266262,119.788720675305));
#51461=CARTESIAN_POINT('Ctrl Pts',(-89.6962562825846,39.4267037361566,119.630772152113));
#51462=CARTESIAN_POINT('Ctrl Pts',(-86.2502055794825,39.6483228920224,119.47282362892));
#51463=CARTESIAN_POINT('Ctrl Pts',(-84.1807964437643,36.8839191095796,119.314875105728));
#51464=CARTESIAN_POINT('Ctrl Pts',(-85.3642995086962,33.6398935322125,119.156926582536));
#51465=CARTESIAN_POINT('Ctrl Pts',(-88.727668390087,32.8575053379033,118.998978059343));
#51466=CARTESIAN_POINT('Ctrl Pts',(-91.2214388882784,35.2461221803218,118.841029536151));
#51467=CARTESIAN_POINT('Ctrl Pts',(-90.5845851017341,38.6400577793749,118.683081012958));
#51468=CARTESIAN_POINT('Ctrl Pts',(-87.394523006908,39.962133966582,118.525132489766));
#51469=CARTESIAN_POINT('Ctrl Pts',(-84.5435848754497,38.0136644637222,118.367183966573));
#51470=CARTESIAN_POINT('Ctrl Pts',(-84.6166296078616,34.5612673131065,118.209235443381));
#51471=CARTESIAN_POINT('Ctrl Pts',(-87.5474297648405,32.7351260092969,118.051286920188));
#51472=CARTESIAN_POINT('Ctrl Pts',(-90.6787179812742,34.1909473338473,117.893338396996));
#51473=CARTESIAN_POINT('Ctrl Pts',(-91.17145046468,37.6087823681217,117.735389873803));
#51474=CARTESIAN_POINT('Ctrl Pts',(-88.5788816583627,39.8897840355259,117.577441350611));
#51475=CARTESIAN_POINT('Ctrl Pts',(-85.2516148494836,38.9658374976431,117.419492827418));
#51476=CARTESIAN_POINT('Ctrl Pts',(-84.2063816594615,35.6746569798619,117.261544304226));
#51477=CARTESIAN_POINT('Ctrl Pts',(-86.3908632323328,33.0002557608977,117.103595781033));
#51478=CARTESIAN_POINT('Ctrl Pts',(-89.8244565639917,33.3674320877617,116.945647257841));
#51479=CARTESIAN_POINT('Ctrl Pts',(-91.3940270086374,36.4432783520433,116.787698734648));
#51480=CARTESIAN_POINT('Ctrl Pts',(-89.6764927804399,39.4390182935569,116.629750211456));
#51481=CARTESIAN_POINT('Ctrl Pts',(-86.2290899276622,39.6385056186423,116.471801688264));
#51482=CARTESIAN_POINT('Ctrl Pts',(-84.1774737689002,36.8608712367781,116.313853165071));
#51483=CARTESIAN_POINT('Ctrl Pts',(-85.3817822782182,33.6245117640691,116.155904641879));
#51484=CARTESIAN_POINT('Ctrl Pts',(-88.7501055576055,32.8637359049969,115.997956118686));
#51485=CARTESIAN_POINT('Ctrl Pts',(-91.228487332563,35.2683159930302,115.840007595494));
#51486=CARTESIAN_POINT('Ctrl Pts',(-90.5698542243114,38.6580923943469,115.682059072301));
#51487=CARTESIAN_POINT('Ctrl Pts',(-87.3713688406819,39.959657941262,115.524110549109));
#51488=CARTESIAN_POINT('Ctrl Pts',(-84.5330006014756,37.9929227377143,115.366162025916));
#51489=CARTESIAN_POINT('Ctrl Pts',(-84.6282116641132,34.5410657772132,115.208213502724));
#51490=CARTESIAN_POINT('Ctrl Pts',(-87.5706770538148,32.7337807823612,115.050264979531));
#51491=CARTESIAN_POINT('Ctrl Pts',(-90.6925528927773,34.2096780919022,114.892316456339));
#51492=CARTESIAN_POINT('Ctrl Pts',(-91.1633293053753,37.630606502663,114.734367933146));
#51493=CARTESIAN_POINT('Ctrl Pts',(-88.5561676363232,39.8949142674411,114.576419409954));
#51494=CARTESIAN_POINT('Ctrl Pts',(-85.2349020777131,38.9496224017201,114.418470886762));
#51495=CARTESIAN_POINT('Ctrl Pts',(-84.2108230998106,35.6517982903965,114.260522363569));
#51496=CARTESIAN_POINT('Ctrl Pts',(-86.412431965926,32.9914787564211,114.102573840377));
#51497=CARTESIAN_POINT('Ctrl Pts',(-89.8435968760591,33.3806946112882,113.944625317184));
#51498=CARTESIAN_POINT('Ctrl Pts',(-91.3933849603557,36.4665556768548,113.786676793992));
#51499=CARTESIAN_POINT('Ctrl Pts',(-89.6566504974584,39.4512055771937,113.628728270799));
#51500=CARTESIAN_POINT('Ctrl Pts',(-86.2080378044846,39.6285530216908,113.470779747607));
#51501=CARTESIAN_POINT('Ctrl Pts',(-84.1742991253402,36.8378024761994,113.312831224414));
#51502=CARTESIAN_POINT('Ctrl Pts',(-85.3993634670394,33.6092425834755,113.154882701222));
#51503=CARTESIAN_POINT('Ctrl Pts',(-88.7725022496111,32.8701104060413,112.996934178029));
#51504=CARTESIAN_POINT('Ctrl Pts',(-91.2353931282765,35.2905546094874,112.838985654837));
#51505=CARTESIAN_POINT('Ctrl Pts',(-90.5550078487894,38.6760320490321,112.681037131644));
#51506=CARTESIAN_POINT('Ctrl Pts',(-87.3482310510782,39.957033294882,112.523088608452));
#51507=CARTESIAN_POINT('Ctrl Pts',(-84.5225497279198,37.9721134773169,112.365140085259));
#51508=CARTESIAN_POINT('Ctrl Pts',(-84.6399231958095,34.5209390263157,112.207191562067));
#51509=CARTESIAN_POINT('Ctrl Pts',(-87.5939325011642,32.7325848538746,112.049243038874));
#51510=CARTESIAN_POINT('Ctrl Pts',(-90.7062672489506,34.2284972978135,111.891294515682));
#51511=CARTESIAN_POINT('Ctrl Pts',(-91.1550681807335,37.6523780413312,111.73334599249));
#51512=CARTESIAN_POINT('Ctrl Pts',(-88.5334211413281,39.8998985469101,111.575397469297));
#51513=CARTESIAN_POINT('Ctrl Pts',(-85.2182937675741,38.9333003273795,111.417448946105));
#51514=CARTESIAN_POINT('Ctrl Pts',(-84.21541122421,35.6289685906495,111.259500422912));
#51515=CARTESIAN_POINT('Ctrl Pts',(-86.4340566120166,32.9828404256698,111.10155189972));
#51516=CARTESIAN_POINT('Ctrl Pts',(-89.8626516349053,33.3940797613523,110.943603376527));
#51517=CARTESIAN_POINT('Ctrl Pts',(-91.3925934616552,36.4898283991584,110.785654853335));
#51518=CARTESIAN_POINT('Ctrl Pts',(-89.6367303689711,39.4632652024454,110.627706330142));
#51519=CARTESIAN_POINT('Ctrl Pts',(-86.1870500209474,39.6184654540127,110.46975780695));
#51520=CARTESIAN_POINT('Ctrl Pts',(-84.1712726716061,36.8147138073089,110.311809283757));
#51521=CARTESIAN_POINT('Ctrl Pts',(-85.417042337004,33.594086605388,110.153860760565));
#51522=CARTESIAN_POINT('Ctrl Pts',(-88.7948575488562,32.8766285869604,109.995912237372));
#51523=CARTESIAN_POINT('Ctrl Pts',(-91.2421559883216,35.3128371051595,109.83796371418));
#51524=CARTESIAN_POINT('Ctrl Pts',(-90.5400465871546,38.6938760144785,109.680015190987));
#51525=CARTESIAN_POINT('Ctrl Pts',(-87.325110594749,39.9542601161072,109.522066667795));
#51526=CARTESIAN_POINT('Ctrl Pts',(-84.512232678954,37.9512375795022,109.364118144602));
#51527=CARTESIAN_POINT('Ctrl Pts',(-84.6517637344715,34.5008878105768,109.20616962141));
#51528=CARTESIAN_POINT('Ctrl Pts',(-87.6171951182148,32.7315384366804,109.048221098217));
#51529=CARTESIAN_POINT('Ctrl Pts',(-90.7198605459008,34.2474038394901,108.890272575025));
#51530=CARTESIAN_POINT('Ctrl Pts',(-91.146667304722,37.6740967778006,108.732324051833));
#51531=CARTESIAN_POINT('Ctrl Pts',(-88.5106433716724,39.9047352467602,108.57437552864));
#51532=CARTESIAN_POINT('Ctrl Pts',(-85.2017900681466,38.9168748712948,108.416427005448));
#51533=CARTESIAN_POINT('Ctrl Pts',(-84.2201469451404,35.6061628091222,108.258478482255));
#51534=CARTESIAN_POINT('Ctrl Pts',(-86.4557340134341,32.9743534903137,108.100529959063));
#51535=CARTESIAN_POINT('Ctrl Pts',(-89.8816247142105,33.4075615558338,107.94258143587));
#51536=CARTESIAN_POINT('Ctrl Pts',(-91.3916429630939,36.5131478579286,107.784632912678));
#51537=CARTESIAN_POINT('Ctrl Pts',(-89.6167529221334,39.4750891176184,107.626684389485));
#51538=CARTESIAN_POINT('Ctrl Pts',(-86.1660869151683,39.6084645219268,107.468735866293));
#51539=CARTESIAN_POINT('Ctrl Pts',(-84.1684778438722,36.7911512436696,107.310787343101));
#51540=CARTESIAN_POINT('Ctrl Pts',(-85.4346465172346,33.5799799853229,107.152838819908));
#51541=CARTESIAN_POINT('Ctrl Pts',(-88.8175140813586,32.8813523470733,106.994890296716));
#51542=CARTESIAN_POINT('Ctrl Pts',(-91.2479897958802,35.3391374795667,106.836941773523));
#51543=CARTESIAN_POINT('Ctrl Pts',(-90.7653388102639,37.5794426551218,106.731642758061));
#51544=CARTESIAN_POINT('Ctrl Pts',(-90.1046182462678,38.3522276316149,106.678993250331));
#51545=CARTESIAN_POINT('Ctrl Pts',(-88.5144884429196,33.5647485048415,122.10700224989));
#51546=CARTESIAN_POINT('Ctrl Pts',(-89.4374976355964,33.8115080262153,122.054352742159));
#51547=CARTESIAN_POINT('Ctrl Pts',(-91.003747041527,35.2895110436928,121.949053726697));
#51548=CARTESIAN_POINT('Ctrl Pts',(-90.4298083661526,38.4865455356597,121.791105203505));
#51549=CARTESIAN_POINT('Ctrl Pts',(-87.4382188903723,39.7461716691758,121.633156680312));
#51550=CARTESIAN_POINT('Ctrl Pts',(-84.7484296139453,37.9333765345252,121.47520815712));
#51551=CARTESIAN_POINT('Ctrl Pts',(-84.7957814030015,34.6883288332973,121.317259633928));
#51552=CARTESIAN_POINT('Ctrl Pts',(-87.5389993536994,32.9548786193897,121.159311110735));
#51553=CARTESIAN_POINT('Ctrl Pts',(-90.4900853053818,34.3038833100721,121.001362587543));
#51554=CARTESIAN_POINT('Ctrl Pts',(-90.9737712371171,37.512634814514,120.84341406435));
#51555=CARTESIAN_POINT('Ctrl Pts',(-88.5513232837166,39.671664425021,120.685465541158));
#51556=CARTESIAN_POINT('Ctrl Pts',(-85.4191939803146,38.8235386816624,120.527517017965));
#51557=CARTESIAN_POINT('Ctrl Pts',(-84.4171446550577,35.7371821682502,120.369568494773));
#51558=CARTESIAN_POINT('Ctrl Pts',(-86.4537248617547,33.2109224628993,120.21161997158));
#51559=CARTESIAN_POINT('Ctrl Pts',(-89.6824186146749,33.5352317127699,120.053671448388));
#51560=CARTESIAN_POINT('Ctrl Pts',(-91.1758726639355,36.4160737848735,119.895722925195));
#51561=CARTESIAN_POINT('Ctrl Pts',(-89.5800151258284,39.2414742605557,119.737774402003));
#51562=CARTESIAN_POINT('Ctrl Pts',(-86.3417627190143,39.4497296887861,119.57982587881));
#51563=CARTESIAN_POINT('Ctrl Pts',(-84.3971398182574,36.8520206086955,119.421877355618));
#51564=CARTESIAN_POINT('Ctrl Pts',(-85.5092771542047,33.8036111281796,119.263928832425));
#51565=CARTESIAN_POINT('Ctrl Pts',(-88.6698334876803,33.0684012686717,119.105980309233));
#51566=CARTESIAN_POINT('Ctrl Pts',(-91.0132285835621,35.3129835181305,118.948031786041));
#51567=CARTESIAN_POINT('Ctrl Pts',(-90.4147773462634,38.5022633834302,118.790083262848));
#51568=CARTESIAN_POINT('Ctrl Pts',(-87.4170773277588,39.7446178245186,118.632134739655));
#51569=CARTESIAN_POINT('Ctrl Pts',(-84.7380519560306,37.9136418462605,118.474186216463));
#51570=CARTESIAN_POINT('Ctrl Pts',(-84.8066920605784,34.669425685368,118.316237693271));
#51571=CARTESIAN_POINT('Ctrl Pts',(-87.5607637443422,32.9534014646795,118.158289170078));
#51572=CARTESIAN_POINT('Ctrl Pts',(-90.5032339738622,34.3214361554844,118.000340646886));
#51573=CARTESIAN_POINT('Ctrl Pts',(-90.9662544827793,37.5331743100824,117.842392123693));
#51574=CARTESIAN_POINT('Ctrl Pts',(-88.5300186580045,39.6766306245147,117.684443600501));
#51575=CARTESIAN_POINT('Ctrl Pts',(-85.4033874269938,38.8083984486582,117.526495077308));
#51576=CARTESIAN_POINT('Ctrl Pts',(-84.421182234765,35.7156774903246,117.368546554116));
#51577=CARTESIAN_POINT('Ctrl Pts',(-86.4739386566664,33.2025437815544,117.210598030923));
#51578=CARTESIAN_POINT('Ctrl Pts',(-89.7004848767369,33.5475792225948,117.052649507731));
#51579=CARTESIAN_POINT('Ctrl Pts',(-91.1754095681997,36.4379506728273,116.894700984538));
#51580=CARTESIAN_POINT('Ctrl Pts',(-89.5614433711151,39.2530462450027,116.736752461346));
#51581=CARTESIAN_POINT('Ctrl Pts',(-86.3219203498158,39.44050440109,116.578803938153));
#51582=CARTESIAN_POINT('Ctrl Pts',(-84.3940175020749,36.8303625322474,116.420855414961));
#51583=CARTESIAN_POINT('Ctrl Pts',(-85.5257057054248,33.7891568870778,116.262906891768));
#51584=CARTESIAN_POINT('Ctrl Pts',(-88.6909176846287,33.074256129968,116.104958368576));
#51585=CARTESIAN_POINT('Ctrl Pts',(-91.0198520037133,35.3338390346656,115.947009845384));
#51586=CARTESIAN_POINT('Ctrl Pts',(-90.4009347469002,38.5192105035891,115.789061322191));
#51587=CARTESIAN_POINT('Ctrl Pts',(-87.3953193674241,39.7422911045592,115.631112798999));
#51588=CARTESIAN_POINT('Ctrl Pts',(-84.7281059181966,37.8941508549915,115.473164275806));
#51589=CARTESIAN_POINT('Ctrl Pts',(-84.817575714002,34.6504423105241,115.315215752614));
#51590=CARTESIAN_POINT('Ctrl Pts',(-87.5826092120844,32.9521373554897,115.157267229421));
#51591=CARTESIAN_POINT('Ctrl Pts',(-90.516234634425,34.3390374410077,114.999318706229));
#51592=CARTESIAN_POINT('Ctrl Pts',(-90.9586230327715,37.5536824401982,114.841370183036));
#51593=CARTESIAN_POINT('Ctrl Pts',(-88.5086743009781,39.6814515013034,114.683421659844));
#51594=CARTESIAN_POINT('Ctrl Pts',(-85.3876824423395,38.7931611297899,114.525473136651));
#51595=CARTESIAN_POINT('Ctrl Pts',(-84.4253558544066,35.6941971893785,114.367524613459));
#51596=CARTESIAN_POINT('Ctrl Pts',(-86.494206786618,33.1942960341126,114.209576090266));
#51597=CARTESIAN_POINT('Ctrl Pts',(-89.7184710199947,33.5600420104149,114.051627567074));
#51598=CARTESIAN_POINT('Ctrl Pts',(-91.1748062356975,36.4598243652332,113.893679043881));
#51599=CARTESIAN_POINT('Ctrl Pts',(-89.5427975860825,39.2644986303475,113.735730520689));
#51600=CARTESIAN_POINT('Ctrl Pts',(-86.302137678456,39.4311519498904,113.577781997497));
#51601=CARTESIAN_POINT('Ctrl Pts',(-84.3910342908472,36.808684827564,113.419833474304));
#51602=CARTESIAN_POINT('Ctrl Pts',(-85.5422267412189,33.7748084444496,113.261884951112));
#51603=CARTESIAN_POINT('Ctrl Pts',(-88.7119638467548,33.0802462459377,113.103936427919));
#51604=CARTESIAN_POINT('Ctrl Pts',(-91.0263413770617,35.3547366532648,112.945987904727));
#51605=CARTESIAN_POINT('Ctrl Pts',(-90.3869836140211,38.536068389606,112.788039381534));
#51606=CARTESIAN_POINT('Ctrl Pts',(-87.3735767961947,39.739824725452,112.630090858342));
#51607=CARTESIAN_POINT('Ctrl Pts',(-84.71828523668,37.874596401685,112.472142335149));
#51608=CARTESIAN_POINT('Ctrl Pts',(-84.8285810354468,34.6315292111096,112.314193811957));
#51609=CARTESIAN_POINT('Ctrl Pts',(-87.6044623462484,32.9510135419902,112.156245288764));
#51610=CARTESIAN_POINT('Ctrl Pts',(-90.5291220091947,34.3567218409445,111.998296765572));
#51611=CARTESIAN_POINT('Ctrl Pts',(-90.950860057395,37.5741411459941,111.840348242379));
#51612=CARTESIAN_POINT('Ctrl Pts',(-88.4872994291289,39.6861352266392,111.682399719187));
#51613=CARTESIAN_POINT('Ctrl Pts',(-85.3720756202366,38.7778232833473,111.524451195994));
#51614=CARTESIAN_POINT('Ctrl Pts',(-84.4296673129889,35.6727441300587,111.366502672802));
#51615=CARTESIAN_POINT('Ctrl Pts',(-86.51452745752,33.1861785983124,111.208554149609));
#51616=CARTESIAN_POINT('Ctrl Pts',(-89.7363767689262,33.5726200303412,111.050605626417));
#51617=CARTESIAN_POINT('Ctrl Pts',(-91.174062464699,36.4816937326644,110.892657103225));
#51618=CARTESIAN_POINT('Ctrl Pts',(-89.5240786496606,39.2758310551611,110.734708580032));
#51619=CARTESIAN_POINT('Ctrl Pts',(-86.2824154670296,39.4216726667553,110.57676005684));
#51620=CARTESIAN_POINT('Ctrl Pts',(-84.3881903335369,36.7869884150482,110.418811533647));
#51621=CARTESIAN_POINT('Ctrl Pts',(-85.5588395679429,33.7605663781691,110.260863010455));
#51622=CARTESIAN_POINT('Ctrl Pts',(-88.7329711121209,33.0863713778258,110.102914487262));
#51623=CARTESIAN_POINT('Ctrl Pts',(-91.0326964338223,35.3756755051439,109.94496596407));
#51624=CARTESIAN_POINT('Ctrl Pts',(-90.37292452271,38.5528363564853,109.787017440877));
#51625=CARTESIAN_POINT('Ctrl Pts',(-87.3518505130362,39.7372187705151,109.629068917685));
#51626=CARTESIAN_POINT('Ctrl Pts',(-84.7085903100746,37.8549793292252,109.471120394492));
#51627=CARTESIAN_POINT('Ctrl Pts',(-84.8397075846835,34.6126870920522,109.3131718713));
#51628=CARTESIAN_POINT('Ctrl Pts',(-87.6263222177776,32.9500302241897,109.155223348107));
#51629=CARTESIAN_POINT('Ctrl Pts',(-90.5418956246628,34.3744883102637,108.997274824915));
#51630=CARTESIAN_POINT('Ctrl Pts',(-90.942965757715,37.5945502335857,108.839326301722));
#51631=CARTESIAN_POINT('Ctrl Pts',(-88.4658951684941,39.6906802714687,108.68137777853));
#51632=CARTESIAN_POINT('Ctrl Pts',(-85.3565671007757,38.7623882891229,108.523429255338));
#51633=CARTESIAN_POINT('Ctrl Pts',(-84.4341174679698,35.65131354668,108.365480732145));
#51634=CARTESIAN_POINT('Ctrl Pts',(-86.5348977025807,33.178203428702,108.207532208953));
#51635=CARTESIAN_POINT('Ctrl Pts',(-89.7542057636271,33.5852888669862,108.04958368576));
#51636=CARTESIAN_POINT('Ctrl Pts',(-91.1731692815978,36.5036070183338,107.891635162568));
#51637=CARTESIAN_POINT('Ctrl Pts',(-89.5053058512089,39.286941983312,107.733686639375));
#51638=CARTESIAN_POINT('Ctrl Pts',(-86.2627164452819,39.4122747950501,107.575738116183));
#51639=CARTESIAN_POINT('Ctrl Pts',(-84.3855640350824,36.7648466838348,107.41778959299));
#51640=CARTESIAN_POINT('Ctrl Pts',(-85.5753822087549,33.7473103931842,107.259841069798));
#51641=CARTESIAN_POINT('Ctrl Pts',(-88.7542614462533,33.0908102932314,107.101892546605));
#51642=CARTESIAN_POINT('Ctrl Pts',(-91.0381784603491,35.4003899559926,106.943944023413));
#51643=CARTESIAN_POINT('Ctrl Pts',(-90.5846315306955,37.5056037940271,106.838645007951));
#51644=CARTESIAN_POINT('Ctrl Pts',(-89.9637526925908,38.2317895137629,106.78599550022));
#51645=CARTESIAN_POINT('Ctrl Pts',(-88.4666220147337,33.743793888745,122.21400449978));
#51646=CARTESIAN_POINT('Ctrl Pts',(-89.3304018103156,33.9747188791149,122.161354992049));
#51647=CARTESIAN_POINT('Ctrl Pts',(-90.7961451663071,35.3578786075719,122.056055976587));
#51648=CARTESIAN_POINT('Ctrl Pts',(-90.2590360718096,38.3497597522559,121.898107453395));
#51649=CARTESIAN_POINT('Ctrl Pts',(-87.4594165595049,39.5285558170738,121.740158930202));
#51650=CARTESIAN_POINT('Ctrl Pts',(-84.9422307613735,37.8320875443154,121.58221040701));
#51651=CARTESIAN_POINT('Ctrl Pts',(-84.9865439913999,34.7952741926615,121.424261883817));
#51652=CARTESIAN_POINT('Ctrl Pts',(-87.5537299517246,33.173059285919,121.266313360625));
#51653=CARTESIAN_POINT('Ctrl Pts',(-90.3154450465617,34.4354984958443,121.108364837432));
#51654=CARTESIAN_POINT('Ctrl Pts',(-90.7680929059277,37.4383447736177,120.95041631424));
#51655=CARTESIAN_POINT('Ctrl Pts',(-88.501093167899,39.4588296944782,120.792467791047));
#51656=CARTESIAN_POINT('Ctrl Pts',(-85.5699522530588,38.6651280856119,120.634519267855));
#51657=CARTESIAN_POINT('Ctrl Pts',(-84.6322043214011,35.7768227259254,120.476570744662));
#51658=CARTESIAN_POINT('Ctrl Pts',(-86.5380974030568,33.4126728245073,120.31862222147));
#51659=CARTESIAN_POINT('Ctrl Pts',(-89.5596062374444,33.7161711859333,120.160673698277));
#51660=CARTESIAN_POINT('Ctrl Pts',(-90.9572255066959,36.4121499431209,120.002725175085));
#51661=CARTESIAN_POINT('Ctrl Pts',(-89.4637739690721,39.0562447849546,119.844776651893));
#51662=CARTESIAN_POINT('Ctrl Pts',(-86.4333198585462,39.2511364855498,119.6868281287));
#51663=CARTESIAN_POINT('Ctrl Pts',(-84.6134831927505,36.8201221078114,119.528879605508));
#51664=CARTESIAN_POINT('Ctrl Pts',(-85.654254799713,33.9673287241466,119.370931082315));
#51665=CARTESIAN_POINT('Ctrl Pts',(-88.6119985852735,33.27929719944,119.212982559123));
#51666=CARTESIAN_POINT('Ctrl Pts',(-90.8050182788458,35.3798448559393,119.05503403593));
#51667=CARTESIAN_POINT('Ctrl Pts',(-90.2449695907927,38.3644689874854,118.897085512738));
#51668=CARTESIAN_POINT('Ctrl Pts',(-87.4396316486096,39.5271016824553,118.739136989545));
#51669=CARTESIAN_POINT('Ctrl Pts',(-84.9325190366115,37.8136192287988,118.581188466353));
#51670=CARTESIAN_POINT('Ctrl Pts',(-84.9967545132952,34.7775840576295,118.42323994316));
#51671=CARTESIAN_POINT('Ctrl Pts',(-87.5740977238439,33.171676920062,118.265291419968));
#51672=CARTESIAN_POINT('Ctrl Pts',(-90.3277499664502,34.4519249771215,118.107342896775));
#51673=CARTESIAN_POINT('Ctrl Pts',(-90.7610585008785,37.4575662520431,117.949394373583));
#51674=CARTESIAN_POINT('Ctrl Pts',(-88.4811556576462,39.4634772135036,117.79144585039));
#51675=CARTESIAN_POINT('Ctrl Pts',(-85.5551600045041,38.6509593996732,117.633497327198));
#51676=CARTESIAN_POINT('Ctrl Pts',(-84.6359828100684,35.7566980007872,117.475548804005));
#51677=CARTESIAN_POINT('Ctrl Pts',(-86.5570140810003,33.404831802211,117.317600280813));
#51678=CARTESIAN_POINT('Ctrl Pts',(-89.576513189482,33.7277263574279,117.159651757621));
#51679=CARTESIAN_POINT('Ctrl Pts',(-90.956792127762,36.4326229936112,117.001703234428));
#51680=CARTESIAN_POINT('Ctrl Pts',(-89.4463939617905,39.0670741964486,116.843754711236));
#51681=CARTESIAN_POINT('Ctrl Pts',(-86.4147507719692,39.2425031835377,116.685806188043));
#51682=CARTESIAN_POINT('Ctrl Pts',(-84.6105612352497,36.7998538277168,116.527857664851));
#51683=CARTESIAN_POINT('Ctrl Pts',(-85.6696291326311,33.9538020100865,116.369909141658));
#51684=CARTESIAN_POINT('Ctrl Pts',(-88.631729811652,33.284776354939,116.211960618466));
#51685=CARTESIAN_POINT('Ctrl Pts',(-90.8112166748635,35.3993620763011,116.054012095273));
#51686=CARTESIAN_POINT('Ctrl Pts',(-90.2320152694889,38.3803286128312,115.896063572081));
#51687=CARTESIAN_POINT('Ctrl Pts',(-87.4192698941663,39.5249242678565,115.738115048888));
#51688=CARTESIAN_POINT('Ctrl Pts',(-84.9232112349175,37.7953789722688,115.580166525696));
#51689=CARTESIAN_POINT('Ctrl Pts',(-85.0069397638907,34.7598188438351,115.422218002503));
#51690=CARTESIAN_POINT('Ctrl Pts',(-87.5945413703541,33.1704939286182,115.264269479311));
#51691=CARTESIAN_POINT('Ctrl Pts',(-90.3399163760726,34.4683967901131,115.106320956119));
#51692=CARTESIAN_POINT('Ctrl Pts',(-90.7539167601679,37.4767583777334,114.948372432926));
#51693=CARTESIAN_POINT('Ctrl Pts',(-88.461180965633,39.4679887351656,114.790423909734));
#51694=CARTESIAN_POINT('Ctrl Pts',(-85.5404628069659,38.6366998578597,114.632475386541));
#51695=CARTESIAN_POINT('Ctrl Pts',(-84.6398886090025,35.7365960883606,114.474526863349));
#51696=CARTESIAN_POINT('Ctrl Pts',(-86.5759816073101,33.397113311804,114.316578340156));
#51697=CARTESIAN_POINT('Ctrl Pts',(-89.5933451639302,33.7393894095416,114.158629816964));
#51698=CARTESIAN_POINT('Ctrl Pts',(-90.9562275110392,36.4530930536116,114.000681293771));
#51699=CARTESIAN_POINT('Ctrl Pts',(-89.4289446747066,39.0777916835012,113.842732770579));
#51700=CARTESIAN_POINT('Ctrl Pts',(-86.3962375524274,39.2337508780899,113.684784247386));
#51701=CARTESIAN_POINT('Ctrl Pts',(-84.6077694563542,36.7795671789286,113.526835724194));
#51702=CARTESIAN_POINT('Ctrl Pts',(-85.6850900153984,33.9403743054237,113.368887201001));
#51703=CARTESIAN_POINT('Ctrl Pts',(-88.6514254438984,33.2903820858341,113.210938677809));
#51704=CARTESIAN_POINT('Ctrl Pts',(-90.8172896258469,35.4189186970422,113.052990154617));
#51705=CARTESIAN_POINT('Ctrl Pts',(-90.2189593792529,38.39610473018,112.895041631424));
#51706=CARTESIAN_POINT('Ctrl Pts',(-87.3989225413111,39.5226161560218,112.737093108232));
#51707=CARTESIAN_POINT('Ctrl Pts',(-84.9140207454401,37.777079326053,112.579144585039));
#51708=CARTESIAN_POINT('Ctrl Pts',(-85.0172388750841,34.7421193959036,112.421196061847));
#51709=CARTESIAN_POINT('Ctrl Pts',(-87.6149921913326,33.1694422301058,112.263247538654));
#51710=CARTESIAN_POINT('Ctrl Pts',(-90.3519767694386,34.4849463840756,112.105299015462));
#51711=CARTESIAN_POINT('Ctrl Pts',(-90.7466519340567,37.4959042506569,111.947350492269));
#51712=CARTESIAN_POINT('Ctrl Pts',(-88.4411777169297,39.4723719063683,111.789401969077));
#51713=CARTESIAN_POINT('Ctrl Pts',(-85.5258574728992,38.622346239315,111.631453445884));
#51714=CARTESIAN_POINT('Ctrl Pts',(-84.6439234017677,35.716519669468,111.473504922692));
#51715=CARTESIAN_POINT('Ctrl Pts',(-86.5949983030236,33.3895167709551,111.315556399499));
#51716=CARTESIAN_POINT('Ctrl Pts',(-89.6101019029469,33.7511602993301,111.157607876307));
#51717=CARTESIAN_POINT('Ctrl Pts',(-90.9555314677429,36.4735590661704,110.999659353114));
#51718=CARTESIAN_POINT('Ctrl Pts',(-89.4114269303503,39.0883969078767,110.841710829922));
#51719=CARTESIAN_POINT('Ctrl Pts',(-86.3777809131116,39.2248798794979,110.683762306729));
#51720=CARTESIAN_POINT('Ctrl Pts',(-84.6051079954678,36.7592630227875,110.525813783537));
#51721=CARTESIAN_POINT('Ctrl Pts',(-85.7006367988817,33.9270461509502,110.367865260344));
#51722=CARTESIAN_POINT('Ctrl Pts',(-88.6710846753857,33.2961141686911,110.209916737152));
#51723=CARTESIAN_POINT('Ctrl Pts',(-90.8232368793229,35.4385139051282,110.05196821396));
#51724=CARTESIAN_POINT('Ctrl Pts',(-90.2058024582654,38.4117966984921,109.894019690767));
#51725=CARTESIAN_POINT('Ctrl Pts',(-87.3785904313232,39.5201774249231,109.736071167575));
#51726=CARTESIAN_POINT('Ctrl Pts',(-84.9049479411952,37.7587210789482,109.578122644382));
#51727=CARTESIAN_POINT('Ctrl Pts',(-85.0276514348956,34.7244863735275,109.42017412119));
#51728=CARTESIAN_POINT('Ctrl Pts',(-87.6354493173403,33.168522011699,109.262225597997));
#51729=CARTESIAN_POINT('Ctrl Pts',(-90.3639307034249,34.5015727810372,109.104277074805));
#51730=CARTESIAN_POINT('Ctrl Pts',(-90.7392642107077,37.5150036893709,108.946328551612));
#51731=CARTESIAN_POINT('Ctrl Pts',(-88.4211469653162,39.4766252961773,108.78838002842));
#51732=CARTESIAN_POINT('Ctrl Pts',(-85.5113441334047,38.607901706951,108.630431505227));
#51733=CARTESIAN_POINT('Ctrl Pts',(-84.6480879907992,35.6964642842379,108.472482982035));
#51734=CARTESIAN_POINT('Ctrl Pts',(-86.6140613917273,33.3820533670904,108.314534458842));
#51735=CARTESIAN_POINT('Ctrl Pts',(-89.6267868130435,33.7630161781385,108.15658593565));
#51736=CARTESIAN_POINT('Ctrl Pts',(-90.9546956001019,36.4940661787389,107.998637412457));
#51737=CARTESIAN_POINT('Ctrl Pts',(-89.3938587802843,39.0987948490057,107.840688889265));
#51738=CARTESIAN_POINT('Ctrl Pts',(-86.3593459753956,39.2160850681732,107.682740366072));
#51739=CARTESIAN_POINT('Ctrl Pts',(-84.6026502262925,36.7385421240001,107.52479184288));
#51740=CARTESIAN_POINT('Ctrl Pts',(-85.7161179002754,33.9146408010454,107.366843319688));
#51741=CARTESIAN_POINT('Ctrl Pts',(-88.6910088111477,33.3002682393896,107.208894796495));
#51742=CARTESIAN_POINT('Ctrl Pts',(-90.8283671248183,35.4616424324185,107.050946273303));
#51743=CARTESIAN_POINT('Ctrl Pts',(-90.4039242511271,37.4317649329324,106.945647257841));
#51744=CARTESIAN_POINT('Ctrl Pts',(-89.8228871389138,38.111351395911,106.89299775011));
#51745=CARTESIAN_POINT('Ctrl Pts',(-88.4187555865477,33.9228392726486,122.321006749669));
#51746=CARTESIAN_POINT('Ctrl Pts',(-89.2233059850348,34.1379297320145,122.268357241939));
#51747=CARTESIAN_POINT('Ctrl Pts',(-90.5885432910872,35.4262461714511,122.163058226477));
#51748=CARTESIAN_POINT('Ctrl Pts',(-90.0882637774666,38.212973968852,122.005109703285));
#51749=CARTESIAN_POINT('Ctrl Pts',(-87.4806142286375,39.3109399649718,121.847161180092));
#51750=CARTESIAN_POINT('Ctrl Pts',(-85.1360319088018,37.7307985541058,121.6892126569));
#51751=CARTESIAN_POINT('Ctrl Pts',(-85.1773065797982,34.9022195520257,121.531264133707));
#51752=CARTESIAN_POINT('Ctrl Pts',(-87.5684605497497,33.3912399524484,121.373315610515));
#51753=CARTESIAN_POINT('Ctrl Pts',(-90.1408047877418,34.5671136816166,121.215367087322));
#51754=CARTESIAN_POINT('Ctrl Pts',(-90.5624145747381,37.3640547327214,121.05741856413));
#51755=CARTESIAN_POINT('Ctrl Pts',(-88.4508630520817,39.2459949639355,120.899470040937));
#51756=CARTESIAN_POINT('Ctrl Pts',(-85.7207105258027,38.5067174895613,120.741521517745));
#51757=CARTESIAN_POINT('Ctrl Pts',(-84.8472639877449,35.8164632836006,120.583572994552));
#51758=CARTESIAN_POINT('Ctrl Pts',(-86.6224699443586,33.6144231861152,120.42562447136));
#51759=CARTESIAN_POINT('Ctrl Pts',(-89.436793860214,33.8971106590967,120.267675948167));
#51760=CARTESIAN_POINT('Ctrl Pts',(-90.7385783494564,36.4082261013683,120.109727424975));
#51761=CARTESIAN_POINT('Ctrl Pts',(-89.3475328123158,38.8710153093537,119.951778901782));
#51762=CARTESIAN_POINT('Ctrl Pts',(-86.5248769980782,39.0525432823135,119.79383037859));
#51763=CARTESIAN_POINT('Ctrl Pts',(-84.8298265672435,36.7882236069272,119.635881855398));
#51764=CARTESIAN_POINT('Ctrl Pts',(-85.7992324452217,34.1310463201136,119.477933332205));
#51765=CARTESIAN_POINT('Ctrl Pts',(-88.5541636828665,33.4901931302084,119.319984809013));
#51766=CARTESIAN_POINT('Ctrl Pts',(-90.5968079741295,35.446706193748,119.16203628582));
#51767=CARTESIAN_POINT('Ctrl Pts',(-90.0751618353219,38.2266745915407,119.004087762628));
#51768=CARTESIAN_POINT('Ctrl Pts',(-87.4621859694605,39.3095855403919,118.846139239435));
#51769=CARTESIAN_POINT('Ctrl Pts',(-85.1269861171924,37.7135966113371,118.688190716243));
#51770=CARTESIAN_POINT('Ctrl Pts',(-85.186816966012,34.8857424298909,118.53024219305));
#51771=CARTESIAN_POINT('Ctrl Pts',(-87.5874317033455,33.3899523754446,118.372293669858));
#51772=CARTESIAN_POINT('Ctrl Pts',(-90.1522659590382,34.5824137987586,118.214345146665));
#51773=CARTESIAN_POINT('Ctrl Pts',(-90.5558625189777,37.3819581940037,118.056396623473));
#51774=CARTESIAN_POINT('Ctrl Pts',(-88.4322926572878,39.2503238024924,117.89844810028));
#51775=CARTESIAN_POINT('Ctrl Pts',(-85.7069325820144,38.4935203506883,117.740499577088));
#51776=CARTESIAN_POINT('Ctrl Pts',(-84.8507833853719,35.7977185112499,117.582551053895));
#51777=CARTESIAN_POINT('Ctrl Pts',(-86.6400895053339,33.6071198228677,117.424602530703));
#51778=CARTESIAN_POINT('Ctrl Pts',(-89.4525415022272,33.907873492261,117.26665400751));
#51779=CARTESIAN_POINT('Ctrl Pts',(-90.7381746873242,36.4272953143951,117.108705484318));
#51780=CARTESIAN_POINT('Ctrl Pts',(-89.3313445524658,38.8811021478944,116.950756961125));
#51781=CARTESIAN_POINT('Ctrl Pts',(-86.5075811941226,39.0445019659854,116.792808437933));
#51782=CARTESIAN_POINT('Ctrl Pts',(-84.8271049684244,36.7693451231862,116.634859914741));
#51783=CARTESIAN_POINT('Ctrl Pts',(-85.8135525598376,34.1184471330952,116.476911391548));
#51784=CARTESIAN_POINT('Ctrl Pts',(-88.5725419386751,33.4952965799101,116.318962868356));
#51785=CARTESIAN_POINT('Ctrl Pts',(-90.602581346014,35.4648851179365,116.161014345163));
#51786=CARTESIAN_POINT('Ctrl Pts',(-90.0630957920775,38.2414467220733,116.003065821971));
#51787=CARTESIAN_POINT('Ctrl Pts',(-87.4432204209086,39.3075574311537,115.845117298778));
#51788=CARTESIAN_POINT('Ctrl Pts',(-85.1183165516385,37.6966070895461,115.687168775586));
#51789=CARTESIAN_POINT('Ctrl Pts',(-85.1963038137795,34.869195377146,115.529220252393));
#51790=CARTESIAN_POINT('Ctrl Pts',(-87.6064735286238,33.3888505017467,115.371271729201));
#51791=CARTESIAN_POINT('Ctrl Pts',(-90.1635981177202,34.5977561392184,115.213323206008));
#51792=CARTESIAN_POINT('Ctrl Pts',(-90.5492104875641,37.3998343152686,115.055374682816));
#51793=CARTESIAN_POINT('Ctrl Pts',(-88.413687630288,39.2545259690279,114.897426159623));
#51794=CARTESIAN_POINT('Ctrl Pts',(-85.6932431715923,38.4802385859295,114.739477636431));
#51795=CARTESIAN_POINT('Ctrl Pts',(-84.8544213635984,35.7789949873425,114.581529113238));
#51796=CARTESIAN_POINT('Ctrl Pts',(-86.6577564280022,33.5999305894954,114.423580590046));
#51797=CARTESIAN_POINT('Ctrl Pts',(-89.4682193078656,33.9187368086683,114.265632066854));
#51798=CARTESIAN_POINT('Ctrl Pts',(-90.737648786381,36.4463617419899,114.107683543661));
#51799=CARTESIAN_POINT('Ctrl Pts',(-89.3150917633309,38.891084736655,113.949735020469));
#51800=CARTESIAN_POINT('Ctrl Pts',(-86.4903374263987,39.0363498062895,113.791786497276));
#51801=CARTESIAN_POINT('Ctrl Pts',(-84.8245046218612,36.7504495302932,113.633837974084));
#51802=CARTESIAN_POINT('Ctrl Pts',(-85.827953289578,34.1059401663978,113.475889450891));
#51803=CARTESIAN_POINT('Ctrl Pts',(-88.5908870410419,33.5005179257306,113.317940927699));
#51804=CARTESIAN_POINT('Ctrl Pts',(-90.6082378746323,35.4831007408195,113.159992404506));
#51805=CARTESIAN_POINT('Ctrl Pts',(-90.0509351444846,38.2561410707539,113.002043881314));
#51806=CARTESIAN_POINT('Ctrl Pts',(-87.4242682864277,39.3054075865917,112.844095358121));
#51807=CARTESIAN_POINT('Ctrl Pts',(-85.1097562542002,37.6795622504211,112.686146834929));
#51808=CARTESIAN_POINT('Ctrl Pts',(-85.2058967147215,34.8527095806976,112.528198311736));
#51809=CARTESIAN_POINT('Ctrl Pts',(-87.6255220364168,33.3878709182214,112.370249788544));
#51810=CARTESIAN_POINT('Ctrl Pts',(-90.1748315296826,34.6131709272066,112.212301265351));
#51811=CARTESIAN_POINT('Ctrl Pts',(-90.5424438107183,37.4176673553198,112.054352742159));
#51812=CARTESIAN_POINT('Ctrl Pts',(-88.3950560047306,39.2586085860974,111.896404218966));
#51813=CARTESIAN_POINT('Ctrl Pts',(-85.6796393255617,38.4668691952829,111.738455695774));
#51814=CARTESIAN_POINT('Ctrl Pts',(-84.8581794905466,35.7602952088772,111.580507172582));
#51815=CARTESIAN_POINT('Ctrl Pts',(-86.6754691485269,33.5928549435978,111.422558649389));
#51816=CARTESIAN_POINT('Ctrl Pts',(-89.4838270369679,33.929700568319,111.264610126197));
#51817=CARTESIAN_POINT('Ctrl Pts',(-90.7370004707867,36.4654243996764,111.106661603004));
#51818=CARTESIAN_POINT('Ctrl Pts',(-89.2987752110399,38.9009627605923,110.948713079812));
#51819=CARTESIAN_POINT('Ctrl Pts',(-86.4731463591935,39.0280870922405,110.790764556619));
#51820=CARTESIAN_POINT('Ctrl Pts',(-84.8220256573987,36.7315376305268,110.632816033427));
#51821=CARTESIAN_POINT('Ctrl Pts',(-85.8424340298206,34.0935259237314,110.474867510234));
#51822=CARTESIAN_POINT('Ctrl Pts',(-88.6091982386503,33.5058569595565,110.316918987042));
#51823=CARTESIAN_POINT('Ctrl Pts',(-90.6137773248237,35.5013523051125,110.158970463849));
#51824=CARTESIAN_POINT('Ctrl Pts',(-90.0386803938207,38.270757040499,110.001021940657));
#51825=CARTESIAN_POINT('Ctrl Pts',(-87.4053303496102,39.303136079331,109.843073417464));
#51826=CARTESIAN_POINT('Ctrl Pts',(-85.1013055723159,37.6624628286712,109.685124894272));
#51827=CARTESIAN_POINT('Ctrl Pts',(-85.2155952851076,34.8362856550028,109.52717637108));
#51828=CARTESIAN_POINT('Ctrl Pts',(-87.6445764169031,33.3870137992084,109.369227847887));
#51829=CARTESIAN_POINT('Ctrl Pts',(-90.1859657821869,34.6286572518108,109.211279324695));
#51830=CARTESIAN_POINT('Ctrl Pts',(-90.5355626637006,37.435457145156,109.053330801502));
#51831=CARTESIAN_POINT('Ctrl Pts',(-88.3763987621381,39.2625703208859,108.89538227831));
#51832=CARTESIAN_POINT('Ctrl Pts',(-85.6661211660339,38.4534151247791,108.737433755117));
#51833=CARTESIAN_POINT('Ctrl Pts',(-84.8620585136285,35.7416150217957,108.579485231925));
#51834=CARTESIAN_POINT('Ctrl Pts',(-86.6932250808741,33.5859033054787,108.421536708732));
#51835=CARTESIAN_POINT('Ctrl Pts',(-89.49936786246,33.9407434892909,108.26358818554));
#51836=CARTESIAN_POINT('Ctrl Pts',(-90.7362219186059,36.4845253391441,108.105639662347));
#51837=CARTESIAN_POINT('Ctrl Pts',(-89.2824117093597,38.9106477146993,107.947691139155));
#51838=CARTESIAN_POINT('Ctrl Pts',(-86.4559755055092,39.0198953412964,107.789742615962));
#51839=CARTESIAN_POINT('Ctrl Pts',(-84.8197364175027,36.7122375641654,107.63179409277));
#51840=CARTESIAN_POINT('Ctrl Pts',(-85.8568535917958,34.0819712089066,107.473845569577));
#51841=CARTESIAN_POINT('Ctrl Pts',(-88.6277561760423,33.5097261855478,107.315897046385));
#51842=CARTESIAN_POINT('Ctrl Pts',(-90.6185557892874,35.5228949088443,107.157948523193));
#51843=CARTESIAN_POINT('Ctrl Pts',(-90.2232169715586,37.3579260718377,107.052649507731));
#51844=CARTESIAN_POINT('Ctrl Pts',(-89.6820215852368,37.9909132780591,107.));
#51845=CARTESIAN_POINT('Ctrl Pts',(-90.2835503128821,36.3566878611388,121.112583302492));
#51846=CARTESIAN_POINT('Ctrl Pts',(-90.2854631783966,36.64824070958,121.094195056371));
#51847=CARTESIAN_POINT('Ctrl Pts',(-90.2385918845246,36.9391987080589,121.07580681025));
#51848=CARTESIAN_POINT('Ctrl Pts',(-90.1402210231293,37.211554596073,121.05741856413));
#51849=CARTESIAN_POINT('Ctrl Pts',(-89.858564067186,37.9913681431261,121.004769056399));
#51850=CARTESIAN_POINT('Ctrl Pts',(-89.1547135596339,38.6186815535308,120.952119548668));
#51851=CARTESIAN_POINT('Ctrl Pts',(-88.3477628848113,38.8091253463374,120.899470040937));
#51852=CARTESIAN_POINT('Ctrl Pts',(-87.5408122099887,38.9995691391441,120.846820533206));
#51853=CARTESIAN_POINT('Ctrl Pts',(-86.6307613678957,38.7531433143527,120.794171025476));
#51854=CARTESIAN_POINT('Ctrl Pts',(-86.0301615238396,38.1815547009635,120.741521517745));
#51855=CARTESIAN_POINT('Ctrl Pts',(-85.4295616797834,37.6099660875744,120.688872010014));
#51856=CARTESIAN_POINT('Ctrl Pts',(-85.1384128337641,36.7132146855875,120.636222502283));
#51857=CARTESIAN_POINT('Ctrl Pts',(-85.2887060701901,35.8978323016798,120.583572994552));
#51858=CARTESIAN_POINT('Ctrl Pts',(-85.4389993066161,35.0824499177722,120.530923486821));
#51859=CARTESIAN_POINT('Ctrl Pts',(-86.0307346254874,34.3484365519437,120.478273979091));
#51860=CARTESIAN_POINT('Ctrl Pts',(-86.7956562708989,34.0285444478597,120.42562447136));
#51861=CARTESIAN_POINT('Ctrl Pts',(-87.5605779163104,33.7086523437757,120.372974963629));
#51862=CARTESIAN_POINT('Ctrl Pts',(-88.4986858882622,33.8028815014362,120.320325455898));
#51863=CARTESIAN_POINT('Ctrl Pts',(-89.1847039557785,34.268515320645,120.267675948167));
#51864=CARTESIAN_POINT('Ctrl Pts',(-89.8583180860134,34.7257299844947,120.215978399609));
#51865=CARTESIAN_POINT('Ctrl Pts',(-90.2888760052472,35.5410399476632,120.16428085105));
#51866=CARTESIAN_POINT('Ctrl Pts',(-90.2901412986672,36.3551993258176,120.112583302492));
#51867=CARTESIAN_POINT('Ctrl Pts',(-88.5623548711056,33.385703120938,122.));
#51868=CARTESIAN_POINT('Ctrl Pts',(-88.655404902989,33.4197412382527,122.));
#51869=CARTESIAN_POINT('Ctrl Pts',(-88.746389770168,33.4585480581623,122.));
#51870=CARTESIAN_POINT('Ctrl Pts',(-88.8351009878334,33.5017952570346,122.));
#51871=CARTESIAN_POINT('Ctrl Pts',(-88.9257791769406,33.5460013651335,122.));
#51872=CARTESIAN_POINT('Ctrl Pts',(-89.0140824405661,33.5948475625466,122.));
#51873=CARTESIAN_POINT('Ctrl Pts',(-89.099759199117,33.6480287402599,122.));
#51874=CARTESIAN_POINT('Ctrl Pts',(-89.1821906340797,33.6991954844978,122.));
#51875=CARTESIAN_POINT('Ctrl Pts',(-89.2621910564892,33.7543758980026,122.));
#51876=CARTESIAN_POINT('Ctrl Pts',(-89.3395034395237,33.8133282931028,122.));
#51877=CARTESIAN_POINT('Ctrl Pts',(-89.407151774679,33.8649116388154,122.));
#51878=CARTESIAN_POINT('Ctrl Pts',(-89.472741789452,33.9193836052977,122.));
#51879=CARTESIAN_POINT('Ctrl Pts',(-89.5360766751279,33.9765949798929,122.));
#51880=CARTESIAN_POINT('Ctrl Pts',(-89.5502131428364,33.9893646682076,122.));
#51881=CARTESIAN_POINT('Ctrl Pts',(-89.56423990469,34.0022735672698,122.));
#51882=CARTESIAN_POINT('Ctrl Pts',(-89.5781351874061,34.0153014850048,122.));
#51883=CARTESIAN_POINT('Ctrl Pts',(-89.650565279181,34.0832103787249,122.));
#51884=CARTESIAN_POINT('Ctrl Pts',(-89.7195296835776,34.1544411891477,122.));
#51885=CARTESIAN_POINT('Ctrl Pts',(-89.7847884509537,34.2287031921864,122.));
#51886=CARTESIAN_POINT('Ctrl Pts',(-89.8496881991125,34.3025566449677,122.));
#51887=CARTESIAN_POINT('Ctrl Pts',(-89.9109234574517,34.3794088270275,122.));
#51888=CARTESIAN_POINT('Ctrl Pts',(-89.9682146052408,34.4590005543629,122.));
#51889=CARTESIAN_POINT('Ctrl Pts',(-90.0233775150845,34.5356356271226,122.));
#51890=CARTESIAN_POINT('Ctrl Pts',(-90.0748840644318,34.6148112269046,122.));
#51891=CARTESIAN_POINT('Ctrl Pts',(-90.1224398052449,34.6963095794444,122.));
#51892=CARTESIAN_POINT('Ctrl Pts',(-90.142386136171,34.7304924789619,122.));
#51893=CARTESIAN_POINT('Ctrl Pts',(-90.1616368636099,34.7650841083823,122.));
#51894=CARTESIAN_POINT('Ctrl Pts',(-90.180167677375,34.8000686960743,122.));
#51895=CARTESIAN_POINT('Ctrl Pts',(-90.1930502182209,34.8243898287366,122.));
#51896=CARTESIAN_POINT('Ctrl Pts',(-90.2055847945378,34.8489008796607,122.));
#51897=CARTESIAN_POINT('Ctrl Pts',(-90.2177627724607,34.8735965555594,122.));
#51898=CARTESIAN_POINT('Ctrl Pts',(-90.2256711134462,34.8896338506758,122.));
#51899=CARTESIAN_POINT('Ctrl Pts',(-90.2334301790788,34.9057516180668,122.));
#51900=CARTESIAN_POINT('Ctrl Pts',(-90.241027428963,34.9219262186558,122.));
#51901=CARTESIAN_POINT('Ctrl Pts',(-90.2831477278551,35.0116006431706,122.));
#51902=CARTESIAN_POINT('Ctrl Pts',(-90.3203691942033,35.1031586544706,122.));
#51903=CARTESIAN_POINT('Ctrl Pts',(-90.3524005445713,35.1963278865285,122.));
#51904=CARTESIAN_POINT('Ctrl Pts',(-90.3822802989988,35.2832387954382,122.));
#51905=CARTESIAN_POINT('Ctrl Pts',(-90.4076436024182,35.3715525302143,122.));
#51906=CARTESIAN_POINT('Ctrl Pts',(-90.4282034771338,35.4610567033496,122.));
#51907=CARTESIAN_POINT('Ctrl Pts',(-90.4296839626272,35.4675017635338,122.));
#51908=CARTESIAN_POINT('Ctrl Pts',(-90.4311395187566,35.4739529975641,122.));
#51909=CARTESIAN_POINT('Ctrl Pts',(-90.4325700277436,35.4804103264538,122.));
#51910=CARTESIAN_POINT('Ctrl Pts',(-90.4531762477541,35.5734269666833,122.));
#51911=CARTESIAN_POINT('Ctrl Pts',(-90.4685894434994,35.6677092665185,122.));
#51912=CARTESIAN_POINT('Ctrl Pts',(-90.4788865349184,35.7628493605361,122.));
#51913=CARTESIAN_POINT('Ctrl Pts',(-90.484683054651,35.8164063709481,122.));
#51914=CARTESIAN_POINT('Ctrl Pts',(-90.4888574145047,35.8702350170487,122.));
#51915=CARTESIAN_POINT('Ctrl Pts',(-90.4914165740776,35.9242599040958,122.));
#51916=CARTESIAN_POINT('Ctrl Pts',(-90.4920774570878,35.9382114100347,122.));
#51917=CARTESIAN_POINT('Ctrl Pts',(-90.4926305034956,35.9521754040169,122.));
#51918=CARTESIAN_POINT('Ctrl Pts',(-90.4930755917552,35.9661372181595,122.));
#51919=CARTESIAN_POINT('Ctrl Pts',(-90.4960470047878,36.0593464089312,122.));
#51920=CARTESIAN_POINT('Ctrl Pts',(-90.4942192639962,36.152613832859,122.));
#51921=CARTESIAN_POINT('Ctrl Pts',(-90.4877272636018,36.2455644111571,122.));
#51922=CARTESIAN_POINT('Ctrl Pts',(-90.481224468874,36.3386695395895,122.));
#51923=CARTESIAN_POINT('Ctrl Pts',(-90.4700415130326,36.4314577475258,122.));
#51924=CARTESIAN_POINT('Ctrl Pts',(-90.4542630315823,36.5235399863453,122.));
#51925=CARTESIAN_POINT('Ctrl Pts',(-90.4387101459247,36.6143056621148,122.));
#51926=CARTESIAN_POINT('Ctrl Pts',(-90.4186917450187,36.7043862559761,122.));
#51927=CARTESIAN_POINT('Ctrl Pts',(-90.3942458608461,36.7933839699538,122.));
#51928=CARTESIAN_POINT('Ctrl Pts',(-90.3851470966912,36.8265089411795,122.));
#51929=CARTESIAN_POINT('Ctrl Pts',(-90.3754345818515,36.8594835809755,122.));
#51930=CARTESIAN_POINT('Ctrl Pts',(-90.3651089158779,36.8922861120309,122.));
#51931=CARTESIAN_POINT('Ctrl Pts',(-90.3581143964109,36.9145062712557,122.));
#51932=CARTESIAN_POINT('Ctrl Pts',(-90.3508385119144,36.9366474415144,122.));
#51933=CARTESIAN_POINT('Ctrl Pts',(-90.3432812696287,36.9587026404511,122.));
#51934=CARTESIAN_POINT('Ctrl Pts',(-90.3387652071146,36.971882402776,122.));
#51935=CARTESIAN_POINT('Ctrl Pts',(-90.3341490168439,36.9850302917945,122.));
#51936=CARTESIAN_POINT('Ctrl Pts',(-90.3294361706385,36.9981356694608,122.));
#51937=CARTESIAN_POINT('Ctrl Pts',(-90.2978044186066,37.0860965403558,122.));
#51938=CARTESIAN_POINT('Ctrl Pts',(-90.2617834495289,37.1722596645947,122.));
#51939=CARTESIAN_POINT('Ctrl Pts',(-90.2214378271335,37.2562107993322,122.));
#51940=CARTESIAN_POINT('Ctrl Pts',(-90.1911786103369,37.3191741503854,122.));
#51941=CARTESIAN_POINT('Ctrl Pts',(-90.1584857287241,37.3808927654021,122.));
#51942=CARTESIAN_POINT('Ctrl Pts',(-90.1233704583289,37.4411763545704,122.));
#51943=CARTESIAN_POINT('Ctrl Pts',(-90.1099010949563,37.4642996726816,122.));
#51944=CARTESIAN_POINT('Ctrl Pts',(-90.0960751912912,37.4872116937309,122.));
#51945=CARTESIAN_POINT('Ctrl Pts',(-90.0818929032749,37.5099010346059,122.));
#51946=CARTESIAN_POINT('Ctrl Pts',(-90.0717687163118,37.5260980776235,122.));
#51947=CARTESIAN_POINT('Ctrl Pts',(-90.0614620799691,37.5421827090904,122.));
#51948=CARTESIAN_POINT('Ctrl Pts',(-90.0509831258029,37.5581357839754,122.));
#51949=CARTESIAN_POINT('Ctrl Pts',(-90.0037965482649,37.6299722471464,122.));
#51950=CARTESIAN_POINT('Ctrl Pts',(-89.9530750443141,37.6992152601097,122.));
#51951=CARTESIAN_POINT('Ctrl Pts',(-89.8988515052545,37.7655128239611,122.));
#51952=CARTESIAN_POINT('Ctrl Pts',(-89.8500550823629,37.8251748087463,122.));
#51953=CARTESIAN_POINT('Ctrl Pts',(-89.7984219626668,37.882451366736,122.));
#51954=CARTESIAN_POINT('Ctrl Pts',(-89.7439556248374,37.9370561588495,122.));
#51955=CARTESIAN_POINT('Ctrl Pts',(-89.7248730539468,37.9561872379343,122.));
#51956=CARTESIAN_POINT('Ctrl Pts',(-89.7054425381007,37.9749900687628,122.));
#51957=CARTESIAN_POINT('Ctrl Pts',(-89.6856746522268,37.9934601639124,122.));
#51958=CARTESIAN_POINT('Origin',(-87.7685555885722,36.3549260746835,114.));
#51959=CARTESIAN_POINT('Origin',(36.3549260746835,-87.7685555885722,106.));
#51960=CARTESIAN_POINT('Origin',(-87.7685555885722,-36.3549260746835,106.));
#51961=CARTESIAN_POINT('Origin',(-36.3549260746835,87.7685555885722,106.));
#51962=CARTESIAN_POINT('Origin',(87.7685555885722,36.3549260746835,106.));
#51963=CARTESIAN_POINT('Origin',(36.3549260746835,87.7685555885722,106.));
#51964=CARTESIAN_POINT('Origin',(-87.7685555885722,36.3549260746835,106.));
#51965=CARTESIAN_POINT('Origin',(-36.3549260746835,-87.7685555885722,106.));
#51966=CARTESIAN_POINT('Origin',(87.7685555885722,-36.3549260746835,106.));
#51967=CARTESIAN_POINT('Origin',(-81.317279836453,-81.3172798364529,5.));
#51968=CARTESIAN_POINT('',(-86.817279836453,-81.3172798364529,10.));
#51969=CARTESIAN_POINT('Origin',(-81.317279836453,-81.3172798364529,10.));
#51970=CARTESIAN_POINT('',(-86.817279836453,-81.3172798364529,0.));
#51971=CARTESIAN_POINT('',(-86.817279836453,-81.3172798364529,5.));
#51972=CARTESIAN_POINT('Origin',(-81.317279836453,-81.3172798364529,0.));
#51973=CARTESIAN_POINT('Origin',(81.317279836453,81.3172798364529,5.));
#51974=CARTESIAN_POINT('',(75.817279836453,81.3172798364529,10.));
#51975=CARTESIAN_POINT('Origin',(81.317279836453,81.3172798364529,10.));
#51976=CARTESIAN_POINT('',(75.817279836453,81.3172798364529,0.));
#51977=CARTESIAN_POINT('',(75.817279836453,81.3172798364529,5.));
#51978=CARTESIAN_POINT('Origin',(81.317279836453,81.3172798364529,0.));
#51979=CARTESIAN_POINT('Origin',(-81.3172798364529,81.317279836453,5.));
#51980=CARTESIAN_POINT('',(-86.817279836453,81.317279836453,10.));
#51981=CARTESIAN_POINT('Origin',(-81.3172798364529,81.317279836453,10.));
#51982=CARTESIAN_POINT('',(-86.817279836453,81.317279836453,0.));
#51983=CARTESIAN_POINT('',(-86.817279836453,81.317279836453,5.));
#51984=CARTESIAN_POINT('Origin',(-81.3172798364529,81.317279836453,0.));
#51985=CARTESIAN_POINT('Origin',(81.3172798364529,-81.317279836453,5.));
#51986=CARTESIAN_POINT('',(75.817279836453,-81.317279836453,10.));
#51987=CARTESIAN_POINT('Origin',(81.3172798364529,-81.317279836453,10.));
#51988=CARTESIAN_POINT('',(75.817279836453,-81.317279836453,0.));
#51989=CARTESIAN_POINT('',(75.817279836453,-81.317279836453,5.));
#51990=CARTESIAN_POINT('Origin',(81.3172798364529,-81.317279836453,0.));
#51991=CARTESIAN_POINT('Origin',(0.,0.,6.));
#51992=CARTESIAN_POINT('',(-18.,2.20436423846524E-15,10.));
#51993=CARTESIAN_POINT('Origin',(0.,0.,10.));
#51994=CARTESIAN_POINT('',(-18.,2.20436423846524E-15,2.));
#51995=CARTESIAN_POINT('',(-18.,2.20436423846524E-15,6.));
#51996=CARTESIAN_POINT('Origin',(0.,0.,2.));
#51997=CARTESIAN_POINT('Origin',(0.,0.,2.));
#51998=CARTESIAN_POINT('',(-17.,-2.0818995585505E-15,2.));
#51999=CARTESIAN_POINT('Origin',(0.,0.,2.));
#52000=CARTESIAN_POINT('Origin',(0.,0.,10.));
#52001=CARTESIAN_POINT('',(-90.,-1.10218211923262E-14,122.));
#52002=CARTESIAN_POINT('Origin',(0.,0.,122.));
#52003=CARTESIAN_POINT('',(-90.,-1.10218211923262E-14,10.));
#52004=CARTESIAN_POINT('',(-90.,-1.10218211923262E-14,10.));
#52005=CARTESIAN_POINT('',(-90.,-1.10218211923262E-14,10.));
#52006=CARTESIAN_POINT('',(-90.,-1.10218211923262E-14,10.));
#52007=CARTESIAN_POINT('',(-90.,-1.10218211923262E-14,10.));
#52008=CARTESIAN_POINT('Origin',(0.,0.,10.));
#52009=CARTESIAN_POINT('Origin',(0.,0.,10.));
#52010=CARTESIAN_POINT('',(-100.,-1.22464679914735E-14,122.));
#52011=CARTESIAN_POINT('Origin',(0.,0.,122.));
#52012=CARTESIAN_POINT('',(-100.,-1.22464679914735E-14,10.));
#52013=CARTESIAN_POINT('',(-100.,-1.22464679914735E-14,10.));
#52014=CARTESIAN_POINT('',(-100.,-1.22464679914735E-14,10.));
#52015=CARTESIAN_POINT('',(-100.,-1.22464679914735E-14,10.));
#52016=CARTESIAN_POINT('',(-100.,-1.22464679914735E-14,10.));
#52017=CARTESIAN_POINT('Origin',(0.,0.,10.));
#52018=CARTESIAN_POINT('Origin',(0.,0.,122.));
#52019=CARTESIAN_POINT('Origin',(0.,0.,10.));
#52020=CARTESIAN_POINT('',(-140.,1.71450551880629E-14,10.));
#52021=CARTESIAN_POINT('Origin',(0.,0.,10.));
#52022=CARTESIAN_POINT('Origin',(0.,0.,0.));
#52023=CARTESIAN_POINT('',(-17.,-2.0818995585505E-15,0.));
#52024=CARTESIAN_POINT('',(-17.,-2.0818995585505E-15,0.));
#52025=CARTESIAN_POINT('Origin',(0.,0.,0.));
#52026=CARTESIAN_POINT('Origin',(0.,0.,0.));
#52027=CARTESIAN_POINT('',(-140.,1.71450551880629E-14,0.));
#52028=CARTESIAN_POINT('',(-140.,-1.71450551880629E-14,0.));
#52029=CARTESIAN_POINT('Origin',(0.,0.,0.));
#52030=CARTESIAN_POINT('Origin',(0.,0.,10.));
#52031=CARTESIAN_POINT('Origin',(0.,0.,0.));
#259182=UNCERTAINTY_MEASURE_WITH_UNIT(LENGTH_MEASURE(0.01),#259225,
'DISTANCE_ACCURACY_VALUE',
'Maximum model space distance between geometric entities at asserted c
onnectivities');
#259202=UNCERTAINTY_MEASURE_WITH_UNIT(LENGTH_MEASURE(0.01),#259225,
'DISTANCE_ACCURACY_VALUE',
'Maximum model space distance between geometric entities at asserted c
onnectivities');
#259204=(
GEOMETRIC_REPRESENTATION_CONTEXT(3)
GLOBAL_UNCERTAINTY_ASSIGNED_CONTEXT((#259182))
GLOBAL_UNIT_ASSIGNED_CONTEXT((#259225,#259227,#259228))
REPRESENTATION_CONTEXT('','3D')
);
#259224=(
GEOMETRIC_REPRESENTATION_CONTEXT(3)
GLOBAL_UNCERTAINTY_ASSIGNED_CONTEXT((#259202))
GLOBAL_UNIT_ASSIGNED_CONTEXT((#259225,#259227,#259228))
REPRESENTATION_CONTEXT('','3D')
);
#259225=(
LENGTH_UNIT()
NAMED_UNIT(*)
SI_UNIT(.MILLI.,.METRE.)
);
#259227=(
NAMED_UNIT(*)
PLANE_ANGLE_UNIT()
SI_UNIT($,.RADIAN.)
);
#259228=(
NAMED_UNIT(*)
SI_UNIT($,.STERADIAN.)
SOLID_ANGLE_UNIT()
);
#259230=SHAPE_DEFINITION_REPRESENTATION(#259251,#259370);
#259251=PRODUCT_DEFINITION_SHAPE('',$,#259392);
#259370=SHAPE_REPRESENTATION('',(#25392),#259204);
#259390=PRODUCT_DEFINITION_CONTEXT('part definition',#259455,'design');
#259392=PRODUCT_DEFINITION('Casing','Casing',#259413,#259390);
#259413=PRODUCT_DEFINITION_FORMATION('',$,#259458);
#259455=APPLICATION_CONTEXT(
'Core Data for Automotive Mechanical Design Process');
#259456=PRODUCT_CONTEXT('part definition',#259455,'mechanical');
#259458=PRODUCT('Casing','Casing',$,(#259456));
#259479=PRESENTATION_STYLE_ASSIGNMENT((#259494));
#259494=SURFACE_STYLE_USAGE(.BOTH.,#259509);
#259509=SURFACE_SIDE_STYLE('',(#259524));
#259524=SURFACE_STYLE_FILL_AREA(#259539);
#259539=FILL_AREA_STYLE('Casing dark blue',(#259554));
#259554=FILL_AREA_STYLE_COLOUR('Casing dark blue',#259569);
#259569=COLOUR_RGB('Casing dark blue',0.0901960784313725,0.270588235294118,
0.513725490196078);
ENDSEC;
END-ISO-10303-21;
